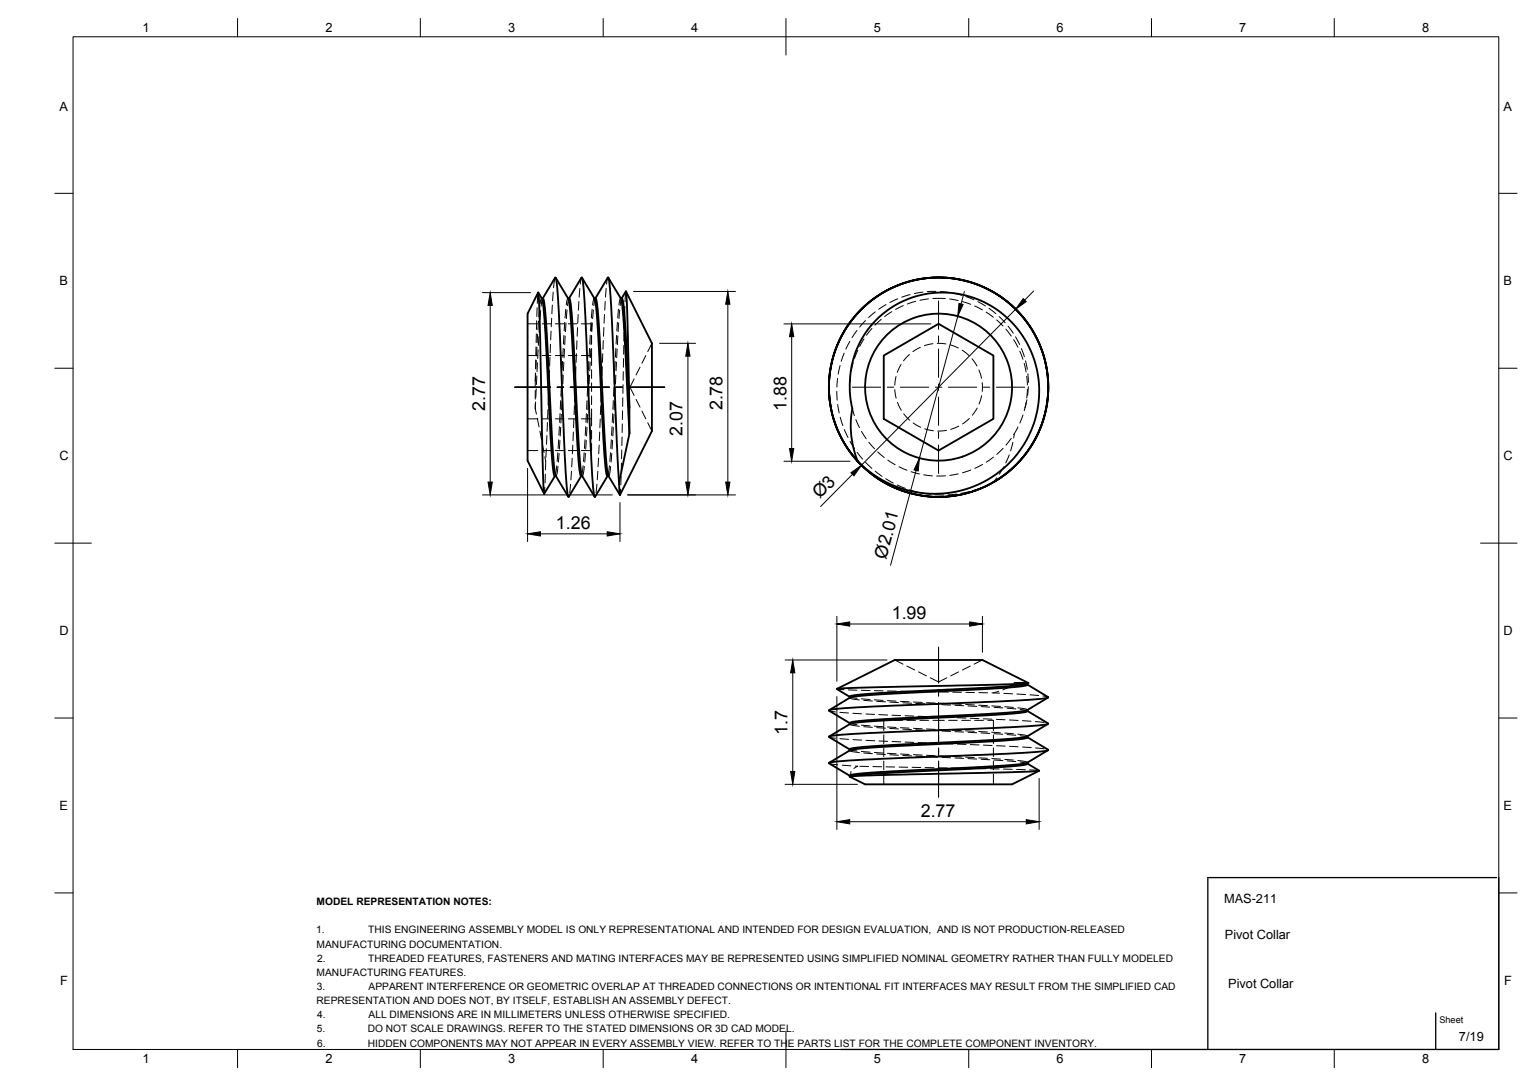
ISO-10303-21;
HEADER;
FILE_DESCRIPTION(
 (''),
 '2;1');
FILE_NAME ( 'Pivot Collar.step', '2026-10-05T20:07:59+06:00', ( '' ), ( '' ), 'STEP AP214', 'Unspecified', '' );
FILE_SCHEMA (('AUTOMOTIVE_DESIGN { 1 0 10303 214 3 1 1 }'));
ENDSEC;
DATA;
#10=MECHANICAL_DESIGN_GEOMETRIC_PRESENTATION_REPRESENTATION('',(#323),#196741);
#313=CONICAL_SURFACE('',#8812,0.119992720241923,1.10714871779409) ;
#314=CONICAL_SURFACE('',#8814,0.239985440483837,1.10714871779409) ;
#315=CONICAL_SURFACE('',#8815,0.199999999999988,1.10714871779409) ;
#323=STYLED_ITEM('',(#196765),#342) ;
#342=MANIFOLD_SOLID_BREP('Pivot Collar',#8719) ;
#369=PLANE('',#8817) ;
#370=PLANE('',#8818) ;
#371=PLANE('',#8819) ;
#372=PLANE('',#8820) ;
#373=PLANE('',#8821) ;
#374=PLANE('',#8822) ;
#375=PLANE('',#8823) ;
#376=PLANE('',#8824) ;
#564=FACE_BOUND('',#1412,.T.) ;
#631=CIRCLE('',#8806,1.21492637222366) ;
#632=CIRCLE('',#8811,1.21492629244945) ;
#633=CIRCLE('',#8813,0.599963601209611) ;
#634=CIRCLE('',#8816,1.00467112588555) ;
#832=B_SPLINE_SURFACE_WITH_KNOTS('',1,3,((#81592,#81593,#81594,#81595,#81596,
#81597,#81598,#81599,#81600,#81601,#81602,#81603,#81604,#81605,#81606,#81607,
#81608,#81609,#81610,#81611,#81612,#81613,#81614,#81615,#81616,#81617,#81618,
#81619,#81620,#81621,#81622,#81623,#81624,#81625,#81626,#81627,#81628,#81629,
#81630,#81631,#81632,#81633,#81634,#81635,#81636,#81637,#81638,#81639,#81640,
#81641,#81642,#81643,#81644,#81645,#81646,#81647,#81648,#81649,#81650,#81651,
#81652,#81653,#81654,#81655,#81656,#81657,#81658,#81659,#81660,#81661,#81662,
#81663,#81664,#81665,#81666,#81667,#81668,#81669,#81670,#81671,#81672,#81673,
#81674,#81675,#81676,#81677,#81678,#81679,#81680,#81681,#81682,#81683,#81684,
#81685,#81686,#81687,#81688,#81689,#81690,#81691,#81692,#81693,#81694,#81695,
#81696,#81697,#81698,#81699,#81700,#81701,#81702,#81703,#81704,#81705,#81706,
#81707,#81708,#81709,#81710,#81711,#81712,#81713,#81714,#81715,#81716,#81717,
#81718,#81719,#81720,#81721,#81722,#81723,#81724,#81725,#81726,#81727,#81728,
#81729,#81730,#81731,#81732,#81733,#81734,#81735,#81736,#81737,#81738,#81739,
#81740,#81741,#81742,#81743,#81744,#81745,#81746,#81747,#81748,#81749,#81750,
#81751,#81752,#81753,#81754,#81755,#81756,#81757,#81758,#81759,#81760,#81761,
#81762,#81763,#81764,#81765,#81766,#81767,#81768,#81769,#81770,#81771,#81772,
#81773,#81774,#81775,#81776,#81777,#81778,#81779,#81780,#81781,#81782,#81783,
#81784,#81785,#81786,#81787,#81788,#81789,#81790,#81791,#81792,#81793,#81794,
#81795,#81796,#81797,#81798,#81799,#81800,#81801,#81802,#81803,#81804,#81805,
#81806,#81807,#81808,#81809,#81810,#81811,#81812,#81813,#81814,#81815,#81816,
#81817,#81818,#81819,#81820,#81821,#81822,#81823,#81824,#81825,#81826,#81827,
#81828,#81829,#81830,#81831,#81832,#81833,#81834,#81835,#81836,#81837,#81838,
#81839,#81840,#81841,#81842,#81843,#81844,#81845,#81846,#81847,#81848,#81849,
#81850,#81851,#81852,#81853,#81854,#81855,#81856,#81857,#81858,#81859,#81860,
#81861,#81862,#81863,#81864,#81865,#81866,#81867,#81868,#81869,#81870,#81871,
#81872,#81873,#81874,#81875,#81876,#81877,#81878,#81879,#81880,#81881,#81882,
#81883,#81884,#81885,#81886,#81887,#81888,#81889,#81890,#81891,#81892,#81893,
#81894,#81895,#81896,#81897,#81898,#81899,#81900,#81901,#81902,#81903,#81904,
#81905,#81906,#81907,#81908,#81909,#81910,#81911,#81912,#81913,#81914,#81915,
#81916,#81917,#81918,#81919,#81920,#81921,#81922,#81923,#81924,#81925,#81926,
#81927,#81928,#81929,#81930,#81931,#81932,#81933,#81934,#81935,#81936,#81937,
#81938,#81939,#81940,#81941,#81942,#81943,#81944,#81945,#81946,#81947,#81948,
#81949,#81950,#81951,#81952,#81953,#81954,#81955,#81956,#81957,#81958,#81959,
#81960,#81961,#81962,#81963,#81964,#81965,#81966,#81967,#81968,#81969,#81970,
#81971,#81972,#81973,#81974,#81975,#81976,#81977,#81978,#81979,#81980,#81981,
#81982,#81983,#81984,#81985,#81986,#81987,#81988,#81989,#81990,#81991,#81992,
#81993,#81994,#81995,#81996,#81997,#81998,#81999,#82000,#82001,#82002,#82003,
#82004,#82005,#82006,#82007,#82008,#82009,#82010,#82011,#82012,#82013,#82014,
#82015,#82016,#82017,#82018,#82019,#82020,#82021,#82022,#82023,#82024,#82025,
#82026,#82027,#82028,#82029,#82030,#82031,#82032,#82033,#82034,#82035,#82036,
#82037,#82038,#82039,#82040,#82041,#82042,#82043,#82044,#82045,#82046,#82047,
#82048,#82049,#82050,#82051,#82052,#82053,#82054,#82055,#82056,#82057,#82058,
#82059,#82060,#82061,#82062,#82063,#82064,#82065,#82066,#82067,#82068,#82069,
#82070,#82071,#82072,#82073,#82074,#82075,#82076,#82077,#82078,#82079,#82080,
#82081,#82082,#82083,#82084,#82085,#82086,#82087,#82088,#82089,#82090,#82091,
#82092,#82093,#82094,#82095,#82096,#82097,#82098,#82099,#82100,#82101,#82102,
#82103,#82104,#82105,#82106,#82107,#82108,#82109,#82110,#82111,#82112,#82113,
#82114,#82115,#82116,#82117,#82118,#82119,#82120,#82121,#82122,#82123,#82124,
#82125,#82126,#82127,#82128,#82129,#82130,#82131,#82132,#82133,#82134,#82135,
#82136,#82137,#82138,#82139,#82140,#82141,#82142,#82143,#82144,#82145,#82146,
#82147,#82148,#82149,#82150,#82151,#82152,#82153,#82154,#82155,#82156,#82157,
#82158,#82159,#82160,#82161,#82162,#82163,#82164,#82165,#82166,#82167,#82168,
#82169,#82170,#82171,#82172,#82173,#82174,#82175,#82176,#82177,#82178,#82179,
#82180,#82181,#82182,#82183,#82184,#82185,#82186,#82187,#82188,#82189,#82190,
#82191,#82192,#82193,#82194,#82195,#82196,#82197,#82198,#82199,#82200,#82201,
#82202,#82203,#82204,#82205,#82206,#82207,#82208,#82209,#82210,#82211,#82212,
#82213,#82214,#82215,#82216,#82217,#82218,#82219,#82220,#82221,#82222,#82223,
#82224,#82225,#82226,#82227,#82228,#82229,#82230,#82231,#82232,#82233,#82234,
#82235,#82236,#82237,#82238,#82239,#82240,#82241,#82242,#82243,#82244,#82245,
#82246,#82247,#82248,#82249,#82250,#82251,#82252,#82253,#82254,#82255,#82256,
#82257,#82258,#82259,#82260,#82261,#82262,#82263,#82264,#82265,#82266,#82267,
#82268,#82269,#82270,#82271,#82272,#82273,#82274,#82275,#82276,#82277,#82278,
#82279,#82280,#82281,#82282,#82283,#82284,#82285,#82286,#82287,#82288,#82289,
#82290,#82291,#82292,#82293,#82294,#82295,#82296,#82297,#82298,#82299,#82300,
#82301,#82302,#82303,#82304,#82305,#82306,#82307,#82308,#82309,#82310,#82311,
#82312,#82313,#82314,#82315,#82316,#82317,#82318,#82319,#82320,#82321,#82322,
#82323,#82324,#82325,#82326,#82327,#82328,#82329,#82330,#82331,#82332,#82333,
#82334,#82335,#82336,#82337,#82338,#82339,#82340,#82341,#82342,#82343,#82344,
#82345,#82346,#82347,#82348,#82349,#82350,#82351,#82352,#82353,#82354,#82355,
#82356,#82357,#82358,#82359,#82360,#82361,#82362,#82363,#82364,#82365,#82366,
#82367,#82368,#82369,#82370,#82371,#82372,#82373,#82374,#82375,#82376,#82377,
#82378,#82379,#82380,#82381,#82382,#82383,#82384,#82385,#82386,#82387,#82388,
#82389,#82390,#82391,#82392,#82393,#82394,#82395,#82396,#82397,#82398,#82399,
#82400,#82401,#82402,#82403,#82404,#82405,#82406,#82407,#82408,#82409,#82410,
#82411,#82412,#82413,#82414,#82415,#82416,#82417,#82418,#82419,#82420,#82421,
#82422,#82423,#82424,#82425,#82426,#82427,#82428,#82429,#82430,#82431,#82432,
#82433,#82434,#82435,#82436,#82437,#82438,#82439,#82440,#82441,#82442,#82443,
#82444,#82445,#82446,#82447,#82448,#82449,#82450,#82451,#82452,#82453,#82454,
#82455,#82456,#82457,#82458,#82459,#82460,#82461,#82462,#82463,#82464,#82465,
#82466,#82467,#82468,#82469,#82470,#82471,#82472,#82473,#82474,#82475,#82476,
#82477,#82478,#82479,#82480,#82481,#82482,#82483,#82484,#82485,#82486,#82487,
#82488,#82489,#82490,#82491,#82492,#82493,#82494,#82495,#82496,#82497,#82498,
#82499,#82500,#82501,#82502,#82503,#82504,#82505,#82506,#82507,#82508,#82509,
#82510,#82511,#82512,#82513,#82514,#82515,#82516,#82517,#82518,#82519,#82520,
#82521,#82522,#82523,#82524,#82525,#82526,#82527,#82528,#82529,#82530,#82531,
#82532,#82533,#82534,#82535,#82536,#82537,#82538,#82539,#82540,#82541,#82542,
#82543,#82544,#82545,#82546,#82547,#82548,#82549,#82550,#82551,#82552,#82553,
#82554,#82555,#82556,#82557,#82558,#82559,#82560,#82561,#82562,#82563,#82564,
#82565,#82566,#82567,#82568,#82569,#82570,#82571,#82572,#82573,#82574,#82575,
#82576,#82577,#82578,#82579,#82580,#82581,#82582,#82583,#82584,#82585,#82586,
#82587,#82588,#82589,#82590,#82591,#82592,#82593,#82594,#82595,#82596,#82597,
#82598,#82599,#82600,#82601,#82602,#82603,#82604,#82605,#82606,#82607,#82608,
#82609,#82610,#82611,#82612,#82613,#82614,#82615,#82616,#82617,#82618,#82619,
#82620,#82621,#82622,#82623,#82624,#82625,#82626,#82627,#82628,#82629,#82630,
#82631,#82632,#82633,#82634,#82635,#82636,#82637,#82638,#82639,#82640,#82641,
#82642,#82643,#82644,#82645,#82646,#82647,#82648,#82649,#82650,#82651,#82652,
#82653,#82654,#82655,#82656,#82657,#82658,#82659,#82660,#82661,#82662,#82663,
#82664,#82665,#82666,#82667,#82668,#82669,#82670,#82671,#82672,#82673,#82674,
#82675,#82676,#82677,#82678,#82679,#82680,#82681,#82682,#82683,#82684,#82685,
#82686,#82687,#82688,#82689,#82690,#82691,#82692,#82693,#82694,#82695,#82696,
#82697,#82698,#82699,#82700,#82701,#82702,#82703,#82704,#82705,#82706,#82707,
#82708,#82709,#82710,#82711,#82712,#82713,#82714,#82715,#82716,#82717,#82718,
#82719,#82720,#82721,#82722,#82723,#82724,#82725,#82726,#82727,#82728,#82729,
#82730,#82731,#82732,#82733,#82734,#82735,#82736,#82737,#82738,#82739,#82740,
#82741,#82742,#82743,#82744,#82745,#82746,#82747,#82748,#82749,#82750,#82751,
#82752,#82753,#82754,#82755,#82756,#82757,#82758,#82759,#82760,#82761,#82762,
#82763,#82764,#82765,#82766,#82767,#82768,#82769,#82770,#82771,#82772,#82773,
#82774,#82775,#82776,#82777,#82778,#82779,#82780,#82781,#82782,#82783,#82784,
#82785,#82786,#82787,#82788,#82789,#82790,#82791,#82792,#82793,#82794,#82795,
#82796,#82797,#82798,#82799,#82800,#82801,#82802,#82803,#82804,#82805,#82806,
#82807,#82808,#82809,#82810,#82811,#82812,#82813,#82814,#82815,#82816,#82817,
#82818,#82819,#82820,#82821,#82822,#82823,#82824,#82825,#82826,#82827,#82828,
#82829,#82830,#82831,#82832,#82833,#82834,#82835,#82836,#82837,#82838,#82839,
#82840,#82841,#82842,#82843,#82844,#82845,#82846,#82847,#82848,#82849,#82850,
#82851,#82852,#82853,#82854,#82855,#82856,#82857,#82858,#82859,#82860,#82861,
#82862,#82863,#82864,#82865,#82866,#82867,#82868,#82869,#82870,#82871,#82872,
#82873,#82874,#82875,#82876,#82877,#82878,#82879,#82880,#82881,#82882,#82883,
#82884,#82885,#82886,#82887,#82888,#82889,#82890,#82891,#82892,#82893,#82894,
#82895,#82896,#82897,#82898,#82899,#82900,#82901,#82902,#82903,#82904,#82905,
#82906,#82907,#82908,#82909,#82910,#82911,#82912,#82913,#82914,#82915,#82916,
#82917,#82918,#82919,#82920,#82921,#82922,#82923,#82924,#82925,#82926,#82927,
#82928,#82929,#82930,#82931,#82932,#82933,#82934,#82935,#82936,#82937,#82938,
#82939,#82940,#82941,#82942,#82943,#82944,#82945,#82946,#82947,#82948,#82949,
#82950,#82951,#82952,#82953,#82954,#82955,#82956,#82957,#82958,#82959,#82960,
#82961,#82962,#82963,#82964,#82965,#82966,#82967,#82968,#82969,#82970,#82971,
#82972,#82973,#82974,#82975,#82976,#82977,#82978,#82979,#82980,#82981,#82982,
#82983,#82984,#82985,#82986,#82987,#82988,#82989,#82990,#82991,#82992,#82993,
#82994,#82995,#82996,#82997,#82998,#82999,#83000,#83001,#83002,#83003,#83004,
#83005,#83006,#83007,#83008,#83009,#83010,#83011,#83012,#83013,#83014,#83015,
#83016,#83017,#83018,#83019,#83020,#83021,#83022,#83023,#83024,#83025,#83026,
#83027,#83028,#83029,#83030,#83031,#83032,#83033,#83034,#83035,#83036,#83037,
#83038,#83039,#83040,#83041,#83042,#83043,#83044,#83045,#83046,#83047,#83048,
#83049,#83050,#83051,#83052,#83053,#83054,#83055,#83056,#83057,#83058,#83059,
#83060,#83061,#83062,#83063,#83064,#83065,#83066,#83067,#83068,#83069,#83070,
#83071,#83072,#83073,#83074,#83075,#83076,#83077,#83078,#83079,#83080,#83081,
#83082,#83083,#83084,#83085,#83086,#83087,#83088,#83089,#83090,#83091,#83092,
#83093,#83094,#83095,#83096,#83097,#83098,#83099,#83100,#83101,#83102,#83103,
#83104,#83105,#83106,#83107,#83108,#83109,#83110,#83111,#83112,#83113,#83114,
#83115,#83116,#83117,#83118,#83119,#83120,#83121,#83122,#83123,#83124,#83125,
#83126,#83127,#83128,#83129,#83130,#83131,#83132,#83133,#83134,#83135,#83136,
#83137,#83138,#83139,#83140,#83141,#83142,#83143,#83144,#83145,#83146,#83147,
#83148,#83149,#83150,#83151,#83152,#83153,#83154,#83155,#83156,#83157,#83158,
#83159,#83160,#83161,#83162,#83163,#83164,#83165,#83166,#83167,#83168,#83169,
#83170,#83171,#83172,#83173,#83174,#83175,#83176,#83177,#83178,#83179,#83180,
#83181,#83182,#83183,#83184,#83185,#83186,#83187,#83188,#83189,#83190,#83191,
#83192,#83193,#83194,#83195,#83196,#83197,#83198,#83199,#83200,#83201,#83202,
#83203,#83204,#83205,#83206,#83207,#83208,#83209,#83210,#83211,#83212,#83213,
#83214,#83215,#83216,#83217,#83218,#83219,#83220,#83221,#83222,#83223,#83224,
#83225,#83226,#83227,#83228,#83229,#83230,#83231,#83232,#83233,#83234,#83235,
#83236,#83237,#83238,#83239,#83240,#83241,#83242,#83243,#83244,#83245,#83246,
#83247,#83248,#83249,#83250,#83251,#83252,#83253,#83254,#83255,#83256,#83257,
#83258,#83259,#83260,#83261,#83262,#83263,#83264,#83265,#83266,#83267,#83268,
#83269,#83270,#83271,#83272,#83273,#83274,#83275,#83276,#83277,#83278,#83279,
#83280,#83281,#83282,#83283,#83284,#83285,#83286,#83287,#83288,#83289,#83290,
#83291,#83292,#83293,#83294,#83295,#83296,#83297,#83298,#83299,#83300,#83301,
#83302,#83303,#83304,#83305,#83306,#83307,#83308,#83309,#83310,#83311,#83312,
#83313,#83314,#83315,#83316,#83317,#83318,#83319,#83320,#83321,#83322,#83323,
#83324,#83325,#83326,#83327,#83328,#83329,#83330,#83331,#83332,#83333,#83334,
#83335,#83336,#83337,#83338,#83339,#83340,#83341,#83342,#83343,#83344,#83345,
#83346,#83347,#83348,#83349,#83350,#83351,#83352,#83353,#83354,#83355,#83356,
#83357,#83358,#83359,#83360,#83361,#83362,#83363,#83364,#83365,#83366,#83367,
#83368,#83369,#83370,#83371,#83372,#83373,#83374,#83375,#83376,#83377,#83378,
#83379,#83380,#83381,#83382,#83383,#83384,#83385,#83386,#83387,#83388,#83389,
#83390,#83391,#83392,#83393,#83394,#83395,#83396,#83397,#83398,#83399,#83400,
#83401,#83402,#83403,#83404,#83405,#83406,#83407,#83408,#83409,#83410,#83411,
#83412,#83413,#83414,#83415,#83416,#83417,#83418,#83419,#83420,#83421,#83422,
#83423,#83424,#83425,#83426,#83427,#83428,#83429,#83430,#83431,#83432,#83433,
#83434,#83435,#83436,#83437,#83438,#83439,#83440,#83441,#83442,#83443,#83444,
#83445,#83446,#83447,#83448,#83449,#83450,#83451,#83452,#83453,#83454,#83455,
#83456,#83457,#83458,#83459,#83460,#83461,#83462,#83463,#83464,#83465,#83466,
#83467,#83468,#83469,#83470,#83471,#83472,#83473,#83474,#83475,#83476,#83477,
#83478,#83479,#83480,#83481,#83482,#83483,#83484,#83485,#83486,#83487,#83488,
#83489,#83490,#83491,#83492,#83493,#83494,#83495,#83496,#83497,#83498,#83499,
#83500,#83501,#83502,#83503,#83504,#83505,#83506,#83507,#83508,#83509,#83510,
#83511,#83512,#83513,#83514,#83515,#83516,#83517,#83518,#83519,#83520,#83521,
#83522,#83523,#83524,#83525,#83526,#83527,#83528,#83529,#83530,#83531,#83532,
#83533,#83534,#83535,#83536,#83537,#83538,#83539,#83540,#83541,#83542,#83543,
#83544,#83545,#83546,#83547,#83548,#83549,#83550,#83551,#83552,#83553,#83554,
#83555,#83556,#83557,#83558,#83559,#83560,#83561,#83562,#83563,#83564,#83565,
#83566,#83567,#83568,#83569,#83570,#83571,#83572,#83573,#83574,#83575,#83576,
#83577,#83578,#83579,#83580,#83581,#83582,#83583,#83584,#83585,#83586,#83587,
#83588,#83589,#83590,#83591,#83592,#83593,#83594,#83595,#83596,#83597,#83598,
#83599,#83600,#83601,#83602,#83603,#83604,#83605,#83606,#83607,#83608,#83609,
#83610,#83611,#83612,#83613,#83614,#83615,#83616,#83617,#83618,#83619,#83620,
#83621,#83622,#83623,#83624,#83625,#83626,#83627,#83628,#83629,#83630,#83631,
#83632,#83633,#83634,#83635,#83636,#83637,#83638,#83639,#83640,#83641,#83642,
#83643,#83644,#83645,#83646,#83647,#83648,#83649,#83650,#83651,#83652,#83653,
#83654,#83655,#83656,#83657,#83658,#83659,#83660,#83661,#83662,#83663,#83664,
#83665,#83666,#83667,#83668,#83669,#83670,#83671,#83672,#83673,#83674,#83675,
#83676,#83677,#83678,#83679,#83680,#83681,#83682,#83683,#83684,#83685,#83686,
#83687,#83688,#83689,#83690,#83691,#83692,#83693,#83694,#83695,#83696,#83697,
#83698,#83699,#83700,#83701,#83702,#83703,#83704,#83705,#83706,#83707,#83708,
#83709,#83710,#83711,#83712,#83713,#83714,#83715,#83716,#83717,#83718,#83719,
#83720,#83721,#83722,#83723,#83724,#83725,#83726,#83727,#83728,#83729,#83730,
#83731,#83732,#83733,#83734,#83735,#83736,#83737,#83738,#83739,#83740,#83741,
#83742,#83743,#83744,#83745,#83746,#83747,#83748,#83749,#83750,#83751,#83752,
#83753,#83754,#83755,#83756,#83757,#83758,#83759,#83760,#83761,#83762,#83763,
#83764,#83765,#83766,#83767,#83768,#83769,#83770,#83771,#83772,#83773,#83774,
#83775,#83776,#83777,#83778,#83779,#83780,#83781,#83782,#83783,#83784,#83785,
#83786,#83787,#83788,#83789,#83790,#83791,#83792,#83793,#83794,#83795,#83796,
#83797,#83798,#83799,#83800,#83801,#83802,#83803,#83804,#83805,#83806,#83807,
#83808,#83809,#83810,#83811,#83812,#83813,#83814,#83815,#83816,#83817,#83818,
#83819,#83820,#83821,#83822,#83823,#83824,#83825,#83826,#83827,#83828,#83829,
#83830,#83831,#83832,#83833,#83834,#83835,#83836,#83837,#83838,#83839,#83840,
#83841,#83842,#83843,#83844,#83845,#83846,#83847,#83848,#83849,#83850,#83851,
#83852,#83853,#83854,#83855,#83856,#83857,#83858,#83859,#83860,#83861,#83862,
#83863,#83864,#83865,#83866,#83867,#83868,#83869,#83870,#83871,#83872,#83873,
#83874,#83875,#83876,#83877,#83878,#83879,#83880,#83881,#83882,#83883,#83884,
#83885,#83886,#83887,#83888,#83889,#83890,#83891,#83892,#83893,#83894,#83895,
#83896,#83897,#83898,#83899,#83900,#83901,#83902,#83903,#83904,#83905,#83906,
#83907,#83908,#83909,#83910,#83911,#83912,#83913,#83914,#83915,#83916,#83917,
#83918,#83919,#83920,#83921,#83922,#83923,#83924,#83925,#83926,#83927,#83928,
#83929,#83930,#83931,#83932,#83933,#83934,#83935,#83936,#83937,#83938,#83939,
#83940,#83941,#83942,#83943,#83944,#83945,#83946,#83947,#83948,#83949,#83950,
#83951,#83952,#83953,#83954,#83955,#83956,#83957,#83958,#83959,#83960,#83961,
#83962,#83963,#83964,#83965,#83966,#83967,#83968,#83969,#83970,#83971,#83972,
#83973,#83974,#83975,#83976,#83977,#83978,#83979,#83980,#83981,#83982,#83983,
#83984,#83985,#83986,#83987,#83988,#83989,#83990,#83991,#83992,#83993,#83994,
#83995,#83996,#83997,#83998,#83999,#84000,#84001,#84002,#84003,#84004,#84005,
#84006,#84007,#84008,#84009,#84010,#84011,#84012,#84013,#84014,#84015,#84016,
#84017,#84018,#84019,#84020,#84021,#84022,#84023,#84024,#84025,#84026,#84027,
#84028,#84029,#84030,#84031,#84032,#84033,#84034,#84035,#84036,#84037,#84038,
#84039,#84040,#84041,#84042,#84043,#84044,#84045,#84046,#84047,#84048,#84049,
#84050,#84051,#84052,#84053,#84054,#84055,#84056,#84057,#84058,#84059,#84060,
#84061,#84062,#84063,#84064,#84065,#84066,#84067,#84068,#84069,#84070,#84071,
#84072,#84073,#84074,#84075,#84076,#84077,#84078,#84079,#84080,#84081,#84082,
#84083,#84084,#84085,#84086,#84087,#84088,#84089,#84090,#84091,#84092,#84093,
#84094,#84095,#84096,#84097,#84098,#84099,#84100,#84101,#84102,#84103,#84104,
#84105,#84106,#84107,#84108,#84109,#84110,#84111,#84112,#84113,#84114,#84115,
#84116,#84117,#84118,#84119,#84120,#84121,#84122,#84123,#84124,#84125,#84126,
#84127,#84128,#84129,#84130,#84131,#84132,#84133,#84134,#84135,#84136,#84137,
#84138,#84139,#84140,#84141,#84142,#84143,#84144,#84145,#84146,#84147,#84148,
#84149,#84150,#84151,#84152,#84153,#84154,#84155,#84156,#84157,#84158,#84159,
#84160,#84161,#84162,#84163,#84164,#84165,#84166,#84167,#84168,#84169,#84170,
#84171,#84172,#84173,#84174,#84175,#84176,#84177,#84178,#84179,#84180,#84181,
#84182,#84183,#84184,#84185,#84186,#84187,#84188,#84189,#84190,#84191,#84192,
#84193,#84194,#84195,#84196,#84197,#84198,#84199,#84200,#84201,#84202,#84203,
#84204,#84205,#84206,#84207,#84208,#84209,#84210,#84211,#84212,#84213,#84214,
#84215,#84216,#84217,#84218,#84219,#84220,#84221,#84222,#84223,#84224,#84225,
#84226,#84227,#84228,#84229,#84230,#84231,#84232,#84233,#84234,#84235,#84236,
#84237,#84238,#84239,#84240,#84241,#84242,#84243,#84244,#84245,#84246,#84247,
#84248,#84249,#84250,#84251,#84252,#84253,#84254,#84255,#84256,#84257,#84258,
#84259,#84260,#84261,#84262,#84263,#84264,#84265,#84266,#84267,#84268,#84269,
#84270,#84271,#84272,#84273,#84274,#84275,#84276,#84277,#84278,#84279,#84280,
#84281,#84282,#84283,#84284,#84285,#84286,#84287,#84288,#84289,#84290,#84291,
#84292,#84293,#84294,#84295,#84296,#84297,#84298,#84299,#84300,#84301,#84302,
#84303,#84304,#84305,#84306,#84307,#84308,#84309,#84310,#84311,#84312,#84313,
#84314,#84315,#84316,#84317,#84318,#84319,#84320,#84321,#84322,#84323,#84324,
#84325,#84326,#84327,#84328,#84329,#84330,#84331,#84332,#84333,#84334,#84335,
#84336,#84337,#84338,#84339,#84340,#84341,#84342,#84343,#84344,#84345,#84346,
#84347,#84348,#84349,#84350,#84351,#84352,#84353,#84354,#84355,#84356,#84357,
#84358,#84359,#84360,#84361,#84362,#84363,#84364,#84365,#84366,#84367,#84368,
#84369,#84370,#84371,#84372,#84373,#84374,#84375,#84376,#84377,#84378,#84379,
#84380,#84381,#84382,#84383,#84384,#84385,#84386,#84387,#84388,#84389,#84390,
#84391,#84392,#84393,#84394,#84395,#84396,#84397,#84398,#84399,#84400,#84401,
#84402,#84403,#84404,#84405,#84406,#84407,#84408,#84409,#84410,#84411,#84412,
#84413,#84414,#84415,#84416,#84417,#84418,#84419,#84420,#84421,#84422,#84423,
#84424,#84425,#84426,#84427,#84428,#84429,#84430,#84431,#84432,#84433,#84434,
#84435,#84436,#84437,#84438,#84439,#84440,#84441,#84442,#84443,#84444,#84445,
#84446,#84447,#84448,#84449,#84450,#84451,#84452,#84453,#84454,#84455,#84456,
#84457,#84458,#84459,#84460,#84461,#84462,#84463,#84464,#84465,#84466,#84467,
#84468,#84469,#84470,#84471,#84472,#84473,#84474,#84475,#84476,#84477,#84478,
#84479,#84480,#84481,#84482,#84483,#84484,#84485,#84486,#84487,#84488,#84489,
#84490,#84491,#84492,#84493,#84494,#84495,#84496,#84497,#84498,#84499,#84500,
#84501,#84502,#84503,#84504,#84505,#84506,#84507,#84508,#84509,#84510,#84511,
#84512,#84513,#84514,#84515,#84516,#84517,#84518,#84519,#84520,#84521,#84522,
#84523,#84524,#84525,#84526,#84527,#84528,#84529,#84530,#84531,#84532,#84533,
#84534,#84535,#84536,#84537,#84538,#84539,#84540,#84541,#84542,#84543,#84544,
#84545,#84546,#84547,#84548,#84549,#84550,#84551,#84552,#84553,#84554,#84555,
#84556,#84557,#84558,#84559,#84560,#84561,#84562,#84563,#84564,#84565,#84566,
#84567,#84568,#84569,#84570,#84571,#84572,#84573,#84574,#84575,#84576,#84577,
#84578,#84579,#84580,#84581,#84582,#84583,#84584,#84585,#84586,#84587,#84588,
#84589,#84590,#84591,#84592,#84593,#84594,#84595,#84596,#84597,#84598,#84599,
#84600,#84601,#84602,#84603,#84604,#84605,#84606,#84607,#84608,#84609,#84610,
#84611,#84612,#84613,#84614,#84615,#84616,#84617,#84618,#84619,#84620,#84621,
#84622,#84623,#84624,#84625,#84626,#84627,#84628,#84629,#84630,#84631,#84632,
#84633,#84634,#84635,#84636,#84637,#84638,#84639,#84640,#84641,#84642,#84643,
#84644,#84645,#84646,#84647,#84648,#84649,#84650,#84651,#84652,#84653,#84654,
#84655,#84656,#84657,#84658,#84659,#84660,#84661,#84662,#84663,#84664,#84665,
#84666,#84667,#84668,#84669,#84670,#84671,#84672,#84673,#84674,#84675,#84676,
#84677,#84678,#84679,#84680,#84681,#84682,#84683,#84684,#84685,#84686,#84687,
#84688,#84689,#84690,#84691,#84692,#84693,#84694,#84695,#84696,#84697,#84698,
#84699,#84700,#84701,#84702,#84703,#84704,#84705,#84706,#84707,#84708,#84709,
#84710,#84711,#84712,#84713,#84714,#84715,#84716,#84717,#84718,#84719,#84720,
#84721,#84722,#84723,#84724,#84725,#84726,#84727,#84728,#84729,#84730,#84731,
#84732,#84733,#84734,#84735,#84736,#84737,#84738,#84739,#84740,#84741,#84742,
#84743,#84744,#84745,#84746,#84747,#84748,#84749,#84750,#84751,#84752,#84753,
#84754,#84755,#84756,#84757,#84758,#84759,#84760,#84761,#84762,#84763,#84764,
#84765,#84766,#84767,#84768,#84769,#84770,#84771,#84772,#84773,#84774,#84775,
#84776,#84777,#84778,#84779,#84780,#84781,#84782,#84783,#84784,#84785,#84786,
#84787,#84788,#84789,#84790,#84791,#84792,#84793,#84794,#84795,#84796,#84797,
#84798,#84799,#84800,#84801,#84802,#84803,#84804,#84805,#84806,#84807,#84808,
#84809,#84810,#84811,#84812,#84813,#84814,#84815,#84816,#84817,#84818,#84819,
#84820,#84821,#84822,#84823,#84824,#84825,#84826,#84827,#84828,#84829,#84830,
#84831,#84832,#84833,#84834,#84835,#84836,#84837,#84838,#84839,#84840,#84841,
#84842,#84843,#84844,#84845,#84846,#84847,#84848,#84849,#84850,#84851,#84852,
#84853,#84854,#84855,#84856,#84857,#84858,#84859,#84860,#84861,#84862,#84863,
#84864,#84865,#84866,#84867,#84868,#84869,#84870,#84871,#84872,#84873,#84874,
#84875,#84876,#84877,#84878,#84879,#84880,#84881,#84882,#84883,#84884,#84885,
#84886,#84887,#84888,#84889,#84890,#84891,#84892,#84893,#84894,#84895,#84896,
#84897,#84898,#84899,#84900,#84901,#84902,#84903,#84904,#84905,#84906,#84907,
#84908,#84909,#84910,#84911,#84912,#84913,#84914,#84915,#84916,#84917,#84918,
#84919,#84920,#84921,#84922,#84923,#84924,#84925,#84926,#84927,#84928,#84929,
#84930,#84931,#84932,#84933,#84934,#84935,#84936,#84937,#84938,#84939,#84940,
#84941,#84942,#84943,#84944,#84945,#84946,#84947,#84948,#84949,#84950,#84951,
#84952,#84953,#84954,#84955,#84956,#84957,#84958,#84959,#84960,#84961,#84962,
#84963,#84964,#84965,#84966,#84967,#84968,#84969,#84970,#84971,#84972,#84973,
#84974,#84975,#84976,#84977,#84978,#84979,#84980,#84981,#84982,#84983,#84984,
#84985,#84986,#84987,#84988,#84989,#84990,#84991,#84992,#84993,#84994,#84995,
#84996,#84997,#84998,#84999,#85000,#85001,#85002,#85003,#85004,#85005,#85006,
#85007,#85008,#85009,#85010,#85011,#85012,#85013,#85014,#85015,#85016,#85017,
#85018,#85019,#85020,#85021,#85022,#85023,#85024,#85025,#85026,#85027,#85028,
#85029,#85030,#85031,#85032,#85033,#85034,#85035,#85036,#85037,#85038,#85039,
#85040,#85041,#85042,#85043,#85044,#85045,#85046,#85047,#85048,#85049,#85050,
#85051,#85052,#85053,#85054,#85055,#85056,#85057,#85058,#85059,#85060,#85061,
#85062,#85063,#85064,#85065,#85066,#85067,#85068,#85069,#85070,#85071,#85072,
#85073,#85074,#85075,#85076),(#85077,#85078,#85079,#85080,#85081,#85082,
#85083,#85084,#85085,#85086,#85087,#85088,#85089,#85090,#85091,#85092,#85093,
#85094,#85095,#85096,#85097,#85098,#85099,#85100,#85101,#85102,#85103,#85104,
#85105,#85106,#85107,#85108,#85109,#85110,#85111,#85112,#85113,#85114,#85115,
#85116,#85117,#85118,#85119,#85120,#85121,#85122,#85123,#85124,#85125,#85126,
#85127,#85128,#85129,#85130,#85131,#85132,#85133,#85134,#85135,#85136,#85137,
#85138,#85139,#85140,#85141,#85142,#85143,#85144,#85145,#85146,#85147,#85148,
#85149,#85150,#85151,#85152,#85153,#85154,#85155,#85156,#85157,#85158,#85159,
#85160,#85161,#85162,#85163,#85164,#85165,#85166,#85167,#85168,#85169,#85170,
#85171,#85172,#85173,#85174,#85175,#85176,#85177,#85178,#85179,#85180,#85181,
#85182,#85183,#85184,#85185,#85186,#85187,#85188,#85189,#85190,#85191,#85192,
#85193,#85194,#85195,#85196,#85197,#85198,#85199,#85200,#85201,#85202,#85203,
#85204,#85205,#85206,#85207,#85208,#85209,#85210,#85211,#85212,#85213,#85214,
#85215,#85216,#85217,#85218,#85219,#85220,#85221,#85222,#85223,#85224,#85225,
#85226,#85227,#85228,#85229,#85230,#85231,#85232,#85233,#85234,#85235,#85236,
#85237,#85238,#85239,#85240,#85241,#85242,#85243,#85244,#85245,#85246,#85247,
#85248,#85249,#85250,#85251,#85252,#85253,#85254,#85255,#85256,#85257,#85258,
#85259,#85260,#85261,#85262,#85263,#85264,#85265,#85266,#85267,#85268,#85269,
#85270,#85271,#85272,#85273,#85274,#85275,#85276,#85277,#85278,#85279,#85280,
#85281,#85282,#85283,#85284,#85285,#85286,#85287,#85288,#85289,#85290,#85291,
#85292,#85293,#85294,#85295,#85296,#85297,#85298,#85299,#85300,#85301,#85302,
#85303,#85304,#85305,#85306,#85307,#85308,#85309,#85310,#85311,#85312,#85313,
#85314,#85315,#85316,#85317,#85318,#85319,#85320,#85321,#85322,#85323,#85324,
#85325,#85326,#85327,#85328,#85329,#85330,#85331,#85332,#85333,#85334,#85335,
#85336,#85337,#85338,#85339,#85340,#85341,#85342,#85343,#85344,#85345,#85346,
#85347,#85348,#85349,#85350,#85351,#85352,#85353,#85354,#85355,#85356,#85357,
#85358,#85359,#85360,#85361,#85362,#85363,#85364,#85365,#85366,#85367,#85368,
#85369,#85370,#85371,#85372,#85373,#85374,#85375,#85376,#85377,#85378,#85379,
#85380,#85381,#85382,#85383,#85384,#85385,#85386,#85387,#85388,#85389,#85390,
#85391,#85392,#85393,#85394,#85395,#85396,#85397,#85398,#85399,#85400,#85401,
#85402,#85403,#85404,#85405,#85406,#85407,#85408,#85409,#85410,#85411,#85412,
#85413,#85414,#85415,#85416,#85417,#85418,#85419,#85420,#85421,#85422,#85423,
#85424,#85425,#85426,#85427,#85428,#85429,#85430,#85431,#85432,#85433,#85434,
#85435,#85436,#85437,#85438,#85439,#85440,#85441,#85442,#85443,#85444,#85445,
#85446,#85447,#85448,#85449,#85450,#85451,#85452,#85453,#85454,#85455,#85456,
#85457,#85458,#85459,#85460,#85461,#85462,#85463,#85464,#85465,#85466,#85467,
#85468,#85469,#85470,#85471,#85472,#85473,#85474,#85475,#85476,#85477,#85478,
#85479,#85480,#85481,#85482,#85483,#85484,#85485,#85486,#85487,#85488,#85489,
#85490,#85491,#85492,#85493,#85494,#85495,#85496,#85497,#85498,#85499,#85500,
#85501,#85502,#85503,#85504,#85505,#85506,#85507,#85508,#85509,#85510,#85511,
#85512,#85513,#85514,#85515,#85516,#85517,#85518,#85519,#85520,#85521,#85522,
#85523,#85524,#85525,#85526,#85527,#85528,#85529,#85530,#85531,#85532,#85533,
#85534,#85535,#85536,#85537,#85538,#85539,#85540,#85541,#85542,#85543,#85544,
#85545,#85546,#85547,#85548,#85549,#85550,#85551,#85552,#85553,#85554,#85555,
#85556,#85557,#85558,#85559,#85560,#85561,#85562,#85563,#85564,#85565,#85566,
#85567,#85568,#85569,#85570,#85571,#85572,#85573,#85574,#85575,#85576,#85577,
#85578,#85579,#85580,#85581,#85582,#85583,#85584,#85585,#85586,#85587,#85588,
#85589,#85590,#85591,#85592,#85593,#85594,#85595,#85596,#85597,#85598,#85599,
#85600,#85601,#85602,#85603,#85604,#85605,#85606,#85607,#85608,#85609,#85610,
#85611,#85612,#85613,#85614,#85615,#85616,#85617,#85618,#85619,#85620,#85621,
#85622,#85623,#85624,#85625,#85626,#85627,#85628,#85629,#85630,#85631,#85632,
#85633,#85634,#85635,#85636,#85637,#85638,#85639,#85640,#85641,#85642,#85643,
#85644,#85645,#85646,#85647,#85648,#85649,#85650,#85651,#85652,#85653,#85654,
#85655,#85656,#85657,#85658,#85659,#85660,#85661,#85662,#85663,#85664,#85665,
#85666,#85667,#85668,#85669,#85670,#85671,#85672,#85673,#85674,#85675,#85676,
#85677,#85678,#85679,#85680,#85681,#85682,#85683,#85684,#85685,#85686,#85687,
#85688,#85689,#85690,#85691,#85692,#85693,#85694,#85695,#85696,#85697,#85698,
#85699,#85700,#85701,#85702,#85703,#85704,#85705,#85706,#85707,#85708,#85709,
#85710,#85711,#85712,#85713,#85714,#85715,#85716,#85717,#85718,#85719,#85720,
#85721,#85722,#85723,#85724,#85725,#85726,#85727,#85728,#85729,#85730,#85731,
#85732,#85733,#85734,#85735,#85736,#85737,#85738,#85739,#85740,#85741,#85742,
#85743,#85744,#85745,#85746,#85747,#85748,#85749,#85750,#85751,#85752,#85753,
#85754,#85755,#85756,#85757,#85758,#85759,#85760,#85761,#85762,#85763,#85764,
#85765,#85766,#85767,#85768,#85769,#85770,#85771,#85772,#85773,#85774,#85775,
#85776,#85777,#85778,#85779,#85780,#85781,#85782,#85783,#85784,#85785,#85786,
#85787,#85788,#85789,#85790,#85791,#85792,#85793,#85794,#85795,#85796,#85797,
#85798,#85799,#85800,#85801,#85802,#85803,#85804,#85805,#85806,#85807,#85808,
#85809,#85810,#85811,#85812,#85813,#85814,#85815,#85816,#85817,#85818,#85819,
#85820,#85821,#85822,#85823,#85824,#85825,#85826,#85827,#85828,#85829,#85830,
#85831,#85832,#85833,#85834,#85835,#85836,#85837,#85838,#85839,#85840,#85841,
#85842,#85843,#85844,#85845,#85846,#85847,#85848,#85849,#85850,#85851,#85852,
#85853,#85854,#85855,#85856,#85857,#85858,#85859,#85860,#85861,#85862,#85863,
#85864,#85865,#85866,#85867,#85868,#85869,#85870,#85871,#85872,#85873,#85874,
#85875,#85876,#85877,#85878,#85879,#85880,#85881,#85882,#85883,#85884,#85885,
#85886,#85887,#85888,#85889,#85890,#85891,#85892,#85893,#85894,#85895,#85896,
#85897,#85898,#85899,#85900,#85901,#85902,#85903,#85904,#85905,#85906,#85907,
#85908,#85909,#85910,#85911,#85912,#85913,#85914,#85915,#85916,#85917,#85918,
#85919,#85920,#85921,#85922,#85923,#85924,#85925,#85926,#85927,#85928,#85929,
#85930,#85931,#85932,#85933,#85934,#85935,#85936,#85937,#85938,#85939,#85940,
#85941,#85942,#85943,#85944,#85945,#85946,#85947,#85948,#85949,#85950,#85951,
#85952,#85953,#85954,#85955,#85956,#85957,#85958,#85959,#85960,#85961,#85962,
#85963,#85964,#85965,#85966,#85967,#85968,#85969,#85970,#85971,#85972,#85973,
#85974,#85975,#85976,#85977,#85978,#85979,#85980,#85981,#85982,#85983,#85984,
#85985,#85986,#85987,#85988,#85989,#85990,#85991,#85992,#85993,#85994,#85995,
#85996,#85997,#85998,#85999,#86000,#86001,#86002,#86003,#86004,#86005,#86006,
#86007,#86008,#86009,#86010,#86011,#86012,#86013,#86014,#86015,#86016,#86017,
#86018,#86019,#86020,#86021,#86022,#86023,#86024,#86025,#86026,#86027,#86028,
#86029,#86030,#86031,#86032,#86033,#86034,#86035,#86036,#86037,#86038,#86039,
#86040,#86041,#86042,#86043,#86044,#86045,#86046,#86047,#86048,#86049,#86050,
#86051,#86052,#86053,#86054,#86055,#86056,#86057,#86058,#86059,#86060,#86061,
#86062,#86063,#86064,#86065,#86066,#86067,#86068,#86069,#86070,#86071,#86072,
#86073,#86074,#86075,#86076,#86077,#86078,#86079,#86080,#86081,#86082,#86083,
#86084,#86085,#86086,#86087,#86088,#86089,#86090,#86091,#86092,#86093,#86094,
#86095,#86096,#86097,#86098,#86099,#86100,#86101,#86102,#86103,#86104,#86105,
#86106,#86107,#86108,#86109,#86110,#86111,#86112,#86113,#86114,#86115,#86116,
#86117,#86118,#86119,#86120,#86121,#86122,#86123,#86124,#86125,#86126,#86127,
#86128,#86129,#86130,#86131,#86132,#86133,#86134,#86135,#86136,#86137,#86138,
#86139,#86140,#86141,#86142,#86143,#86144,#86145,#86146,#86147,#86148,#86149,
#86150,#86151,#86152,#86153,#86154,#86155,#86156,#86157,#86158,#86159,#86160,
#86161,#86162,#86163,#86164,#86165,#86166,#86167,#86168,#86169,#86170,#86171,
#86172,#86173,#86174,#86175,#86176,#86177,#86178,#86179,#86180,#86181,#86182,
#86183,#86184,#86185,#86186,#86187,#86188,#86189,#86190,#86191,#86192,#86193,
#86194,#86195,#86196,#86197,#86198,#86199,#86200,#86201,#86202,#86203,#86204,
#86205,#86206,#86207,#86208,#86209,#86210,#86211,#86212,#86213,#86214,#86215,
#86216,#86217,#86218,#86219,#86220,#86221,#86222,#86223,#86224,#86225,#86226,
#86227,#86228,#86229,#86230,#86231,#86232,#86233,#86234,#86235,#86236,#86237,
#86238,#86239,#86240,#86241,#86242,#86243,#86244,#86245,#86246,#86247,#86248,
#86249,#86250,#86251,#86252,#86253,#86254,#86255,#86256,#86257,#86258,#86259,
#86260,#86261,#86262,#86263,#86264,#86265,#86266,#86267,#86268,#86269,#86270,
#86271,#86272,#86273,#86274,#86275,#86276,#86277,#86278,#86279,#86280,#86281,
#86282,#86283,#86284,#86285,#86286,#86287,#86288,#86289,#86290,#86291,#86292,
#86293,#86294,#86295,#86296,#86297,#86298,#86299,#86300,#86301,#86302,#86303,
#86304,#86305,#86306,#86307,#86308,#86309,#86310,#86311,#86312,#86313,#86314,
#86315,#86316,#86317,#86318,#86319,#86320,#86321,#86322,#86323,#86324,#86325,
#86326,#86327,#86328,#86329,#86330,#86331,#86332,#86333,#86334,#86335,#86336,
#86337,#86338,#86339,#86340,#86341,#86342,#86343,#86344,#86345,#86346,#86347,
#86348,#86349,#86350,#86351,#86352,#86353,#86354,#86355,#86356,#86357,#86358,
#86359,#86360,#86361,#86362,#86363,#86364,#86365,#86366,#86367,#86368,#86369,
#86370,#86371,#86372,#86373,#86374,#86375,#86376,#86377,#86378,#86379,#86380,
#86381,#86382,#86383,#86384,#86385,#86386,#86387,#86388,#86389,#86390,#86391,
#86392,#86393,#86394,#86395,#86396,#86397,#86398,#86399,#86400,#86401,#86402,
#86403,#86404,#86405,#86406,#86407,#86408,#86409,#86410,#86411,#86412,#86413,
#86414,#86415,#86416,#86417,#86418,#86419,#86420,#86421,#86422,#86423,#86424,
#86425,#86426,#86427,#86428,#86429,#86430,#86431,#86432,#86433,#86434,#86435,
#86436,#86437,#86438,#86439,#86440,#86441,#86442,#86443,#86444,#86445,#86446,
#86447,#86448,#86449,#86450,#86451,#86452,#86453,#86454,#86455,#86456,#86457,
#86458,#86459,#86460,#86461,#86462,#86463,#86464,#86465,#86466,#86467,#86468,
#86469,#86470,#86471,#86472,#86473,#86474,#86475,#86476,#86477,#86478,#86479,
#86480,#86481,#86482,#86483,#86484,#86485,#86486,#86487,#86488,#86489,#86490,
#86491,#86492,#86493,#86494,#86495,#86496,#86497,#86498,#86499,#86500,#86501,
#86502,#86503,#86504,#86505,#86506,#86507,#86508,#86509,#86510,#86511,#86512,
#86513,#86514,#86515,#86516,#86517,#86518,#86519,#86520,#86521,#86522,#86523,
#86524,#86525,#86526,#86527,#86528,#86529,#86530,#86531,#86532,#86533,#86534,
#86535,#86536,#86537,#86538,#86539,#86540,#86541,#86542,#86543,#86544,#86545,
#86546,#86547,#86548,#86549,#86550,#86551,#86552,#86553,#86554,#86555,#86556,
#86557,#86558,#86559,#86560,#86561,#86562,#86563,#86564,#86565,#86566,#86567,
#86568,#86569,#86570,#86571,#86572,#86573,#86574,#86575,#86576,#86577,#86578,
#86579,#86580,#86581,#86582,#86583,#86584,#86585,#86586,#86587,#86588,#86589,
#86590,#86591,#86592,#86593,#86594,#86595,#86596,#86597,#86598,#86599,#86600,
#86601,#86602,#86603,#86604,#86605,#86606,#86607,#86608,#86609,#86610,#86611,
#86612,#86613,#86614,#86615,#86616,#86617,#86618,#86619,#86620,#86621,#86622,
#86623,#86624,#86625,#86626,#86627,#86628,#86629,#86630,#86631,#86632,#86633,
#86634,#86635,#86636,#86637,#86638,#86639,#86640,#86641,#86642,#86643,#86644,
#86645,#86646,#86647,#86648,#86649,#86650,#86651,#86652,#86653,#86654,#86655,
#86656,#86657,#86658,#86659,#86660,#86661,#86662,#86663,#86664,#86665,#86666,
#86667,#86668,#86669,#86670,#86671,#86672,#86673,#86674,#86675,#86676,#86677,
#86678,#86679,#86680,#86681,#86682,#86683,#86684,#86685,#86686,#86687,#86688,
#86689,#86690,#86691,#86692,#86693,#86694,#86695,#86696,#86697,#86698,#86699,
#86700,#86701,#86702,#86703,#86704,#86705,#86706,#86707,#86708,#86709,#86710,
#86711,#86712,#86713,#86714,#86715,#86716,#86717,#86718,#86719,#86720,#86721,
#86722,#86723,#86724,#86725,#86726,#86727,#86728,#86729,#86730,#86731,#86732,
#86733,#86734,#86735,#86736,#86737,#86738,#86739,#86740,#86741,#86742,#86743,
#86744,#86745,#86746,#86747,#86748,#86749,#86750,#86751,#86752,#86753,#86754,
#86755,#86756,#86757,#86758,#86759,#86760,#86761,#86762,#86763,#86764,#86765,
#86766,#86767,#86768,#86769,#86770,#86771,#86772,#86773,#86774,#86775,#86776,
#86777,#86778,#86779,#86780,#86781,#86782,#86783,#86784,#86785,#86786,#86787,
#86788,#86789,#86790,#86791,#86792,#86793,#86794,#86795,#86796,#86797,#86798,
#86799,#86800,#86801,#86802,#86803,#86804,#86805,#86806,#86807,#86808,#86809,
#86810,#86811,#86812,#86813,#86814,#86815,#86816,#86817,#86818,#86819,#86820,
#86821,#86822,#86823,#86824,#86825,#86826,#86827,#86828,#86829,#86830,#86831,
#86832,#86833,#86834,#86835,#86836,#86837,#86838,#86839,#86840,#86841,#86842,
#86843,#86844,#86845,#86846,#86847,#86848,#86849,#86850,#86851,#86852,#86853,
#86854,#86855,#86856,#86857,#86858,#86859,#86860,#86861,#86862,#86863,#86864,
#86865,#86866,#86867,#86868,#86869,#86870,#86871,#86872,#86873,#86874,#86875,
#86876,#86877,#86878,#86879,#86880,#86881,#86882,#86883,#86884,#86885,#86886,
#86887,#86888,#86889,#86890,#86891,#86892,#86893,#86894,#86895,#86896,#86897,
#86898,#86899,#86900,#86901,#86902,#86903,#86904,#86905,#86906,#86907,#86908,
#86909,#86910,#86911,#86912,#86913,#86914,#86915,#86916,#86917,#86918,#86919,
#86920,#86921,#86922,#86923,#86924,#86925,#86926,#86927,#86928,#86929,#86930,
#86931,#86932,#86933,#86934,#86935,#86936,#86937,#86938,#86939,#86940,#86941,
#86942,#86943,#86944,#86945,#86946,#86947,#86948,#86949,#86950,#86951,#86952,
#86953,#86954,#86955,#86956,#86957,#86958,#86959,#86960,#86961,#86962,#86963,
#86964,#86965,#86966,#86967,#86968,#86969,#86970,#86971,#86972,#86973,#86974,
#86975,#86976,#86977,#86978,#86979,#86980,#86981,#86982,#86983,#86984,#86985,
#86986,#86987,#86988,#86989,#86990,#86991,#86992,#86993,#86994,#86995,#86996,
#86997,#86998,#86999,#87000,#87001,#87002,#87003,#87004,#87005,#87006,#87007,
#87008,#87009,#87010,#87011,#87012,#87013,#87014,#87015,#87016,#87017,#87018,
#87019,#87020,#87021,#87022,#87023,#87024,#87025,#87026,#87027,#87028,#87029,
#87030,#87031,#87032,#87033,#87034,#87035,#87036,#87037,#87038,#87039,#87040,
#87041,#87042,#87043,#87044,#87045,#87046,#87047,#87048,#87049,#87050,#87051,
#87052,#87053,#87054,#87055,#87056,#87057,#87058,#87059,#87060,#87061,#87062,
#87063,#87064,#87065,#87066,#87067,#87068,#87069,#87070,#87071,#87072,#87073,
#87074,#87075,#87076,#87077,#87078,#87079,#87080,#87081,#87082,#87083,#87084,
#87085,#87086,#87087,#87088,#87089,#87090,#87091,#87092,#87093,#87094,#87095,
#87096,#87097,#87098,#87099,#87100,#87101,#87102,#87103,#87104,#87105,#87106,
#87107,#87108,#87109,#87110,#87111,#87112,#87113,#87114,#87115,#87116,#87117,
#87118,#87119,#87120,#87121,#87122,#87123,#87124,#87125,#87126,#87127,#87128,
#87129,#87130,#87131,#87132,#87133,#87134,#87135,#87136,#87137,#87138,#87139,
#87140,#87141,#87142,#87143,#87144,#87145,#87146,#87147,#87148,#87149,#87150,
#87151,#87152,#87153,#87154,#87155,#87156,#87157,#87158,#87159,#87160,#87161,
#87162,#87163,#87164,#87165,#87166,#87167,#87168,#87169,#87170,#87171,#87172,
#87173,#87174,#87175,#87176,#87177,#87178,#87179,#87180,#87181,#87182,#87183,
#87184,#87185,#87186,#87187,#87188,#87189,#87190,#87191,#87192,#87193,#87194,
#87195,#87196,#87197,#87198,#87199,#87200,#87201,#87202,#87203,#87204,#87205,
#87206,#87207,#87208,#87209,#87210,#87211,#87212,#87213,#87214,#87215,#87216,
#87217,#87218,#87219,#87220,#87221,#87222,#87223,#87224,#87225,#87226,#87227,
#87228,#87229,#87230,#87231,#87232,#87233,#87234,#87235,#87236,#87237,#87238,
#87239,#87240,#87241,#87242,#87243,#87244,#87245,#87246,#87247,#87248,#87249,
#87250,#87251,#87252,#87253,#87254,#87255,#87256,#87257,#87258,#87259,#87260,
#87261,#87262,#87263,#87264,#87265,#87266,#87267,#87268,#87269,#87270,#87271,
#87272,#87273,#87274,#87275,#87276,#87277,#87278,#87279,#87280,#87281,#87282,
#87283,#87284,#87285,#87286,#87287,#87288,#87289,#87290,#87291,#87292,#87293,
#87294,#87295,#87296,#87297,#87298,#87299,#87300,#87301,#87302,#87303,#87304,
#87305,#87306,#87307,#87308,#87309,#87310,#87311,#87312,#87313,#87314,#87315,
#87316,#87317,#87318,#87319,#87320,#87321,#87322,#87323,#87324,#87325,#87326,
#87327,#87328,#87329,#87330,#87331,#87332,#87333,#87334,#87335,#87336,#87337,
#87338,#87339,#87340,#87341,#87342,#87343,#87344,#87345,#87346,#87347,#87348,
#87349,#87350,#87351,#87352,#87353,#87354,#87355,#87356,#87357,#87358,#87359,
#87360,#87361,#87362,#87363,#87364,#87365,#87366,#87367,#87368,#87369,#87370,
#87371,#87372,#87373,#87374,#87375,#87376,#87377,#87378,#87379,#87380,#87381,
#87382,#87383,#87384,#87385,#87386,#87387,#87388,#87389,#87390,#87391,#87392,
#87393,#87394,#87395,#87396,#87397,#87398,#87399,#87400,#87401,#87402,#87403,
#87404,#87405,#87406,#87407,#87408,#87409,#87410,#87411,#87412,#87413,#87414,
#87415,#87416,#87417,#87418,#87419,#87420,#87421,#87422,#87423,#87424,#87425,
#87426,#87427,#87428,#87429,#87430,#87431,#87432,#87433,#87434,#87435,#87436,
#87437,#87438,#87439,#87440,#87441,#87442,#87443,#87444,#87445,#87446,#87447,
#87448,#87449,#87450,#87451,#87452,#87453,#87454,#87455,#87456,#87457,#87458,
#87459,#87460,#87461,#87462,#87463,#87464,#87465,#87466,#87467,#87468,#87469,
#87470,#87471,#87472,#87473,#87474,#87475,#87476,#87477,#87478,#87479,#87480,
#87481,#87482,#87483,#87484,#87485,#87486,#87487,#87488,#87489,#87490,#87491,
#87492,#87493,#87494,#87495,#87496,#87497,#87498,#87499,#87500,#87501,#87502,
#87503,#87504,#87505,#87506,#87507,#87508,#87509,#87510,#87511,#87512,#87513,
#87514,#87515,#87516,#87517,#87518,#87519,#87520,#87521,#87522,#87523,#87524,
#87525,#87526,#87527,#87528,#87529,#87530,#87531,#87532,#87533,#87534,#87535,
#87536,#87537,#87538,#87539,#87540,#87541,#87542,#87543,#87544,#87545,#87546,
#87547,#87548,#87549,#87550,#87551,#87552,#87553,#87554,#87555,#87556,#87557,
#87558,#87559,#87560,#87561,#87562,#87563,#87564,#87565,#87566,#87567,#87568,
#87569,#87570,#87571,#87572,#87573,#87574,#87575,#87576,#87577,#87578,#87579,
#87580,#87581,#87582,#87583,#87584,#87585,#87586,#87587,#87588,#87589,#87590,
#87591,#87592,#87593,#87594,#87595,#87596,#87597,#87598,#87599,#87600,#87601,
#87602,#87603,#87604,#87605,#87606,#87607,#87608,#87609,#87610,#87611,#87612,
#87613,#87614,#87615,#87616,#87617,#87618,#87619,#87620,#87621,#87622,#87623,
#87624,#87625,#87626,#87627,#87628,#87629,#87630,#87631,#87632,#87633,#87634,
#87635,#87636,#87637,#87638,#87639,#87640,#87641,#87642,#87643,#87644,#87645,
#87646,#87647,#87648,#87649,#87650,#87651,#87652,#87653,#87654,#87655,#87656,
#87657,#87658,#87659,#87660,#87661,#87662,#87663,#87664,#87665,#87666,#87667,
#87668,#87669,#87670,#87671,#87672,#87673,#87674,#87675,#87676,#87677,#87678,
#87679,#87680,#87681,#87682,#87683,#87684,#87685,#87686,#87687,#87688,#87689,
#87690,#87691,#87692,#87693,#87694,#87695,#87696,#87697,#87698,#87699,#87700,
#87701,#87702,#87703,#87704,#87705,#87706,#87707,#87708,#87709,#87710,#87711,
#87712,#87713,#87714,#87715,#87716,#87717,#87718,#87719,#87720,#87721,#87722,
#87723,#87724,#87725,#87726,#87727,#87728,#87729,#87730,#87731,#87732,#87733,
#87734,#87735,#87736,#87737,#87738,#87739,#87740,#87741,#87742,#87743,#87744,
#87745,#87746,#87747,#87748,#87749,#87750,#87751,#87752,#87753,#87754,#87755,
#87756,#87757,#87758,#87759,#87760,#87761,#87762,#87763,#87764,#87765,#87766,
#87767,#87768,#87769,#87770,#87771,#87772,#87773,#87774,#87775,#87776,#87777,
#87778,#87779,#87780,#87781,#87782,#87783,#87784,#87785,#87786,#87787,#87788,
#87789,#87790,#87791,#87792,#87793,#87794,#87795,#87796,#87797,#87798,#87799,
#87800,#87801,#87802,#87803,#87804,#87805,#87806,#87807,#87808,#87809,#87810,
#87811,#87812,#87813,#87814,#87815,#87816,#87817,#87818,#87819,#87820,#87821,
#87822,#87823,#87824,#87825,#87826,#87827,#87828,#87829,#87830,#87831,#87832,
#87833,#87834,#87835,#87836,#87837,#87838,#87839,#87840,#87841,#87842,#87843,
#87844,#87845,#87846,#87847,#87848,#87849,#87850,#87851,#87852,#87853,#87854,
#87855,#87856,#87857,#87858,#87859,#87860,#87861,#87862,#87863,#87864,#87865,
#87866,#87867,#87868,#87869,#87870,#87871,#87872,#87873,#87874,#87875,#87876,
#87877,#87878,#87879,#87880,#87881,#87882,#87883,#87884,#87885,#87886,#87887,
#87888,#87889,#87890,#87891,#87892,#87893,#87894,#87895,#87896,#87897,#87898,
#87899,#87900,#87901,#87902,#87903,#87904,#87905,#87906,#87907,#87908,#87909,
#87910,#87911,#87912,#87913,#87914,#87915,#87916,#87917,#87918,#87919,#87920,
#87921,#87922,#87923,#87924,#87925,#87926,#87927,#87928,#87929,#87930,#87931,
#87932,#87933,#87934,#87935,#87936,#87937,#87938,#87939,#87940,#87941,#87942,
#87943,#87944,#87945,#87946,#87947,#87948,#87949,#87950,#87951,#87952,#87953,
#87954,#87955,#87956,#87957,#87958,#87959,#87960,#87961,#87962,#87963,#87964,
#87965,#87966,#87967,#87968,#87969,#87970,#87971,#87972,#87973,#87974,#87975,
#87976,#87977,#87978,#87979,#87980,#87981,#87982,#87983,#87984,#87985,#87986,
#87987,#87988,#87989,#87990,#87991,#87992,#87993,#87994,#87995,#87996,#87997,
#87998,#87999,#88000,#88001,#88002,#88003,#88004,#88005,#88006,#88007,#88008,
#88009,#88010,#88011,#88012,#88013,#88014,#88015,#88016,#88017,#88018,#88019,
#88020,#88021,#88022,#88023,#88024,#88025,#88026,#88027,#88028,#88029,#88030,
#88031,#88032,#88033,#88034,#88035,#88036,#88037,#88038,#88039,#88040,#88041,
#88042,#88043,#88044,#88045,#88046,#88047,#88048,#88049,#88050,#88051,#88052,
#88053,#88054,#88055,#88056,#88057,#88058,#88059,#88060,#88061,#88062,#88063,
#88064,#88065,#88066,#88067,#88068,#88069,#88070,#88071,#88072,#88073,#88074,
#88075,#88076,#88077,#88078,#88079,#88080,#88081,#88082,#88083,#88084,#88085,
#88086,#88087,#88088,#88089,#88090,#88091,#88092,#88093,#88094,#88095,#88096,
#88097,#88098,#88099,#88100,#88101,#88102,#88103,#88104,#88105,#88106,#88107,
#88108,#88109,#88110,#88111,#88112,#88113,#88114,#88115,#88116,#88117,#88118,
#88119,#88120,#88121,#88122,#88123,#88124,#88125,#88126,#88127,#88128,#88129,
#88130,#88131,#88132,#88133,#88134,#88135,#88136,#88137,#88138,#88139,#88140,
#88141,#88142,#88143,#88144,#88145,#88146,#88147,#88148,#88149,#88150,#88151,
#88152,#88153,#88154,#88155,#88156,#88157,#88158,#88159,#88160,#88161,#88162,
#88163,#88164,#88165,#88166,#88167,#88168,#88169,#88170,#88171,#88172,#88173,
#88174,#88175,#88176,#88177,#88178,#88179,#88180,#88181,#88182,#88183,#88184,
#88185,#88186,#88187,#88188,#88189,#88190,#88191,#88192,#88193,#88194,#88195,
#88196,#88197,#88198,#88199,#88200,#88201,#88202,#88203,#88204,#88205,#88206,
#88207,#88208,#88209,#88210,#88211,#88212,#88213,#88214,#88215,#88216,#88217,
#88218,#88219,#88220,#88221,#88222,#88223,#88224,#88225,#88226,#88227,#88228,
#88229,#88230,#88231,#88232,#88233,#88234,#88235,#88236,#88237,#88238,#88239,
#88240,#88241,#88242,#88243,#88244,#88245,#88246,#88247,#88248,#88249,#88250,
#88251,#88252,#88253,#88254,#88255,#88256,#88257,#88258,#88259,#88260,#88261,
#88262,#88263,#88264,#88265,#88266,#88267,#88268,#88269,#88270,#88271,#88272,
#88273,#88274,#88275,#88276,#88277,#88278,#88279,#88280,#88281,#88282,#88283,
#88284,#88285,#88286,#88287,#88288,#88289,#88290,#88291,#88292,#88293,#88294,
#88295,#88296,#88297,#88298,#88299,#88300,#88301,#88302,#88303,#88304,#88305,
#88306,#88307,#88308,#88309,#88310,#88311,#88312,#88313,#88314,#88315,#88316,
#88317,#88318,#88319,#88320,#88321,#88322,#88323,#88324,#88325,#88326,#88327,
#88328,#88329,#88330,#88331,#88332,#88333,#88334,#88335,#88336,#88337,#88338,
#88339,#88340,#88341,#88342,#88343,#88344,#88345,#88346,#88347,#88348,#88349,
#88350,#88351,#88352,#88353,#88354,#88355,#88356,#88357,#88358,#88359,#88360,
#88361,#88362,#88363,#88364,#88365,#88366,#88367,#88368,#88369,#88370,#88371,
#88372,#88373,#88374,#88375,#88376,#88377,#88378,#88379,#88380,#88381,#88382,
#88383,#88384,#88385,#88386,#88387,#88388,#88389,#88390,#88391,#88392,#88393,
#88394,#88395,#88396,#88397,#88398,#88399,#88400,#88401,#88402,#88403,#88404,
#88405,#88406,#88407,#88408,#88409,#88410,#88411,#88412,#88413,#88414,#88415,
#88416,#88417,#88418,#88419,#88420,#88421,#88422,#88423,#88424,#88425,#88426,
#88427,#88428,#88429,#88430,#88431,#88432,#88433,#88434,#88435,#88436,#88437,
#88438,#88439,#88440,#88441,#88442,#88443,#88444,#88445,#88446,#88447,#88448,
#88449,#88450,#88451,#88452,#88453,#88454,#88455,#88456,#88457,#88458,#88459,
#88460,#88461,#88462,#88463,#88464,#88465,#88466,#88467,#88468,#88469,#88470,
#88471,#88472,#88473,#88474,#88475,#88476,#88477,#88478,#88479,#88480,#88481,
#88482,#88483,#88484,#88485,#88486,#88487,#88488,#88489,#88490,#88491,#88492,
#88493,#88494,#88495,#88496,#88497,#88498,#88499,#88500,#88501,#88502,#88503,
#88504,#88505,#88506,#88507,#88508,#88509,#88510,#88511,#88512,#88513,#88514,
#88515,#88516,#88517,#88518,#88519,#88520,#88521,#88522,#88523,#88524,#88525,
#88526,#88527,#88528,#88529,#88530,#88531,#88532,#88533,#88534,#88535,#88536,
#88537,#88538,#88539,#88540,#88541,#88542,#88543,#88544,#88545,#88546,#88547,
#88548,#88549,#88550,#88551,#88552,#88553,#88554,#88555,#88556,#88557,#88558,
#88559,#88560,#88561)),.UNSPECIFIED.,.F.,.F.,.F.,(2,2),(4,1,1,1,1,1,1,1,
1,1,1,1,1,1,1,1,1,1,1,1,1,1,1,1,1,1,1,1,1,1,1,1,1,1,1,1,1,1,1,1,1,1,1,1,
1,1,1,1,1,1,1,1,1,1,1,1,1,1,1,1,1,1,1,1,1,1,1,1,1,1,1,1,1,1,1,1,1,1,1,1,
1,1,1,1,1,1,1,1,1,1,1,1,1,1,1,1,1,1,1,1,1,1,1,1,1,1,1,1,1,1,1,1,1,1,1,1,
1,1,1,1,1,1,1,1,1,1,1,1,1,1,1,1,1,1,1,1,1,1,1,1,1,1,1,1,1,1,1,1,1,1,1,1,
1,1,1,1,1,1,1,1,1,1,1,1,1,1,1,1,1,1,1,1,1,1,1,1,1,1,1,1,1,1,1,1,1,1,1,1,
1,1,1,1,1,1,1,1,1,1,1,1,1,1,1,1,1,1,1,1,1,1,1,1,1,1,1,1,1,1,1,1,1,1,1,1,
1,1,1,1,1,1,1,1,1,1,1,1,1,1,1,1,1,1,1,1,1,1,1,1,1,1,1,1,1,1,1,1,1,1,1,1,
1,1,1,1,1,1,1,1,1,1,1,1,1,1,1,1,1,1,1,1,1,1,1,1,1,1,1,1,1,1,1,1,1,1,1,1,
1,1,1,1,1,1,1,1,1,1,1,1,1,1,1,1,1,1,1,1,1,1,1,1,1,1,1,1,1,1,1,1,1,1,1,1,
1,1,1,1,1,1,1,1,1,1,1,1,1,1,1,1,1,1,1,1,1,1,1,1,1,1,1,1,1,1,1,1,1,1,1,1,
1,1,1,1,1,1,1,1,1,1,1,1,1,1,1,1,1,1,1,1,1,1,1,1,1,1,1,1,1,1,1,1,1,1,1,1,
1,1,1,1,1,1,1,1,1,1,1,1,1,1,1,1,1,1,1,1,1,1,1,1,1,1,1,1,1,1,1,1,1,1,1,1,
1,1,1,1,1,1,1,1,1,1,1,1,1,1,1,1,1,1,1,1,1,1,1,1,1,1,1,1,1,1,1,1,1,1,1,1,
1,1,1,1,1,1,1,1,1,1,1,1,1,1,1,1,1,1,1,1,1,1,1,1,1,1,1,1,1,1,1,1,1,1,1,1,
1,1,1,1,1,1,1,1,1,1,1,1,1,1,1,1,1,1,1,1,1,1,1,1,1,1,1,1,1,1,1,1,1,1,1,1,
1,1,1,1,1,1,1,1,1,1,1,1,1,1,1,1,1,1,1,1,1,1,1,1,1,1,1,1,1,1,1,1,1,1,1,1,
1,1,1,1,1,1,1,1,1,1,1,1,1,1,1,1,1,1,1,1,1,1,1,1,1,1,1,1,1,1,1,1,1,1,1,1,
1,1,1,1,1,1,1,1,1,1,1,1,1,1,1,1,1,1,1,1,1,1,1,1,1,1,1,1,1,1,1,1,1,1,1,1,
1,1,1,1,1,1,1,1,1,1,1,1,1,1,1,1,1,1,1,1,1,1,1,1,1,1,1,1,1,1,1,1,1,1,1,1,
1,1,1,1,1,1,1,1,1,1,1,1,1,1,1,1,1,1,1,1,1,1,1,1,1,1,1,1,1,1,1,1,1,1,1,1,
1,1,1,1,1,1,1,1,1,1,1,1,1,1,1,1,1,1,1,1,1,1,1,1,1,1,1,1,1,1,1,1,1,1,1,1,
1,1,1,1,1,1,1,1,1,1,1,1,1,1,1,1,1,1,1,1,1,1,1,1,1,1,1,1,1,1,1,1,1,1,1,1,
1,1,1,1,1,1,1,1,1,1,1,1,1,1,1,1,1,1,1,1,1,1,1,1,1,1,1,1,1,1,1,1,1,1,1,1,
1,1,1,1,1,1,1,1,1,1,1,1,1,1,1,1,1,1,1,1,1,1,1,1,1,1,1,1,1,1,1,1,1,1,1,1,
1,1,1,1,1,1,1,1,1,1,1,1,1,1,1,1,1,1,1,1,1,1,1,1,1,1,1,1,1,1,1,1,1,1,1,1,
1,1,1,1,1,1,1,1,1,1,1,1,1,1,1,1,1,1,1,1,1,1,1,1,1,1,1,1,1,1,1,1,1,1,1,1,
1,1,1,1,1,1,1,1,1,1,1,1,1,1,1,1,1,1,1,1,1,1,1,1,1,1,1,1,1,1,1,1,1,1,1,1,
1,1,1,1,1,1,1,1,1,1,1,1,1,1,1,1,1,1,1,1,1,1,1,1,1,1,1,1,1,1,1,1,1,1,1,1,
1,1,1,1,1,1,1,1,1,1,1,1,1,1,1,1,1,1,1,1,1,1,1,1,1,1,1,1,1,1,1,1,1,1,1,1,
1,1,1,1,1,1,1,1,1,1,1,1,1,1,1,1,1,1,1,1,1,1,1,1,1,1,1,1,1,1,1,1,1,1,1,1,
1,1,1,1,1,1,1,1,1,1,1,1,1,1,1,1,1,1,1,1,1,1,1,1,1,1,1,1,1,1,1,1,1,1,1,1,
1,1,1,1,1,1,1,1,1,1,1,1,1,1,1,1,1,1,1,1,1,1,1,1,1,1,1,1,1,1,1,1,1,1,1,1,
1,1,1,1,1,1,1,1,1,1,1,1,1,1,1,1,1,1,1,1,1,1,1,1,1,1,1,1,1,1,1,1,1,1,1,1,
1,1,1,1,1,1,1,1,1,1,1,1,1,1,1,1,1,1,1,1,1,1,1,1,1,1,1,1,1,1,1,1,1,1,1,1,
1,1,1,1,1,1,1,1,1,1,1,1,1,1,1,1,1,1,1,1,1,1,1,1,1,1,1,1,1,1,1,1,1,1,1,1,
1,1,1,1,1,1,1,1,1,1,1,1,1,1,1,1,1,1,1,1,1,1,1,1,1,1,1,1,1,1,1,1,1,1,1,1,
1,1,1,1,1,1,1,1,1,1,1,1,1,1,1,1,1,1,1,1,1,1,1,1,1,1,1,1,1,1,1,1,1,1,1,1,
1,1,1,1,1,1,1,1,1,1,1,1,1,1,1,1,1,1,1,1,1,1,1,1,1,1,1,1,1,1,1,1,1,1,1,1,
1,1,1,1,1,1,1,1,1,1,1,1,1,1,1,1,1,1,1,1,1,1,1,1,1,1,1,1,1,1,1,1,1,1,1,1,
1,1,1,1,1,1,1,1,1,1,1,1,1,1,1,1,1,1,1,1,1,1,1,1,1,1,1,1,1,1,1,1,1,1,1,1,
1,1,1,1,1,1,1,1,1,1,1,1,1,1,1,1,1,1,1,1,1,1,1,1,1,1,1,1,1,1,1,1,1,1,1,1,
1,1,1,1,1,1,1,1,1,1,1,1,1,1,1,1,1,1,1,1,1,1,1,1,1,1,1,1,1,1,1,1,1,1,1,1,
1,1,1,1,1,1,1,1,1,1,1,1,1,1,1,1,1,1,1,1,1,1,1,1,1,1,1,1,1,1,1,1,1,1,1,1,
1,1,1,1,1,1,1,1,1,1,1,1,1,1,1,1,1,1,1,1,1,1,1,1,1,1,1,1,1,1,1,1,1,1,1,1,
1,1,1,1,1,1,1,1,1,1,1,1,1,1,1,1,1,1,1,1,1,1,1,1,1,1,1,1,1,1,1,1,1,1,1,1,
1,1,1,1,1,1,1,1,1,1,1,1,1,1,1,1,1,1,1,1,1,1,1,1,1,1,1,1,1,1,1,1,1,1,1,1,
1,1,1,1,1,1,1,1,1,1,1,1,1,1,1,1,1,1,1,1,1,1,1,1,1,1,1,1,1,1,1,1,1,1,1,1,
1,1,1,1,1,1,1,1,1,1,1,1,1,1,1,1,1,1,1,1,1,1,1,1,1,1,1,1,1,1,1,1,1,1,1,1,
1,1,1,1,1,1,1,1,1,1,1,1,1,1,1,1,1,1,1,1,1,1,1,1,1,1,1,1,1,1,1,1,1,1,1,1,
1,1,1,1,1,1,1,1,1,1,1,1,1,1,1,1,1,1,1,1,1,1,1,1,1,1,1,1,1,1,1,1,1,1,1,1,
1,1,1,1,1,1,1,1,1,1,1,1,1,1,1,1,1,1,1,1,1,1,1,1,1,1,1,1,1,1,1,1,1,1,1,1,
1,1,1,1,1,1,1,1,1,1,1,1,1,1,1,1,1,1,1,1,1,1,1,1,1,1,1,1,1,1,1,1,1,1,1,1,
1,1,1,1,1,1,1,1,1,1,1,1,1,1,1,1,1,1,1,1,1,1,1,1,1,1,1,1,1,1,1,1,1,1,1,1,
1,1,1,1,1,1,1,1,1,1,1,1,1,1,1,1,1,1,1,1,1,1,1,1,1,1,1,1,1,1,1,1,1,1,1,1,
1,1,1,1,1,1,1,1,1,1,1,1,1,1,1,1,1,1,1,1,1,1,1,1,1,1,1,1,1,1,1,1,1,1,1,1,
1,1,1,1,1,1,1,1,1,1,1,1,1,1,1,1,1,1,1,1,1,1,1,1,1,1,1,1,1,1,1,1,1,1,1,1,
1,1,1,1,1,1,1,1,1,1,1,1,1,1,1,1,1,1,1,1,1,1,1,1,1,1,1,1,1,1,1,1,1,1,1,1,
1,1,1,1,1,1,1,1,1,1,1,1,1,1,1,1,1,1,1,1,1,1,1,1,1,1,1,1,1,1,1,1,1,1,1,1,
1,1,1,1,1,1,1,1,1,1,1,1,1,1,1,1,1,1,1,1,1,1,1,1,1,1,1,1,1,1,1,1,1,1,1,1,
1,1,1,1,1,1,1,1,1,1,1,1,1,1,1,1,1,1,1,1,1,1,1,1,1,1,1,1,1,1,1,1,1,1,1,1,
1,1,1,1,1,1,1,1,1,1,1,1,1,1,1,1,1,1,1,1,1,1,1,1,1,1,1,1,1,1,1,1,1,1,1,1,
1,1,1,1,1,1,1,1,1,1,1,1,1,1,1,1,1,1,1,1,1,1,1,1,1,1,1,1,1,1,1,1,1,1,1,1,
1,1,1,1,1,1,1,1,1,1,1,1,1,1,1,1,1,1,1,1,1,1,1,1,1,1,1,1,1,1,1,1,1,1,1,1,
1,1,1,1,1,1,1,1,1,1,1,1,1,1,1,1,1,1,1,1,1,1,1,1,1,1,1,1,1,1,1,1,1,1,1,1,
1,1,1,1,1,1,1,1,1,1,1,1,1,1,1,1,1,1,1,1,1,1,1,1,1,1,1,1,1,1,1,1,1,1,1,1,
1,1,1,1,1,1,1,1,1,1,1,1,1,1,1,1,1,1,1,1,1,1,1,1,1,1,1,1,1,1,1,1,1,1,1,1,
1,1,1,1,1,1,1,1,1,1,1,1,1,1,1,1,1,1,1,1,1,1,1,1,1,1,1,1,1,1,1,1,1,1,1,1,
1,1,1,1,1,1,1,1,1,1,1,1,1,1,1,1,1,1,1,1,1,1,1,1,1,1,1,1,1,1,1,1,1,1,1,1,
1,1,1,1,1,1,1,1,1,1,1,1,1,1,1,1,1,1,1,1,1,1,1,1,1,1,1,1,1,1,1,1,1,1,1,1,
1,1,1,1,1,1,1,1,1,1,1,1,1,1,1,1,1,1,1,1,1,1,1,1,1,1,1,1,1,1,1,1,1,1,1,1,
1,1,1,1,1,1,1,1,1,1,1,1,1,1,1,1,1,1,1,1,1,1,1,1,1,1,1,1,1,1,1,1,1,1,1,1,
1,1,1,1,1,1,1,1,1,1,1,1,1,1,1,1,1,1,1,1,1,1,1,1,1,1,1,1,1,1,1,1,1,1,1,1,
1,1,1,1,1,1,1,1,1,1,1,1,1,1,1,1,1,1,1,1,1,1,1,1,1,1,1,1,1,1,1,1,1,1,1,1,
1,1,1,1,1,1,1,1,1,1,1,1,1,1,1,1,1,1,1,1,1,1,1,1,1,1,1,1,1,1,1,1,1,1,1,1,
1,1,1,1,1,1,1,1,1,1,1,1,1,1,1,1,1,1,1,1,1,1,1,1,1,1,1,1,1,1,1,1,1,1,1,1,
1,1,1,1,1,1,1,1,1,1,1,1,1,1,1,1,1,1,1,1,1,1,1,1,1,1,1,1,1,1,1,1,1,1,1,1,
1,1,1,1,1,1,1,1,1,1,1,1,1,1,1,1,1,1,1,1,1,1,1,1,1,1,1,1,1,1,1,1,1,1,1,1,
1,1,1,1,1,1,1,1,1,1,1,1,1,1,1,1,1,1,1,1,1,1,1,1,1,1,1,1,1,1,1,1,1,1,1,1,
1,1,1,1,1,1,1,1,1,1,1,1,1,1,1,1,1,1,1,1,1,1,1,1,1,1,1,1,1,1,1,1,1,1,1,1,
1,1,1,1,1,1,1,1,1,1,1,1,1,1,1,1,1,1,1,1,1,1,1,1,1,1,1,1,1,1,1,1,1,1,1,1,
1,1,1,1,1,1,1,1,1,1,1,1,1,1,1,1,1,1,1,1,1,1,1,1,1,1,1,1,1,1,1,1,1,1,1,1,
1,1,1,1,1,1,1,1,1,1,1,1,1,1,1,1,1,1,1,1,1,1,1,1,1,1,1,1,1,1,1,1,1,1,1,1,
1,1,1,1,1,1,1,1,1,1,1,1,1,1,1,1,1,1,1,1,1,1,1,1,1,1,1,1,1,1,1,1,1,1,1,1,
1,1,1,1,1,1,1,1,1,1,1,1,1,1,1,1,1,1,1,1,1,1,1,1,1,1,1,1,1,1,1,1,1,1,1,1,
1,1,1,1,1,1,1,1,1,1,1,1,1,1,1,1,1,1,1,1,1,1,1,1,1,1,1,1,1,1,1,1,1,1,1,1,
1,1,1,1,1,1,1,1,1,1,1,1,1,1,1,1,1,1,1,1,1,1,1,1,1,1,1,1,1,1,1,1,1,1,1,1,
1,1,1,1,1,1,1,1,1,1,1,1,1,1,1,1,1,1,1,1,1,1,1,1,1,1,1,1,1,1,1,1,1,1,1,1,
1,1,1,1,1,1,1,1,1,1,1,1,1,1,1,1,1,1,1,1,1,1,1,1,1,1,1,1,1,1,1,1,1,1,1,1,
1,1,1,1,1,1,1,1,1,1,1,1,1,1,1,1,1,1,1,1,1,1,1,1,1,1,1,1,1,1,1,1,1,1,1,1,
1,1,1,1,1,1,1,1,1,1,1,1,1,1,1,1,1,1,1,1,1,1,1,1,1,1,1,1,1,1,1,1,1,1,1,1,
1,1,1,1,1,1,1,1,1,1,1,1,1,1,1,1,1,1,1,1,1,1,1,1,1,1,1,1,1,1,1,1,1,1,1,1,
1,1,1,1,1,1,1,1,1,1,1,1,1,1,1,1,1,1,1,1,1,1,1,1,1,1,1,1,1,1,1,1,1,1,1,1,
1,1,1,1,1,1,1,1,1,1,1,1,1,1,1,1,1,1,1,1,1,1,1,1,1,1,1,1,1,1,1,1,1,1,1,1,
1,1,1,1,1,1,1,1,1,1,1,1,1,1,1,1,1,1,1,1,1,1,1,1,1,1,1,1,1,1,1,1,1,1,1,1,
1,1,1,1,1,1,1,1,1,1,1,1,1,1,1,1,1,1,1,1,1,1,1,1,1,1,1,1,1,1,1,1,1,1,1,1,
1,1,1,1,1,1,1,1,1,1,1,1,1,1,1,1,1,1,1,1,1,1,1,1,1,1,1,1,1,1,1,1,1,1,1,1,
1,1,1,1,1,1,1,1,1,1,1,1,1,1,1,1,1,1,4),(-0.58309518948453,0.),(0.,0.869746702321014,
1.7394931589914,2.60923976624962,3.47983908319159,4.35043840179749,5.22018503077054,
6.08993165951504,6.95967828799171,7.82942491616733,8.69917154401062,9.56891817149224,
10.4395174886835,11.3101168056706,12.179863432132,13.049610058144,13.9193566836854,
14.7891033087372,15.6588499332817,16.5285965573034,17.3991958717975,18.2697951860185,
18.7046684974166,19.1395418086746,19.5744151197912,20.0092884307654,20.4441617415962,
20.8790350522825,21.7487816732187,22.1836549834672,22.6185282935685,23.0534016035221,
23.4882749133276,23.9231482229848,24.3588742245859,24.794600226187,25.2294735355468,
26.0992201538203,26.5340934627341,26.9689667714994,27.4038400801166,27.838713388586,
28.2735866969081,28.7084600050832,29.143333313112,29.5782066209952,30.0130799287334,
30.4479532363275,30.8828265437783,31.3185525442794,31.7542785447804,32.1891518519474,
32.6240251589741,33.0588984658616,33.4937717726112,33.928645079224,34.3635183857014,
34.7983916920448,35.2332649982556,35.6681383043353,36.1030116102854,36.5378849161076,
36.9727582218035,37.4076315273749,37.8425048328235,38.2782308323341,38.7139568318446,
39.1488301370532,39.5837034421446,40.0185767471208,40.4534500519838,40.8883233567357,
41.3231966613787,41.7580699659148,42.1929432703463,42.6278165746754,43.0626898789044,
43.4975631830356,43.9324364870714,44.3673097910142,44.8021830948664,45.2379090935952,
45.673635092324,46.1085083960024,46.5433816995978,46.9782550031127,47.4131283065497,
47.8480016099115,48.2828749132006,48.7177482164198,49.1526215195718,49.5874948226593,
50.0223681256851,50.457241428652,50.8921147315628,51.3269880344203,51.7618613372274,
52.197587335454,52.6333133336805,53.0681866363954,53.5030599390685,53.9379332417027,
54.3728065443011,54.8076798468664,55.2425531494018,55.6774264519101,56.1122997543943,
56.5471730568575,56.9820463593026,57.4169196617326,57.8517929641506,58.2866662665595,
58.7215395689624,59.157265567009,59.5929915650557,60.0278648674556,60.4627381698584,
60.8976114722673,61.3324847746853,61.7673580771153,62.2022313795604,62.6371046820236,
63.0719779845079,63.5068512870162,63.9417245895516,64.376597892117,64.8114711947155,
65.2463444973499,65.6812178000231,66.1169437982275,66.5526697964318,66.9875430991915,
67.4224164019987,67.8572897048563,68.2921630077673,68.7270363107343,69.1619096137603,
69.5967829168479,70.0316562200001,70.4665295232194,70.9014028265087,71.3362761298705,
71.7711494333077,72.2060227368227,72.6408960404182,73.0766220391044,73.5123480377905,
73.9472213415547,74.382094645407,74.8169679493499,75.2518412533859,75.6867145575172,
76.1215878617464,76.5564611660756,76.9913344705072,77.4262077750435,77.8610810796866,
78.2959543844386,78.7308276893018,79.1657009942781,79.6005742993696,80.0363002988208,
80.4720262982719,80.9068996035997,81.3417729090484,81.7766462146199,82.211519520316,
82.6463928261383,83.0812661320886,83.5161394381684,83.9510127443794,84.3858860507229,
84.8207593572004,85.2556326638134,85.6905059705631,86.1253792774507,86.5602525844776,
86.995978584908,87.4317045853384,87.8665778926469,88.3014512000977,88.7363245076919,
89.1711978154302,89.6060711233134,90.0409444313423,90.4758177395175,90.9106910478396,
91.345564356309,91.7804376649263,92.2153109736917,92.6501842826055,93.085057591668,
93.5199309008791,93.9556569024059,94.3913829039327,94.8262562134414,95.2611295230986,
95.6960028329042,96.1308761428578,96.5657494529591,97.0006227632077,97.4354960736028,
97.870369384144,98.3052426948304,98.7401160056612,99.1749893166354,99.6098626277522,
100.04473593901,100.915335253024,101.351061255639,101.785934567313,102.220807879124,
102.655681191068,103.090554503145,103.525427815353,104.395174440154,105.264921065453,
105.699794378283,106.134667691232,106.569541004295,107.004414317471,107.8750136343,
108.745612951339,109.615359578629,110.485106206296,111.354852834309,112.224599462639,
113.094346091254,113.964092720119,114.834692038763,115.705291357499,116.575037986826,
117.444784616267,118.314531245777,119.184277875311,120.054024504821,120.923771134261,
121.794370453112,122.66496977189,123.534716400968,124.404463029834,125.274209658448,
126.143956286779,127.013702914792,127.883449542458,128.754048859798,129.624648176939,
130.494394803617,131.364141429857,132.233888055637,133.103634680937,133.973381305737,
134.843127930023,135.71372724472,136.584326559147,137.019199870684,137.454073182083,
137.888946493341,138.323819804458,139.193566426263,140.063313047491,140.498186357887,
140.933059668136,141.367932978237,141.802806288191,142.237679597997,142.673405599673,
143.109131601348,143.544004910857,143.978878220217,144.413751529429,144.848624838491,
145.283498147405,145.718371456171,146.153244764789,146.588118073258,147.022991381581,
147.457864689756,147.892737997785,148.327611305669,148.762484613407,149.197357921002,
149.633083921574,150.068809922147,150.503683229455,150.938556536623,151.37342984365,
151.808303150538,152.243176457288,152.678049763901,153.112923070379,153.547796376722,
153.982669682934,154.417542989014,154.852416294964,155.287289600787,155.722162906483,
156.157036212055,156.592762211626,157.028488211198,157.463361516526,157.898234821735,
158.333108126826,158.767981431803,159.202854736666,159.637728041419,160.072601346062,
160.507474650599,160.94234795503,161.37722125936,161.812094563589,162.246967867721,
162.681841171757,163.1167144757,163.552440474473,163.988166473247,164.423039777011,
164.85791308069,165.292786384286,165.727659687801,166.162532991238,166.597406294601,
167.03227959789,167.46715290111,167.902026204262,168.33689950735,168.771772810376,
169.206646113343,169.641519416254,170.076392719112,170.512118717363,170.947844715614,
171.382718018374,171.817591321089,172.252464623762,172.687337926397,173.122211228996,
173.557084531561,173.991957834097,174.426831136606,174.86170443909,175.296577741554,
175.731451044,176.16632434643,176.601197648848,177.036070951258,177.471796949306,
177.907522947355,178.342396249755,178.777269552155,179.212142854558,179.647016156968,
180.081889459386,180.516762761816,180.951636064262,181.386509366726,181.82138266921,
182.256255971719,182.691129274255,183.12600257682,183.560875879419,183.995749182054,
184.431475180237,184.867201178421,185.302074481136,185.736947783896,186.171821086704,
186.606694389561,187.041567692473,187.47644099544,187.911314298466,188.346187601554,
188.781060904706,189.215934207926,189.650807511215,190.085680814577,190.520554118015,
190.95542742153,191.391153420175,191.82687941882,192.261752722499,192.696626026263,
193.131499330116,193.566372634059,194.001245938095,194.436119242227,194.870992546456,
195.305865850785,195.740739155217,196.175612459754,196.610485764397,197.045359069149,
197.480232374013,197.915105678989,198.350831678382,198.786557677775,199.221430982984,
199.656304288312,200.091177593761,200.526050899333,200.960924205029,201.395797510852,
201.830670816802,202.265544122882,202.700417429093,203.135290735437,203.570164041915,
204.005037348528,204.439910655278,204.874783962166,205.310509962526,205.746235962887,
206.181109270054,206.615982577363,207.050855884814,207.485729192409,207.920602500147,
208.355475808031,208.79034911606,209.225222424235,209.660095732558,210.094969041027,
210.529842349645,210.96471565841,211.399588967324,211.834462276387,212.27018827784,
212.705914279292,213.140787588653,213.575660898161,214.010534207819,214.880280827579,
215.31515413768,215.750027447929,216.184900758324,216.619774068866,217.054647379553,
217.489520690384,218.359267312475,219.22986662628,219.665592628826,220.100465940363,
220.535339252038,220.970212563848,221.83995918787,222.709705812416,223.579452437468,
224.014325750179,224.44919906301,225.318945689022,226.189545005688,227.060144322571,
227.929890949664,228.799637577146,229.66938420499,230.539130833166,231.408877461643,
232.278624090388,233.149223408954,234.019822727623,234.889569356878,235.759315986267,
236.629062615749,237.498809245277,238.368555874806,239.238302504287,240.108901823183,
240.979501142017,241.849247771189,242.718994400167,243.588741028911,244.458487657389,
245.328234285565,246.197980913409,247.068580230891,247.939179548182,248.80892617507,
249.678672801532,250.548419427545,251.418166053087,252.287912678139,253.157659302684,
254.028258617581,254.898857932211,255.333731243885,255.768604555423,256.203477866821,
256.63835117808,257.508097800171,258.377844421689,258.812717732231,259.247591042627,
259.682464352876,260.117337662977,260.552210972931,260.987936974682,261.858536286089,
262.293409595598,262.728282904958,263.16315621417,263.598029523233,264.032902832147,
264.467776140913,264.902649449531,265.337522758001,265.772396066323,266.207269374499,
266.642142682528,267.077015990412,267.511889298151,267.947615298795,268.383341299439,
268.81821460689,269.2530879142,269.687961221367,270.122834528394,270.557707835282,
270.992581142032,271.427454448646,271.862327755124,272.297201061468,272.732074367679,
273.166947673759,273.60182097971,274.036694285533,274.471567591229,274.907293590862,
275.343019590495,275.777892895944,276.212766201272,276.647639506481,277.082512811573,
277.51738611655,277.952259421414,278.387132726166,278.82200603081,279.256879335346,
279.691752639779,280.126625944108,280.561499248338,280.996372552469,281.431245856506,
281.866971855324,282.302697854143,282.737571157996,283.172444461761,283.60731776544,
284.042191069036,284.477064372551,284.911937675989,285.346810979351,285.781684282641,
286.216557585861,286.651430889013,287.086304192101,287.521177495128,287.956050798095,
288.390924101007,288.826650099283,289.262376097559,289.697249400366,290.132122703127,
290.566996005842,291.001869308516,291.43674261115,291.871615913749,292.306489216315,
292.741362518851,293.17623582136,293.611109123845,294.045982426308,294.480855728754,
294.915729031185,295.350602333603,295.786328331655,296.222054329707,296.65692763211,
297.091800934511,297.526674236911,297.961547539314,298.396420841724,298.831294144142,
299.266167446573,299.701040749018,300.135914051482,300.570787353967,301.005660656476,
301.440533959012,301.875407261578,302.310280564177,302.746006562341,303.181732560506,
303.616605863179,304.051479165895,304.486352468655,304.921225771462,305.35609907432,
305.790972377232,306.225845680199,306.660718983226,307.095592286314,307.530465589466,
307.965338892686,308.400212195976,308.835085499338,309.269958802776,309.705684801381,
310.141410799985,310.576284103581,311.01115740726,311.446030711025,311.880904014878,
312.315777318821,312.750650622858,313.185523926989,313.620397231219,314.055270535549,
314.490143839981,314.925017144517,315.359890449161,315.794763753913,316.229637058777,
316.665363058112,317.101089057448,317.53596236254,317.970835667749,318.405708973077,
318.840582278526,319.275455584098,319.710328889795,320.145202195618,320.580075501568,
321.014948807648,321.44982211386,321.884695420204,322.319568726682,322.754442033295,
323.189315340045,323.625041340336,324.060767340628,324.495640647655,324.930513954822,
325.365387262131,325.800260569583,326.235133877177,326.670007184916,327.1048804928,
327.539753800829,327.974627109005,328.409500417327,328.844373725797,329.279247034415,
329.714120343181,330.148993652095,330.584719653474,331.020445654852,331.455318964064,
331.890192273424,332.325065582933,332.759938892591,333.194812202397,333.629685512351,
334.064558822453,334.499432132702,334.934305443098,335.369178753639,335.804052064326,
336.673798686132,337.108671997249,337.544397999725,337.980124002201,338.4149973136,
338.849870625137,339.284743936812,340.154490560568,341.024237184854,341.459110497191,
341.893983809655,342.328857122244,342.763730434955,343.633477060735,344.504076377234,
345.374675693955,346.244422320844,347.114168948136,347.983915575803,348.853662203817,
349.723408832148,350.593155460764,351.463754779246,352.334354097839,353.204100727012,
354.07384735634,354.943593985781,355.813340615292,356.683087244827,357.552833874338,
358.423433193272,359.294032512154,360.163779141409,361.033525770489,361.903272399355,
362.77301902797,363.642765656301,364.512512284316,365.383111601936,366.253710919371,
367.123457546465,367.993204173143,368.862950799383,369.732697425164,370.602444050463,
371.472190675265,372.342789990359,373.21338930519,373.648262617,374.083135928675,
374.952882551611,375.822629173987,376.257502484962,376.692375795793,377.12724910648,
377.562122417021,377.996995727417,378.431869037666,378.866742347767,379.302468349591,
379.738194351416,380.173067661222,380.607940970879,381.042814280388,381.477687589749,
381.91256089896,382.347434208023,382.782307516937,383.217180825703,383.652054134321,
384.086927442791,384.521800751113,384.956674059289,385.391547367318,385.826420675202,
386.262146675918,386.697872676635,387.13274598423,387.567619291681,388.00249259899,
388.437365906157,388.872239213185,389.307112520073,389.741985826823,390.176859133436,
390.611732439914,391.046605746258,391.48147905247,391.91635235855,392.351225664501,
392.786098970323,393.221824970019,393.657550969714,394.092424275286,394.527297580735,
394.962170886063,395.397044191272,395.831917496364,396.266790801341,396.701664106204,
397.136537410957,397.5714107156,398.006284020137,398.441157324569,398.876030628899,
399.310903933128,399.74577723726,400.181503236126,400.617229234991,401.052102538934,
401.486975842787,401.921849146551,402.356722450231,402.791595753827,403.226469057342,
403.66134236078,404.096215664142,404.531088967432,404.965962270651,405.400835573804,
405.835708876892,406.270582179918,406.705455482886,407.141181481189,407.576907479491,
408.01178078235,408.446654085157,408.881527387917,409.316400690633,409.751273993306,
410.186147295941,410.62102059854,411.055893901106,411.490767203642,411.925640506151,
412.360513808636,412.795387111099,413.230260413545,413.665133715976,414.100859714032,
414.536585712088,414.971459014498,415.406332316901,415.841205619301,416.276078921702,
416.710952224105,417.145825526515,417.580698828933,418.015572131364,418.45044543381,
418.885318736273,419.320192038758,419.755065341267,420.189938643803,420.624811946369,
421.060537944515,421.496263942662,421.931137245297,422.36601054797,422.800883850686,
423.235757153446,423.670630456253,424.105503759112,424.540377062023,424.975250364991,
425.410123668017,425.844996971105,426.279870274258,426.714743577477,427.149616880767,
427.584490184129,428.020216182695,428.455942181261,428.890815484776,429.325688788373,
429.760562092052,430.195435395816,430.630308699669,431.065182003612,431.500055307649,
431.93492861178,432.36980191601,432.80467522034,433.239548524772,433.674421829309,
434.109295133952,434.544168438705,434.979894437984,435.415620437262,435.850493742239,
436.285367047331,436.72024035254,437.155113657869,437.589986963318,438.024860268889,
438.459733574586,438.894606880409,439.32948018636,439.76435349244,440.199226798651,
440.634100104995,441.068973411473,441.503846718087,441.939572718309,442.375298718531,
442.810172025419,443.245045332447,443.679918639614,444.114791946923,444.549665254374,
444.984538561969,445.419411869708,445.854285177591,446.289158485621,446.724031793796,
447.158905102119,447.593778410589,448.028651719207,448.463525027973,448.899251029277,
449.334977030581,449.769850339644,450.639596958216,451.074470267725,451.509343577383,
451.944216887189,452.379090197143,452.813963507244,453.248836817493,453.683710127889,
454.118583438431,454.553456749117,454.988330059949,455.423203370923,455.858929373329,
456.294655375734,456.729528686993,457.164401998391,457.599275309929,458.469021933414,
458.90389524536,459.338768557437,459.773641869646,460.208515181983,460.643388494447,
461.078261807036,461.948008432578,462.818607748906,463.689207065461,464.55895369214,
465.428700319234,466.298446946716,467.16819357456,468.037940202737,468.907686831215,
469.778286149605,470.648885468116,471.518632097196,472.388378726451,473.258125355841,
474.127871985322,474.997618614851,475.86736524438,476.737964563343,477.608563882265,
478.478310511593,479.348057140765,480.217803769743,481.087550398488,481.957297026966,
482.827043655142,483.697642972895,484.568242290469,485.43798891776,486.307735544649,
487.177482171112,488.047228797125,488.916975422667,489.78672204772,490.657321363009,
491.09304736596,491.527920678038,492.397667301793,493.267413925005,494.137160547663,
494.57203385878,495.006907169755,495.441780480586,495.876653791273,496.311527101814,
496.74640041221,497.616999724357,498.052725726255,498.487599036209,498.922472346015,
499.357345655673,499.792218965182,500.227092274542,500.661965583754,501.096838892816,
501.531712201731,501.966585510497,502.401458819114,502.836332127584,503.271205435907,
503.706078744082,504.140952052112,504.576678052901,505.01240405369,505.447277361429,
505.882150669023,506.317023976474,506.751897283783,507.186770590951,507.621643897978,
508.056517204866,508.491390511616,508.92626381823,509.361137124708,509.796010431052,
510.230883737263,510.665757043344,511.100630349294,511.536356349053,511.972082348811,
512.406955654506,512.841828960076,513.276702265523,513.711575570849,514.146448876056,
514.581322181146,515.016195486121,515.451068790983,515.885942095733,516.320815400375,
516.75568870491,517.19056200934,517.625435313668,518.060308617896,518.496034616807,
518.931760615718,519.366633919752,519.801507223694,520.236380527545,520.671253831307,
521.106127134985,521.541000438579,521.975873742092,522.410747045528,522.845620348888,
523.280493652176,523.715366955394,524.150240258545,524.585113561631,525.019986864656,
525.455712862985,525.891438861313,526.326312164223,526.761185467079,527.196058769885,
527.630932072643,528.065805375356,528.500678678029,528.935551980661,529.370425283258,
529.805298585822,530.240171888356,530.675045190863,531.109918493346,531.544791795808,
531.979665098252,532.415391096312,532.851117094373,533.285990396789,533.720863699197,
534.155737001598,534.590610303997,535.025483606395,535.460356908796,535.895230211204,
536.330103513621,536.764976816049,537.199850118493,537.634723420955,538.069596723438,
538.504470025945,538.93934332848,539.375069326608,539.810795324736,540.245668627333,
540.680541929966,541.115415232637,541.550288535351,541.985161838109,542.420035140915,
542.854908443771,543.28978174668,543.724655049646,544.15952835267,544.594401655757,
545.029274958907,545.464148262125,545.899021565413,546.334747563939,546.770473562465,
547.205346865901,547.640220169415,548.075093473009,548.509966776686,548.944840080449,
549.3797133843,549.814586688241,550.249459992276,550.684333296405,551.119206600633,
551.554079904961,551.988953209391,552.423826513926,552.858699818567,553.294425817789,
553.73015181701,554.165025121872,554.599898426846,555.034771731937,555.469645037144,
555.90451834247,556.339391647917,556.774264953487,557.209138259182,557.644011565003,
558.078884870951,558.51375817703,558.948631483239,559.383504789581,559.818378096058,
560.254104096209,560.689830096361,561.12470340311,561.559576709996,561.994450017021,
562.429323324187,562.864196631494,563.299069938943,563.733943246536,564.168816554273,
564.603689862154,565.038563170182,565.473436478355,565.908309786676,566.343183095144,
566.77805640376,567.213782404988,567.649508406216,568.084381715128,568.519255024189,
568.954128333399,569.389001642757,569.823874952264,570.258748261921,570.693621571725,
571.128494881677,571.563368191777,572.433114812417,572.867988122957,573.302861433642,
573.737734744471,574.173460746804,574.609186749136,575.044060060251,575.913806682904,
576.783553306113,577.218426617922,577.653299929865,578.08817324194,578.523046554147,
579.392793178944,580.26253980424,581.13313912039,581.568865123709,582.003738436771,
582.87348506323,583.743231690115,584.612978317402,585.482724945065,586.352471573076,
587.222218201403,588.092817519691,588.963416838109,589.833163467083,590.702910096251,
591.572656725575,592.442403355013,593.31214998452,594.181896614051,595.05249593303,
595.92309525198,596.792841881366,597.662588510618,598.532335139693,599.402081768556,
600.271828397167,601.141575025495,602.012174343369,602.882773661074,603.752520288553,
604.622266915642,605.492013542317,606.361760168553,607.23150679433,608.101253419626,
608.971852735101,609.842452050322,610.71219867434,611.581945297822,612.451691920754,
612.886565232011,613.321438543126,613.756311854099,614.191185164928,615.060931786153,
615.931531098516,616.367257100486,616.802130410586,617.237003720538,617.671877030342,
618.106750339998,618.541623649505,618.976496958863,619.411370268073,619.846243577134,
620.281116886046,620.71599019481,621.150863503426,621.585736811894,622.020610120214,
622.455483428388,622.891209429248,623.326935430108,623.761808737989,624.196682045726,
624.631555353319,625.066428660769,625.501301968075,625.936175275241,626.371048582266,
626.805921889153,627.240795195901,627.675668502512,628.110541808988,628.54541511533,
628.98028842154,629.415161727618,629.850887727438,630.286613727259,630.72148703308,
631.156360338774,631.591233644344,632.026106949791,632.460980255118,632.895853560325,
633.330726865415,633.76560017039,634.200473475251,634.635346780002,635.070220084644,
635.505093389179,635.939966693609,636.374839997937,636.810565996897,637.246291995857,
637.681165299986,638.116038604021,638.550911907962,638.985785211813,639.420658515576,
639.855531819253,640.290405122847,640.725278426361,641.160151729796,641.595025033157,
642.029898336444,642.464771639662,642.899644942813,643.334518245899,643.770244244257,
644.205970242616,644.640843545581,645.075716848491,645.510590151347,645.945463454153,
646.380336756911,646.815210059625,647.250083362296,647.684956664929,648.119829967526,
648.55470327009,648.989576572624,649.424449875131,649.859323177614,650.294196480076,
650.729922478144,651.165648476212,651.600521778641,652.035395081057,652.470268383465,
652.905141685866,653.340014988265,653.774888290663,654.209761593065,654.644634895472,
655.079508197889,655.514381500318,655.949254802762,656.384128105224,656.819001407706,
657.253874710213,657.689600708326,658.12532670644,658.560200009004,658.995073311601,
659.429946614234,659.864819916905,660.299693219619,660.734566522377,661.169439825183,
661.604313128039,662.039186430948,662.474059733914,662.908933036938,663.343806340025,
663.778679643175,664.213552946393,664.649278944883,665.085004943373,665.519878246733,
665.954751550169,666.389624853683,666.824498157277,667.259371460954,667.694244764717,
668.129118068568,668.563991372509,668.998864676544,669.433737980674,669.868611284901,
670.303484589229,670.738357893659,671.173231198194,671.608957197361,672.044683196528,
672.479556501278,672.91442980614,673.349303111115,673.784176416205,674.219049721412,
674.653923026738,675.088796332185,675.523669637755,675.95854294345,676.393416249271,
676.82828955522,677.263162861298,677.698036167508,678.13290947385,678.568635473934,
679.004361474018,679.439234780629,679.874108087377,680.308981394264,680.743854701289,
681.178728008455,681.613601315762,682.048474623211,682.483347930804,682.91822123854,
683.353094546422,683.78796785445,684.222841162623,684.657714470944,685.092587779412,
685.528313780566,685.96403978172,686.398913090483,686.833786399396,687.268659708457,
687.703533017666,688.138406327025,688.573279636532,689.008152946187,689.443026255992,
689.877899565944,690.312772876043,690.74764618629,691.182519496684,691.617392807224,
692.052266117909,692.487992120169,692.92371812243,693.358591433403,694.228338055774,
694.663211367171,695.098084678707,695.532957990379,695.967831302188,696.402704614131,
696.837577926207,697.707324550749,698.577071175797,699.011944488507,699.447670491767,
699.883396495028,700.318269807975,701.188016434211,702.057763060886,702.927509687976,
703.797256315454,704.667002943295,705.536749571467,706.407348889651,707.277948207973,
708.147694836835,709.017441465911,709.887188095163,710.756934724548,711.626681354026,
712.496427983551,713.367027302543,714.237626621516,715.107373250954,715.977119880277,
716.846866509446,717.716613138419,718.586359767161,719.456106395635,720.32670571363,
721.197305031464,722.067051659126,722.936798286414,723.806544913299,724.676291539758,
725.546038165767,726.415784791305,727.286384106969,728.156983422381,729.026730046663,
729.896476670415,730.331349982088,730.766223293624,731.201096605021,731.635969916278,
732.505716538366,733.37546315988,733.81033647042,734.246062472462,734.681788474505,
735.116661784752,735.551535094852,735.986408404804,736.421281714608,736.856155024264,
737.291028333771,737.72590164313,738.160774952339,738.5956482614,739.030521570312,
739.465394879076,739.900268187692,740.33514149616,740.77001480448,741.205740805414,
741.641466806347,742.076340114374,742.511213422256,742.946086729993,743.380960037585,
743.815833345035,744.250706652341,744.685579959507,745.120453266533,745.555326573419,
745.990199880167,746.425073186778,746.859946493254,747.294819799596,747.729693105806,
748.165419105691,748.601145105576,749.036018411525,749.470891717346,749.90576502304,
750.34063832861,750.775511634057,751.210384939384,751.645258244591,752.080131549682,
752.515004854656,752.949878159518,753.384751464269,753.81962476891,754.254498073445,
754.689371377875,755.125097376885,755.560823375895,755.995696680123,756.430569984253,
756.865443288287,757.300316592228,757.735189896079,758.170063199842,758.604936503519,
759.039809807113,759.474683110627,759.909556414062,760.344429717423,760.779303020711,
761.214176323929,761.649049627079,762.084775625469,762.520501623858,762.955374926883,
763.390248229848,763.825121532758,764.259994835614,764.694868138419,765.129741441178,
765.564614743891,765.999488046563,766.434361349196,766.869234651793,767.304107954357,
767.738981256891,768.173854559398,768.608727861881,769.044453859958,769.480179858035,
769.915053160479,770.349926462907,770.784799765324,771.219673067731,771.654546370133,
772.089419672531,772.52429297493,772.959166277331,773.394039579739,773.828912882155,
774.263786184584,774.698659487028,775.13353278949,775.568406091973,776.004132090072,
776.439858088172,776.874731390706,777.30960469327,777.744477995867,778.1793512985,
778.614224601171,779.049097903885,779.483971206643,779.918844509449,780.353717812305,
780.788591115215,781.22346441818,781.658337721205,782.093211024291,782.528084327442,
782.963810325897,783.399536324352,783.834409627639,784.269282931,784.704156234435,
785.139029537949,785.573902841543,786.00877614522,786.443649448983,786.878522752834,
787.313396056775,787.74826936081,788.183142664939,788.618015969167,789.052889273495,
789.487762577925,789.923488577038,790.359214576152,790.794087880793,791.228961185544,
791.663834490406,792.098707795381,792.533581100471,792.968454405678,793.403327711004,
793.838201016451,794.273074322021,794.707947627716,795.142820933537,795.577694239486,
796.012567545564,796.447440851774,796.883166851791,797.318892851808,797.753766158284,
798.188639464895,798.623512771643,799.058386078529,799.493259385555,799.92813269272,
800.363006000027,800.797879307477,801.232752615069,801.667625922806,802.102499230688,
802.537372538715,802.972245846889,803.40711915521,803.84284515629,804.27857115737,
804.713444465985,805.148317774749,805.583191083662,806.018064392723,806.452937701933,
806.887811011291,807.322684320798,808.192430940258,808.62730425021,809.06217756031,
809.497050870557,809.931924180951,810.36679749149,810.802523493679,811.238249495867,
811.673122806697,812.542869428785,812.977742740041,813.412616051438,813.847489362974,
814.282362674646,814.717235986455,815.152109298398,816.021855922681,816.891602547478,
817.326475860065,817.762201863265,818.197927866466,818.632801179295,819.502547805304,
820.372294431763,821.242041058648,822.111787685935,822.981534313598,823.851280941609,
824.721880259681,825.5924795779,826.462226206642,827.331972835616,828.201719464785,
829.071466094109,829.941212723546,830.810959353053,831.681558672047,832.552157991036,
833.421904620514,834.2916512499,835.161397879151,836.031144508226,836.900891137089,
837.770637765701,838.641237083811,839.511836401767,840.381583029608,841.251329657086,
842.121076284176,842.990822910851,843.860569537087,844.730316162863,845.600915478712,
846.471514794314,847.341261418855,848.211008042874,848.645881354683,849.080754666356,
849.515627977891,849.950501289288,850.82024791166,851.689994533462,852.124867844147,
852.560593846263,852.996319848379,853.431193158772,853.866066469019,854.300939779119,
855.170686398875,855.605559708531,856.040433018038,856.475306327397,856.910179636606,
857.345052945667,857.77992625458,858.214799563344,858.64967287196,859.084546180427,
859.520272181434,859.95599818244,860.390871490614,860.825744798641,861.260618106523,
861.69549141426,862.130364721852,862.565238029302,863.000111336609,863.434984643774,
863.8698579508,864.304731257686,864.739604564434,865.174477871045,865.609351177521,
866.044224483863,866.479950483814,866.915676483765,867.350549789843,867.785423095792,
868.220296401613,868.655169707307,869.090043012877,869.524916318325,869.959789623651,
870.394662928858,870.829536233948,871.264409538923,871.699282843785,872.134156148535,
872.569029453177,873.003902757712,873.439628756773,873.875354755834,874.310228060162,
874.745101364389,875.179974668519,875.614847972553,876.049721276495,876.484594580346,
876.919467884108,877.354341187786,877.78921449138,878.224087794893,878.658961098329,
879.093834401689,879.528707704977,879.963581008195,880.399307006616,880.835033005038,
881.269906308124,881.704779611148,882.139652914114,882.574526217024,883.00939951988,
883.444272822685,883.879146125444,884.314019428157,884.748892730829,885.183766033462,
885.618639336059,886.053512638623,886.488385941157,886.923259243664,887.358985241751,
887.794711239839,888.2295845423,888.664457844744,889.099331147173,889.534204449589,
889.969077751997,890.403951054398,890.838824356797,891.273697659195,891.708570961597,
892.143444264004,892.578317566421,893.01319086885,893.448064171293,893.882937473755,
894.318663471843,894.75438946993,895.189262772437,895.624136074971,896.059009377535,
896.493882680132,896.928755982765,897.363629285437,897.798502588151,898.233375890909,
898.668249193715,899.103122496571,899.53799579948,899.972869102446,900.40774240547,
900.842615708556,901.278341706978,901.714067705399,902.148941008617,902.583814311905,
903.018687615265,903.453560918701,903.888434222214,904.323307525808,904.758180829485,
905.193054133248,905.627927437099,906.06280074104,906.497674045075,906.932547349205,
907.367420653433,907.80229395776,908.238019956821,908.673745955883,909.108619260417,
909.543492565059,909.978365869809,910.413239174671,910.848112479646,911.282985784736,
911.717859089943,912.152732395269,912.587605700716,913.022479006287,913.457352311981,
913.892225617802,914.327098923751,914.761972229829,915.19769822978,915.633424229731,
916.068297536072,916.503170842548,916.93804414916,917.372917455908,917.807790762794,
918.24266406982,918.677537376985,919.112410684292,919.547283991742,919.982157299334,
920.417030607071,920.851903914953,921.28677722298,921.721650531154,922.15737653216,
922.593102533167,923.027975841635,923.46284915025,923.897722459014,924.332595767926,
924.767469076987,925.202342386197,925.637215695556,926.072089005063,926.506962314719,
926.941835624523,927.376708934475,927.811582244575,928.246455554822,928.681328865215,
929.117054867331,929.987654180132,930.422527490961,930.857400801934,931.292274113049,
931.727147424306,932.162020735703,932.596894047238,933.46664067072,934.336387294739,
934.771260606945,935.20613391928,935.641007231742,936.076733234882,936.94733255073,
937.817079176507,938.686825802743,939.556572429418,940.426319056508,941.296065683986,
942.165812311827,943.036411629783,943.907010947893,944.776757576505,945.646504205367,
946.516250834443,947.385997463694,948.25574409308,949.125490722558,949.996090041546,
950.86668936054,951.736435990048,952.606182619485,953.475929248809,954.345675877978,
955.215422506951,956.085169135693,956.955768453912,957.826367771985,958.696114399995,
959.565861027658,960.435607654946,961.305354281831,962.175100908289,963.044847534298,
963.915446850328,964.786046166116,965.655792790913,966.525539415195,966.960412727138,
967.395286038947,968.265032662155,969.134779284809,969.569652595924,970.004525906897,
970.439399217726,970.875125219914,971.310851222103,971.745724532643,972.615471153283,
973.485217773335,973.920091083139,974.354964392795,974.789837702302,975.22471101166,
975.65958432087,976.094457629931,976.529330938844,976.964204247608,977.399077556223,
977.834803557303,978.270529558383,978.705402866704,979.140276174877,979.575149482905,
980.010022790786,980.444896098523,980.879769406116,981.314642713565,981.749516020872,
982.184389328038,982.619262635063,983.05413594195,983.489009248698,983.923882555309,
984.358755861785,984.794481861802,985.230207861819,985.665081168029,986.099954474107,
986.534827780056,986.969701085877,987.404574391571,987.839447697141,988.274321002589,
988.709194307915,989.144067613122,989.578940918212,990.013814223187,990.448687528048,
990.883560832799,991.31843413744,991.754160136554,992.189886135667,992.624759440097,
993.059632744425,993.494506048653,993.929379352783,994.364252656817,994.799125960758,
995.233999264609,995.668872568372,996.103745872049,996.538619175643,996.973492479157,
997.408365782593,997.843239085953,998.278112389241,998.713838387696,999.149564386151,
999.584437689301,1000.01931099239,1000.45418429541,1000.88905759838,1001.32393090129,
1001.75880420414,1002.19367750695,1002.62855080971,1003.06342411242,1003.49829741509,
1003.93317071773,1004.36804402032,1004.80291732289,1005.23779062542,1005.67351662352,
1006.10924262162,1006.5441159241,1006.97898922656,1007.41386252901,1007.84873583144,
1008.28360913385,1008.71848243626,1009.15335573866,1009.58822904106,1010.02310234346,
1010.45797564586,1010.89284894827,1011.32772225069,1011.76259555311,1012.19746885556,
1012.63319485364,1013.06892085171,1013.5037941542,1013.9386674567,1014.37354075924,
1014.8084140618,1015.2432873644,1015.67816066703,1016.1130339697,1016.54790727242,
1016.98278057517,1017.41765387798,1017.85252718084,1018.28740048375,1018.72227378671,
1019.15714708974,1019.59287308813,1020.02859908651,1020.46347238967,1020.89834569288,
1021.33321899617,1021.76809229953,1022.20296560297,1022.63783890648,1023.07271221007,
1023.50758551375,1023.94245881752,1024.37733212137,1024.81220542531,1025.24707872935,
1025.68195203348,1026.11682533771,1026.55255133672,1026.98827733573,1027.42315064016,
1027.8580239447,1028.29289724934,1028.72777055409,1029.16264385896,1029.59751716393,
1030.03239046902,1030.46726377423,1030.90213707956,1031.33701038501,1031.77188369058,
1032.20675699628,1032.6416303021,1033.07650360805,1033.51222960793,1033.94795560782,
1034.38282891403,1034.81770222038,1035.25257552685,1035.68744883347,1036.12232214022,
1036.5571954471,1036.99206875413,1037.4269420613,1037.86181536861,1038.29668867606,
1038.73156198365,1039.16643529139,1039.60130859927,1040.0361819073,1040.47190790824,
1040.90763390917,1041.34250721749,1041.77738052596,1042.21225383458,1042.64712714334,
1043.08200045226,1043.95174707053,1044.38662037989,1044.8214936894,1045.25636699906,
1045.69124030886,1046.12611361882,1046.56098692892,1046.99586023917,1047.43158624121,
1047.86731224325,1048.3021855538,1048.73705886448,1049.17193217531,1049.60680548629,
1050.0416787974,1050.47655210866,1050.91142542006,1051.78117204327,1052.21604535508,
1052.65091866703,1053.0857919791,1053.52066529131,1053.95553860365,1054.39126460673,
1055.26186392239,1056.13161054793,1057.00135717395,1057.43623048712,1057.87110380041,
1058.7408504273,1059.61059705459,1060.48034368225,1061.35094300009,1062.22154231809,
1063.09128894656,1063.96103557531,1064.83078220429,1065.70052883346,1066.57027546278,
1067.44002209222,1068.3106214112,1069.18122073019,1070.05096735972,1070.9207139892,
1071.79046061859,1072.66020724785,1073.52995387693,1074.39970050579,1075.27029982411,
1076.1408991423,1077.01064577048,1077.88039239832,1078.7501390258,1079.61988565289,
1080.48963227957,1081.35937890581,1082.22997822202,1083.100577538,1083.97032416305,
1084.84007078759,1085.70981741161,1086.5795640351,1087.44931065803,1087.88418396929,
1088.31905728041,1088.75393059138,1089.18965659365,1089.62538259591,1090.06025590659,
1090.93000252753,1091.36487583778,1091.79974914788,1092.23462245783,1092.66949576764,
1093.1043690773,1093.5392423868,1093.97411569616,1094.40898900538,1094.84386231444,
1095.27873562335,1095.71360893212,1096.14933493327,1096.58506093443,1097.0199342429,
1097.45480755122,1097.88968085939,1098.32455416742,1098.75942747531,1099.19430078305,
1099.62917409064,1100.06404739809,1100.4989207054,1100.93379401257,1101.36866731959,
1101.80354062648,1102.23841393323,1102.67328723984,1103.10901323993,1103.54473924001,
1103.97961254636,1104.41448585257,1104.84935915865,1105.2842324646,1105.71910577042,
1106.15397907612,1106.58885238169,1107.02372568714,1107.45859899246,1107.89347229767,
1108.32834560276,1108.76321890774,1109.1980922126,1109.63296551736,1110.06869151652,
1110.50441751569,1110.93929082023,1111.37416412466,1111.80903742899,1112.24391073322,
1112.67878403735,1113.11365734139,1113.54853064533,1113.98340394918,1114.41827725295,
1114.85315055662,1115.28802386022,1115.72289716374,1116.15777046717,1116.59264377053,
1117.02836976903,1117.46409576752,1117.89896907074,1118.33384237389,1118.76871567698,
1119.20358898,1119.63846228297,1120.07333558588,1120.50820888874,1120.94308219154,
1121.3779554943,1121.81282879702,1122.24770209969,1122.68257540233,1123.11744870492,
1123.55232200749,1123.98804800561,1124.42377400372,1124.85864730623,1125.29352060871,
1125.72839391118,1126.16326721362,1126.59814051605,1127.03301381847,1127.46788712088,
1127.90276042328,1128.33763372568,1128.77250702808,1129.20738033048,1129.64225363289,
1130.07712693531,1130.51200023774,1130.94772623581,1131.38345223388,1131.81832553634,
1132.25319883883,1132.68807214134,1133.12294544387,1133.55781874644,1133.99269204904,
1134.42756535167,1134.86243865434,1135.29731195706,1135.73218525982,1136.16705856263,
1136.60193186548,1137.03680516839,1137.47167847136,1137.90740446972,1138.34313046808,
1138.77800377117,1139.21287707432,1139.64775037754,1140.08262368083,1140.51749698419,
1140.95237028763,1141.38724359114,1141.82211689474,1142.25699019842,1142.69186350218,
1143.12673680603,1143.56161010998,1143.99648341401,1144.43135671814,1144.86708271711,
1145.30280871607,1145.7376820204,1146.17255532483,1146.60742862936,1147.04230193401,
1147.47717523876,1147.91204854362,1148.3469218486,1148.78179515369,1149.2166684589,
1149.65154176423,1150.08641506968,1150.52128837525,1150.95616168094,1151.39103498677,
1151.82676098659,1152.26248698641,1152.69736029249,1153.1322335987,1153.56710690504,
1154.00198021152,1154.43685351813,1154.87172682488,1155.30660013177,1155.7414734388,
1156.17634674597,1156.61122005327,1157.04609336073,1157.48096666832,1157.91583997606,
1158.35071328394,1158.7864392848,1159.22216528566,1159.65703859384,1160.09191190216,
1160.52678521063,1160.96165851925,1161.39653182801,1161.83140513693,1162.26627844599,
1162.7011517552,1163.13602506456,1163.57089837407,1164.00577168373,1164.44064499353,
1164.87551830349,1165.74611761556,1166.18184361753,1166.61671692792,1167.05159023846,
1167.48646354915,1167.92133685998,1168.35621017096,1169.22595679333,1170.09570341627,
1170.53057672794,1170.96545003975,1171.4003233517,1171.83519666377,1172.27006997598,
1172.705795979,1173.57639529447,1174.44614191977,1174.8810152326,1175.31588854555,
1176.18563517179,1177.05538179847,1177.92512842556,1178.79487505304,1179.66547437075,
1180.53607368863,1181.40582031696,1182.27556694557,1183.14531357444,1184.01506020352,
1184.88480683277,1185.75455346216,1186.62515278112,1187.4957521001,1188.36549872963,
1189.23524535914,1190.10499198858,1190.97473861791,1191.84448524708,1192.71423187606,
1193.58483119448,1194.45543051277,1195.3251771411,1196.19492376911,1197.06467039678,
1197.93441702407,1198.80416365096,1199.67391027742,1200.5445095938,1201.41510890996,
1202.28485553525,1203.15460216005,1204.02434878434,1204.89409540809,1205.76384203131,
1206.1987153427,1206.63358865396,1207.06846196508,1207.50418796741,1208.37478728058,
1209.2445339018,1209.6794072122,1210.11428052245,1210.54915383255,1210.9840271425,
1211.41890045231,1211.85377376197,1212.28864707147,1212.72352038083,1213.15839369005,
1213.59326699911,1214.02814030802,1214.46386630925,1214.89959231048,1215.3344656191,
1215.76933892757,1216.20421223589,1216.63908554406,1217.07395885209,1217.50883215998,
1217.94370546771,1218.37857877531,1218.81345208276,1219.24832539007,1219.68319869724,
1220.11807200426,1220.55294531115,1220.9878186179,1221.42354461805,1221.85927061821,
1222.29414392468,1222.72901723103,1223.16389053724,1223.59876384332,1224.03363714927,
1224.46851045509,1224.90338376079,1225.33825706636,1225.77313037181,1226.20800367713,
1226.64287698234,1227.07775028743,1227.51262359241,1227.94749689727,1228.3832228965,
1228.81894889572,1229.25382220036,1229.6886955049,1230.12356880933,1230.55844211366,
1230.99331541789,1231.42818872202,1231.86306202606,1232.29793533,1232.73280863385,
1233.16768193762,1233.60255524129,1234.03742854489,1234.4723018484,1234.90717515184,
1235.34290115037,1235.7786271489,1236.21350045219,1236.64837375541,1237.08324705856,
1237.51812036165,1237.95299366467,1238.38786696764,1238.82274027055,1239.25761357341,
1239.69248687621,1240.12736017897,1240.56223348169,1240.99710678436,1241.431980087,
1241.8668533896,1242.30257938773,1242.73830538585,1243.17317868839,1243.6080519909,
1244.04292529338,1244.47779859585,1244.91267189829,1245.34754520072,1245.78241850314,
1246.21729180555,1246.65216510795,1247.08703841035,1247.52191171275,1247.95678501515,
1248.39165831756,1248.82653161998,1249.26225761804,1249.69798361611,1250.13285691855,
1250.56773022101,1251.0026035235,1251.43747682601,1251.87235012854,1252.30722343111,
1252.74209673371,1253.17697003634,1253.61184333901,1254.04671664173,1254.48158994449,
1254.9164632473,1255.35133655015,1255.78620985306,1256.22193585139,1256.65766184973,
1257.09253515275,1257.52740845584,1257.96228175899,1258.39715506221,1258.8320283655,
1259.26690166886,1259.7017749723,1260.13664827581,1260.57152157941,1261.00639488309,
1261.44126818685,1261.8761414907,1262.31101479465,1262.74588809868,1263.1816140976,
1263.61734009651,1264.05221340074,1264.48708670507,1264.9219600095,1265.35683331403,
1265.79170661868,1266.22657992343,1266.66145322829,1267.09632653327,1267.53119983836,
1267.96607314357,1268.4009464489,1268.83581975434,1269.27069305992,1269.70556636561,
1270.14129236537,1270.57701836513,1271.01189167108,1271.44676497716,1271.88163828337,
1272.31651158971,1272.75138489619,1273.1862582028,1273.62113150955,1274.05600481644,
1274.49087812347,1274.92575143063,1275.36062473794,1275.79549804539,1276.23037135299,
1276.66524466073,1277.10097066151,1277.5366966623,1277.97156997033,1278.40644327851,
1278.84131658683,1279.2761898953,1279.71106320392,1280.14593651268,1280.5808098216,
1281.01568313066,1281.45055643987,1281.88542974923,1282.32030305874,1282.75517636839,
1283.1900496782,1283.62492298815,1284.06064899005,1284.49637499195,1284.9312483022,
1285.36612161259,1285.80099492313,1286.23586823382,1286.67074154465,1287.54048816674,
1287.975361478,1288.4102347894,1288.84510810093,1289.27998141261,1289.71485472442,
1290.14972803636,1291.02032735139,1291.89092666668,1292.32579997914,1292.76067329173,
1293.19554660444,1293.63041991727,1294.50016654328,1295.36991316974,1296.23965979663,
1297.10940642392,1297.9800057415,1298.85060505925,1299.72035168742,1300.5900983159,
1301.45984494464,1302.32959157362,1303.19933820279,1304.06908483212,1304.93968415104,
1305.81028347,1306.68003009953,1307.54977672906,1308.41952335854,1309.28926998793,
1310.15901661718,1311.02876324626,1311.89936256477,1312.76996188316,1313.63970851164,
1314.50945513981,1315.37920176765,1316.24894839514,1317.11869502223,1317.98844164891,
1318.85904096546,1319.72964028179,1320.59938690733,1321.46913353238,1322.33888015692,
1323.20862678095,1323.64350009276,1324.07837340443,1324.51324671597,1324.94812002737,
1325.81871934103,1326.68931865441,1327.12419196524,1327.55906527593,1327.99393858647,
1328.42881189686,1328.86368520711,1329.29855851721,1329.73343182716,1330.16830513697,
1330.60317844663,1331.03805175614,1331.4729250655,1331.90779837471,1332.34267168377,
1332.77839768507,1333.21412368638,1333.64899699514,1334.08387030376,1334.51874361223,
1334.95361692055,1335.38849022873,1335.82336353676,1336.25823684464,1336.69311015238,
1337.12798345997,1337.56285676742,1337.99773007473,1338.4326033819,1338.86747668892,
1339.30234999581,1339.73807599603,1340.17380199625,1340.60867530287,1341.04354860934,
1341.47842191569,1341.9132952219,1342.34816852798,1342.78304183393,1343.21791513975,
1343.65278844545,1344.08766175102,1344.52253505647,1344.95740836179,1345.392281667,
1345.82715497209,1346.26202827707,1346.69775427635,1347.13348027563,1347.56835358038,
1348.00322688502,1348.43810018956,1348.87297349399,1349.30784679832,1349.74272010255,
1350.17759340668,1350.61246671072,1351.04734001466,1351.48221331851,1351.91708662228,
1352.35195992595,1352.78683322955,1353.22170653306,1353.65743253163,1354.09315853019,
1354.52803183356,1354.96290513685,1355.39777844007,1355.83265174322,1356.26752504631,
1356.70239834933,1357.1372716523,1357.57214495521,1358.00701825807,1358.44189156087,
1358.87676486363,1359.31163816635,1359.74651146902,1360.18138477166,1360.6171107698,
1361.05283676795,1361.48771007051,1361.92258337305,1362.35745667556,1362.79232997804,
1363.2272032805,1363.66207658295,1364.09694988538,1364.5318231878,1364.96669649021,
1365.40156979261,1365.83644309501,1366.27131639741,1366.70618969981,1367.14106300222,
1367.57678900028,1368.01251499834,1368.44738830077,1368.88226160321,1369.31713490567,
1369.75200820816,1370.18688151067,1370.6217548132,1371.05662811577,1371.49150141837,
1371.926374721,1372.36124802367,1372.79612132639,1373.23099462915,1373.66586793196,
1374.10074123481,1374.53646723311,1374.97219323142,1375.40706653438,1375.84193983741,
1376.2768131405,1376.71168644365,1377.14655974687,1377.58143305016,1378.01630635352,
1378.45117965696,1378.88605296047,1379.32092626407,1379.75579956775,1380.19067287151,
1380.62554617536,1381.06041947931,1381.49614547817,1381.93187147704,1382.36674478117,
1382.8016180854,1383.23649138973,1383.67136469416,1384.10623799869,1384.54111130334,
1384.97598460809,1385.41085791295,1385.84573121793,1386.28060452302,1386.71547782823,
1387.15035113356,1387.585224439,1388.02009774458,1388.45582374427,1388.89154974397,
1389.32642304979,1389.76129635574,1390.19616966182,1390.63104296803,1391.06591627437,
1391.50078958085,1391.93566288746,1392.37053619421,1392.8054095011,1393.24028280813,
1393.6751561153,1394.1100294226,1394.54490273005,1394.97977603765,1395.41550203836,
1395.85122803908,1396.28610134696,1396.72097465499,1397.15584796317,1397.59072127149,
1398.02559457996,1398.46046788858,1398.89534119734,1399.33021450626,1399.76508781532,
1400.19996112453,1400.63483443389,1401.50458105306,1401.93945436286,1402.37518036469,
1402.81090636651,1403.24577967661,1403.68065298686,1404.11552629725,1404.5503996078,
1404.98527291848,1405.85501954029,1406.2898928514,1406.72476616266,1407.15963947406,
1407.5945127856,1408.02938609727,1408.46425940908,1409.33485872391,1410.205458039,
1410.64033135134,1411.07520466381,1411.51007797639,1411.9449512891,1412.81469791488,
1413.68444454112,1414.5541911678,1415.42393779489,1416.29453711233,1417.16513642995,
1418.03488305796,1418.90462968629,1419.77437631491,1420.64412294377,1421.51386957285,
1422.38361620211,1423.25421552099,1424.12481483992,1424.99456146943,1425.86430809896,
1426.73405472847,1427.60380135791,1428.47354798724,1429.34329461641,1430.21389393501,
1431.08449325349,1431.9542398821,1432.82398651043,1433.69373313844,1434.56347976611,
1435.4332263934,1436.30297302029,1437.17357233701,1438.04417165351,1438.91391827929,
1439.78366490459,1440.65341152939,1441.52315815367,1441.95803146562,1442.39290477743,
1442.8277780891,1443.26265140064,1444.13325071451,1445.00385002811,1445.43872333908,
1445.87359664991,1446.3084699606,1446.74334327114,1447.17821658153,1447.61308989178,
1448.48283651184,1448.91770982164,1449.3525831313,1449.78745644081,1450.22232975017,
1450.65720305938,1451.09292906076,1451.52865506214,1451.96352837105,1452.39840167982,
1452.83327498843,1453.2681482969,1453.70302160522,1454.1378949134,1454.57276822143,
1455.00764152931,1455.44251483705,1455.87738814464,1456.31226145209,1456.7471347594,
1457.18200806657,1457.6168813736,1458.05260737389,1458.48833337418,1458.92320668093,
1459.35807998754,1459.79295329402,1460.22782660036,1460.66269990657,1461.09757321265,
1461.5324465186,1461.96731982443,1462.40219313012,1462.83706643569,1463.27193974114,
1463.70681304647,1464.14168635168,1464.57655965677,1465.0122856561,1465.44801165544,
1465.8828849603,1466.31775826505,1466.7526315697,1467.18750487423,1467.62237817866,
1468.05725148299,1468.49212478722,1468.92699809135,1469.36187139539,1469.79674469933,
1470.23161800319,1470.66649130695,1471.10136461063,1471.53623791422,1471.97196391283,
1472.40768991143,1472.84256321487,1473.27743651823,1473.71230982152,1474.14718312474,
1474.58205642789,1475.01692973098,1475.451803034,1475.88667633697,1476.32154963988,
1476.75642294274,1477.19129624555,1477.62616954831,1478.06104285102,1478.4959161537,
1478.93164215186,1479.36736815002,1479.80224145262,1480.23711475519,1480.67198805772,
1481.10686136023,1481.54173466272,1481.97660796518,1482.41148126762,1482.84635457005,
1483.28122787247,1483.71610117488,1484.15097447728,1484.58584777968,1485.02072108208,
1485.45559438449,1485.89132038254,1486.32704638059,1486.76191968301,1487.19679298544,
1487.63166628788,1488.06653959035,1488.50141289283,1488.93628619534,1489.37115949787,
1489.80603280044,1490.24090610304,1490.67577940567,1491.11065270835,1491.54552601106,
1491.98039931382,1492.41527261663,1492.8509986149,1493.28672461318,1493.72159791609,
1494.15647121906,1494.59134452208,1495.02621782517,1495.46109112832,1495.89596443154,
1496.33083773483,1496.76571103819,1497.20058434163,1497.63545764515,1498.07033094874,
1498.50520425242,1498.94007755618,1499.37495086004,1499.81067685885,1500.24640285767,
1500.68127616171,1501.11614946584,1501.55102277007,1501.9858960744,1502.42076937883,
1502.85564268337,1503.29051598801,1503.72538929276,1504.16026259762,1504.5951359026,
1505.03000920769,1505.4648825129,1505.89975581823,1506.33462912368,1506.77035512331,
1507.20608112294,1507.64095442864,1508.07582773446,1508.51070104041,1508.94557434649,
1509.3804476527,1509.81532095904,1510.25019426552,1510.68506757213,1511.11994087888,
1511.55481418577,1511.9896874928,1512.42456079996,1512.85943410727,1513.29430741472,
1513.73003341537,1514.16575941601,1514.60063272375,1515.03550603163,1515.47037933966,
1515.90525264784,1516.34012595616,1516.77499926463,1517.20987257325,1517.64474588201,
1518.07961919093,1518.51449249999,1518.9493658092,1519.38423911856,1519.81911242807,
1520.25398573772,1520.68971173947,1521.12543774122,1521.56031105118,1521.99518436128,
1522.43005767153,1523.29980429246,1523.73467760315,1524.16955091398,1524.60442422495,
1525.03929753607,1525.47417084733,1525.90904415873,1526.77879078194,1527.64939009657,
1528.08511609939,1528.51998941146,1528.95486272367,1529.38973603601,1530.25948266106,
1531.1292292866,1531.99897591261,1532.86872253907,1533.73846916596,1534.60906848325,
1535.47966780073,1536.34941442858,1537.21916105675,1538.08890768523,1538.95865431398,
1539.82840094295,1540.69814757212,1541.56874689096,1542.43934620985,1543.30909283933,
1544.17883946886,1545.04858609839,1545.91833272787,1546.78807935726,1547.65782598651,
1548.52842530518,1549.39902462375,1550.26877125249,1551.13851788097,1552.00826450914,
1552.87801113699,1553.74775776447,1554.61750439156,1555.48810370844,1556.35870302511,
1557.22844965112,1558.09819627666,1558.96794290171,1559.83768952626,1560.27256283834,
1560.70743615028,1561.57718277377,1562.44778208785,1563.31838140165,1563.75325471277,
1564.18812802374,1564.62300133457,1565.05787464526,1565.9276212662,1566.79736788655,
1567.2322411965,1567.66711450631,1568.10198781596,1568.53686112547,1568.97173443483,
1569.40746043628,1569.84318643774,1570.2780597468,1570.71293305571,1571.14780636448,
1571.5826796731,1572.01755298157,1572.45242628989,1572.88729959806,1573.32217290609,
1573.75704621397,1574.19191952171,1574.62679282931,1575.06166613676,1575.49653944407,
1575.93141275123,1576.36713875159,1576.80286475195,1577.23773805884,1577.67261136559,
1578.1074846722,1578.54235797868,1578.97723128502,1579.41210459124,1579.84697789732,
1580.28185120327,1580.71672450909,1581.15159781478,1581.58647112036,1582.0213444258,
1582.45621773113,1582.89109103634,1583.32681703573,1583.76254303513,1584.1974163401,
1584.63228964497,1585.06716294972,1585.50203625436,1585.9369095589,1586.37178286333,
1586.80665616766,1587.24152947189,1587.67640277602,1588.11127608005,1588.546149384,
1588.98102268785,1589.41589599161,1589.85076929529,1590.28649529394,1590.72222129258,
1591.1570945961,1591.59196789953,1592.0268412029,1592.46171450619,1592.8965878094,
1593.33146111256,1593.76633441564,1594.20120771867,1594.63608102164,1595.07095432455,
1595.50582762741,1595.94070093021,1596.37557423297,1596.81044753569,1597.24617353387,
1597.68189953206,1598.11677283469,1598.55164613729,1598.98651943985,1599.42139274239,
1599.8562660449,1600.29113934738,1600.72601264985,1601.16088595229,1601.59575925472,
1602.03063255714,1602.46550585955,1602.90037916195,1603.33525246435,1603.77012576675,
1604.2058517648,1604.64157776285,1605.07645106526,1605.51132436768,1605.94619767011,
1606.38107097255,1606.81594427502,1607.2508175775,1607.68569088001,1608.12056418254,
1608.55543748511,1608.99031078771,1609.42518409034,1609.86005739302,1610.29493069573,
1610.72980399849,1611.16552999674,1611.60125599499,1612.03612929785,1612.47100260076,
1612.90587590373,1613.34074920675,1613.77562250984,1614.21049581299,1614.64536911621,
1615.0802424195,1615.51511572286,1615.9499890263,1616.38486232981,1616.81973563341,
1617.25460893709,1617.68948224085,1618.12520823963,1618.5609342384,1618.99580754234,
1619.43068084638,1619.86555415051,1620.30042745474,1620.73530075907,1621.1701740635,
1621.60504736804,1622.03992067268,1622.47479397743,1622.90966728229,1623.34454058727,
1623.77941389236,1624.21428719757,1624.6491605029,1625.08488650247,1625.52061250204,
1625.95548580761,1626.39035911331,1626.82523241913,1627.26010572508,1627.69497903116,
1628.12985233737,1628.56472564372,1628.99959895019,1629.43447225681,1629.86934556356,
1630.30421887044,1630.73909217747,1631.17396548464,1631.60883879195,1632.04456479252,
1632.48029079309,1632.91516410068,1633.35003740842,1633.78491071631,1634.21978402433,
1634.65465733251,1635.08953064083,1635.5244039493,1635.95927725792,1636.39415056668,
1636.8290238756,1637.26389718466,1637.69877049387,1638.13364380323,1638.56851711274,
1639.00424311442,1639.43996911609,1639.8748424259,1640.30971573585,1640.74458904595,
1641.6143356666,1642.04920897714,1642.48408228782,1642.91895559865,1643.35382890963,
1643.78870222074,1644.223575532,1645.09332215494,1645.52819546661,1645.96392146936,
1646.39964747212,1646.83452078406,1647.26939409614,1647.70426740834,1648.57401403314,
1649.44376065844,1650.31350728422,1650.74838059729,1651.18325391046,1652.05300053714,
1652.92359985428,1653.79419917162,1654.66394579929,1655.5336924273,1656.40343905563,
1657.27318568424,1658.14293231311,1659.01267894219,1659.88327826096,1660.75387757982,
1661.62362420926,1662.49337083877,1663.3631174683,1664.23286409781,1665.10261072725,
1665.97235735658,1666.84295667531,1667.71355599396,1668.58330262282,1669.45304925143,
1670.32279587976,1671.19254250778,1672.06228913544,1672.93203576273,1673.80263507977,
1674.6732343966,1675.54298102284,1676.41272764862,1677.28247427392,1678.15222089872,
1679.021967523,1679.89171414676,1680.76231346105,1681.19803946366,1681.63291277506,
1682.06778608632,1682.50265939743,1682.93753270841,1683.37240601924,1684.24215264047,
1684.67702595086,1685.11189926111,1685.54677257121,1685.98164588116,1686.41651919097,
1686.85139250063,1687.28626581014,1687.72199181166,1688.15771781319,1688.5925911224,
1689.02746443146,1689.46233774038,1689.89721104914,1690.33208435776,1690.76695766623,
1691.20183097455,1691.63670428272,1692.07157759075,1692.50645089864,1692.94132420637,
1693.37619751397,1693.81107082142,1694.24594412873,1694.68167012916,1695.11739612959,
1695.55226943662,1695.9871427435,1696.42201605025,1696.85688935687,1697.29176266334,
1697.72663596969,1698.1615092759,1698.59638258198,1699.03125588793,1699.46612919375,
1699.90100249945,1700.33587580502,1700.77074911047,1701.20562241579,1701.64134841525,
1702.0770744147,1702.51194771979,1702.94682102476,1703.38169432963,1703.81656763438,
1704.25144093902,1704.68631424356,1705.12118754799,1705.55606085232,1705.99093415655,
1706.42580746068,1706.86068076471,1707.29555406866,1707.73042737251,1708.16530067627,
1708.60102667496,1709.03675267365,1709.47162597724,1709.90649928076,1710.34137258419,
1710.77624588756,1711.21111919085,1711.64599249406,1712.08086579722,1712.5157391003,
1712.95061240333,1713.3854857063,1713.82035900921,1714.25523231207,1714.69010561487,
1715.12497891763,1715.56070491584,1715.99643091404,1716.43130421671,1716.86617751935,
1717.30105082195,1717.73592412451,1718.17079742705,1718.60567072956,1719.04054403204,
1719.4754173345,1719.91029063695,1720.34516393938,1720.7800372418,1721.21491054421,
1721.64978384661,1722.08465714901,1722.52038314706,1722.9561091451,1723.39098244751,
1723.82585574992,1724.26072905233,1724.69560235476,1725.13047565721,1725.56534895967,
1726.00022226216,1726.43509556467,1726.8699688672,1727.30484216977,1727.73971547236,
1728.174588775,1728.60946207767,1729.04433538039,1729.48006137861,1729.91578737684,
1730.35066067965,1730.78553398251,1731.22040728542,1731.65528058838,1732.09015389141,
1732.5250271945,1732.95990049765,1733.39477380087,1733.82964710416,1734.26452040752,
1734.69939371096,1735.13426701447,1735.56914031807,1736.00401362175,1736.43973962048,
1736.8754656192,1737.31033892306,1737.745212227,1738.18008553104,1738.61495883517,
1739.0498321394,1739.48470544373,1739.91957874816,1740.35445205269,1740.78932535734,
1741.22419866209,1741.65907196695,1742.09394527193,1742.52881857702,1742.96369188223,
1743.39941788174,1743.83514388125,1744.2700171867,1744.70489049227,1745.13976379797,
1745.57463710379,1746.00951040974,1746.44438371582,1746.87925702203,1747.31413032837,
1747.74900363485,1748.18387694146,1748.61875024821,1749.0536235551,1749.48849686213,
1749.92337016929,1750.3590961698,1750.7948221703,1751.22969547775,1751.66456878534,
1752.09944209308,1752.53431540096,1752.96918870899,1753.40406201717,1753.83893532549,
1754.27380863396,1754.70868194258,1755.14355525134,1755.57842856026,1756.01330186932,
1756.44817517853,1756.88304848789,1757.31877448949,1757.75450049109,1758.18937380075,
1759.05912042051,1759.49399373061,1759.92886704086,1760.36374035125,1760.79861366179,
1761.23348697248,1761.66836028331,1762.10323359429,1762.5381069054,1763.40785352806,
1763.8427268396,1764.27845284228,1764.71417884496,1765.14905215677,1765.58392546872,
1766.0187987808,1766.88854540534,1767.75829203039,1768.1931653431,1768.62803865593,
1769.06291196888,1769.49778528195,1770.36753190841,1771.2381312254,1772.10873054259,
1772.97847717007,1773.84822379791,1774.71797042609,1775.58771705456,1776.45746368331,
1777.32721031228,1778.19780963089,1779.06840894783,1779.93815555508,1780.80790201176,
1781.67764871408),.UNSPECIFIED.) ;
#833=B_SPLINE_SURFACE_WITH_KNOTS('',1,3,((#88677,#88678,#88679,#88680,#88681,
#88682,#88683,#88684,#88685,#88686,#88687,#88688,#88689,#88690,#88691,#88692,
#88693,#88694,#88695,#88696,#88697,#88698,#88699,#88700,#88701,#88702,#88703,
#88704,#88705,#88706,#88707,#88708,#88709,#88710,#88711,#88712,#88713,#88714,
#88715,#88716,#88717,#88718,#88719,#88720,#88721,#88722,#88723,#88724,#88725,
#88726,#88727,#88728,#88729,#88730,#88731,#88732,#88733,#88734,#88735,#88736,
#88737,#88738,#88739,#88740,#88741,#88742,#88743,#88744,#88745,#88746,#88747,
#88748,#88749,#88750,#88751,#88752,#88753,#88754,#88755,#88756,#88757,#88758,
#88759,#88760,#88761,#88762,#88763,#88764,#88765,#88766,#88767,#88768,#88769,
#88770,#88771,#88772,#88773,#88774,#88775,#88776,#88777,#88778,#88779,#88780,
#88781,#88782,#88783,#88784,#88785,#88786,#88787,#88788,#88789,#88790,#88791,
#88792,#88793,#88794,#88795,#88796,#88797,#88798,#88799,#88800,#88801,#88802,
#88803,#88804,#88805,#88806,#88807,#88808,#88809,#88810,#88811,#88812,#88813,
#88814,#88815,#88816,#88817,#88818,#88819,#88820,#88821,#88822,#88823,#88824,
#88825,#88826,#88827,#88828,#88829,#88830,#88831,#88832,#88833,#88834,#88835,
#88836,#88837,#88838,#88839,#88840,#88841,#88842,#88843,#88844,#88845,#88846,
#88847,#88848,#88849,#88850,#88851,#88852,#88853,#88854,#88855,#88856,#88857,
#88858,#88859,#88860,#88861,#88862,#88863,#88864,#88865,#88866,#88867,#88868,
#88869,#88870,#88871,#88872,#88873,#88874,#88875,#88876,#88877,#88878,#88879,
#88880,#88881,#88882,#88883,#88884,#88885,#88886,#88887,#88888,#88889,#88890,
#88891,#88892,#88893,#88894,#88895,#88896,#88897,#88898,#88899,#88900,#88901,
#88902,#88903,#88904,#88905,#88906,#88907,#88908,#88909,#88910,#88911,#88912,
#88913,#88914,#88915,#88916,#88917,#88918,#88919,#88920,#88921,#88922,#88923,
#88924,#88925,#88926,#88927,#88928,#88929,#88930,#88931,#88932,#88933,#88934,
#88935,#88936,#88937,#88938,#88939,#88940,#88941,#88942,#88943,#88944,#88945,
#88946,#88947,#88948,#88949,#88950,#88951,#88952,#88953,#88954,#88955,#88956,
#88957,#88958,#88959,#88960,#88961,#88962,#88963,#88964,#88965,#88966,#88967,
#88968,#88969,#88970,#88971,#88972,#88973,#88974,#88975,#88976,#88977,#88978,
#88979,#88980,#88981,#88982,#88983,#88984,#88985,#88986,#88987,#88988,#88989,
#88990,#88991,#88992,#88993,#88994,#88995,#88996,#88997,#88998,#88999,#89000,
#89001,#89002,#89003,#89004,#89005,#89006,#89007,#89008,#89009,#89010,#89011,
#89012,#89013,#89014,#89015,#89016,#89017,#89018,#89019,#89020,#89021,#89022,
#89023,#89024,#89025,#89026,#89027,#89028,#89029,#89030,#89031,#89032,#89033,
#89034,#89035,#89036,#89037,#89038,#89039,#89040,#89041,#89042,#89043,#89044,
#89045,#89046,#89047,#89048,#89049,#89050,#89051,#89052,#89053,#89054,#89055,
#89056,#89057,#89058,#89059,#89060,#89061,#89062,#89063,#89064,#89065,#89066,
#89067,#89068,#89069,#89070,#89071,#89072,#89073,#89074,#89075,#89076,#89077,
#89078,#89079,#89080,#89081,#89082,#89083,#89084,#89085,#89086,#89087,#89088,
#89089,#89090,#89091,#89092,#89093,#89094,#89095,#89096,#89097,#89098,#89099,
#89100,#89101,#89102,#89103,#89104,#89105,#89106,#89107,#89108,#89109,#89110,
#89111,#89112,#89113,#89114,#89115,#89116,#89117,#89118,#89119,#89120,#89121,
#89122,#89123,#89124,#89125,#89126,#89127,#89128,#89129,#89130,#89131,#89132,
#89133,#89134,#89135,#89136,#89137,#89138,#89139,#89140,#89141,#89142,#89143,
#89144,#89145,#89146,#89147,#89148,#89149,#89150,#89151,#89152,#89153,#89154,
#89155,#89156,#89157,#89158,#89159,#89160,#89161,#89162,#89163,#89164,#89165,
#89166,#89167,#89168,#89169,#89170,#89171,#89172,#89173,#89174,#89175,#89176,
#89177,#89178,#89179,#89180,#89181,#89182,#89183,#89184,#89185,#89186,#89187,
#89188,#89189,#89190,#89191,#89192,#89193,#89194,#89195,#89196,#89197,#89198,
#89199,#89200,#89201,#89202,#89203,#89204,#89205,#89206,#89207,#89208,#89209,
#89210,#89211,#89212,#89213,#89214,#89215,#89216,#89217,#89218,#89219,#89220,
#89221,#89222,#89223,#89224,#89225,#89226,#89227,#89228,#89229,#89230,#89231,
#89232,#89233,#89234,#89235,#89236,#89237,#89238,#89239,#89240,#89241,#89242,
#89243,#89244,#89245,#89246,#89247,#89248,#89249,#89250,#89251,#89252,#89253,
#89254,#89255,#89256,#89257,#89258,#89259,#89260,#89261,#89262,#89263,#89264,
#89265,#89266,#89267,#89268,#89269,#89270,#89271,#89272,#89273,#89274,#89275,
#89276,#89277,#89278,#89279,#89280,#89281,#89282,#89283,#89284,#89285,#89286,
#89287,#89288,#89289,#89290,#89291,#89292,#89293,#89294,#89295,#89296,#89297,
#89298,#89299,#89300,#89301,#89302,#89303,#89304,#89305,#89306,#89307,#89308,
#89309,#89310,#89311,#89312,#89313,#89314,#89315,#89316,#89317,#89318,#89319,
#89320,#89321,#89322,#89323,#89324,#89325,#89326,#89327,#89328,#89329,#89330,
#89331,#89332,#89333,#89334,#89335,#89336,#89337,#89338,#89339,#89340,#89341,
#89342,#89343,#89344,#89345,#89346,#89347,#89348,#89349,#89350,#89351,#89352,
#89353,#89354,#89355,#89356,#89357,#89358,#89359,#89360,#89361,#89362,#89363,
#89364,#89365,#89366,#89367,#89368,#89369,#89370,#89371,#89372,#89373,#89374,
#89375,#89376,#89377,#89378,#89379,#89380,#89381,#89382,#89383,#89384,#89385,
#89386,#89387,#89388,#89389,#89390,#89391,#89392,#89393,#89394,#89395,#89396,
#89397,#89398,#89399,#89400,#89401,#89402,#89403,#89404,#89405,#89406,#89407,
#89408,#89409,#89410,#89411,#89412,#89413,#89414,#89415,#89416,#89417,#89418,
#89419,#89420,#89421,#89422,#89423,#89424,#89425,#89426,#89427,#89428,#89429,
#89430,#89431,#89432,#89433,#89434,#89435,#89436,#89437,#89438,#89439,#89440,
#89441,#89442,#89443,#89444,#89445,#89446,#89447,#89448,#89449,#89450,#89451,
#89452,#89453,#89454,#89455,#89456,#89457,#89458,#89459,#89460,#89461,#89462,
#89463,#89464,#89465,#89466,#89467,#89468,#89469,#89470,#89471,#89472,#89473,
#89474,#89475,#89476,#89477,#89478,#89479,#89480,#89481,#89482,#89483,#89484,
#89485,#89486,#89487,#89488,#89489,#89490,#89491,#89492,#89493,#89494,#89495,
#89496,#89497,#89498,#89499,#89500,#89501,#89502,#89503,#89504,#89505,#89506,
#89507,#89508,#89509,#89510,#89511,#89512,#89513,#89514,#89515,#89516,#89517,
#89518,#89519,#89520,#89521,#89522,#89523,#89524,#89525,#89526,#89527,#89528,
#89529,#89530,#89531,#89532,#89533,#89534,#89535,#89536,#89537,#89538,#89539,
#89540,#89541,#89542,#89543,#89544,#89545,#89546,#89547,#89548,#89549,#89550,
#89551,#89552,#89553,#89554,#89555,#89556,#89557,#89558,#89559,#89560,#89561,
#89562,#89563,#89564,#89565,#89566,#89567,#89568,#89569,#89570,#89571,#89572,
#89573,#89574,#89575,#89576,#89577,#89578,#89579,#89580,#89581,#89582,#89583,
#89584,#89585,#89586,#89587,#89588,#89589,#89590,#89591,#89592,#89593,#89594,
#89595,#89596,#89597,#89598,#89599,#89600,#89601,#89602,#89603,#89604,#89605,
#89606,#89607,#89608,#89609,#89610,#89611,#89612,#89613,#89614,#89615,#89616,
#89617,#89618,#89619,#89620,#89621,#89622,#89623,#89624,#89625,#89626,#89627,
#89628,#89629,#89630,#89631,#89632,#89633,#89634,#89635,#89636,#89637,#89638,
#89639,#89640,#89641,#89642,#89643,#89644,#89645,#89646,#89647,#89648,#89649,
#89650,#89651,#89652,#89653,#89654,#89655,#89656,#89657,#89658,#89659,#89660,
#89661,#89662,#89663,#89664,#89665,#89666,#89667,#89668,#89669,#89670,#89671,
#89672,#89673,#89674,#89675,#89676,#89677,#89678,#89679,#89680,#89681,#89682,
#89683,#89684,#89685,#89686,#89687,#89688,#89689,#89690,#89691,#89692,#89693,
#89694,#89695,#89696,#89697,#89698,#89699,#89700,#89701,#89702,#89703,#89704,
#89705,#89706,#89707,#89708,#89709,#89710,#89711,#89712,#89713,#89714,#89715,
#89716,#89717,#89718,#89719,#89720,#89721,#89722,#89723,#89724,#89725,#89726,
#89727,#89728,#89729,#89730,#89731,#89732,#89733,#89734,#89735,#89736,#89737,
#89738,#89739,#89740,#89741,#89742,#89743,#89744,#89745,#89746,#89747,#89748,
#89749,#89750,#89751,#89752,#89753,#89754,#89755,#89756,#89757,#89758,#89759,
#89760,#89761,#89762,#89763,#89764,#89765,#89766,#89767,#89768,#89769,#89770,
#89771,#89772,#89773,#89774,#89775,#89776,#89777,#89778,#89779,#89780,#89781,
#89782,#89783,#89784,#89785,#89786,#89787,#89788,#89789,#89790,#89791,#89792,
#89793,#89794,#89795,#89796,#89797,#89798,#89799,#89800,#89801,#89802,#89803,
#89804,#89805,#89806,#89807,#89808,#89809,#89810,#89811,#89812,#89813,#89814,
#89815,#89816,#89817,#89818,#89819,#89820,#89821,#89822,#89823,#89824,#89825,
#89826,#89827,#89828,#89829,#89830,#89831,#89832,#89833,#89834,#89835,#89836,
#89837,#89838,#89839,#89840,#89841,#89842,#89843,#89844,#89845,#89846,#89847,
#89848,#89849,#89850,#89851,#89852,#89853,#89854,#89855,#89856,#89857,#89858,
#89859,#89860,#89861,#89862,#89863,#89864,#89865,#89866,#89867,#89868,#89869,
#89870,#89871,#89872,#89873,#89874,#89875,#89876,#89877,#89878,#89879,#89880,
#89881,#89882,#89883,#89884,#89885,#89886,#89887,#89888,#89889,#89890,#89891,
#89892,#89893,#89894,#89895,#89896,#89897,#89898,#89899,#89900,#89901,#89902,
#89903,#89904,#89905,#89906,#89907,#89908,#89909,#89910,#89911,#89912,#89913,
#89914,#89915,#89916,#89917,#89918,#89919,#89920,#89921,#89922,#89923,#89924,
#89925,#89926,#89927,#89928,#89929,#89930,#89931,#89932,#89933,#89934,#89935,
#89936,#89937,#89938,#89939,#89940,#89941,#89942,#89943,#89944,#89945,#89946,
#89947,#89948,#89949,#89950,#89951,#89952,#89953,#89954,#89955,#89956,#89957,
#89958,#89959,#89960,#89961,#89962,#89963,#89964,#89965,#89966,#89967,#89968,
#89969,#89970,#89971,#89972,#89973,#89974,#89975,#89976,#89977,#89978,#89979,
#89980,#89981,#89982,#89983,#89984,#89985,#89986,#89987,#89988,#89989,#89990,
#89991,#89992,#89993,#89994,#89995,#89996,#89997,#89998,#89999,#90000,#90001,
#90002,#90003,#90004,#90005,#90006,#90007,#90008,#90009,#90010,#90011,#90012,
#90013,#90014,#90015,#90016,#90017,#90018,#90019,#90020,#90021,#90022,#90023,
#90024,#90025,#90026,#90027,#90028,#90029,#90030,#90031,#90032,#90033,#90034,
#90035,#90036,#90037,#90038,#90039,#90040,#90041,#90042,#90043,#90044,#90045,
#90046,#90047,#90048,#90049,#90050,#90051,#90052,#90053,#90054,#90055,#90056,
#90057,#90058,#90059,#90060,#90061,#90062,#90063,#90064,#90065,#90066,#90067,
#90068,#90069,#90070,#90071,#90072,#90073,#90074,#90075,#90076,#90077,#90078,
#90079,#90080,#90081,#90082,#90083,#90084,#90085,#90086,#90087,#90088,#90089,
#90090,#90091,#90092,#90093,#90094,#90095,#90096,#90097,#90098,#90099,#90100,
#90101,#90102,#90103,#90104,#90105,#90106,#90107,#90108,#90109,#90110,#90111,
#90112,#90113,#90114,#90115,#90116,#90117,#90118,#90119,#90120,#90121,#90122,
#90123,#90124,#90125,#90126,#90127,#90128,#90129,#90130,#90131,#90132,#90133,
#90134,#90135,#90136,#90137,#90138,#90139,#90140,#90141,#90142,#90143,#90144,
#90145,#90146,#90147,#90148,#90149,#90150,#90151,#90152,#90153,#90154,#90155,
#90156,#90157,#90158,#90159,#90160,#90161,#90162,#90163,#90164,#90165,#90166,
#90167,#90168,#90169,#90170,#90171,#90172,#90173,#90174,#90175,#90176,#90177,
#90178,#90179,#90180,#90181,#90182,#90183,#90184,#90185,#90186,#90187,#90188,
#90189,#90190,#90191,#90192,#90193,#90194,#90195,#90196,#90197,#90198,#90199,
#90200,#90201,#90202,#90203,#90204,#90205,#90206,#90207,#90208,#90209,#90210,
#90211,#90212,#90213,#90214,#90215,#90216,#90217,#90218,#90219,#90220,#90221,
#90222,#90223,#90224,#90225,#90226,#90227,#90228,#90229,#90230,#90231,#90232,
#90233,#90234,#90235,#90236,#90237,#90238,#90239,#90240,#90241,#90242,#90243,
#90244,#90245,#90246,#90247,#90248,#90249,#90250,#90251,#90252,#90253,#90254,
#90255,#90256,#90257,#90258,#90259,#90260,#90261,#90262,#90263,#90264,#90265,
#90266,#90267,#90268,#90269,#90270,#90271,#90272,#90273,#90274,#90275,#90276,
#90277,#90278,#90279,#90280,#90281,#90282,#90283,#90284,#90285,#90286,#90287,
#90288,#90289,#90290,#90291,#90292,#90293,#90294,#90295,#90296,#90297,#90298,
#90299,#90300,#90301,#90302,#90303,#90304,#90305,#90306,#90307,#90308,#90309,
#90310,#90311,#90312,#90313,#90314,#90315,#90316,#90317,#90318,#90319,#90320,
#90321,#90322,#90323,#90324,#90325,#90326,#90327,#90328,#90329,#90330,#90331,
#90332,#90333,#90334,#90335,#90336,#90337,#90338,#90339,#90340,#90341,#90342,
#90343,#90344,#90345,#90346,#90347,#90348,#90349,#90350,#90351,#90352,#90353,
#90354,#90355,#90356,#90357,#90358,#90359,#90360,#90361,#90362,#90363,#90364,
#90365,#90366,#90367,#90368,#90369,#90370,#90371,#90372,#90373,#90374,#90375,
#90376,#90377,#90378,#90379,#90380,#90381,#90382,#90383,#90384,#90385,#90386,
#90387,#90388,#90389,#90390,#90391,#90392,#90393,#90394,#90395,#90396,#90397,
#90398,#90399,#90400,#90401,#90402,#90403,#90404,#90405,#90406,#90407,#90408,
#90409,#90410,#90411,#90412,#90413,#90414,#90415,#90416,#90417,#90418,#90419,
#90420,#90421,#90422,#90423,#90424,#90425,#90426,#90427,#90428,#90429,#90430,
#90431,#90432,#90433,#90434,#90435,#90436,#90437,#90438,#90439,#90440,#90441,
#90442,#90443,#90444,#90445,#90446,#90447,#90448,#90449,#90450,#90451,#90452,
#90453,#90454,#90455,#90456,#90457,#90458,#90459,#90460,#90461,#90462,#90463,
#90464,#90465,#90466,#90467,#90468,#90469,#90470,#90471,#90472,#90473,#90474,
#90475,#90476,#90477,#90478,#90479,#90480,#90481,#90482,#90483,#90484,#90485,
#90486,#90487,#90488,#90489,#90490,#90491,#90492,#90493,#90494,#90495,#90496,
#90497,#90498,#90499,#90500,#90501,#90502,#90503,#90504,#90505,#90506,#90507,
#90508,#90509,#90510,#90511,#90512,#90513,#90514,#90515,#90516,#90517,#90518,
#90519,#90520,#90521,#90522,#90523,#90524,#90525,#90526,#90527,#90528,#90529,
#90530,#90531,#90532,#90533,#90534,#90535,#90536,#90537,#90538,#90539,#90540,
#90541,#90542,#90543,#90544,#90545,#90546,#90547,#90548,#90549,#90550,#90551,
#90552,#90553,#90554,#90555,#90556,#90557,#90558,#90559,#90560,#90561,#90562,
#90563,#90564,#90565,#90566,#90567,#90568,#90569,#90570,#90571,#90572,#90573,
#90574,#90575,#90576,#90577,#90578,#90579,#90580,#90581,#90582,#90583,#90584,
#90585,#90586,#90587,#90588,#90589,#90590,#90591,#90592,#90593,#90594,#90595,
#90596,#90597,#90598,#90599,#90600,#90601,#90602,#90603,#90604,#90605,#90606,
#90607,#90608,#90609,#90610,#90611,#90612,#90613,#90614,#90615,#90616,#90617,
#90618,#90619,#90620,#90621,#90622,#90623,#90624,#90625,#90626,#90627,#90628,
#90629,#90630,#90631,#90632,#90633,#90634,#90635,#90636,#90637,#90638,#90639,
#90640,#90641,#90642,#90643,#90644,#90645,#90646,#90647,#90648,#90649,#90650,
#90651,#90652,#90653,#90654,#90655,#90656,#90657,#90658,#90659,#90660,#90661,
#90662,#90663,#90664,#90665,#90666,#90667,#90668,#90669,#90670,#90671,#90672,
#90673,#90674,#90675,#90676,#90677,#90678,#90679,#90680,#90681,#90682,#90683,
#90684,#90685,#90686,#90687,#90688,#90689,#90690,#90691,#90692,#90693,#90694,
#90695,#90696,#90697,#90698,#90699,#90700,#90701,#90702,#90703,#90704,#90705,
#90706,#90707,#90708,#90709,#90710,#90711,#90712,#90713,#90714,#90715,#90716,
#90717,#90718,#90719,#90720,#90721,#90722,#90723,#90724,#90725,#90726,#90727,
#90728,#90729,#90730,#90731,#90732,#90733,#90734,#90735,#90736,#90737,#90738,
#90739,#90740,#90741,#90742,#90743,#90744,#90745,#90746,#90747,#90748,#90749,
#90750,#90751,#90752,#90753,#90754,#90755,#90756,#90757,#90758,#90759,#90760,
#90761,#90762,#90763,#90764,#90765,#90766,#90767,#90768,#90769,#90770,#90771,
#90772,#90773,#90774,#90775,#90776,#90777,#90778,#90779,#90780,#90781,#90782,
#90783,#90784,#90785,#90786,#90787,#90788,#90789,#90790,#90791,#90792,#90793,
#90794,#90795,#90796,#90797,#90798,#90799,#90800,#90801,#90802,#90803,#90804,
#90805,#90806,#90807,#90808,#90809,#90810,#90811,#90812,#90813,#90814,#90815,
#90816,#90817,#90818,#90819,#90820,#90821,#90822,#90823,#90824,#90825,#90826,
#90827,#90828,#90829,#90830,#90831,#90832,#90833,#90834,#90835,#90836,#90837,
#90838,#90839,#90840,#90841,#90842,#90843,#90844,#90845,#90846,#90847,#90848,
#90849,#90850,#90851,#90852,#90853,#90854,#90855,#90856,#90857,#90858,#90859,
#90860,#90861,#90862,#90863,#90864,#90865,#90866,#90867,#90868,#90869,#90870,
#90871,#90872,#90873,#90874,#90875,#90876,#90877,#90878,#90879,#90880,#90881,
#90882,#90883,#90884,#90885,#90886,#90887,#90888,#90889,#90890,#90891,#90892,
#90893,#90894,#90895,#90896,#90897,#90898,#90899,#90900,#90901,#90902,#90903,
#90904,#90905,#90906,#90907,#90908,#90909,#90910,#90911,#90912,#90913,#90914,
#90915,#90916,#90917,#90918,#90919,#90920,#90921,#90922,#90923,#90924,#90925,
#90926,#90927,#90928,#90929,#90930,#90931,#90932,#90933,#90934,#90935,#90936,
#90937,#90938,#90939,#90940,#90941,#90942,#90943,#90944,#90945,#90946,#90947,
#90948,#90949,#90950,#90951,#90952,#90953,#90954,#90955,#90956,#90957,#90958,
#90959,#90960,#90961,#90962,#90963,#90964,#90965,#90966,#90967,#90968,#90969,
#90970,#90971,#90972,#90973,#90974,#90975,#90976,#90977,#90978,#90979,#90980,
#90981,#90982,#90983,#90984,#90985,#90986,#90987,#90988,#90989,#90990,#90991,
#90992,#90993,#90994,#90995,#90996,#90997,#90998,#90999,#91000,#91001,#91002,
#91003,#91004,#91005,#91006,#91007,#91008,#91009,#91010,#91011,#91012,#91013,
#91014,#91015,#91016,#91017,#91018,#91019,#91020,#91021,#91022,#91023,#91024,
#91025,#91026,#91027,#91028,#91029,#91030,#91031,#91032,#91033,#91034,#91035,
#91036,#91037,#91038,#91039,#91040,#91041,#91042,#91043,#91044,#91045,#91046,
#91047,#91048,#91049,#91050,#91051,#91052,#91053,#91054,#91055,#91056,#91057,
#91058,#91059,#91060,#91061,#91062,#91063,#91064,#91065,#91066,#91067,#91068,
#91069,#91070,#91071,#91072,#91073,#91074,#91075,#91076,#91077,#91078,#91079,
#91080,#91081,#91082,#91083,#91084,#91085,#91086,#91087,#91088,#91089,#91090,
#91091,#91092,#91093,#91094,#91095,#91096,#91097,#91098,#91099,#91100,#91101,
#91102,#91103,#91104,#91105,#91106,#91107,#91108,#91109,#91110,#91111,#91112,
#91113,#91114,#91115,#91116,#91117,#91118,#91119,#91120,#91121,#91122,#91123,
#91124,#91125,#91126,#91127,#91128,#91129,#91130,#91131,#91132,#91133,#91134,
#91135,#91136,#91137,#91138,#91139,#91140,#91141,#91142,#91143,#91144,#91145,
#91146,#91147,#91148,#91149,#91150,#91151,#91152,#91153,#91154,#91155,#91156,
#91157,#91158,#91159,#91160,#91161,#91162,#91163,#91164,#91165,#91166,#91167,
#91168,#91169,#91170,#91171,#91172,#91173,#91174,#91175,#91176,#91177,#91178,
#91179,#91180,#91181,#91182,#91183,#91184,#91185,#91186,#91187,#91188,#91189,
#91190,#91191,#91192,#91193,#91194,#91195,#91196,#91197,#91198,#91199,#91200,
#91201,#91202,#91203,#91204,#91205,#91206,#91207,#91208,#91209,#91210,#91211,
#91212,#91213,#91214,#91215,#91216,#91217,#91218,#91219,#91220,#91221,#91222,
#91223,#91224,#91225,#91226,#91227,#91228,#91229,#91230,#91231,#91232,#91233,
#91234,#91235,#91236,#91237,#91238,#91239,#91240,#91241,#91242,#91243,#91244,
#91245,#91246,#91247,#91248,#91249,#91250,#91251,#91252,#91253,#91254,#91255,
#91256,#91257,#91258,#91259,#91260,#91261,#91262,#91263,#91264,#91265,#91266,
#91267,#91268,#91269,#91270,#91271,#91272,#91273,#91274,#91275,#91276,#91277,
#91278,#91279,#91280,#91281,#91282,#91283,#91284,#91285,#91286,#91287,#91288,
#91289,#91290,#91291,#91292,#91293,#91294,#91295,#91296,#91297,#91298,#91299,
#91300,#91301,#91302,#91303,#91304,#91305,#91306,#91307,#91308,#91309,#91310,
#91311,#91312,#91313,#91314,#91315,#91316,#91317,#91318,#91319,#91320,#91321,
#91322,#91323,#91324,#91325,#91326,#91327,#91328,#91329,#91330,#91331,#91332,
#91333,#91334,#91335,#91336,#91337,#91338,#91339,#91340,#91341,#91342,#91343,
#91344,#91345,#91346,#91347,#91348,#91349,#91350,#91351,#91352,#91353,#91354,
#91355,#91356,#91357,#91358,#91359,#91360,#91361,#91362,#91363,#91364,#91365,
#91366,#91367,#91368,#91369,#91370,#91371,#91372,#91373,#91374,#91375,#91376,
#91377,#91378,#91379,#91380,#91381,#91382,#91383,#91384,#91385,#91386,#91387,
#91388,#91389,#91390,#91391,#91392,#91393,#91394,#91395,#91396,#91397,#91398,
#91399,#91400,#91401,#91402,#91403,#91404,#91405,#91406,#91407,#91408,#91409,
#91410,#91411,#91412,#91413,#91414,#91415,#91416,#91417,#91418,#91419,#91420,
#91421,#91422,#91423,#91424,#91425,#91426,#91427,#91428,#91429,#91430,#91431,
#91432,#91433,#91434,#91435,#91436,#91437,#91438,#91439,#91440,#91441,#91442,
#91443,#91444,#91445,#91446,#91447,#91448,#91449,#91450,#91451,#91452,#91453,
#91454,#91455,#91456,#91457,#91458,#91459,#91460,#91461,#91462,#91463,#91464,
#91465,#91466,#91467,#91468,#91469,#91470,#91471,#91472,#91473,#91474,#91475,
#91476,#91477,#91478,#91479,#91480,#91481,#91482,#91483,#91484,#91485,#91486,
#91487,#91488,#91489,#91490,#91491,#91492,#91493,#91494,#91495,#91496,#91497,
#91498,#91499,#91500,#91501,#91502,#91503,#91504,#91505,#91506,#91507,#91508,
#91509,#91510,#91511,#91512,#91513,#91514,#91515,#91516,#91517,#91518,#91519,
#91520,#91521,#91522,#91523,#91524,#91525,#91526,#91527,#91528,#91529,#91530,
#91531,#91532,#91533,#91534,#91535,#91536,#91537,#91538,#91539,#91540,#91541,
#91542,#91543,#91544,#91545,#91546,#91547,#91548,#91549,#91550,#91551,#91552,
#91553,#91554,#91555,#91556,#91557,#91558,#91559,#91560,#91561,#91562,#91563,
#91564,#91565,#91566,#91567,#91568,#91569,#91570,#91571,#91572,#91573,#91574,
#91575,#91576,#91577,#91578,#91579,#91580,#91581,#91582,#91583,#91584,#91585,
#91586,#91587,#91588,#91589,#91590,#91591,#91592,#91593,#91594,#91595,#91596,
#91597,#91598,#91599,#91600,#91601,#91602,#91603,#91604,#91605,#91606,#91607,
#91608,#91609,#91610,#91611,#91612,#91613,#91614,#91615,#91616,#91617,#91618,
#91619,#91620,#91621,#91622,#91623,#91624,#91625,#91626,#91627,#91628,#91629,
#91630,#91631,#91632,#91633,#91634,#91635,#91636,#91637,#91638,#91639,#91640,
#91641,#91642,#91643,#91644,#91645,#91646,#91647,#91648,#91649,#91650,#91651,
#91652,#91653,#91654,#91655,#91656,#91657,#91658,#91659,#91660,#91661,#91662,
#91663,#91664,#91665,#91666,#91667,#91668,#91669,#91670,#91671,#91672,#91673,
#91674,#91675,#91676,#91677,#91678,#91679,#91680,#91681,#91682,#91683,#91684,
#91685,#91686,#91687,#91688,#91689,#91690,#91691,#91692,#91693,#91694,#91695,
#91696,#91697,#91698,#91699,#91700,#91701,#91702,#91703,#91704,#91705,#91706,
#91707,#91708,#91709,#91710,#91711,#91712,#91713,#91714,#91715,#91716,#91717,
#91718,#91719,#91720,#91721,#91722,#91723,#91724,#91725,#91726,#91727,#91728,
#91729,#91730,#91731,#91732,#91733,#91734,#91735,#91736,#91737,#91738,#91739,
#91740,#91741,#91742,#91743,#91744,#91745,#91746,#91747,#91748,#91749,#91750,
#91751,#91752,#91753,#91754,#91755,#91756,#91757,#91758,#91759,#91760,#91761,
#91762,#91763,#91764,#91765,#91766,#91767,#91768,#91769,#91770,#91771,#91772,
#91773,#91774,#91775,#91776,#91777,#91778,#91779,#91780,#91781,#91782,#91783,
#91784,#91785,#91786,#91787,#91788,#91789,#91790,#91791,#91792,#91793,#91794,
#91795,#91796,#91797,#91798,#91799,#91800,#91801,#91802,#91803,#91804,#91805,
#91806,#91807,#91808,#91809,#91810,#91811,#91812,#91813,#91814,#91815,#91816,
#91817,#91818,#91819,#91820,#91821,#91822,#91823,#91824,#91825,#91826,#91827,
#91828,#91829,#91830,#91831,#91832,#91833,#91834,#91835,#91836,#91837,#91838,
#91839,#91840,#91841,#91842,#91843,#91844,#91845,#91846,#91847,#91848,#91849,
#91850,#91851,#91852,#91853,#91854,#91855,#91856,#91857,#91858,#91859,#91860,
#91861,#91862,#91863,#91864,#91865,#91866,#91867,#91868,#91869,#91870,#91871,
#91872,#91873,#91874,#91875,#91876,#91877,#91878,#91879,#91880,#91881,#91882,
#91883,#91884,#91885,#91886,#91887,#91888,#91889,#91890,#91891,#91892,#91893,
#91894,#91895,#91896,#91897,#91898,#91899,#91900,#91901,#91902,#91903,#91904,
#91905,#91906,#91907,#91908,#91909,#91910,#91911,#91912,#91913,#91914,#91915,
#91916,#91917,#91918,#91919,#91920,#91921,#91922,#91923,#91924,#91925,#91926,
#91927,#91928,#91929,#91930,#91931,#91932,#91933,#91934,#91935,#91936,#91937,
#91938,#91939,#91940,#91941,#91942,#91943,#91944,#91945,#91946,#91947,#91948,
#91949,#91950,#91951,#91952,#91953,#91954,#91955,#91956,#91957,#91958,#91959,
#91960,#91961,#91962,#91963,#91964,#91965,#91966,#91967,#91968,#91969,#91970,
#91971,#91972,#91973,#91974,#91975,#91976,#91977,#91978,#91979,#91980,#91981,
#91982,#91983,#91984,#91985,#91986,#91987,#91988,#91989,#91990,#91991,#91992,
#91993,#91994,#91995,#91996,#91997,#91998,#91999,#92000,#92001,#92002,#92003,
#92004,#92005,#92006,#92007,#92008,#92009,#92010,#92011,#92012,#92013,#92014,
#92015,#92016,#92017,#92018,#92019,#92020,#92021,#92022,#92023,#92024,#92025,
#92026,#92027,#92028,#92029,#92030,#92031,#92032,#92033,#92034,#92035,#92036,
#92037,#92038,#92039,#92040,#92041,#92042,#92043,#92044,#92045,#92046,#92047,
#92048,#92049,#92050,#92051,#92052,#92053,#92054,#92055,#92056,#92057,#92058,
#92059,#92060,#92061,#92062,#92063,#92064,#92065,#92066,#92067,#92068,#92069,
#92070,#92071,#92072,#92073,#92074,#92075,#92076,#92077,#92078,#92079,#92080,
#92081,#92082,#92083,#92084,#92085,#92086,#92087,#92088,#92089,#92090,#92091,
#92092,#92093,#92094,#92095,#92096,#92097,#92098,#92099,#92100,#92101,#92102,
#92103,#92104,#92105,#92106,#92107,#92108,#92109,#92110,#92111,#92112,#92113,
#92114,#92115,#92116,#92117,#92118,#92119,#92120,#92121,#92122,#92123,#92124,
#92125,#92126,#92127,#92128,#92129,#92130,#92131,#92132,#92133,#92134,#92135,
#92136,#92137,#92138,#92139,#92140,#92141,#92142,#92143,#92144,#92145,#92146,
#92147,#92148,#92149,#92150,#92151,#92152,#92153,#92154,#92155,#92156,#92157,
#92158,#92159,#92160,#92161),(#92162,#92163,#92164,#92165,#92166,#92167,
#92168,#92169,#92170,#92171,#92172,#92173,#92174,#92175,#92176,#92177,#92178,
#92179,#92180,#92181,#92182,#92183,#92184,#92185,#92186,#92187,#92188,#92189,
#92190,#92191,#92192,#92193,#92194,#92195,#92196,#92197,#92198,#92199,#92200,
#92201,#92202,#92203,#92204,#92205,#92206,#92207,#92208,#92209,#92210,#92211,
#92212,#92213,#92214,#92215,#92216,#92217,#92218,#92219,#92220,#92221,#92222,
#92223,#92224,#92225,#92226,#92227,#92228,#92229,#92230,#92231,#92232,#92233,
#92234,#92235,#92236,#92237,#92238,#92239,#92240,#92241,#92242,#92243,#92244,
#92245,#92246,#92247,#92248,#92249,#92250,#92251,#92252,#92253,#92254,#92255,
#92256,#92257,#92258,#92259,#92260,#92261,#92262,#92263,#92264,#92265,#92266,
#92267,#92268,#92269,#92270,#92271,#92272,#92273,#92274,#92275,#92276,#92277,
#92278,#92279,#92280,#92281,#92282,#92283,#92284,#92285,#92286,#92287,#92288,
#92289,#92290,#92291,#92292,#92293,#92294,#92295,#92296,#92297,#92298,#92299,
#92300,#92301,#92302,#92303,#92304,#92305,#92306,#92307,#92308,#92309,#92310,
#92311,#92312,#92313,#92314,#92315,#92316,#92317,#92318,#92319,#92320,#92321,
#92322,#92323,#92324,#92325,#92326,#92327,#92328,#92329,#92330,#92331,#92332,
#92333,#92334,#92335,#92336,#92337,#92338,#92339,#92340,#92341,#92342,#92343,
#92344,#92345,#92346,#92347,#92348,#92349,#92350,#92351,#92352,#92353,#92354,
#92355,#92356,#92357,#92358,#92359,#92360,#92361,#92362,#92363,#92364,#92365,
#92366,#92367,#92368,#92369,#92370,#92371,#92372,#92373,#92374,#92375,#92376,
#92377,#92378,#92379,#92380,#92381,#92382,#92383,#92384,#92385,#92386,#92387,
#92388,#92389,#92390,#92391,#92392,#92393,#92394,#92395,#92396,#92397,#92398,
#92399,#92400,#92401,#92402,#92403,#92404,#92405,#92406,#92407,#92408,#92409,
#92410,#92411,#92412,#92413,#92414,#92415,#92416,#92417,#92418,#92419,#92420,
#92421,#92422,#92423,#92424,#92425,#92426,#92427,#92428,#92429,#92430,#92431,
#92432,#92433,#92434,#92435,#92436,#92437,#92438,#92439,#92440,#92441,#92442,
#92443,#92444,#92445,#92446,#92447,#92448,#92449,#92450,#92451,#92452,#92453,
#92454,#92455,#92456,#92457,#92458,#92459,#92460,#92461,#92462,#92463,#92464,
#92465,#92466,#92467,#92468,#92469,#92470,#92471,#92472,#92473,#92474,#92475,
#92476,#92477,#92478,#92479,#92480,#92481,#92482,#92483,#92484,#92485,#92486,
#92487,#92488,#92489,#92490,#92491,#92492,#92493,#92494,#92495,#92496,#92497,
#92498,#92499,#92500,#92501,#92502,#92503,#92504,#92505,#92506,#92507,#92508,
#92509,#92510,#92511,#92512,#92513,#92514,#92515,#92516,#92517,#92518,#92519,
#92520,#92521,#92522,#92523,#92524,#92525,#92526,#92527,#92528,#92529,#92530,
#92531,#92532,#92533,#92534,#92535,#92536,#92537,#92538,#92539,#92540,#92541,
#92542,#92543,#92544,#92545,#92546,#92547,#92548,#92549,#92550,#92551,#92552,
#92553,#92554,#92555,#92556,#92557,#92558,#92559,#92560,#92561,#92562,#92563,
#92564,#92565,#92566,#92567,#92568,#92569,#92570,#92571,#92572,#92573,#92574,
#92575,#92576,#92577,#92578,#92579,#92580,#92581,#92582,#92583,#92584,#92585,
#92586,#92587,#92588,#92589,#92590,#92591,#92592,#92593,#92594,#92595,#92596,
#92597,#92598,#92599,#92600,#92601,#92602,#92603,#92604,#92605,#92606,#92607,
#92608,#92609,#92610,#92611,#92612,#92613,#92614,#92615,#92616,#92617,#92618,
#92619,#92620,#92621,#92622,#92623,#92624,#92625,#92626,#92627,#92628,#92629,
#92630,#92631,#92632,#92633,#92634,#92635,#92636,#92637,#92638,#92639,#92640,
#92641,#92642,#92643,#92644,#92645,#92646,#92647,#92648,#92649,#92650,#92651,
#92652,#92653,#92654,#92655,#92656,#92657,#92658,#92659,#92660,#92661,#92662,
#92663,#92664,#92665,#92666,#92667,#92668,#92669,#92670,#92671,#92672,#92673,
#92674,#92675,#92676,#92677,#92678,#92679,#92680,#92681,#92682,#92683,#92684,
#92685,#92686,#92687,#92688,#92689,#92690,#92691,#92692,#92693,#92694,#92695,
#92696,#92697,#92698,#92699,#92700,#92701,#92702,#92703,#92704,#92705,#92706,
#92707,#92708,#92709,#92710,#92711,#92712,#92713,#92714,#92715,#92716,#92717,
#92718,#92719,#92720,#92721,#92722,#92723,#92724,#92725,#92726,#92727,#92728,
#92729,#92730,#92731,#92732,#92733,#92734,#92735,#92736,#92737,#92738,#92739,
#92740,#92741,#92742,#92743,#92744,#92745,#92746,#92747,#92748,#92749,#92750,
#92751,#92752,#92753,#92754,#92755,#92756,#92757,#92758,#92759,#92760,#92761,
#92762,#92763,#92764,#92765,#92766,#92767,#92768,#92769,#92770,#92771,#92772,
#92773,#92774,#92775,#92776,#92777,#92778,#92779,#92780,#92781,#92782,#92783,
#92784,#92785,#92786,#92787,#92788,#92789,#92790,#92791,#92792,#92793,#92794,
#92795,#92796,#92797,#92798,#92799,#92800,#92801,#92802,#92803,#92804,#92805,
#92806,#92807,#92808,#92809,#92810,#92811,#92812,#92813,#92814,#92815,#92816,
#92817,#92818,#92819,#92820,#92821,#92822,#92823,#92824,#92825,#92826,#92827,
#92828,#92829,#92830,#92831,#92832,#92833,#92834,#92835,#92836,#92837,#92838,
#92839,#92840,#92841,#92842,#92843,#92844,#92845,#92846,#92847,#92848,#92849,
#92850,#92851,#92852,#92853,#92854,#92855,#92856,#92857,#92858,#92859,#92860,
#92861,#92862,#92863,#92864,#92865,#92866,#92867,#92868,#92869,#92870,#92871,
#92872,#92873,#92874,#92875,#92876,#92877,#92878,#92879,#92880,#92881,#92882,
#92883,#92884,#92885,#92886,#92887,#92888,#92889,#92890,#92891,#92892,#92893,
#92894,#92895,#92896,#92897,#92898,#92899,#92900,#92901,#92902,#92903,#92904,
#92905,#92906,#92907,#92908,#92909,#92910,#92911,#92912,#92913,#92914,#92915,
#92916,#92917,#92918,#92919,#92920,#92921,#92922,#92923,#92924,#92925,#92926,
#92927,#92928,#92929,#92930,#92931,#92932,#92933,#92934,#92935,#92936,#92937,
#92938,#92939,#92940,#92941,#92942,#92943,#92944,#92945,#92946,#92947,#92948,
#92949,#92950,#92951,#92952,#92953,#92954,#92955,#92956,#92957,#92958,#92959,
#92960,#92961,#92962,#92963,#92964,#92965,#92966,#92967,#92968,#92969,#92970,
#92971,#92972,#92973,#92974,#92975,#92976,#92977,#92978,#92979,#92980,#92981,
#92982,#92983,#92984,#92985,#92986,#92987,#92988,#92989,#92990,#92991,#92992,
#92993,#92994,#92995,#92996,#92997,#92998,#92999,#93000,#93001,#93002,#93003,
#93004,#93005,#93006,#93007,#93008,#93009,#93010,#93011,#93012,#93013,#93014,
#93015,#93016,#93017,#93018,#93019,#93020,#93021,#93022,#93023,#93024,#93025,
#93026,#93027,#93028,#93029,#93030,#93031,#93032,#93033,#93034,#93035,#93036,
#93037,#93038,#93039,#93040,#93041,#93042,#93043,#93044,#93045,#93046,#93047,
#93048,#93049,#93050,#93051,#93052,#93053,#93054,#93055,#93056,#93057,#93058,
#93059,#93060,#93061,#93062,#93063,#93064,#93065,#93066,#93067,#93068,#93069,
#93070,#93071,#93072,#93073,#93074,#93075,#93076,#93077,#93078,#93079,#93080,
#93081,#93082,#93083,#93084,#93085,#93086,#93087,#93088,#93089,#93090,#93091,
#93092,#93093,#93094,#93095,#93096,#93097,#93098,#93099,#93100,#93101,#93102,
#93103,#93104,#93105,#93106,#93107,#93108,#93109,#93110,#93111,#93112,#93113,
#93114,#93115,#93116,#93117,#93118,#93119,#93120,#93121,#93122,#93123,#93124,
#93125,#93126,#93127,#93128,#93129,#93130,#93131,#93132,#93133,#93134,#93135,
#93136,#93137,#93138,#93139,#93140,#93141,#93142,#93143,#93144,#93145,#93146,
#93147,#93148,#93149,#93150,#93151,#93152,#93153,#93154,#93155,#93156,#93157,
#93158,#93159,#93160,#93161,#93162,#93163,#93164,#93165,#93166,#93167,#93168,
#93169,#93170,#93171,#93172,#93173,#93174,#93175,#93176,#93177,#93178,#93179,
#93180,#93181,#93182,#93183,#93184,#93185,#93186,#93187,#93188,#93189,#93190,
#93191,#93192,#93193,#93194,#93195,#93196,#93197,#93198,#93199,#93200,#93201,
#93202,#93203,#93204,#93205,#93206,#93207,#93208,#93209,#93210,#93211,#93212,
#93213,#93214,#93215,#93216,#93217,#93218,#93219,#93220,#93221,#93222,#93223,
#93224,#93225,#93226,#93227,#93228,#93229,#93230,#93231,#93232,#93233,#93234,
#93235,#93236,#93237,#93238,#93239,#93240,#93241,#93242,#93243,#93244,#93245,
#93246,#93247,#93248,#93249,#93250,#93251,#93252,#93253,#93254,#93255,#93256,
#93257,#93258,#93259,#93260,#93261,#93262,#93263,#93264,#93265,#93266,#93267,
#93268,#93269,#93270,#93271,#93272,#93273,#93274,#93275,#93276,#93277,#93278,
#93279,#93280,#93281,#93282,#93283,#93284,#93285,#93286,#93287,#93288,#93289,
#93290,#93291,#93292,#93293,#93294,#93295,#93296,#93297,#93298,#93299,#93300,
#93301,#93302,#93303,#93304,#93305,#93306,#93307,#93308,#93309,#93310,#93311,
#93312,#93313,#93314,#93315,#93316,#93317,#93318,#93319,#93320,#93321,#93322,
#93323,#93324,#93325,#93326,#93327,#93328,#93329,#93330,#93331,#93332,#93333,
#93334,#93335,#93336,#93337,#93338,#93339,#93340,#93341,#93342,#93343,#93344,
#93345,#93346,#93347,#93348,#93349,#93350,#93351,#93352,#93353,#93354,#93355,
#93356,#93357,#93358,#93359,#93360,#93361,#93362,#93363,#93364,#93365,#93366,
#93367,#93368,#93369,#93370,#93371,#93372,#93373,#93374,#93375,#93376,#93377,
#93378,#93379,#93380,#93381,#93382,#93383,#93384,#93385,#93386,#93387,#93388,
#93389,#93390,#93391,#93392,#93393,#93394,#93395,#93396,#93397,#93398,#93399,
#93400,#93401,#93402,#93403,#93404,#93405,#93406,#93407,#93408,#93409,#93410,
#93411,#93412,#93413,#93414,#93415,#93416,#93417,#93418,#93419,#93420,#93421,
#93422,#93423,#93424,#93425,#93426,#93427,#93428,#93429,#93430,#93431,#93432,
#93433,#93434,#93435,#93436,#93437,#93438,#93439,#93440,#93441,#93442,#93443,
#93444,#93445,#93446,#93447,#93448,#93449,#93450,#93451,#93452,#93453,#93454,
#93455,#93456,#93457,#93458,#93459,#93460,#93461,#93462,#93463,#93464,#93465,
#93466,#93467,#93468,#93469,#93470,#93471,#93472,#93473,#93474,#93475,#93476,
#93477,#93478,#93479,#93480,#93481,#93482,#93483,#93484,#93485,#93486,#93487,
#93488,#93489,#93490,#93491,#93492,#93493,#93494,#93495,#93496,#93497,#93498,
#93499,#93500,#93501,#93502,#93503,#93504,#93505,#93506,#93507,#93508,#93509,
#93510,#93511,#93512,#93513,#93514,#93515,#93516,#93517,#93518,#93519,#93520,
#93521,#93522,#93523,#93524,#93525,#93526,#93527,#93528,#93529,#93530,#93531,
#93532,#93533,#93534,#93535,#93536,#93537,#93538,#93539,#93540,#93541,#93542,
#93543,#93544,#93545,#93546,#93547,#93548,#93549,#93550,#93551,#93552,#93553,
#93554,#93555,#93556,#93557,#93558,#93559,#93560,#93561,#93562,#93563,#93564,
#93565,#93566,#93567,#93568,#93569,#93570,#93571,#93572,#93573,#93574,#93575,
#93576,#93577,#93578,#93579,#93580,#93581,#93582,#93583,#93584,#93585,#93586,
#93587,#93588,#93589,#93590,#93591,#93592,#93593,#93594,#93595,#93596,#93597,
#93598,#93599,#93600,#93601,#93602,#93603,#93604,#93605,#93606,#93607,#93608,
#93609,#93610,#93611,#93612,#93613,#93614,#93615,#93616,#93617,#93618,#93619,
#93620,#93621,#93622,#93623,#93624,#93625,#93626,#93627,#93628,#93629,#93630,
#93631,#93632,#93633,#93634,#93635,#93636,#93637,#93638,#93639,#93640,#93641,
#93642,#93643,#93644,#93645,#93646,#93647,#93648,#93649,#93650,#93651,#93652,
#93653,#93654,#93655,#93656,#93657,#93658,#93659,#93660,#93661,#93662,#93663,
#93664,#93665,#93666,#93667,#93668,#93669,#93670,#93671,#93672,#93673,#93674,
#93675,#93676,#93677,#93678,#93679,#93680,#93681,#93682,#93683,#93684,#93685,
#93686,#93687,#93688,#93689,#93690,#93691,#93692,#93693,#93694,#93695,#93696,
#93697,#93698,#93699,#93700,#93701,#93702,#93703,#93704,#93705,#93706,#93707,
#93708,#93709,#93710,#93711,#93712,#93713,#93714,#93715,#93716,#93717,#93718,
#93719,#93720,#93721,#93722,#93723,#93724,#93725,#93726,#93727,#93728,#93729,
#93730,#93731,#93732,#93733,#93734,#93735,#93736,#93737,#93738,#93739,#93740,
#93741,#93742,#93743,#93744,#93745,#93746,#93747,#93748,#93749,#93750,#93751,
#93752,#93753,#93754,#93755,#93756,#93757,#93758,#93759,#93760,#93761,#93762,
#93763,#93764,#93765,#93766,#93767,#93768,#93769,#93770,#93771,#93772,#93773,
#93774,#93775,#93776,#93777,#93778,#93779,#93780,#93781,#93782,#93783,#93784,
#93785,#93786,#93787,#93788,#93789,#93790,#93791,#93792,#93793,#93794,#93795,
#93796,#93797,#93798,#93799,#93800,#93801,#93802,#93803,#93804,#93805,#93806,
#93807,#93808,#93809,#93810,#93811,#93812,#93813,#93814,#93815,#93816,#93817,
#93818,#93819,#93820,#93821,#93822,#93823,#93824,#93825,#93826,#93827,#93828,
#93829,#93830,#93831,#93832,#93833,#93834,#93835,#93836,#93837,#93838,#93839,
#93840,#93841,#93842,#93843,#93844,#93845,#93846,#93847,#93848,#93849,#93850,
#93851,#93852,#93853,#93854,#93855,#93856,#93857,#93858,#93859,#93860,#93861,
#93862,#93863,#93864,#93865,#93866,#93867,#93868,#93869,#93870,#93871,#93872,
#93873,#93874,#93875,#93876,#93877,#93878,#93879,#93880,#93881,#93882,#93883,
#93884,#93885,#93886,#93887,#93888,#93889,#93890,#93891,#93892,#93893,#93894,
#93895,#93896,#93897,#93898,#93899,#93900,#93901,#93902,#93903,#93904,#93905,
#93906,#93907,#93908,#93909,#93910,#93911,#93912,#93913,#93914,#93915,#93916,
#93917,#93918,#93919,#93920,#93921,#93922,#93923,#93924,#93925,#93926,#93927,
#93928,#93929,#93930,#93931,#93932,#93933,#93934,#93935,#93936,#93937,#93938,
#93939,#93940,#93941,#93942,#93943,#93944,#93945,#93946,#93947,#93948,#93949,
#93950,#93951,#93952,#93953,#93954,#93955,#93956,#93957,#93958,#93959,#93960,
#93961,#93962,#93963,#93964,#93965,#93966,#93967,#93968,#93969,#93970,#93971,
#93972,#93973,#93974,#93975,#93976,#93977,#93978,#93979,#93980,#93981,#93982,
#93983,#93984,#93985,#93986,#93987,#93988,#93989,#93990,#93991,#93992,#93993,
#93994,#93995,#93996,#93997,#93998,#93999,#94000,#94001,#94002,#94003,#94004,
#94005,#94006,#94007,#94008,#94009,#94010,#94011,#94012,#94013,#94014,#94015,
#94016,#94017,#94018,#94019,#94020,#94021,#94022,#94023,#94024,#94025,#94026,
#94027,#94028,#94029,#94030,#94031,#94032,#94033,#94034,#94035,#94036,#94037,
#94038,#94039,#94040,#94041,#94042,#94043,#94044,#94045,#94046,#94047,#94048,
#94049,#94050,#94051,#94052,#94053,#94054,#94055,#94056,#94057,#94058,#94059,
#94060,#94061,#94062,#94063,#94064,#94065,#94066,#94067,#94068,#94069,#94070,
#94071,#94072,#94073,#94074,#94075,#94076,#94077,#94078,#94079,#94080,#94081,
#94082,#94083,#94084,#94085,#94086,#94087,#94088,#94089,#94090,#94091,#94092,
#94093,#94094,#94095,#94096,#94097,#94098,#94099,#94100,#94101,#94102,#94103,
#94104,#94105,#94106,#94107,#94108,#94109,#94110,#94111,#94112,#94113,#94114,
#94115,#94116,#94117,#94118,#94119,#94120,#94121,#94122,#94123,#94124,#94125,
#94126,#94127,#94128,#94129,#94130,#94131,#94132,#94133,#94134,#94135,#94136,
#94137,#94138,#94139,#94140,#94141,#94142,#94143,#94144,#94145,#94146,#94147,
#94148,#94149,#94150,#94151,#94152,#94153,#94154,#94155,#94156,#94157,#94158,
#94159,#94160,#94161,#94162,#94163,#94164,#94165,#94166,#94167,#94168,#94169,
#94170,#94171,#94172,#94173,#94174,#94175,#94176,#94177,#94178,#94179,#94180,
#94181,#94182,#94183,#94184,#94185,#94186,#94187,#94188,#94189,#94190,#94191,
#94192,#94193,#94194,#94195,#94196,#94197,#94198,#94199,#94200,#94201,#94202,
#94203,#94204,#94205,#94206,#94207,#94208,#94209,#94210,#94211,#94212,#94213,
#94214,#94215,#94216,#94217,#94218,#94219,#94220,#94221,#94222,#94223,#94224,
#94225,#94226,#94227,#94228,#94229,#94230,#94231,#94232,#94233,#94234,#94235,
#94236,#94237,#94238,#94239,#94240,#94241,#94242,#94243,#94244,#94245,#94246,
#94247,#94248,#94249,#94250,#94251,#94252,#94253,#94254,#94255,#94256,#94257,
#94258,#94259,#94260,#94261,#94262,#94263,#94264,#94265,#94266,#94267,#94268,
#94269,#94270,#94271,#94272,#94273,#94274,#94275,#94276,#94277,#94278,#94279,
#94280,#94281,#94282,#94283,#94284,#94285,#94286,#94287,#94288,#94289,#94290,
#94291,#94292,#94293,#94294,#94295,#94296,#94297,#94298,#94299,#94300,#94301,
#94302,#94303,#94304,#94305,#94306,#94307,#94308,#94309,#94310,#94311,#94312,
#94313,#94314,#94315,#94316,#94317,#94318,#94319,#94320,#94321,#94322,#94323,
#94324,#94325,#94326,#94327,#94328,#94329,#94330,#94331,#94332,#94333,#94334,
#94335,#94336,#94337,#94338,#94339,#94340,#94341,#94342,#94343,#94344,#94345,
#94346,#94347,#94348,#94349,#94350,#94351,#94352,#94353,#94354,#94355,#94356,
#94357,#94358,#94359,#94360,#94361,#94362,#94363,#94364,#94365,#94366,#94367,
#94368,#94369,#94370,#94371,#94372,#94373,#94374,#94375,#94376,#94377,#94378,
#94379,#94380,#94381,#94382,#94383,#94384,#94385,#94386,#94387,#94388,#94389,
#94390,#94391,#94392,#94393,#94394,#94395,#94396,#94397,#94398,#94399,#94400,
#94401,#94402,#94403,#94404,#94405,#94406,#94407,#94408,#94409,#94410,#94411,
#94412,#94413,#94414,#94415,#94416,#94417,#94418,#94419,#94420,#94421,#94422,
#94423,#94424,#94425,#94426,#94427,#94428,#94429,#94430,#94431,#94432,#94433,
#94434,#94435,#94436,#94437,#94438,#94439,#94440,#94441,#94442,#94443,#94444,
#94445,#94446,#94447,#94448,#94449,#94450,#94451,#94452,#94453,#94454,#94455,
#94456,#94457,#94458,#94459,#94460,#94461,#94462,#94463,#94464,#94465,#94466,
#94467,#94468,#94469,#94470,#94471,#94472,#94473,#94474,#94475,#94476,#94477,
#94478,#94479,#94480,#94481,#94482,#94483,#94484,#94485,#94486,#94487,#94488,
#94489,#94490,#94491,#94492,#94493,#94494,#94495,#94496,#94497,#94498,#94499,
#94500,#94501,#94502,#94503,#94504,#94505,#94506,#94507,#94508,#94509,#94510,
#94511,#94512,#94513,#94514,#94515,#94516,#94517,#94518,#94519,#94520,#94521,
#94522,#94523,#94524,#94525,#94526,#94527,#94528,#94529,#94530,#94531,#94532,
#94533,#94534,#94535,#94536,#94537,#94538,#94539,#94540,#94541,#94542,#94543,
#94544,#94545,#94546,#94547,#94548,#94549,#94550,#94551,#94552,#94553,#94554,
#94555,#94556,#94557,#94558,#94559,#94560,#94561,#94562,#94563,#94564,#94565,
#94566,#94567,#94568,#94569,#94570,#94571,#94572,#94573,#94574,#94575,#94576,
#94577,#94578,#94579,#94580,#94581,#94582,#94583,#94584,#94585,#94586,#94587,
#94588,#94589,#94590,#94591,#94592,#94593,#94594,#94595,#94596,#94597,#94598,
#94599,#94600,#94601,#94602,#94603,#94604,#94605,#94606,#94607,#94608,#94609,
#94610,#94611,#94612,#94613,#94614,#94615,#94616,#94617,#94618,#94619,#94620,
#94621,#94622,#94623,#94624,#94625,#94626,#94627,#94628,#94629,#94630,#94631,
#94632,#94633,#94634,#94635,#94636,#94637,#94638,#94639,#94640,#94641,#94642,
#94643,#94644,#94645,#94646,#94647,#94648,#94649,#94650,#94651,#94652,#94653,
#94654,#94655,#94656,#94657,#94658,#94659,#94660,#94661,#94662,#94663,#94664,
#94665,#94666,#94667,#94668,#94669,#94670,#94671,#94672,#94673,#94674,#94675,
#94676,#94677,#94678,#94679,#94680,#94681,#94682,#94683,#94684,#94685,#94686,
#94687,#94688,#94689,#94690,#94691,#94692,#94693,#94694,#94695,#94696,#94697,
#94698,#94699,#94700,#94701,#94702,#94703,#94704,#94705,#94706,#94707,#94708,
#94709,#94710,#94711,#94712,#94713,#94714,#94715,#94716,#94717,#94718,#94719,
#94720,#94721,#94722,#94723,#94724,#94725,#94726,#94727,#94728,#94729,#94730,
#94731,#94732,#94733,#94734,#94735,#94736,#94737,#94738,#94739,#94740,#94741,
#94742,#94743,#94744,#94745,#94746,#94747,#94748,#94749,#94750,#94751,#94752,
#94753,#94754,#94755,#94756,#94757,#94758,#94759,#94760,#94761,#94762,#94763,
#94764,#94765,#94766,#94767,#94768,#94769,#94770,#94771,#94772,#94773,#94774,
#94775,#94776,#94777,#94778,#94779,#94780,#94781,#94782,#94783,#94784,#94785,
#94786,#94787,#94788,#94789,#94790,#94791,#94792,#94793,#94794,#94795,#94796,
#94797,#94798,#94799,#94800,#94801,#94802,#94803,#94804,#94805,#94806,#94807,
#94808,#94809,#94810,#94811,#94812,#94813,#94814,#94815,#94816,#94817,#94818,
#94819,#94820,#94821,#94822,#94823,#94824,#94825,#94826,#94827,#94828,#94829,
#94830,#94831,#94832,#94833,#94834,#94835,#94836,#94837,#94838,#94839,#94840,
#94841,#94842,#94843,#94844,#94845,#94846,#94847,#94848,#94849,#94850,#94851,
#94852,#94853,#94854,#94855,#94856,#94857,#94858,#94859,#94860,#94861,#94862,
#94863,#94864,#94865,#94866,#94867,#94868,#94869,#94870,#94871,#94872,#94873,
#94874,#94875,#94876,#94877,#94878,#94879,#94880,#94881,#94882,#94883,#94884,
#94885,#94886,#94887,#94888,#94889,#94890,#94891,#94892,#94893,#94894,#94895,
#94896,#94897,#94898,#94899,#94900,#94901,#94902,#94903,#94904,#94905,#94906,
#94907,#94908,#94909,#94910,#94911,#94912,#94913,#94914,#94915,#94916,#94917,
#94918,#94919,#94920,#94921,#94922,#94923,#94924,#94925,#94926,#94927,#94928,
#94929,#94930,#94931,#94932,#94933,#94934,#94935,#94936,#94937,#94938,#94939,
#94940,#94941,#94942,#94943,#94944,#94945,#94946,#94947,#94948,#94949,#94950,
#94951,#94952,#94953,#94954,#94955,#94956,#94957,#94958,#94959,#94960,#94961,
#94962,#94963,#94964,#94965,#94966,#94967,#94968,#94969,#94970,#94971,#94972,
#94973,#94974,#94975,#94976,#94977,#94978,#94979,#94980,#94981,#94982,#94983,
#94984,#94985,#94986,#94987,#94988,#94989,#94990,#94991,#94992,#94993,#94994,
#94995,#94996,#94997,#94998,#94999,#95000,#95001,#95002,#95003,#95004,#95005,
#95006,#95007,#95008,#95009,#95010,#95011,#95012,#95013,#95014,#95015,#95016,
#95017,#95018,#95019,#95020,#95021,#95022,#95023,#95024,#95025,#95026,#95027,
#95028,#95029,#95030,#95031,#95032,#95033,#95034,#95035,#95036,#95037,#95038,
#95039,#95040,#95041,#95042,#95043,#95044,#95045,#95046,#95047,#95048,#95049,
#95050,#95051,#95052,#95053,#95054,#95055,#95056,#95057,#95058,#95059,#95060,
#95061,#95062,#95063,#95064,#95065,#95066,#95067,#95068,#95069,#95070,#95071,
#95072,#95073,#95074,#95075,#95076,#95077,#95078,#95079,#95080,#95081,#95082,
#95083,#95084,#95085,#95086,#95087,#95088,#95089,#95090,#95091,#95092,#95093,
#95094,#95095,#95096,#95097,#95098,#95099,#95100,#95101,#95102,#95103,#95104,
#95105,#95106,#95107,#95108,#95109,#95110,#95111,#95112,#95113,#95114,#95115,
#95116,#95117,#95118,#95119,#95120,#95121,#95122,#95123,#95124,#95125,#95126,
#95127,#95128,#95129,#95130,#95131,#95132,#95133,#95134,#95135,#95136,#95137,
#95138,#95139,#95140,#95141,#95142,#95143,#95144,#95145,#95146,#95147,#95148,
#95149,#95150,#95151,#95152,#95153,#95154,#95155,#95156,#95157,#95158,#95159,
#95160,#95161,#95162,#95163,#95164,#95165,#95166,#95167,#95168,#95169,#95170,
#95171,#95172,#95173,#95174,#95175,#95176,#95177,#95178,#95179,#95180,#95181,
#95182,#95183,#95184,#95185,#95186,#95187,#95188,#95189,#95190,#95191,#95192,
#95193,#95194,#95195,#95196,#95197,#95198,#95199,#95200,#95201,#95202,#95203,
#95204,#95205,#95206,#95207,#95208,#95209,#95210,#95211,#95212,#95213,#95214,
#95215,#95216,#95217,#95218,#95219,#95220,#95221,#95222,#95223,#95224,#95225,
#95226,#95227,#95228,#95229,#95230,#95231,#95232,#95233,#95234,#95235,#95236,
#95237,#95238,#95239,#95240,#95241,#95242,#95243,#95244,#95245,#95246,#95247,
#95248,#95249,#95250,#95251,#95252,#95253,#95254,#95255,#95256,#95257,#95258,
#95259,#95260,#95261,#95262,#95263,#95264,#95265,#95266,#95267,#95268,#95269,
#95270,#95271,#95272,#95273,#95274,#95275,#95276,#95277,#95278,#95279,#95280,
#95281,#95282,#95283,#95284,#95285,#95286,#95287,#95288,#95289,#95290,#95291,
#95292,#95293,#95294,#95295,#95296,#95297,#95298,#95299,#95300,#95301,#95302,
#95303,#95304,#95305,#95306,#95307,#95308,#95309,#95310,#95311,#95312,#95313,
#95314,#95315,#95316,#95317,#95318,#95319,#95320,#95321,#95322,#95323,#95324,
#95325,#95326,#95327,#95328,#95329,#95330,#95331,#95332,#95333,#95334,#95335,
#95336,#95337,#95338,#95339,#95340,#95341,#95342,#95343,#95344,#95345,#95346,
#95347,#95348,#95349,#95350,#95351,#95352,#95353,#95354,#95355,#95356,#95357,
#95358,#95359,#95360,#95361,#95362,#95363,#95364,#95365,#95366,#95367,#95368,
#95369,#95370,#95371,#95372,#95373,#95374,#95375,#95376,#95377,#95378,#95379,
#95380,#95381,#95382,#95383,#95384,#95385,#95386,#95387,#95388,#95389,#95390,
#95391,#95392,#95393,#95394,#95395,#95396,#95397,#95398,#95399,#95400,#95401,
#95402,#95403,#95404,#95405,#95406,#95407,#95408,#95409,#95410,#95411,#95412,
#95413,#95414,#95415,#95416,#95417,#95418,#95419,#95420,#95421,#95422,#95423,
#95424,#95425,#95426,#95427,#95428,#95429,#95430,#95431,#95432,#95433,#95434,
#95435,#95436,#95437,#95438,#95439,#95440,#95441,#95442,#95443,#95444,#95445,
#95446,#95447,#95448,#95449,#95450,#95451,#95452,#95453,#95454,#95455,#95456,
#95457,#95458,#95459,#95460,#95461,#95462,#95463,#95464,#95465,#95466,#95467,
#95468,#95469,#95470,#95471,#95472,#95473,#95474,#95475,#95476,#95477,#95478,
#95479,#95480,#95481,#95482,#95483,#95484,#95485,#95486,#95487,#95488,#95489,
#95490,#95491,#95492,#95493,#95494,#95495,#95496,#95497,#95498,#95499,#95500,
#95501,#95502,#95503,#95504,#95505,#95506,#95507,#95508,#95509,#95510,#95511,
#95512,#95513,#95514,#95515,#95516,#95517,#95518,#95519,#95520,#95521,#95522,
#95523,#95524,#95525,#95526,#95527,#95528,#95529,#95530,#95531,#95532,#95533,
#95534,#95535,#95536,#95537,#95538,#95539,#95540,#95541,#95542,#95543,#95544,
#95545,#95546,#95547,#95548,#95549,#95550,#95551,#95552,#95553,#95554,#95555,
#95556,#95557,#95558,#95559,#95560,#95561,#95562,#95563,#95564,#95565,#95566,
#95567,#95568,#95569,#95570,#95571,#95572,#95573,#95574,#95575,#95576,#95577,
#95578,#95579,#95580,#95581,#95582,#95583,#95584,#95585,#95586,#95587,#95588,
#95589,#95590,#95591,#95592,#95593,#95594,#95595,#95596,#95597,#95598,#95599,
#95600,#95601,#95602,#95603,#95604,#95605,#95606,#95607,#95608,#95609,#95610,
#95611,#95612,#95613,#95614,#95615,#95616,#95617,#95618,#95619,#95620,#95621,
#95622,#95623,#95624,#95625,#95626,#95627,#95628,#95629,#95630,#95631,#95632,
#95633,#95634,#95635,#95636,#95637,#95638,#95639,#95640,#95641,#95642,#95643,
#95644,#95645,#95646)),.UNSPECIFIED.,.F.,.F.,.F.,(2,2),(4,1,1,1,1,1,1,1,
1,1,1,1,1,1,1,1,1,1,1,1,1,1,1,1,1,1,1,1,1,1,1,1,1,1,1,1,1,1,1,1,1,1,1,1,
1,1,1,1,1,1,1,1,1,1,1,1,1,1,1,1,1,1,1,1,1,1,1,1,1,1,1,1,1,1,1,1,1,1,1,1,
1,1,1,1,1,1,1,1,1,1,1,1,1,1,1,1,1,1,1,1,1,1,1,1,1,1,1,1,1,1,1,1,1,1,1,1,
1,1,1,1,1,1,1,1,1,1,1,1,1,1,1,1,1,1,1,1,1,1,1,1,1,1,1,1,1,1,1,1,1,1,1,1,
1,1,1,1,1,1,1,1,1,1,1,1,1,1,1,1,1,1,1,1,1,1,1,1,1,1,1,1,1,1,1,1,1,1,1,1,
1,1,1,1,1,1,1,1,1,1,1,1,1,1,1,1,1,1,1,1,1,1,1,1,1,1,1,1,1,1,1,1,1,1,1,1,
1,1,1,1,1,1,1,1,1,1,1,1,1,1,1,1,1,1,1,1,1,1,1,1,1,1,1,1,1,1,1,1,1,1,1,1,
1,1,1,1,1,1,1,1,1,1,1,1,1,1,1,1,1,1,1,1,1,1,1,1,1,1,1,1,1,1,1,1,1,1,1,1,
1,1,1,1,1,1,1,1,1,1,1,1,1,1,1,1,1,1,1,1,1,1,1,1,1,1,1,1,1,1,1,1,1,1,1,1,
1,1,1,1,1,1,1,1,1,1,1,1,1,1,1,1,1,1,1,1,1,1,1,1,1,1,1,1,1,1,1,1,1,1,1,1,
1,1,1,1,1,1,1,1,1,1,1,1,1,1,1,1,1,1,1,1,1,1,1,1,1,1,1,1,1,1,1,1,1,1,1,1,
1,1,1,1,1,1,1,1,1,1,1,1,1,1,1,1,1,1,1,1,1,1,1,1,1,1,1,1,1,1,1,1,1,1,1,1,
1,1,1,1,1,1,1,1,1,1,1,1,1,1,1,1,1,1,1,1,1,1,1,1,1,1,1,1,1,1,1,1,1,1,1,1,
1,1,1,1,1,1,1,1,1,1,1,1,1,1,1,1,1,1,1,1,1,1,1,1,1,1,1,1,1,1,1,1,1,1,1,1,
1,1,1,1,1,1,1,1,1,1,1,1,1,1,1,1,1,1,1,1,1,1,1,1,1,1,1,1,1,1,1,1,1,1,1,1,
1,1,1,1,1,1,1,1,1,1,1,1,1,1,1,1,1,1,1,1,1,1,1,1,1,1,1,1,1,1,1,1,1,1,1,1,
1,1,1,1,1,1,1,1,1,1,1,1,1,1,1,1,1,1,1,1,1,1,1,1,1,1,1,1,1,1,1,1,1,1,1,1,
1,1,1,1,1,1,1,1,1,1,1,1,1,1,1,1,1,1,1,1,1,1,1,1,1,1,1,1,1,1,1,1,1,1,1,1,
1,1,1,1,1,1,1,1,1,1,1,1,1,1,1,1,1,1,1,1,1,1,1,1,1,1,1,1,1,1,1,1,1,1,1,1,
1,1,1,1,1,1,1,1,1,1,1,1,1,1,1,1,1,1,1,1,1,1,1,1,1,1,1,1,1,1,1,1,1,1,1,1,
1,1,1,1,1,1,1,1,1,1,1,1,1,1,1,1,1,1,1,1,1,1,1,1,1,1,1,1,1,1,1,1,1,1,1,1,
1,1,1,1,1,1,1,1,1,1,1,1,1,1,1,1,1,1,1,1,1,1,1,1,1,1,1,1,1,1,1,1,1,1,1,1,
1,1,1,1,1,1,1,1,1,1,1,1,1,1,1,1,1,1,1,1,1,1,1,1,1,1,1,1,1,1,1,1,1,1,1,1,
1,1,1,1,1,1,1,1,1,1,1,1,1,1,1,1,1,1,1,1,1,1,1,1,1,1,1,1,1,1,1,1,1,1,1,1,
1,1,1,1,1,1,1,1,1,1,1,1,1,1,1,1,1,1,1,1,1,1,1,1,1,1,1,1,1,1,1,1,1,1,1,1,
1,1,1,1,1,1,1,1,1,1,1,1,1,1,1,1,1,1,1,1,1,1,1,1,1,1,1,1,1,1,1,1,1,1,1,1,
1,1,1,1,1,1,1,1,1,1,1,1,1,1,1,1,1,1,1,1,1,1,1,1,1,1,1,1,1,1,1,1,1,1,1,1,
1,1,1,1,1,1,1,1,1,1,1,1,1,1,1,1,1,1,1,1,1,1,1,1,1,1,1,1,1,1,1,1,1,1,1,1,
1,1,1,1,1,1,1,1,1,1,1,1,1,1,1,1,1,1,1,1,1,1,1,1,1,1,1,1,1,1,1,1,1,1,1,1,
1,1,1,1,1,1,1,1,1,1,1,1,1,1,1,1,1,1,1,1,1,1,1,1,1,1,1,1,1,1,1,1,1,1,1,1,
1,1,1,1,1,1,1,1,1,1,1,1,1,1,1,1,1,1,1,1,1,1,1,1,1,1,1,1,1,1,1,1,1,1,1,1,
1,1,1,1,1,1,1,1,1,1,1,1,1,1,1,1,1,1,1,1,1,1,1,1,1,1,1,1,1,1,1,1,1,1,1,1,
1,1,1,1,1,1,1,1,1,1,1,1,1,1,1,1,1,1,1,1,1,1,1,1,1,1,1,1,1,1,1,1,1,1,1,1,
1,1,1,1,1,1,1,1,1,1,1,1,1,1,1,1,1,1,1,1,1,1,1,1,1,1,1,1,1,1,1,1,1,1,1,1,
1,1,1,1,1,1,1,1,1,1,1,1,1,1,1,1,1,1,1,1,1,1,1,1,1,1,1,1,1,1,1,1,1,1,1,1,
1,1,1,1,1,1,1,1,1,1,1,1,1,1,1,1,1,1,1,1,1,1,1,1,1,1,1,1,1,1,1,1,1,1,1,1,
1,1,1,1,1,1,1,1,1,1,1,1,1,1,1,1,1,1,1,1,1,1,1,1,1,1,1,1,1,1,1,1,1,1,1,1,
1,1,1,1,1,1,1,1,1,1,1,1,1,1,1,1,1,1,1,1,1,1,1,1,1,1,1,1,1,1,1,1,1,1,1,1,
1,1,1,1,1,1,1,1,1,1,1,1,1,1,1,1,1,1,1,1,1,1,1,1,1,1,1,1,1,1,1,1,1,1,1,1,
1,1,1,1,1,1,1,1,1,1,1,1,1,1,1,1,1,1,1,1,1,1,1,1,1,1,1,1,1,1,1,1,1,1,1,1,
1,1,1,1,1,1,1,1,1,1,1,1,1,1,1,1,1,1,1,1,1,1,1,1,1,1,1,1,1,1,1,1,1,1,1,1,
1,1,1,1,1,1,1,1,1,1,1,1,1,1,1,1,1,1,1,1,1,1,1,1,1,1,1,1,1,1,1,1,1,1,1,1,
1,1,1,1,1,1,1,1,1,1,1,1,1,1,1,1,1,1,1,1,1,1,1,1,1,1,1,1,1,1,1,1,1,1,1,1,
1,1,1,1,1,1,1,1,1,1,1,1,1,1,1,1,1,1,1,1,1,1,1,1,1,1,1,1,1,1,1,1,1,1,1,1,
1,1,1,1,1,1,1,1,1,1,1,1,1,1,1,1,1,1,1,1,1,1,1,1,1,1,1,1,1,1,1,1,1,1,1,1,
1,1,1,1,1,1,1,1,1,1,1,1,1,1,1,1,1,1,1,1,1,1,1,1,1,1,1,1,1,1,1,1,1,1,1,1,
1,1,1,1,1,1,1,1,1,1,1,1,1,1,1,1,1,1,1,1,1,1,1,1,1,1,1,1,1,1,1,1,1,1,1,1,
1,1,1,1,1,1,1,1,1,1,1,1,1,1,1,1,1,1,1,1,1,1,1,1,1,1,1,1,1,1,1,1,1,1,1,1,
1,1,1,1,1,1,1,1,1,1,1,1,1,1,1,1,1,1,1,1,1,1,1,1,1,1,1,1,1,1,1,1,1,1,1,1,
1,1,1,1,1,1,1,1,1,1,1,1,1,1,1,1,1,1,1,1,1,1,1,1,1,1,1,1,1,1,1,1,1,1,1,1,
1,1,1,1,1,1,1,1,1,1,1,1,1,1,1,1,1,1,1,1,1,1,1,1,1,1,1,1,1,1,1,1,1,1,1,1,
1,1,1,1,1,1,1,1,1,1,1,1,1,1,1,1,1,1,1,1,1,1,1,1,1,1,1,1,1,1,1,1,1,1,1,1,
1,1,1,1,1,1,1,1,1,1,1,1,1,1,1,1,1,1,1,1,1,1,1,1,1,1,1,1,1,1,1,1,1,1,1,1,
1,1,1,1,1,1,1,1,1,1,1,1,1,1,1,1,1,1,1,1,1,1,1,1,1,1,1,1,1,1,1,1,1,1,1,1,
1,1,1,1,1,1,1,1,1,1,1,1,1,1,1,1,1,1,1,1,1,1,1,1,1,1,1,1,1,1,1,1,1,1,1,1,
1,1,1,1,1,1,1,1,1,1,1,1,1,1,1,1,1,1,1,1,1,1,1,1,1,1,1,1,1,1,1,1,1,1,1,1,
1,1,1,1,1,1,1,1,1,1,1,1,1,1,1,1,1,1,1,1,1,1,1,1,1,1,1,1,1,1,1,1,1,1,1,1,
1,1,1,1,1,1,1,1,1,1,1,1,1,1,1,1,1,1,1,1,1,1,1,1,1,1,1,1,1,1,1,1,1,1,1,1,
1,1,1,1,1,1,1,1,1,1,1,1,1,1,1,1,1,1,1,1,1,1,1,1,1,1,1,1,1,1,1,1,1,1,1,1,
1,1,1,1,1,1,1,1,1,1,1,1,1,1,1,1,1,1,1,1,1,1,1,1,1,1,1,1,1,1,1,1,1,1,1,1,
1,1,1,1,1,1,1,1,1,1,1,1,1,1,1,1,1,1,1,1,1,1,1,1,1,1,1,1,1,1,1,1,1,1,1,1,
1,1,1,1,1,1,1,1,1,1,1,1,1,1,1,1,1,1,1,1,1,1,1,1,1,1,1,1,1,1,1,1,1,1,1,1,
1,1,1,1,1,1,1,1,1,1,1,1,1,1,1,1,1,1,1,1,1,1,1,1,1,1,1,1,1,1,1,1,1,1,1,1,
1,1,1,1,1,1,1,1,1,1,1,1,1,1,1,1,1,1,1,1,1,1,1,1,1,1,1,1,1,1,1,1,1,1,1,1,
1,1,1,1,1,1,1,1,1,1,1,1,1,1,1,1,1,1,1,1,1,1,1,1,1,1,1,1,1,1,1,1,1,1,1,1,
1,1,1,1,1,1,1,1,1,1,1,1,1,1,1,1,1,1,1,1,1,1,1,1,1,1,1,1,1,1,1,1,1,1,1,1,
1,1,1,1,1,1,1,1,1,1,1,1,1,1,1,1,1,1,1,1,1,1,1,1,1,1,1,1,1,1,1,1,1,1,1,1,
1,1,1,1,1,1,1,1,1,1,1,1,1,1,1,1,1,1,1,1,1,1,1,1,1,1,1,1,1,1,1,1,1,1,1,1,
1,1,1,1,1,1,1,1,1,1,1,1,1,1,1,1,1,1,1,1,1,1,1,1,1,1,1,1,1,1,1,1,1,1,1,1,
1,1,1,1,1,1,1,1,1,1,1,1,1,1,1,1,1,1,1,1,1,1,1,1,1,1,1,1,1,1,1,1,1,1,1,1,
1,1,1,1,1,1,1,1,1,1,1,1,1,1,1,1,1,1,1,1,1,1,1,1,1,1,1,1,1,1,1,1,1,1,1,1,
1,1,1,1,1,1,1,1,1,1,1,1,1,1,1,1,1,1,1,1,1,1,1,1,1,1,1,1,1,1,1,1,1,1,1,1,
1,1,1,1,1,1,1,1,1,1,1,1,1,1,1,1,1,1,1,1,1,1,1,1,1,1,1,1,1,1,1,1,1,1,1,1,
1,1,1,1,1,1,1,1,1,1,1,1,1,1,1,1,1,1,1,1,1,1,1,1,1,1,1,1,1,1,1,1,1,1,1,1,
1,1,1,1,1,1,1,1,1,1,1,1,1,1,1,1,1,1,1,1,1,1,1,1,1,1,1,1,1,1,1,1,1,1,1,1,
1,1,1,1,1,1,1,1,1,1,1,1,1,1,1,1,1,1,1,1,1,1,1,1,1,1,1,1,1,1,1,1,1,1,1,1,
1,1,1,1,1,1,1,1,1,1,1,1,1,1,1,1,1,1,1,1,1,1,1,1,1,1,1,1,1,1,1,1,1,1,1,1,
1,1,1,1,1,1,1,1,1,1,1,1,1,1,1,1,1,1,1,1,1,1,1,1,1,1,1,1,1,1,1,1,1,1,1,1,
1,1,1,1,1,1,1,1,1,1,1,1,1,1,1,1,1,1,1,1,1,1,1,1,1,1,1,1,1,1,1,1,1,1,1,1,
1,1,1,1,1,1,1,1,1,1,1,1,1,1,1,1,1,1,1,1,1,1,1,1,1,1,1,1,1,1,1,1,1,1,1,1,
1,1,1,1,1,1,1,1,1,1,1,1,1,1,1,1,1,1,1,1,1,1,1,1,1,1,1,1,1,1,1,1,1,1,1,1,
1,1,1,1,1,1,1,1,1,1,1,1,1,1,1,1,1,1,1,1,1,1,1,1,1,1,1,1,1,1,1,1,1,1,1,1,
1,1,1,1,1,1,1,1,1,1,1,1,1,1,1,1,1,1,1,1,1,1,1,1,1,1,1,1,1,1,1,1,1,1,1,1,
1,1,1,1,1,1,1,1,1,1,1,1,1,1,1,1,1,1,1,1,1,1,1,1,1,1,1,1,1,1,1,1,1,1,1,1,
1,1,1,1,1,1,1,1,1,1,1,1,1,1,1,1,1,1,1,1,1,1,1,1,1,1,1,1,1,1,1,1,1,1,1,1,
1,1,1,1,1,1,1,1,1,1,1,1,1,1,1,1,1,1,1,1,1,1,1,1,1,1,1,1,1,1,1,1,1,1,1,1,
1,1,1,1,1,1,1,1,1,1,1,1,1,1,1,1,1,1,1,1,1,1,1,1,1,1,1,1,1,1,1,1,1,1,1,1,
1,1,1,1,1,1,1,1,1,1,1,1,1,1,1,1,1,1,1,1,1,1,1,1,1,1,1,1,1,1,1,1,1,1,1,1,
1,1,1,1,1,1,1,1,1,1,1,1,1,1,1,1,1,1,1,1,1,1,1,1,1,1,1,1,1,1,1,1,1,1,1,1,
1,1,1,1,1,1,1,1,1,1,1,1,1,1,1,1,1,1,1,1,1,1,1,1,1,1,1,1,1,1,1,1,1,1,1,1,
1,1,1,1,1,1,1,1,1,1,1,1,1,1,1,1,1,1,1,1,1,1,1,1,1,1,1,1,1,1,1,1,1,1,1,1,
1,1,1,1,1,1,1,1,1,1,1,1,1,1,1,1,1,1,1,1,1,1,1,1,1,1,1,1,1,1,1,1,1,1,1,1,
1,1,1,1,1,1,1,1,1,1,1,1,1,1,1,1,1,1,1,1,1,1,1,1,1,1,1,1,1,1,1,1,1,1,1,1,
1,1,1,1,1,1,1,1,1,1,1,1,1,1,1,1,1,1,1,1,1,1,1,1,1,1,1,1,1,1,1,1,1,1,1,1,
1,1,1,1,1,1,1,1,1,1,1,1,1,1,1,1,1,1,1,1,1,1,1,1,1,1,1,1,1,1,1,1,1,1,1,1,
1,1,1,1,1,1,1,1,1,1,1,1,1,1,1,1,1,1,1,1,1,1,1,1,1,1,1,1,1,1,1,1,1,1,1,1,
1,1,1,1,1,1,1,1,1,1,1,1,1,1,1,1,1,1,4),(-1.76619037896906,-1.18309518948453),
(0.,0.869746702321014,1.7394931589914,2.60923976624962,3.47983908319159,
4.35043840179749,5.22018503077054,6.08993165951504,6.95967828799171,7.82942491616733,
8.69917154401062,9.56891817149224,10.4395174886835,11.3101168056706,12.179863432132,
13.049610058144,13.9193566836854,14.7891033087372,15.6588499332817,16.5285965573034,
17.3991958717975,18.2697951860185,18.7046684974166,19.1395418086746,19.5744151197912,
20.0092884307654,20.4441617415962,20.8790350522825,21.7487816732187,22.1836549834672,
22.6185282935685,23.0534016035221,23.4882749133276,23.9231482229848,24.3588742245859,
24.794600226187,25.2294735355468,26.0992201538203,26.5340934627341,26.9689667714994,
27.4038400801166,27.838713388586,28.2735866969081,28.7084600050832,29.143333313112,
29.5782066209952,30.0130799287334,30.4479532363275,30.8828265437783,31.3185525442794,
31.7542785447804,32.1891518519474,32.6240251589741,33.0588984658616,33.4937717726112,
33.928645079224,34.3635183857014,34.7983916920448,35.2332649982556,35.6681383043353,
36.1030116102854,36.5378849161076,36.9727582218035,37.4076315273749,37.8425048328235,
38.2782308323341,38.7139568318446,39.1488301370532,39.5837034421446,40.0185767471208,
40.4534500519838,40.8883233567357,41.3231966613787,41.7580699659148,42.1929432703463,
42.6278165746754,43.0626898789044,43.4975631830356,43.9324364870714,44.3673097910142,
44.8021830948664,45.2379090935952,45.673635092324,46.1085083960024,46.5433816995978,
46.9782550031127,47.4131283065497,47.8480016099115,48.2828749132006,48.7177482164198,
49.1526215195718,49.5874948226593,50.0223681256851,50.457241428652,50.8921147315628,
51.3269880344203,51.7618613372274,52.197587335454,52.6333133336805,53.0681866363954,
53.5030599390685,53.9379332417027,54.3728065443011,54.8076798468664,55.2425531494018,
55.6774264519101,56.1122997543943,56.5471730568575,56.9820463593026,57.4169196617326,
57.8517929641506,58.2866662665595,58.7215395689624,59.157265567009,59.5929915650557,
60.0278648674556,60.4627381698584,60.8976114722673,61.3324847746853,61.7673580771153,
62.2022313795604,62.6371046820236,63.0719779845079,63.5068512870162,63.9417245895516,
64.376597892117,64.8114711947155,65.2463444973499,65.6812178000231,66.1169437982275,
66.5526697964318,66.9875430991915,67.4224164019987,67.8572897048563,68.2921630077673,
68.7270363107343,69.1619096137603,69.5967829168479,70.0316562200001,70.4665295232194,
70.9014028265087,71.3362761298705,71.7711494333077,72.2060227368227,72.6408960404182,
73.0766220391044,73.5123480377905,73.9472213415547,74.382094645407,74.8169679493499,
75.2518412533859,75.6867145575172,76.1215878617464,76.5564611660756,76.9913344705072,
77.4262077750435,77.8610810796866,78.2959543844386,78.7308276893018,79.1657009942781,
79.6005742993696,80.0363002988208,80.4720262982719,80.9068996035997,81.3417729090484,
81.7766462146199,82.211519520316,82.6463928261383,83.0812661320886,83.5161394381684,
83.9510127443794,84.3858860507229,84.8207593572004,85.2556326638134,85.6905059705631,
86.1253792774507,86.5602525844776,86.995978584908,87.4317045853384,87.8665778926469,
88.3014512000977,88.7363245076919,89.1711978154302,89.6060711233134,90.0409444313423,
90.4758177395175,90.9106910478396,91.345564356309,91.7804376649263,92.2153109736917,
92.6501842826055,93.085057591668,93.5199309008791,93.9556569024059,94.3913829039327,
94.8262562134414,95.2611295230986,95.6960028329042,96.1308761428578,96.5657494529591,
97.0006227632077,97.4354960736028,97.870369384144,98.3052426948304,98.7401160056612,
99.1749893166354,99.6098626277522,100.04473593901,100.915335253024,101.351061255639,
101.785934567313,102.220807879124,102.655681191068,103.090554503145,103.525427815353,
104.395174440154,105.264921065453,105.699794378283,106.134667691232,106.569541004295,
107.004414317471,107.8750136343,108.745612951339,109.615359578629,110.485106206296,
111.354852834309,112.224599462639,113.094346091254,113.964092720119,114.834692038763,
115.705291357499,116.575037986826,117.444784616267,118.314531245777,119.184277875311,
120.054024504821,120.923771134261,121.794370453112,122.66496977189,123.534716400968,
124.404463029834,125.274209658448,126.143956286779,127.013702914792,127.883449542458,
128.754048859798,129.624648176939,130.494394803617,131.364141429857,132.233888055637,
133.103634680937,133.973381305737,134.843127930023,135.71372724472,136.584326559147,
137.019199870684,137.454073182083,137.888946493341,138.323819804458,139.193566426263,
140.063313047491,140.498186357887,140.933059668136,141.367932978237,141.802806288191,
142.237679597997,142.673405599673,143.109131601348,143.544004910857,143.978878220217,
144.413751529429,144.848624838491,145.283498147405,145.718371456171,146.153244764789,
146.588118073258,147.022991381581,147.457864689756,147.892737997785,148.327611305669,
148.762484613407,149.197357921002,149.633083921574,150.068809922147,150.503683229455,
150.938556536623,151.37342984365,151.808303150538,152.243176457288,152.678049763901,
153.112923070379,153.547796376722,153.982669682934,154.417542989014,154.852416294964,
155.287289600787,155.722162906483,156.157036212055,156.592762211626,157.028488211198,
157.463361516526,157.898234821735,158.333108126826,158.767981431803,159.202854736666,
159.637728041419,160.072601346062,160.507474650599,160.94234795503,161.37722125936,
161.812094563589,162.246967867721,162.681841171757,163.1167144757,163.552440474473,
163.988166473247,164.423039777011,164.85791308069,165.292786384286,165.727659687801,
166.162532991238,166.597406294601,167.03227959789,167.46715290111,167.902026204262,
168.33689950735,168.771772810376,169.206646113343,169.641519416254,170.076392719112,
170.512118717363,170.947844715614,171.382718018374,171.817591321089,172.252464623762,
172.687337926397,173.122211228996,173.557084531561,173.991957834097,174.426831136606,
174.86170443909,175.296577741554,175.731451044,176.16632434643,176.601197648848,
177.036070951258,177.471796949306,177.907522947355,178.342396249755,178.777269552155,
179.212142854558,179.647016156968,180.081889459386,180.516762761816,180.951636064262,
181.386509366726,181.82138266921,182.256255971719,182.691129274255,183.12600257682,
183.560875879419,183.995749182054,184.431475180237,184.867201178421,185.302074481136,
185.736947783896,186.171821086704,186.606694389561,187.041567692473,187.47644099544,
187.911314298466,188.346187601554,188.781060904706,189.215934207926,189.650807511215,
190.085680814577,190.520554118015,190.95542742153,191.391153420175,191.82687941882,
192.261752722499,192.696626026263,193.131499330116,193.566372634059,194.001245938095,
194.436119242227,194.870992546456,195.305865850785,195.740739155217,196.175612459754,
196.610485764397,197.045359069149,197.480232374013,197.915105678989,198.350831678382,
198.786557677775,199.221430982984,199.656304288312,200.091177593761,200.526050899333,
200.960924205029,201.395797510852,201.830670816802,202.265544122882,202.700417429093,
203.135290735437,203.570164041915,204.005037348528,204.439910655278,204.874783962166,
205.310509962526,205.746235962887,206.181109270054,206.615982577363,207.050855884814,
207.485729192409,207.920602500147,208.355475808031,208.79034911606,209.225222424235,
209.660095732558,210.094969041027,210.529842349645,210.96471565841,211.399588967324,
211.834462276387,212.27018827784,212.705914279292,213.140787588653,213.575660898161,
214.010534207819,214.880280827579,215.31515413768,215.750027447929,216.184900758324,
216.619774068866,217.054647379553,217.489520690384,218.359267312475,219.22986662628,
219.665592628826,220.100465940363,220.535339252038,220.970212563848,221.83995918787,
222.709705812416,223.579452437468,224.014325750179,224.44919906301,225.318945689022,
226.189545005688,227.060144322571,227.929890949664,228.799637577146,229.66938420499,
230.539130833166,231.408877461643,232.278624090388,233.149223408954,234.019822727623,
234.889569356878,235.759315986267,236.629062615749,237.498809245277,238.368555874806,
239.238302504287,240.108901823183,240.979501142017,241.849247771189,242.718994400167,
243.588741028911,244.458487657389,245.328234285565,246.197980913409,247.068580230891,
247.939179548182,248.80892617507,249.678672801532,250.548419427545,251.418166053087,
252.287912678139,253.157659302684,254.028258617581,254.898857932211,255.333731243885,
255.768604555423,256.203477866821,256.63835117808,257.508097800171,258.377844421689,
258.812717732231,259.247591042627,259.682464352876,260.117337662977,260.552210972931,
260.987936974682,261.858536286089,262.293409595598,262.728282904958,263.16315621417,
263.598029523233,264.032902832147,264.467776140913,264.902649449531,265.337522758001,
265.772396066323,266.207269374499,266.642142682528,267.077015990412,267.511889298151,
267.947615298795,268.383341299439,268.81821460689,269.2530879142,269.687961221367,
270.122834528394,270.557707835282,270.992581142032,271.427454448646,271.862327755124,
272.297201061468,272.732074367679,273.166947673759,273.60182097971,274.036694285533,
274.471567591229,274.907293590862,275.343019590495,275.777892895944,276.212766201272,
276.647639506481,277.082512811573,277.51738611655,277.952259421414,278.387132726166,
278.82200603081,279.256879335346,279.691752639779,280.126625944108,280.561499248338,
280.996372552469,281.431245856506,281.866971855324,282.302697854143,282.737571157996,
283.172444461761,283.60731776544,284.042191069036,284.477064372551,284.911937675989,
285.346810979351,285.781684282641,286.216557585861,286.651430889013,287.086304192101,
287.521177495128,287.956050798095,288.390924101007,288.826650099283,289.262376097559,
289.697249400366,290.132122703127,290.566996005842,291.001869308516,291.43674261115,
291.871615913749,292.306489216315,292.741362518851,293.17623582136,293.611109123845,
294.045982426308,294.480855728754,294.915729031185,295.350602333603,295.786328331655,
296.222054329707,296.65692763211,297.091800934511,297.526674236911,297.961547539314,
298.396420841724,298.831294144142,299.266167446573,299.701040749018,300.135914051482,
300.570787353967,301.005660656476,301.440533959012,301.875407261578,302.310280564177,
302.746006562341,303.181732560506,303.616605863179,304.051479165895,304.486352468655,
304.921225771462,305.35609907432,305.790972377232,306.225845680199,306.660718983226,
307.095592286314,307.530465589466,307.965338892686,308.400212195976,308.835085499338,
309.269958802776,309.705684801381,310.141410799985,310.576284103581,311.01115740726,
311.446030711025,311.880904014878,312.315777318821,312.750650622858,313.185523926989,
313.620397231219,314.055270535549,314.490143839981,314.925017144517,315.359890449161,
315.794763753913,316.229637058777,316.665363058112,317.101089057448,317.53596236254,
317.970835667749,318.405708973077,318.840582278526,319.275455584098,319.710328889795,
320.145202195618,320.580075501568,321.014948807648,321.44982211386,321.884695420204,
322.319568726682,322.754442033295,323.189315340045,323.625041340336,324.060767340628,
324.495640647655,324.930513954822,325.365387262131,325.800260569583,326.235133877177,
326.670007184916,327.1048804928,327.539753800829,327.974627109005,328.409500417327,
328.844373725797,329.279247034415,329.714120343181,330.148993652095,330.584719653474,
331.020445654852,331.455318964064,331.890192273424,332.325065582933,332.759938892591,
333.194812202397,333.629685512351,334.064558822453,334.499432132702,334.934305443098,
335.369178753639,335.804052064326,336.673798686132,337.108671997249,337.544397999725,
337.980124002201,338.4149973136,338.849870625137,339.284743936812,340.154490560568,
341.024237184854,341.459110497191,341.893983809655,342.328857122244,342.763730434955,
343.633477060735,344.504076377234,345.374675693955,346.244422320844,347.114168948136,
347.983915575803,348.853662203817,349.723408832148,350.593155460764,351.463754779246,
352.334354097839,353.204100727012,354.07384735634,354.943593985781,355.813340615292,
356.683087244827,357.552833874338,358.423433193272,359.294032512154,360.163779141409,
361.033525770489,361.903272399355,362.77301902797,363.642765656301,364.512512284316,
365.383111601936,366.253710919371,367.123457546465,367.993204173143,368.862950799383,
369.732697425164,370.602444050463,371.472190675265,372.342789990359,373.21338930519,
373.648262617,374.083135928675,374.952882551611,375.822629173987,376.257502484962,
376.692375795793,377.12724910648,377.562122417021,377.996995727417,378.431869037666,
378.866742347767,379.302468349591,379.738194351416,380.173067661222,380.607940970879,
381.042814280388,381.477687589749,381.91256089896,382.347434208023,382.782307516937,
383.217180825703,383.652054134321,384.086927442791,384.521800751113,384.956674059289,
385.391547367318,385.826420675202,386.262146675918,386.697872676635,387.13274598423,
387.567619291681,388.00249259899,388.437365906157,388.872239213185,389.307112520073,
389.741985826823,390.176859133436,390.611732439914,391.046605746258,391.48147905247,
391.91635235855,392.351225664501,392.786098970323,393.221824970019,393.657550969714,
394.092424275286,394.527297580735,394.962170886063,395.397044191272,395.831917496364,
396.266790801341,396.701664106204,397.136537410957,397.5714107156,398.006284020137,
398.441157324569,398.876030628899,399.310903933128,399.74577723726,400.181503236126,
400.617229234991,401.052102538934,401.486975842787,401.921849146551,402.356722450231,
402.791595753827,403.226469057342,403.66134236078,404.096215664142,404.531088967432,
404.965962270651,405.400835573804,405.835708876892,406.270582179918,406.705455482886,
407.141181481189,407.576907479491,408.01178078235,408.446654085157,408.881527387917,
409.316400690633,409.751273993306,410.186147295941,410.62102059854,411.055893901106,
411.490767203642,411.925640506151,412.360513808636,412.795387111099,413.230260413545,
413.665133715976,414.100859714032,414.536585712088,414.971459014498,415.406332316901,
415.841205619301,416.276078921702,416.710952224105,417.145825526515,417.580698828933,
418.015572131364,418.45044543381,418.885318736273,419.320192038758,419.755065341267,
420.189938643803,420.624811946369,421.060537944515,421.496263942662,421.931137245297,
422.36601054797,422.800883850686,423.235757153446,423.670630456253,424.105503759112,
424.540377062023,424.975250364991,425.410123668017,425.844996971105,426.279870274258,
426.714743577477,427.149616880767,427.584490184129,428.020216182695,428.455942181261,
428.890815484776,429.325688788373,429.760562092052,430.195435395816,430.630308699669,
431.065182003612,431.500055307649,431.93492861178,432.36980191601,432.80467522034,
433.239548524772,433.674421829309,434.109295133952,434.544168438705,434.979894437984,
435.415620437262,435.850493742239,436.285367047331,436.72024035254,437.155113657869,
437.589986963318,438.024860268889,438.459733574586,438.894606880409,439.32948018636,
439.76435349244,440.199226798651,440.634100104995,441.068973411473,441.503846718087,
441.939572718309,442.375298718531,442.810172025419,443.245045332447,443.679918639614,
444.114791946923,444.549665254374,444.984538561969,445.419411869708,445.854285177591,
446.289158485621,446.724031793796,447.158905102119,447.593778410589,448.028651719207,
448.463525027973,448.899251029277,449.334977030581,449.769850339644,450.639596958216,
451.074470267725,451.509343577383,451.944216887189,452.379090197143,452.813963507244,
453.248836817493,453.683710127889,454.118583438431,454.553456749117,454.988330059949,
455.423203370923,455.858929373329,456.294655375734,456.729528686993,457.164401998391,
457.599275309929,458.469021933414,458.90389524536,459.338768557437,459.773641869646,
460.208515181983,460.643388494447,461.078261807036,461.948008432578,462.818607748906,
463.689207065461,464.55895369214,465.428700319234,466.298446946716,467.16819357456,
468.037940202737,468.907686831215,469.778286149605,470.648885468116,471.518632097196,
472.388378726451,473.258125355841,474.127871985322,474.997618614851,475.86736524438,
476.737964563343,477.608563882265,478.478310511593,479.348057140765,480.217803769743,
481.087550398488,481.957297026966,482.827043655142,483.697642972895,484.568242290469,
485.43798891776,486.307735544649,487.177482171112,488.047228797125,488.916975422667,
489.78672204772,490.657321363009,491.09304736596,491.527920678038,492.397667301793,
493.267413925005,494.137160547663,494.57203385878,495.006907169755,495.441780480586,
495.876653791273,496.311527101814,496.74640041221,497.616999724357,498.052725726255,
498.487599036209,498.922472346015,499.357345655673,499.792218965182,500.227092274542,
500.661965583754,501.096838892816,501.531712201731,501.966585510497,502.401458819114,
502.836332127584,503.271205435907,503.706078744082,504.140952052112,504.576678052901,
505.01240405369,505.447277361429,505.882150669023,506.317023976474,506.751897283783,
507.186770590951,507.621643897978,508.056517204866,508.491390511616,508.92626381823,
509.361137124708,509.796010431052,510.230883737263,510.665757043344,511.100630349294,
511.536356349053,511.972082348811,512.406955654506,512.841828960076,513.276702265523,
513.711575570849,514.146448876056,514.581322181146,515.016195486121,515.451068790983,
515.885942095733,516.320815400375,516.75568870491,517.19056200934,517.625435313668,
518.060308617896,518.496034616807,518.931760615718,519.366633919752,519.801507223694,
520.236380527545,520.671253831307,521.106127134985,521.541000438579,521.975873742092,
522.410747045528,522.845620348888,523.280493652176,523.715366955394,524.150240258545,
524.585113561631,525.019986864656,525.455712862985,525.891438861313,526.326312164223,
526.761185467079,527.196058769885,527.630932072643,528.065805375356,528.500678678029,
528.935551980661,529.370425283258,529.805298585822,530.240171888356,530.675045190863,
531.109918493346,531.544791795808,531.979665098252,532.415391096312,532.851117094373,
533.285990396789,533.720863699197,534.155737001598,534.590610303997,535.025483606395,
535.460356908796,535.895230211204,536.330103513621,536.764976816049,537.199850118493,
537.634723420955,538.069596723438,538.504470025945,538.93934332848,539.375069326608,
539.810795324736,540.245668627333,540.680541929966,541.115415232637,541.550288535351,
541.985161838109,542.420035140915,542.854908443771,543.28978174668,543.724655049646,
544.15952835267,544.594401655757,545.029274958907,545.464148262125,545.899021565413,
546.334747563939,546.770473562465,547.205346865901,547.640220169415,548.075093473009,
548.509966776686,548.944840080449,549.3797133843,549.814586688241,550.249459992276,
550.684333296405,551.119206600633,551.554079904961,551.988953209391,552.423826513926,
552.858699818567,553.294425817789,553.73015181701,554.165025121872,554.599898426846,
555.034771731937,555.469645037144,555.90451834247,556.339391647917,556.774264953487,
557.209138259182,557.644011565003,558.078884870951,558.51375817703,558.948631483239,
559.383504789581,559.818378096058,560.254104096209,560.689830096361,561.12470340311,
561.559576709996,561.994450017021,562.429323324187,562.864196631494,563.299069938943,
563.733943246536,564.168816554273,564.603689862154,565.038563170182,565.473436478355,
565.908309786676,566.343183095144,566.77805640376,567.213782404988,567.649508406216,
568.084381715128,568.519255024189,568.954128333399,569.389001642757,569.823874952264,
570.258748261921,570.693621571725,571.128494881677,571.563368191777,572.433114812417,
572.867988122957,573.302861433642,573.737734744471,574.173460746804,574.609186749136,
575.044060060251,575.913806682904,576.783553306113,577.218426617922,577.653299929865,
578.08817324194,578.523046554147,579.392793178944,580.26253980424,581.13313912039,
581.568865123709,582.003738436771,582.87348506323,583.743231690115,584.612978317402,
585.482724945065,586.352471573076,587.222218201403,588.092817519691,588.963416838109,
589.833163467083,590.702910096251,591.572656725575,592.442403355013,593.31214998452,
594.181896614051,595.05249593303,595.92309525198,596.792841881366,597.662588510618,
598.532335139693,599.402081768556,600.271828397167,601.141575025495,602.012174343369,
602.882773661074,603.752520288553,604.622266915642,605.492013542317,606.361760168553,
607.23150679433,608.101253419626,608.971852735101,609.842452050322,610.71219867434,
611.581945297822,612.451691920754,612.886565232011,613.321438543126,613.756311854099,
614.191185164928,615.060931786153,615.931531098516,616.367257100486,616.802130410586,
617.237003720538,617.671877030342,618.106750339998,618.541623649505,618.976496958863,
619.411370268073,619.846243577134,620.281116886046,620.71599019481,621.150863503426,
621.585736811894,622.020610120214,622.455483428388,622.891209429248,623.326935430108,
623.761808737989,624.196682045726,624.631555353319,625.066428660769,625.501301968075,
625.936175275241,626.371048582266,626.805921889153,627.240795195901,627.675668502512,
628.110541808988,628.54541511533,628.98028842154,629.415161727618,629.850887727438,
630.286613727259,630.72148703308,631.156360338774,631.591233644344,632.026106949791,
632.460980255118,632.895853560325,633.330726865415,633.76560017039,634.200473475251,
634.635346780002,635.070220084644,635.505093389179,635.939966693609,636.374839997937,
636.810565996897,637.246291995857,637.681165299986,638.116038604021,638.550911907962,
638.985785211813,639.420658515576,639.855531819253,640.290405122847,640.725278426361,
641.160151729796,641.595025033157,642.029898336444,642.464771639662,642.899644942813,
643.334518245899,643.770244244257,644.205970242616,644.640843545581,645.075716848491,
645.510590151347,645.945463454153,646.380336756911,646.815210059625,647.250083362296,
647.684956664929,648.119829967526,648.55470327009,648.989576572624,649.424449875131,
649.859323177614,650.294196480076,650.729922478144,651.165648476212,651.600521778641,
652.035395081057,652.470268383465,652.905141685866,653.340014988265,653.774888290663,
654.209761593065,654.644634895472,655.079508197889,655.514381500318,655.949254802762,
656.384128105224,656.819001407706,657.253874710213,657.689600708326,658.12532670644,
658.560200009004,658.995073311601,659.429946614234,659.864819916905,660.299693219619,
660.734566522377,661.169439825183,661.604313128039,662.039186430948,662.474059733914,
662.908933036938,663.343806340025,663.778679643175,664.213552946393,664.649278944883,
665.085004943373,665.519878246733,665.954751550169,666.389624853683,666.824498157277,
667.259371460954,667.694244764717,668.129118068568,668.563991372509,668.998864676544,
669.433737980674,669.868611284901,670.303484589229,670.738357893659,671.173231198194,
671.608957197361,672.044683196528,672.479556501278,672.91442980614,673.349303111115,
673.784176416205,674.219049721412,674.653923026738,675.088796332185,675.523669637755,
675.95854294345,676.393416249271,676.82828955522,677.263162861298,677.698036167508,
678.13290947385,678.568635473934,679.004361474018,679.439234780629,679.874108087377,
680.308981394264,680.743854701289,681.178728008455,681.613601315762,682.048474623211,
682.483347930804,682.91822123854,683.353094546422,683.78796785445,684.222841162623,
684.657714470944,685.092587779412,685.528313780566,685.96403978172,686.398913090483,
686.833786399396,687.268659708457,687.703533017666,688.138406327025,688.573279636532,
689.008152946187,689.443026255992,689.877899565944,690.312772876043,690.74764618629,
691.182519496684,691.617392807224,692.052266117909,692.487992120169,692.92371812243,
693.358591433403,694.228338055774,694.663211367171,695.098084678707,695.532957990379,
695.967831302188,696.402704614131,696.837577926207,697.707324550749,698.577071175797,
699.011944488507,699.447670491767,699.883396495028,700.318269807975,701.188016434211,
702.057763060886,702.927509687976,703.797256315454,704.667002943295,705.536749571467,
706.407348889651,707.277948207973,708.147694836835,709.017441465911,709.887188095163,
710.756934724548,711.626681354026,712.496427983551,713.367027302543,714.237626621516,
715.107373250954,715.977119880277,716.846866509446,717.716613138419,718.586359767161,
719.456106395635,720.32670571363,721.197305031464,722.067051659126,722.936798286414,
723.806544913299,724.676291539758,725.546038165767,726.415784791305,727.286384106969,
728.156983422381,729.026730046663,729.896476670415,730.331349982088,730.766223293624,
731.201096605021,731.635969916278,732.505716538366,733.37546315988,733.81033647042,
734.246062472462,734.681788474505,735.116661784752,735.551535094852,735.986408404804,
736.421281714608,736.856155024264,737.291028333771,737.72590164313,738.160774952339,
738.5956482614,739.030521570312,739.465394879076,739.900268187692,740.33514149616,
740.77001480448,741.205740805414,741.641466806347,742.076340114374,742.511213422256,
742.946086729993,743.380960037585,743.815833345035,744.250706652341,744.685579959507,
745.120453266533,745.555326573419,745.990199880167,746.425073186778,746.859946493254,
747.294819799596,747.729693105806,748.165419105691,748.601145105576,749.036018411525,
749.470891717346,749.90576502304,750.34063832861,750.775511634057,751.210384939384,
751.645258244591,752.080131549682,752.515004854656,752.949878159518,753.384751464269,
753.81962476891,754.254498073445,754.689371377875,755.125097376885,755.560823375895,
755.995696680123,756.430569984253,756.865443288287,757.300316592228,757.735189896079,
758.170063199842,758.604936503519,759.039809807113,759.474683110627,759.909556414062,
760.344429717423,760.779303020711,761.214176323929,761.649049627079,762.084775625469,
762.520501623858,762.955374926883,763.390248229848,763.825121532758,764.259994835614,
764.694868138419,765.129741441178,765.564614743891,765.999488046563,766.434361349196,
766.869234651793,767.304107954357,767.738981256891,768.173854559398,768.608727861881,
769.044453859958,769.480179858035,769.915053160479,770.349926462907,770.784799765324,
771.219673067731,771.654546370133,772.089419672531,772.52429297493,772.959166277331,
773.394039579739,773.828912882155,774.263786184584,774.698659487028,775.13353278949,
775.568406091973,776.004132090072,776.439858088172,776.874731390706,777.30960469327,
777.744477995867,778.1793512985,778.614224601171,779.049097903885,779.483971206643,
779.918844509449,780.353717812305,780.788591115215,781.22346441818,781.658337721205,
782.093211024291,782.528084327442,782.963810325897,783.399536324352,783.834409627639,
784.269282931,784.704156234435,785.139029537949,785.573902841543,786.00877614522,
786.443649448983,786.878522752834,787.313396056775,787.74826936081,788.183142664939,
788.618015969167,789.052889273495,789.487762577925,789.923488577038,790.359214576152,
790.794087880793,791.228961185544,791.663834490406,792.098707795381,792.533581100471,
792.968454405678,793.403327711004,793.838201016451,794.273074322021,794.707947627716,
795.142820933537,795.577694239486,796.012567545564,796.447440851774,796.883166851791,
797.318892851808,797.753766158284,798.188639464895,798.623512771643,799.058386078529,
799.493259385555,799.92813269272,800.363006000027,800.797879307477,801.232752615069,
801.667625922806,802.102499230688,802.537372538715,802.972245846889,803.40711915521,
803.84284515629,804.27857115737,804.713444465985,805.148317774749,805.583191083662,
806.018064392723,806.452937701933,806.887811011291,807.322684320798,808.192430940258,
808.62730425021,809.06217756031,809.497050870557,809.931924180951,810.36679749149,
810.802523493679,811.238249495867,811.673122806697,812.542869428785,812.977742740041,
813.412616051438,813.847489362974,814.282362674646,814.717235986455,815.152109298398,
816.021855922681,816.891602547478,817.326475860065,817.762201863265,818.197927866466,
818.632801179295,819.502547805304,820.372294431763,821.242041058648,822.111787685935,
822.981534313598,823.851280941609,824.721880259681,825.5924795779,826.462226206642,
827.331972835616,828.201719464785,829.071466094109,829.941212723546,830.810959353053,
831.681558672047,832.552157991036,833.421904620514,834.2916512499,835.161397879151,
836.031144508226,836.900891137089,837.770637765701,838.641237083811,839.511836401767,
840.381583029608,841.251329657086,842.121076284176,842.990822910851,843.860569537087,
844.730316162863,845.600915478712,846.471514794314,847.341261418855,848.211008042874,
848.645881354683,849.080754666356,849.515627977891,849.950501289288,850.82024791166,
851.689994533462,852.124867844147,852.560593846263,852.996319848379,853.431193158772,
853.866066469019,854.300939779119,855.170686398875,855.605559708531,856.040433018038,
856.475306327397,856.910179636606,857.345052945667,857.77992625458,858.214799563344,
858.64967287196,859.084546180427,859.520272181434,859.95599818244,860.390871490614,
860.825744798641,861.260618106523,861.69549141426,862.130364721852,862.565238029302,
863.000111336609,863.434984643774,863.8698579508,864.304731257686,864.739604564434,
865.174477871045,865.609351177521,866.044224483863,866.479950483814,866.915676483765,
867.350549789843,867.785423095792,868.220296401613,868.655169707307,869.090043012877,
869.524916318325,869.959789623651,870.394662928858,870.829536233948,871.264409538923,
871.699282843785,872.134156148535,872.569029453177,873.003902757712,873.439628756773,
873.875354755834,874.310228060162,874.745101364389,875.179974668519,875.614847972553,
876.049721276495,876.484594580346,876.919467884108,877.354341187786,877.78921449138,
878.224087794893,878.658961098329,879.093834401689,879.528707704977,879.963581008195,
880.399307006616,880.835033005038,881.269906308124,881.704779611148,882.139652914114,
882.574526217024,883.00939951988,883.444272822685,883.879146125444,884.314019428157,
884.748892730829,885.183766033462,885.618639336059,886.053512638623,886.488385941157,
886.923259243664,887.358985241751,887.794711239839,888.2295845423,888.664457844744,
889.099331147173,889.534204449589,889.969077751997,890.403951054398,890.838824356797,
891.273697659195,891.708570961597,892.143444264004,892.578317566421,893.01319086885,
893.448064171293,893.882937473755,894.318663471843,894.75438946993,895.189262772437,
895.624136074971,896.059009377535,896.493882680132,896.928755982765,897.363629285437,
897.798502588151,898.233375890909,898.668249193715,899.103122496571,899.53799579948,
899.972869102446,900.40774240547,900.842615708556,901.278341706978,901.714067705399,
902.148941008617,902.583814311905,903.018687615265,903.453560918701,903.888434222214,
904.323307525808,904.758180829485,905.193054133248,905.627927437099,906.06280074104,
906.497674045075,906.932547349205,907.367420653433,907.80229395776,908.238019956821,
908.673745955883,909.108619260417,909.543492565059,909.978365869809,910.413239174671,
910.848112479646,911.282985784736,911.717859089943,912.152732395269,912.587605700716,
913.022479006287,913.457352311981,913.892225617802,914.327098923751,914.761972229829,
915.19769822978,915.633424229731,916.068297536072,916.503170842548,916.93804414916,
917.372917455908,917.807790762794,918.24266406982,918.677537376985,919.112410684292,
919.547283991742,919.982157299334,920.417030607071,920.851903914953,921.28677722298,
921.721650531154,922.15737653216,922.593102533167,923.027975841635,923.46284915025,
923.897722459014,924.332595767926,924.767469076987,925.202342386197,925.637215695556,
926.072089005063,926.506962314719,926.941835624523,927.376708934475,927.811582244575,
928.246455554822,928.681328865215,929.117054867331,929.987654180132,930.422527490961,
930.857400801934,931.292274113049,931.727147424306,932.162020735703,932.596894047238,
933.46664067072,934.336387294739,934.771260606945,935.20613391928,935.641007231742,
936.076733234882,936.94733255073,937.817079176507,938.686825802743,939.556572429418,
940.426319056508,941.296065683986,942.165812311827,943.036411629783,943.907010947893,
944.776757576505,945.646504205367,946.516250834443,947.385997463694,948.25574409308,
949.125490722558,949.996090041546,950.86668936054,951.736435990048,952.606182619485,
953.475929248809,954.345675877978,955.215422506951,956.085169135693,956.955768453912,
957.826367771985,958.696114399995,959.565861027658,960.435607654946,961.305354281831,
962.175100908289,963.044847534298,963.915446850328,964.786046166116,965.655792790913,
966.525539415195,966.960412727138,967.395286038947,968.265032662155,969.134779284809,
969.569652595924,970.004525906897,970.439399217726,970.875125219914,971.310851222103,
971.745724532643,972.615471153283,973.485217773335,973.920091083139,974.354964392795,
974.789837702302,975.22471101166,975.65958432087,976.094457629931,976.529330938844,
976.964204247608,977.399077556223,977.834803557303,978.270529558383,978.705402866704,
979.140276174877,979.575149482905,980.010022790786,980.444896098523,980.879769406116,
981.314642713565,981.749516020872,982.184389328038,982.619262635063,983.05413594195,
983.489009248698,983.923882555309,984.358755861785,984.794481861802,985.230207861819,
985.665081168029,986.099954474107,986.534827780056,986.969701085877,987.404574391571,
987.839447697141,988.274321002589,988.709194307915,989.144067613122,989.578940918212,
990.013814223187,990.448687528048,990.883560832799,991.31843413744,991.754160136554,
992.189886135667,992.624759440097,993.059632744425,993.494506048653,993.929379352783,
994.364252656817,994.799125960758,995.233999264609,995.668872568372,996.103745872049,
996.538619175643,996.973492479157,997.408365782593,997.843239085953,998.278112389241,
998.713838387696,999.149564386151,999.584437689301,1000.01931099239,1000.45418429541,
1000.88905759838,1001.32393090129,1001.75880420414,1002.19367750695,1002.62855080971,
1003.06342411242,1003.49829741509,1003.93317071773,1004.36804402032,1004.80291732289,
1005.23779062542,1005.67351662352,1006.10924262162,1006.5441159241,1006.97898922656,
1007.41386252901,1007.84873583144,1008.28360913385,1008.71848243626,1009.15335573866,
1009.58822904106,1010.02310234346,1010.45797564586,1010.89284894827,1011.32772225069,
1011.76259555311,1012.19746885556,1012.63319485364,1013.06892085171,1013.5037941542,
1013.9386674567,1014.37354075924,1014.8084140618,1015.2432873644,1015.67816066703,
1016.1130339697,1016.54790727242,1016.98278057517,1017.41765387798,1017.85252718084,
1018.28740048375,1018.72227378671,1019.15714708974,1019.59287308813,1020.02859908651,
1020.46347238967,1020.89834569288,1021.33321899617,1021.76809229953,1022.20296560297,
1022.63783890648,1023.07271221007,1023.50758551375,1023.94245881752,1024.37733212137,
1024.81220542531,1025.24707872935,1025.68195203348,1026.11682533771,1026.55255133672,
1026.98827733573,1027.42315064016,1027.8580239447,1028.29289724934,1028.72777055409,
1029.16264385896,1029.59751716393,1030.03239046902,1030.46726377423,1030.90213707956,
1031.33701038501,1031.77188369058,1032.20675699628,1032.6416303021,1033.07650360805,
1033.51222960793,1033.94795560782,1034.38282891403,1034.81770222038,1035.25257552685,
1035.68744883347,1036.12232214022,1036.5571954471,1036.99206875413,1037.4269420613,
1037.86181536861,1038.29668867606,1038.73156198365,1039.16643529139,1039.60130859927,
1040.0361819073,1040.47190790824,1040.90763390917,1041.34250721749,1041.77738052596,
1042.21225383458,1042.64712714334,1043.08200045226,1043.95174707053,1044.38662037989,
1044.8214936894,1045.25636699906,1045.69124030886,1046.12611361882,1046.56098692892,
1046.99586023917,1047.43158624121,1047.86731224325,1048.3021855538,1048.73705886448,
1049.17193217531,1049.60680548629,1050.0416787974,1050.47655210866,1050.91142542006,
1051.78117204327,1052.21604535508,1052.65091866703,1053.0857919791,1053.52066529131,
1053.95553860365,1054.39126460673,1055.26186392239,1056.13161054793,1057.00135717395,
1057.43623048712,1057.87110380041,1058.7408504273,1059.61059705459,1060.48034368225,
1061.35094300009,1062.22154231809,1063.09128894656,1063.96103557531,1064.83078220429,
1065.70052883346,1066.57027546278,1067.44002209222,1068.3106214112,1069.18122073019,
1070.05096735972,1070.9207139892,1071.79046061859,1072.66020724785,1073.52995387693,
1074.39970050579,1075.27029982411,1076.1408991423,1077.01064577048,1077.88039239832,
1078.7501390258,1079.61988565289,1080.48963227957,1081.35937890581,1082.22997822202,
1083.100577538,1083.97032416305,1084.84007078759,1085.70981741161,1086.5795640351,
1087.44931065803,1087.88418396929,1088.31905728041,1088.75393059138,1089.18965659365,
1089.62538259591,1090.06025590659,1090.93000252753,1091.36487583778,1091.79974914788,
1092.23462245783,1092.66949576764,1093.1043690773,1093.5392423868,1093.97411569616,
1094.40898900538,1094.84386231444,1095.27873562335,1095.71360893212,1096.14933493327,
1096.58506093443,1097.0199342429,1097.45480755122,1097.88968085939,1098.32455416742,
1098.75942747531,1099.19430078305,1099.62917409064,1100.06404739809,1100.4989207054,
1100.93379401257,1101.36866731959,1101.80354062648,1102.23841393323,1102.67328723984,
1103.10901323993,1103.54473924001,1103.97961254636,1104.41448585257,1104.84935915865,
1105.2842324646,1105.71910577042,1106.15397907612,1106.58885238169,1107.02372568714,
1107.45859899246,1107.89347229767,1108.32834560276,1108.76321890774,1109.1980922126,
1109.63296551736,1110.06869151652,1110.50441751569,1110.93929082023,1111.37416412466,
1111.80903742899,1112.24391073322,1112.67878403735,1113.11365734139,1113.54853064533,
1113.98340394918,1114.41827725295,1114.85315055662,1115.28802386022,1115.72289716374,
1116.15777046717,1116.59264377053,1117.02836976903,1117.46409576752,1117.89896907074,
1118.33384237389,1118.76871567698,1119.20358898,1119.63846228297,1120.07333558588,
1120.50820888874,1120.94308219154,1121.3779554943,1121.81282879702,1122.24770209969,
1122.68257540233,1123.11744870492,1123.55232200749,1123.98804800561,1124.42377400372,
1124.85864730623,1125.29352060871,1125.72839391118,1126.16326721362,1126.59814051605,
1127.03301381847,1127.46788712088,1127.90276042328,1128.33763372568,1128.77250702808,
1129.20738033048,1129.64225363289,1130.07712693531,1130.51200023774,1130.94772623581,
1131.38345223388,1131.81832553634,1132.25319883883,1132.68807214134,1133.12294544387,
1133.55781874644,1133.99269204904,1134.42756535167,1134.86243865434,1135.29731195706,
1135.73218525982,1136.16705856263,1136.60193186548,1137.03680516839,1137.47167847136,
1137.90740446972,1138.34313046808,1138.77800377117,1139.21287707432,1139.64775037754,
1140.08262368083,1140.51749698419,1140.95237028763,1141.38724359114,1141.82211689474,
1142.25699019842,1142.69186350218,1143.12673680603,1143.56161010998,1143.99648341401,
1144.43135671814,1144.86708271711,1145.30280871607,1145.7376820204,1146.17255532483,
1146.60742862936,1147.04230193401,1147.47717523876,1147.91204854362,1148.3469218486,
1148.78179515369,1149.2166684589,1149.65154176423,1150.08641506968,1150.52128837525,
1150.95616168094,1151.39103498677,1151.82676098659,1152.26248698641,1152.69736029249,
1153.1322335987,1153.56710690504,1154.00198021152,1154.43685351813,1154.87172682488,
1155.30660013177,1155.7414734388,1156.17634674597,1156.61122005327,1157.04609336073,
1157.48096666832,1157.91583997606,1158.35071328394,1158.7864392848,1159.22216528566,
1159.65703859384,1160.09191190216,1160.52678521063,1160.96165851925,1161.39653182801,
1161.83140513693,1162.26627844599,1162.7011517552,1163.13602506456,1163.57089837407,
1164.00577168373,1164.44064499353,1164.87551830349,1165.74611761556,1166.18184361753,
1166.61671692792,1167.05159023846,1167.48646354915,1167.92133685998,1168.35621017096,
1169.22595679333,1170.09570341627,1170.53057672794,1170.96545003975,1171.4003233517,
1171.83519666377,1172.27006997598,1172.705795979,1173.57639529447,1174.44614191977,
1174.8810152326,1175.31588854555,1176.18563517179,1177.05538179847,1177.92512842556,
1178.79487505304,1179.66547437075,1180.53607368863,1181.40582031696,1182.27556694557,
1183.14531357444,1184.01506020352,1184.88480683277,1185.75455346216,1186.62515278112,
1187.4957521001,1188.36549872963,1189.23524535914,1190.10499198858,1190.97473861791,
1191.84448524708,1192.71423187606,1193.58483119448,1194.45543051277,1195.3251771411,
1196.19492376911,1197.06467039678,1197.93441702407,1198.80416365096,1199.67391027742,
1200.5445095938,1201.41510890996,1202.28485553525,1203.15460216005,1204.02434878434,
1204.89409540809,1205.76384203131,1206.1987153427,1206.63358865396,1207.06846196508,
1207.50418796741,1208.37478728058,1209.2445339018,1209.6794072122,1210.11428052245,
1210.54915383255,1210.9840271425,1211.41890045231,1211.85377376197,1212.28864707147,
1212.72352038083,1213.15839369005,1213.59326699911,1214.02814030802,1214.46386630925,
1214.89959231048,1215.3344656191,1215.76933892757,1216.20421223589,1216.63908554406,
1217.07395885209,1217.50883215998,1217.94370546771,1218.37857877531,1218.81345208276,
1219.24832539007,1219.68319869724,1220.11807200426,1220.55294531115,1220.9878186179,
1221.42354461805,1221.85927061821,1222.29414392468,1222.72901723103,1223.16389053724,
1223.59876384332,1224.03363714927,1224.46851045509,1224.90338376079,1225.33825706636,
1225.77313037181,1226.20800367713,1226.64287698234,1227.07775028743,1227.51262359241,
1227.94749689727,1228.3832228965,1228.81894889572,1229.25382220036,1229.6886955049,
1230.12356880933,1230.55844211366,1230.99331541789,1231.42818872202,1231.86306202606,
1232.29793533,1232.73280863385,1233.16768193762,1233.60255524129,1234.03742854489,
1234.4723018484,1234.90717515184,1235.34290115037,1235.7786271489,1236.21350045219,
1236.64837375541,1237.08324705856,1237.51812036165,1237.95299366467,1238.38786696764,
1238.82274027055,1239.25761357341,1239.69248687621,1240.12736017897,1240.56223348169,
1240.99710678436,1241.431980087,1241.8668533896,1242.30257938773,1242.73830538585,
1243.17317868839,1243.6080519909,1244.04292529338,1244.47779859585,1244.91267189829,
1245.34754520072,1245.78241850314,1246.21729180555,1246.65216510795,1247.08703841035,
1247.52191171275,1247.95678501515,1248.39165831756,1248.82653161998,1249.26225761804,
1249.69798361611,1250.13285691855,1250.56773022101,1251.0026035235,1251.43747682601,
1251.87235012854,1252.30722343111,1252.74209673371,1253.17697003634,1253.61184333901,
1254.04671664173,1254.48158994449,1254.9164632473,1255.35133655015,1255.78620985306,
1256.22193585139,1256.65766184973,1257.09253515275,1257.52740845584,1257.96228175899,
1258.39715506221,1258.8320283655,1259.26690166886,1259.7017749723,1260.13664827581,
1260.57152157941,1261.00639488309,1261.44126818685,1261.8761414907,1262.31101479465,
1262.74588809868,1263.1816140976,1263.61734009651,1264.05221340074,1264.48708670507,
1264.9219600095,1265.35683331403,1265.79170661868,1266.22657992343,1266.66145322829,
1267.09632653327,1267.53119983836,1267.96607314357,1268.4009464489,1268.83581975434,
1269.27069305992,1269.70556636561,1270.14129236537,1270.57701836513,1271.01189167108,
1271.44676497716,1271.88163828337,1272.31651158971,1272.75138489619,1273.1862582028,
1273.62113150955,1274.05600481644,1274.49087812347,1274.92575143063,1275.36062473794,
1275.79549804539,1276.23037135299,1276.66524466073,1277.10097066151,1277.5366966623,
1277.97156997033,1278.40644327851,1278.84131658683,1279.2761898953,1279.71106320392,
1280.14593651268,1280.5808098216,1281.01568313066,1281.45055643987,1281.88542974923,
1282.32030305874,1282.75517636839,1283.1900496782,1283.62492298815,1284.06064899005,
1284.49637499195,1284.9312483022,1285.36612161259,1285.80099492313,1286.23586823382,
1286.67074154465,1287.54048816674,1287.975361478,1288.4102347894,1288.84510810093,
1289.27998141261,1289.71485472442,1290.14972803636,1291.02032735139,1291.89092666668,
1292.32579997914,1292.76067329173,1293.19554660444,1293.63041991727,1294.50016654328,
1295.36991316974,1296.23965979663,1297.10940642392,1297.9800057415,1298.85060505925,
1299.72035168742,1300.5900983159,1301.45984494464,1302.32959157362,1303.19933820279,
1304.06908483212,1304.93968415104,1305.81028347,1306.68003009953,1307.54977672906,
1308.41952335854,1309.28926998793,1310.15901661718,1311.02876324626,1311.89936256477,
1312.76996188316,1313.63970851164,1314.50945513981,1315.37920176765,1316.24894839514,
1317.11869502223,1317.98844164891,1318.85904096546,1319.72964028179,1320.59938690733,
1321.46913353238,1322.33888015692,1323.20862678095,1323.64350009276,1324.07837340443,
1324.51324671597,1324.94812002737,1325.81871934103,1326.68931865441,1327.12419196524,
1327.55906527593,1327.99393858647,1328.42881189686,1328.86368520711,1329.29855851721,
1329.73343182716,1330.16830513697,1330.60317844663,1331.03805175614,1331.4729250655,
1331.90779837471,1332.34267168377,1332.77839768507,1333.21412368638,1333.64899699514,
1334.08387030376,1334.51874361223,1334.95361692055,1335.38849022873,1335.82336353676,
1336.25823684464,1336.69311015238,1337.12798345997,1337.56285676742,1337.99773007473,
1338.4326033819,1338.86747668892,1339.30234999581,1339.73807599603,1340.17380199625,
1340.60867530287,1341.04354860934,1341.47842191569,1341.9132952219,1342.34816852798,
1342.78304183393,1343.21791513975,1343.65278844545,1344.08766175102,1344.52253505647,
1344.95740836179,1345.392281667,1345.82715497209,1346.26202827707,1346.69775427635,
1347.13348027563,1347.56835358038,1348.00322688502,1348.43810018956,1348.87297349399,
1349.30784679832,1349.74272010255,1350.17759340668,1350.61246671072,1351.04734001466,
1351.48221331851,1351.91708662228,1352.35195992595,1352.78683322955,1353.22170653306,
1353.65743253163,1354.09315853019,1354.52803183356,1354.96290513685,1355.39777844007,
1355.83265174322,1356.26752504631,1356.70239834933,1357.1372716523,1357.57214495521,
1358.00701825807,1358.44189156087,1358.87676486363,1359.31163816635,1359.74651146902,
1360.18138477166,1360.6171107698,1361.05283676795,1361.48771007051,1361.92258337305,
1362.35745667556,1362.79232997804,1363.2272032805,1363.66207658295,1364.09694988538,
1364.5318231878,1364.96669649021,1365.40156979261,1365.83644309501,1366.27131639741,
1366.70618969981,1367.14106300222,1367.57678900028,1368.01251499834,1368.44738830077,
1368.88226160321,1369.31713490567,1369.75200820816,1370.18688151067,1370.6217548132,
1371.05662811577,1371.49150141837,1371.926374721,1372.36124802367,1372.79612132639,
1373.23099462915,1373.66586793196,1374.10074123481,1374.53646723311,1374.97219323142,
1375.40706653438,1375.84193983741,1376.2768131405,1376.71168644365,1377.14655974687,
1377.58143305016,1378.01630635352,1378.45117965696,1378.88605296047,1379.32092626407,
1379.75579956775,1380.19067287151,1380.62554617536,1381.06041947931,1381.49614547817,
1381.93187147704,1382.36674478117,1382.8016180854,1383.23649138973,1383.67136469416,
1384.10623799869,1384.54111130334,1384.97598460809,1385.41085791295,1385.84573121793,
1386.28060452302,1386.71547782823,1387.15035113356,1387.585224439,1388.02009774458,
1388.45582374427,1388.89154974397,1389.32642304979,1389.76129635574,1390.19616966182,
1390.63104296803,1391.06591627437,1391.50078958085,1391.93566288746,1392.37053619421,
1392.8054095011,1393.24028280813,1393.6751561153,1394.1100294226,1394.54490273005,
1394.97977603765,1395.41550203836,1395.85122803908,1396.28610134696,1396.72097465499,
1397.15584796317,1397.59072127149,1398.02559457996,1398.46046788858,1398.89534119734,
1399.33021450626,1399.76508781532,1400.19996112453,1400.63483443389,1401.50458105306,
1401.93945436286,1402.37518036469,1402.81090636651,1403.24577967661,1403.68065298686,
1404.11552629725,1404.5503996078,1404.98527291848,1405.85501954029,1406.2898928514,
1406.72476616266,1407.15963947406,1407.5945127856,1408.02938609727,1408.46425940908,
1409.33485872391,1410.205458039,1410.64033135134,1411.07520466381,1411.51007797639,
1411.9449512891,1412.81469791488,1413.68444454112,1414.5541911678,1415.42393779489,
1416.29453711233,1417.16513642995,1418.03488305796,1418.90462968629,1419.77437631491,
1420.64412294377,1421.51386957285,1422.38361620211,1423.25421552099,1424.12481483992,
1424.99456146943,1425.86430809896,1426.73405472847,1427.60380135791,1428.47354798724,
1429.34329461641,1430.21389393501,1431.08449325349,1431.9542398821,1432.82398651043,
1433.69373313844,1434.56347976611,1435.4332263934,1436.30297302029,1437.17357233701,
1438.04417165351,1438.91391827929,1439.78366490459,1440.65341152939,1441.52315815367,
1441.95803146562,1442.39290477743,1442.8277780891,1443.26265140064,1444.13325071451,
1445.00385002811,1445.43872333908,1445.87359664991,1446.3084699606,1446.74334327114,
1447.17821658153,1447.61308989178,1448.48283651184,1448.91770982164,1449.3525831313,
1449.78745644081,1450.22232975017,1450.65720305938,1451.09292906076,1451.52865506214,
1451.96352837105,1452.39840167982,1452.83327498843,1453.2681482969,1453.70302160522,
1454.1378949134,1454.57276822143,1455.00764152931,1455.44251483705,1455.87738814464,
1456.31226145209,1456.7471347594,1457.18200806657,1457.6168813736,1458.05260737389,
1458.48833337418,1458.92320668093,1459.35807998754,1459.79295329402,1460.22782660036,
1460.66269990657,1461.09757321265,1461.5324465186,1461.96731982443,1462.40219313012,
1462.83706643569,1463.27193974114,1463.70681304647,1464.14168635168,1464.57655965677,
1465.0122856561,1465.44801165544,1465.8828849603,1466.31775826505,1466.7526315697,
1467.18750487423,1467.62237817866,1468.05725148299,1468.49212478722,1468.92699809135,
1469.36187139539,1469.79674469933,1470.23161800319,1470.66649130695,1471.10136461063,
1471.53623791422,1471.97196391283,1472.40768991143,1472.84256321487,1473.27743651823,
1473.71230982152,1474.14718312474,1474.58205642789,1475.01692973098,1475.451803034,
1475.88667633697,1476.32154963988,1476.75642294274,1477.19129624555,1477.62616954831,
1478.06104285102,1478.4959161537,1478.93164215186,1479.36736815002,1479.80224145262,
1480.23711475519,1480.67198805772,1481.10686136023,1481.54173466272,1481.97660796518,
1482.41148126762,1482.84635457005,1483.28122787247,1483.71610117488,1484.15097447728,
1484.58584777968,1485.02072108208,1485.45559438449,1485.89132038254,1486.32704638059,
1486.76191968301,1487.19679298544,1487.63166628788,1488.06653959035,1488.50141289283,
1488.93628619534,1489.37115949787,1489.80603280044,1490.24090610304,1490.67577940567,
1491.11065270835,1491.54552601106,1491.98039931382,1492.41527261663,1492.8509986149,
1493.28672461318,1493.72159791609,1494.15647121906,1494.59134452208,1495.02621782517,
1495.46109112832,1495.89596443154,1496.33083773483,1496.76571103819,1497.20058434163,
1497.63545764515,1498.07033094874,1498.50520425242,1498.94007755618,1499.37495086004,
1499.81067685885,1500.24640285767,1500.68127616171,1501.11614946584,1501.55102277007,
1501.9858960744,1502.42076937883,1502.85564268337,1503.29051598801,1503.72538929276,
1504.16026259762,1504.5951359026,1505.03000920769,1505.4648825129,1505.89975581823,
1506.33462912368,1506.77035512331,1507.20608112294,1507.64095442864,1508.07582773446,
1508.51070104041,1508.94557434649,1509.3804476527,1509.81532095904,1510.25019426552,
1510.68506757213,1511.11994087888,1511.55481418577,1511.9896874928,1512.42456079996,
1512.85943410727,1513.29430741472,1513.73003341537,1514.16575941601,1514.60063272375,
1515.03550603163,1515.47037933966,1515.90525264784,1516.34012595616,1516.77499926463,
1517.20987257325,1517.64474588201,1518.07961919093,1518.51449249999,1518.9493658092,
1519.38423911856,1519.81911242807,1520.25398573772,1520.68971173947,1521.12543774122,
1521.56031105118,1521.99518436128,1522.43005767153,1523.29980429246,1523.73467760315,
1524.16955091398,1524.60442422495,1525.03929753607,1525.47417084733,1525.90904415873,
1526.77879078194,1527.64939009657,1528.08511609939,1528.51998941146,1528.95486272367,
1529.38973603601,1530.25948266106,1531.1292292866,1531.99897591261,1532.86872253907,
1533.73846916596,1534.60906848325,1535.47966780073,1536.34941442858,1537.21916105675,
1538.08890768523,1538.95865431398,1539.82840094295,1540.69814757212,1541.56874689096,
1542.43934620985,1543.30909283933,1544.17883946886,1545.04858609839,1545.91833272787,
1546.78807935726,1547.65782598651,1548.52842530518,1549.39902462375,1550.26877125249,
1551.13851788097,1552.00826450914,1552.87801113699,1553.74775776447,1554.61750439156,
1555.48810370844,1556.35870302511,1557.22844965112,1558.09819627666,1558.96794290171,
1559.83768952626,1560.27256283834,1560.70743615028,1561.57718277377,1562.44778208785,
1563.31838140165,1563.75325471277,1564.18812802374,1564.62300133457,1565.05787464526,
1565.9276212662,1566.79736788655,1567.2322411965,1567.66711450631,1568.10198781596,
1568.53686112547,1568.97173443483,1569.40746043628,1569.84318643774,1570.2780597468,
1570.71293305571,1571.14780636448,1571.5826796731,1572.01755298157,1572.45242628989,
1572.88729959806,1573.32217290609,1573.75704621397,1574.19191952171,1574.62679282931,
1575.06166613676,1575.49653944407,1575.93141275123,1576.36713875159,1576.80286475195,
1577.23773805884,1577.67261136559,1578.1074846722,1578.54235797868,1578.97723128502,
1579.41210459124,1579.84697789732,1580.28185120327,1580.71672450909,1581.15159781478,
1581.58647112036,1582.0213444258,1582.45621773113,1582.89109103634,1583.32681703573,
1583.76254303513,1584.1974163401,1584.63228964497,1585.06716294972,1585.50203625436,
1585.9369095589,1586.37178286333,1586.80665616766,1587.24152947189,1587.67640277602,
1588.11127608005,1588.546149384,1588.98102268785,1589.41589599161,1589.85076929529,
1590.28649529394,1590.72222129258,1591.1570945961,1591.59196789953,1592.0268412029,
1592.46171450619,1592.8965878094,1593.33146111256,1593.76633441564,1594.20120771867,
1594.63608102164,1595.07095432455,1595.50582762741,1595.94070093021,1596.37557423297,
1596.81044753569,1597.24617353387,1597.68189953206,1598.11677283469,1598.55164613729,
1598.98651943985,1599.42139274239,1599.8562660449,1600.29113934738,1600.72601264985,
1601.16088595229,1601.59575925472,1602.03063255714,1602.46550585955,1602.90037916195,
1603.33525246435,1603.77012576675,1604.2058517648,1604.64157776285,1605.07645106526,
1605.51132436768,1605.94619767011,1606.38107097255,1606.81594427502,1607.2508175775,
1607.68569088001,1608.12056418254,1608.55543748511,1608.99031078771,1609.42518409034,
1609.86005739302,1610.29493069573,1610.72980399849,1611.16552999674,1611.60125599499,
1612.03612929785,1612.47100260076,1612.90587590373,1613.34074920675,1613.77562250984,
1614.21049581299,1614.64536911621,1615.0802424195,1615.51511572286,1615.9499890263,
1616.38486232981,1616.81973563341,1617.25460893709,1617.68948224085,1618.12520823963,
1618.5609342384,1618.99580754234,1619.43068084638,1619.86555415051,1620.30042745474,
1620.73530075907,1621.1701740635,1621.60504736804,1622.03992067268,1622.47479397743,
1622.90966728229,1623.34454058727,1623.77941389236,1624.21428719757,1624.6491605029,
1625.08488650247,1625.52061250204,1625.95548580761,1626.39035911331,1626.82523241913,
1627.26010572508,1627.69497903116,1628.12985233737,1628.56472564372,1628.99959895019,
1629.43447225681,1629.86934556356,1630.30421887044,1630.73909217747,1631.17396548464,
1631.60883879195,1632.04456479252,1632.48029079309,1632.91516410068,1633.35003740842,
1633.78491071631,1634.21978402433,1634.65465733251,1635.08953064083,1635.5244039493,
1635.95927725792,1636.39415056668,1636.8290238756,1637.26389718466,1637.69877049387,
1638.13364380323,1638.56851711274,1639.00424311442,1639.43996911609,1639.8748424259,
1640.30971573585,1640.74458904595,1641.6143356666,1642.04920897714,1642.48408228782,
1642.91895559865,1643.35382890963,1643.78870222074,1644.223575532,1645.09332215494,
1645.52819546661,1645.96392146936,1646.39964747212,1646.83452078406,1647.26939409614,
1647.70426740834,1648.57401403314,1649.44376065844,1650.31350728422,1650.74838059729,
1651.18325391046,1652.05300053714,1652.92359985428,1653.79419917162,1654.66394579929,
1655.5336924273,1656.40343905563,1657.27318568424,1658.14293231311,1659.01267894219,
1659.88327826096,1660.75387757982,1661.62362420926,1662.49337083877,1663.3631174683,
1664.23286409781,1665.10261072725,1665.97235735658,1666.84295667531,1667.71355599396,
1668.58330262282,1669.45304925143,1670.32279587976,1671.19254250778,1672.06228913544,
1672.93203576273,1673.80263507977,1674.6732343966,1675.54298102284,1676.41272764862,
1677.28247427392,1678.15222089872,1679.021967523,1679.89171414676,1680.76231346105,
1681.19803946366,1681.63291277506,1682.06778608632,1682.50265939743,1682.93753270841,
1683.37240601924,1684.24215264047,1684.67702595086,1685.11189926111,1685.54677257121,
1685.98164588116,1686.41651919097,1686.85139250063,1687.28626581014,1687.72199181166,
1688.15771781319,1688.5925911224,1689.02746443146,1689.46233774038,1689.89721104914,
1690.33208435776,1690.76695766623,1691.20183097455,1691.63670428272,1692.07157759075,
1692.50645089864,1692.94132420637,1693.37619751397,1693.81107082142,1694.24594412873,
1694.68167012916,1695.11739612959,1695.55226943662,1695.9871427435,1696.42201605025,
1696.85688935687,1697.29176266334,1697.72663596969,1698.1615092759,1698.59638258198,
1699.03125588793,1699.46612919375,1699.90100249945,1700.33587580502,1700.77074911047,
1701.20562241579,1701.64134841525,1702.0770744147,1702.51194771979,1702.94682102476,
1703.38169432963,1703.81656763438,1704.25144093902,1704.68631424356,1705.12118754799,
1705.55606085232,1705.99093415655,1706.42580746068,1706.86068076471,1707.29555406866,
1707.73042737251,1708.16530067627,1708.60102667496,1709.03675267365,1709.47162597724,
1709.90649928076,1710.34137258419,1710.77624588756,1711.21111919085,1711.64599249406,
1712.08086579722,1712.5157391003,1712.95061240333,1713.3854857063,1713.82035900921,
1714.25523231207,1714.69010561487,1715.12497891763,1715.56070491584,1715.99643091404,
1716.43130421671,1716.86617751935,1717.30105082195,1717.73592412451,1718.17079742705,
1718.60567072956,1719.04054403204,1719.4754173345,1719.91029063695,1720.34516393938,
1720.7800372418,1721.21491054421,1721.64978384661,1722.08465714901,1722.52038314706,
1722.9561091451,1723.39098244751,1723.82585574992,1724.26072905233,1724.69560235476,
1725.13047565721,1725.56534895967,1726.00022226216,1726.43509556467,1726.8699688672,
1727.30484216977,1727.73971547236,1728.174588775,1728.60946207767,1729.04433538039,
1729.48006137861,1729.91578737684,1730.35066067965,1730.78553398251,1731.22040728542,
1731.65528058838,1732.09015389141,1732.5250271945,1732.95990049765,1733.39477380087,
1733.82964710416,1734.26452040752,1734.69939371096,1735.13426701447,1735.56914031807,
1736.00401362175,1736.43973962048,1736.8754656192,1737.31033892306,1737.745212227,
1738.18008553104,1738.61495883517,1739.0498321394,1739.48470544373,1739.91957874816,
1740.35445205269,1740.78932535734,1741.22419866209,1741.65907196695,1742.09394527193,
1742.52881857702,1742.96369188223,1743.39941788174,1743.83514388125,1744.2700171867,
1744.70489049227,1745.13976379797,1745.57463710379,1746.00951040974,1746.44438371582,
1746.87925702203,1747.31413032837,1747.74900363485,1748.18387694146,1748.61875024821,
1749.0536235551,1749.48849686213,1749.92337016929,1750.3590961698,1750.7948221703,
1751.22969547775,1751.66456878534,1752.09944209308,1752.53431540096,1752.96918870899,
1753.40406201717,1753.83893532549,1754.27380863396,1754.70868194258,1755.14355525134,
1755.57842856026,1756.01330186932,1756.44817517853,1756.88304848789,1757.31877448949,
1757.75450049109,1758.18937380075,1759.05912042051,1759.49399373061,1759.92886704086,
1760.36374035125,1760.79861366179,1761.23348697248,1761.66836028331,1762.10323359429,
1762.5381069054,1763.40785352806,1763.8427268396,1764.27845284228,1764.71417884496,
1765.14905215677,1765.58392546872,1766.0187987808,1766.88854540534,1767.75829203039,
1768.1931653431,1768.62803865593,1769.06291196888,1769.49778528195,1770.36753190841,
1771.2381312254,1772.10873054259,1772.97847717007,1773.84822379791,1774.71797042609,
1775.58771705456,1776.45746368331,1777.32721031228,1778.19780963089,1779.06840894783,
1779.93815555508,1780.80790201176,1781.67764871408),.UNSPECIFIED.) ;
#918=FACE_OUTER_BOUND('',#1401,.T.) ;
#919=FACE_OUTER_BOUND('',#1402,.T.) ;
#920=FACE_OUTER_BOUND('',#1403,.T.) ;
#921=FACE_OUTER_BOUND('',#1404,.T.) ;
#922=FACE_OUTER_BOUND('',#1405,.T.) ;
#923=FACE_OUTER_BOUND('',#1406,.T.) ;
#924=FACE_OUTER_BOUND('',#1407,.T.) ;
#925=FACE_OUTER_BOUND('',#1408,.T.) ;
#926=FACE_OUTER_BOUND('',#1409,.T.) ;
#927=FACE_OUTER_BOUND('',#1410,.T.) ;
#928=FACE_OUTER_BOUND('',#1411,.T.) ;
#929=FACE_OUTER_BOUND('',#1413,.T.) ;
#930=FACE_OUTER_BOUND('',#1414,.T.) ;
#931=FACE_OUTER_BOUND('',#1415,.T.) ;
#932=FACE_OUTER_BOUND('',#1416,.T.) ;
#933=FACE_OUTER_BOUND('',#1417,.T.) ;
#934=FACE_OUTER_BOUND('',#1418,.T.) ;
#935=FACE_OUTER_BOUND('',#1419,.T.) ;
#1401=EDGE_LOOP('',(#5902,#5903,#5904,#5905)) ;
#1402=EDGE_LOOP('',(#5906,#5907,#5908,#5909)) ;
#1403=EDGE_LOOP('',(#5910,#5911,#5912,#5913)) ;
#1404=EDGE_LOOP('',(#5914,#5915,#5916,#5917)) ;
#1405=EDGE_LOOP('',(#5918,#5919,#5920,#5921)) ;
#1406=EDGE_LOOP('',(#5922,#5923,#5924)) ;
#1407=EDGE_LOOP('',(#5925,#5926,#5927,#5928,#5929,#5930,#5931)) ;
#1408=EDGE_LOOP('',(#5932,#5933,#5934,#5935,#5936,#5937,#5938,#5939,#5940)) ;
#1409=EDGE_LOOP('',(#5941,#5942,#5943,#5944,#5945,#5946,#5947,#5948,#5949)) ;
#1410=EDGE_LOOP('',(#5950,#5951,#5952,#5953,#5954,#5955,#5956)) ;
#1411=EDGE_LOOP('',(#5957)) ;
#1412=EDGE_LOOP('',(#5958,#5959,#5960,#5961,#5962,#5963)) ;
#1413=EDGE_LOOP('',(#5964,#5965,#5966,#5967)) ;
#1414=EDGE_LOOP('',(#5968,#5969,#5970,#5971)) ;
#1415=EDGE_LOOP('',(#5972,#5973,#5974,#5975)) ;
#1416=EDGE_LOOP('',(#5976,#5977,#5978,#5979)) ;
#1417=EDGE_LOOP('',(#5980,#5981,#5982,#5983)) ;
#1418=EDGE_LOOP('',(#5984,#5985,#5986,#5987)) ;
#1419=EDGE_LOOP('',(#5988,#5989,#5990,#5991,#5992,#5993)) ;
#1906=LINE('',#79316,#2609) ;
#1907=LINE('',#79633,#2610) ;
#1908=LINE('',#80089,#2611) ;
#1909=LINE('',#80536,#2612) ;
#1910=LINE('',#81518,#2613) ;
#1911=LINE('',#81591,#2614) ;
#1912=LINE('',#95701,#2615) ;
#1913=LINE('',#95705,#2616) ;
#1914=LINE('',#95707,#2617) ;
#1915=LINE('',#95709,#2618) ;
#1916=LINE('',#95711,#2619) ;
#1917=LINE('',#95713,#2620) ;
#1918=LINE('',#95714,#2621) ;
#1919=LINE('',#95717,#2622) ;
#1920=LINE('',#95719,#2623) ;
#1921=LINE('',#95720,#2624) ;
#1922=LINE('',#95723,#2625) ;
#1923=LINE('',#95724,#2626) ;
#1924=LINE('',#95727,#2627) ;
#1925=LINE('',#95728,#2628) ;
#1926=LINE('',#95731,#2629) ;
#1927=LINE('',#95732,#2630) ;
#1928=LINE('',#95735,#2631) ;
#1929=LINE('',#95736,#2632) ;
#1930=LINE('',#95738,#2633) ;
#2609=VECTOR('',#9618,1.21492629244945) ;
#2610=VECTOR('',#9623,1.21492629244945) ;
#2611=VECTOR('',#9626,1.21492629244945) ;
#2612=VECTOR('',#9629,1.21492629244945) ;
#2613=VECTOR('',#9636,0.119992720241923) ;
#2614=VECTOR('',#9641,0.239985440483837) ;
#2615=VECTOR('',#9646,0.199999999999989) ;
#2616=VECTOR('',#9649,10.) ;
#2617=VECTOR('',#9650,10.) ;
#2618=VECTOR('',#9651,10.) ;
#2619=VECTOR('',#9652,10.) ;
#2620=VECTOR('',#9653,10.) ;
#2621=VECTOR('',#9654,10.) ;
#2622=VECTOR('',#9657,10.) ;
#2623=VECTOR('',#9658,10.) ;
#2624=VECTOR('',#9659,10.) ;
#2625=VECTOR('',#9662,10.) ;
#2626=VECTOR('',#9663,10.) ;
#2627=VECTOR('',#9666,10.) ;
#2628=VECTOR('',#9667,10.) ;
#2629=VECTOR('',#9670,10.) ;
#2630=VECTOR('',#9671,10.) ;
#2631=VECTOR('',#9674,10.) ;
#2632=VECTOR('',#9675,10.) ;
#2633=VECTOR('',#9678,10.) ;
#3374=B_SPLINE_CURVE_WITH_KNOTS('',3,(#79318,#79319,#79320,#79321,#79322,
#79323,#79324,#79325,#79326,#79327,#79328,#79329,#79330,#79331,#79332,#79333,
#79334,#79335,#79336,#79337,#79338,#79339,#79340,#79341,#79342,#79343,#79344,
#79345,#79346,#79347,#79348,#79349,#79350,#79351,#79352,#79353,#79354,#79355,
#79356,#79357,#79358,#79359,#79360,#79361,#79362,#79363,#79364,#79365,#79366,
#79367,#79368,#79369,#79370,#79371,#79372,#79373,#79374,#79375,#79376,#79377,
#79378,#79379,#79380,#79381,#79382,#79383,#79384,#79385,#79386,#79387,#79388,
#79389,#79390,#79391,#79392,#79393,#79394,#79395,#79396,#79397,#79398,#79399,
#79400,#79401,#79402,#79403,#79404,#79405,#79406,#79407,#79408,#79409,#79410,
#79411,#79412,#79413,#79414,#79415,#79416,#79417,#79418,#79419,#79420,#79421,
#79422,#79423,#79424,#79425,#79426,#79427,#79428,#79429,#79430,#79431,#79432,
#79433,#79434,#79435,#79436,#79437,#79438,#79439,#79440,#79441,#79442,#79443,
#79444,#79445,#79446,#79447,#79448,#79449,#79450,#79451,#79452,#79453,#79454,
#79455,#79456,#79457,#79458,#79459,#79460,#79461,#79462,#79463,#79464,#79465,
#79466,#79467,#79468,#79469,#79470,#79471,#79472,#79473,#79474,#79475,#79476,
#79477,#79478,#79479,#79480,#79481,#79482,#79483,#79484,#79485),
 .UNSPECIFIED.,.F.,.F.,(4,2,2,2,2,2,2,2,2,2,2,2,2,2,2,2,2,2,2,2,2,2,2,2,
2,2,2,2,2,2,2,2,2,2,2,2,2,2,2,2,2,2,2,2,2,2,2,2,2,2,2,2,2,2,2,2,2,2,2,2,
2,2,2,2,2,2,2,2,2,2,2,2,2,2,2,2,2,2,2,2,2,2,2,4),(-0.220763983380471,-0.212810338743189,
-0.210826302908365,-0.209271007576308,-0.207760980376256,-0.205729488094328,
-0.198550181809563,-0.194693795352243,-0.191844661325702,-0.190288509145287,
-0.188362306697201,-0.184999537283139,-0.180416472909434,-0.177999557055194,
-0.176979917204659,-0.17545943341679,-0.169329841502711,-0.167326009010082,
-0.165010107168382,-0.163313661316864,-0.161023174884449,-0.15372738344787,
-0.149942801988463,-0.147940388957888,-0.146174507780922,-0.14492471603392,
-0.143254578734082,-0.139977364430561,-0.132761299778805,-0.129907182850962,
-0.12772776186146,-0.12769522261391,-0.127662280121649,-0.127628703111083,
-0.127594235626406,-0.127558587343492,-0.127521421133998,-0.127482336198394,
-0.125819004945782,-0.123790181619449,-0.118018980404149,-0.115257240279385,
-0.113532448213236,-0.112659152515239,-0.111622338612391,-0.110439445580995,
-0.105393490852793,-0.101142710955009,-0.0984836507689282,-0.0959423330614772,
-0.0924670231571394,-0.0856704509335571,-0.0830826422246745,-0.0810670415820549,
-0.0801905444928017,-0.0800237634118451,-0.0798508645920698,-0.0797151871859187,
-0.0796106920962894,-0.0765192041817014,-0.0724898724816029,-0.0649233609992019,
-0.0628333596238857,-0.0625221421103429,-0.0613894549744398,-0.0592211973507973,
-0.0578457591077455,-0.0536661847240215,-0.0503751810208162,-0.0488118397384947,
-0.0471863838408071,-0.0401191690844113,-0.036693088908186,-0.0347854974643231,
-0.0327365419518084,-0.0288818466209434,-0.0233041197359696,-0.0196358343583312,
-0.0180950601031717,-0.016951466256656,-0.0158400932091164,-0.0145364062440794,
-0.0126256867425368,-1.00000005442968E-6),.UNSPECIFIED.) ;
#3375=B_SPLINE_CURVE_WITH_KNOTS('',3,(#79488,#79489,#79490,#79491,#79492,
#79493,#79494,#79495,#79496,#79497,#79498,#79499,#79500,#79501,#79502,#79503,
#79504,#79505,#79506,#79507,#79508,#79509,#79510,#79511,#79512,#79513,#79514,
#79515,#79516,#79517,#79518,#79519,#79520,#79521,#79522,#79523,#79524,#79525,
#79526,#79527,#79528,#79529,#79530,#79531,#79532,#79533,#79534,#79535,#79536,
#79537,#79538,#79539,#79540,#79541,#79542,#79543,#79544,#79545,#79546,#79547,
#79548,#79549,#79550,#79551,#79552,#79553,#79554,#79555,#79556,#79557,#79558,
#79559,#79560,#79561,#79562,#79563,#79564,#79565,#79566,#79567,#79568,#79569,
#79570,#79571,#79572,#79573,#79574,#79575,#79576,#79577,#79578,#79579,#79580,
#79581,#79582,#79583,#79584,#79585,#79586,#79587,#79588,#79589,#79590,#79591,
#79592,#79593,#79594,#79595,#79596,#79597,#79598,#79599,#79600,#79601,#79602,
#79603,#79604,#79605,#79606,#79607,#79608,#79609,#79610,#79611,#79612,#79613,
#79614,#79615,#79616,#79617,#79618,#79619,#79620,#79621,#79622,#79623,#79624,
#79625,#79626,#79627,#79628,#79629),.UNSPECIFIED.,.F.,.F.,(4,2,2,2,2,2,
2,2,2,2,2,2,2,2,2,2,2,2,2,2,2,2,2,2,2,2,2,2,2,2,2,2,2,2,2,2,2,2,2,2,2,2,
2,2,2,2,2,2,2,2,2,2,2,2,2,2,2,2,2,2,2,2,2,2,2,2,2,2,2,2,4),(-0.18252474525029,
-0.179400066977439,-0.175252692305652,-0.169924729691008,-0.168066528920694,
-0.166743109385763,-0.165501096667492,-0.164280350194813,-0.162567505415626,
-0.153584789316722,-0.149881802737214,-0.148075117524774,-0.147659331879399,
-0.147475574264912,-0.147253803230242,-0.147096076826089,-0.146984500314822,
-0.146905539465106,-0.146333073448781,-0.145369009076629,-0.144414998280596,
-0.142823355979458,-0.1369286174308,-0.132413903090164,-0.129285936821479,
-0.127635850380881,-0.12651547712041,-0.125561653504244,-0.124579822074233,
-0.123247741481105,-0.120332181776785,-0.114069642881635,-0.11110441261796,
-0.108953824687521,-0.106802809676022,-0.104459564364395,-0.0976458556504293,
-0.0940738777335949,-0.0913404381349576,-0.0885028731082607,-0.0798366421232186,
-0.0769226509456521,-0.074379646873931,-0.0720421619700198,-0.0689755666210176,
-0.0630996412878632,-0.0613131008382774,-0.0599974512973652,-0.0595480234483862,
-0.0594019673736506,-0.0592683762327051,-0.0591333251245316,-0.0589867853784717,
-0.0588186846865954,-0.0586168250482456,-0.0583652072776119,-0.0566822399161281,
-0.0538546350878509,-0.0440464063710776,-0.04191636283755,-0.0403248468776896,
-0.0387643875176817,-0.0368436467110806,-0.0336193237703689,-0.025875309571662,
-0.0229828527660033,-0.0202624149178314,-0.0102148474703489,-0.00824309809122128,
-0.00659087878765106,-6.19471680093315E-6),.UNSPECIFIED.) ;
#3376=B_SPLINE_CURVE_WITH_KNOTS('',3,(#79634,#79635,#79636,#79637,#79638,
#79639,#79640,#79641,#79642,#79643,#79644,#79645,#79646,#79647,#79648,#79649,
#79650,#79651,#79652,#79653,#79654,#79655,#79656,#79657,#79658,#79659,#79660,
#79661,#79662,#79663,#79664,#79665,#79666,#79667,#79668,#79669,#79670,#79671,
#79672,#79673,#79674,#79675,#79676,#79677,#79678,#79679,#79680,#79681,#79682,
#79683,#79684,#79685,#79686,#79687,#79688,#79689,#79690,#79691,#79692,#79693,
#79694,#79695,#79696,#79697,#79698,#79699,#79700,#79701,#79702,#79703,#79704,
#79705,#79706,#79707,#79708,#79709,#79710,#79711,#79712,#79713,#79714,#79715,
#79716,#79717,#79718,#79719,#79720,#79721,#79722,#79723,#79724,#79725,#79726,
#79727,#79728,#79729,#79730,#79731,#79732,#79733,#79734,#79735,#79736,#79737,
#79738,#79739,#79740,#79741,#79742,#79743,#79744,#79745,#79746,#79747,#79748,
#79749,#79750,#79751,#79752,#79753,#79754,#79755,#79756,#79757,#79758,#79759,
#79760,#79761,#79762,#79763,#79764,#79765,#79766,#79767,#79768,#79769,#79770,
#79771,#79772,#79773,#79774,#79775,#79776,#79777,#79778,#79779,#79780,#79781,
#79782,#79783,#79784,#79785,#79786,#79787,#79788,#79789,#79790,#79791,#79792,
#79793,#79794,#79795,#79796,#79797,#79798,#79799,#79800,#79801,#79802,#79803,
#79804,#79805,#79806,#79807,#79808,#79809,#79810,#79811,#79812,#79813,#79814,
#79815,#79816,#79817,#79818,#79819,#79820,#79821,#79822,#79823,#79824,#79825,
#79826,#79827,#79828,#79829,#79830,#79831,#79832,#79833,#79834,#79835,#79836,
#79837,#79838,#79839,#79840,#79841,#79842,#79843,#79844,#79845,#79846,#79847,
#79848,#79849,#79850,#79851,#79852,#79853),.UNSPECIFIED.,.F.,.F.,(4,3,3,
3,3,3,3,3,3,3,3,3,3,3,3,3,3,3,3,3,3,3,3,3,3,3,3,3,3,3,3,3,3,3,3,3,3,3,3,
3,3,3,3,3,3,3,3,3,3,3,3,3,3,3,3,3,3,3,3,3,3,3,3,3,3,3,3,3,3,3,3,3,3,4),
(0.,0.114554107952554,0.219999579637262,0.40798083050021,0.571675274172504,
0.925887608273928,1.24364764883742,1.27682344199313,1.56513289539867,1.63103573085445,
1.92276380563121,1.98481039669498,2.30553261810542,2.33719940646081,2.68985168871465,
2.85597213219828,3.02278753371246,3.04298755913573,3.13367446983352,3.18807481875432,
3.3009537204216,3.39425414698803,3.57785099270887,3.7486975888156,4.10139086880436,
4.41302871221882,4.45537183311384,4.74928777620892,4.80732327925073,5.09839243438881,
5.16153555014084,5.47412129432304,5.51418781350788,5.86492791526386,6.04203405015412,
6.21914018504438,6.31436263900441,6.37615253991527,6.48557261069783,6.57181603734208,
6.75160383616011,6.92446829765038,7.27760414977274,7.59380314034735,7.6294205837199,
7.91857835915048,7.98363285125545,8.27582882629675,8.33593536794668,8.66001538388278,
8.6877517844213,9.04173195324679,9.21866661258249,9.39560127191819,9.49526269149975,
9.56422015730585,9.66918811922697,9.74731942042791,9.92430999212726,10.1013005638266,
10.4534629350241,10.7676564343516,10.8062607636447,11.0976054309995,11.1594970582837,
11.454185960616,11.5115370732495,11.8216297039995,11.8657493811883,12.2168162078705,
12.3939223660536,12.5710285242368,12.6749025971548,12.7522862024853),
 .UNSPECIFIED.) ;
#3377=B_SPLINE_CURVE_WITH_KNOTS('',3,(#79854,#79855,#79856,#79857,#79858,
#79859,#79860,#79861,#79862,#79863,#79864,#79865,#79866,#79867,#79868,#79869,
#79870,#79871,#79872,#79873,#79874,#79875,#79876,#79877,#79878,#79879,#79880,
#79881,#79882,#79883,#79884,#79885,#79886,#79887,#79888,#79889,#79890,#79891,
#79892,#79893,#79894,#79895,#79896,#79897,#79898,#79899,#79900,#79901,#79902,
#79903,#79904,#79905,#79906,#79907,#79908,#79909,#79910,#79911,#79912,#79913,
#79914,#79915,#79916,#79917,#79918,#79919,#79920,#79921,#79922,#79923,#79924,
#79925,#79926,#79927,#79928,#79929,#79930,#79931,#79932,#79933,#79934,#79935,
#79936,#79937,#79938,#79939,#79940,#79941,#79942,#79943,#79944,#79945,#79946,
#79947,#79948,#79949,#79950,#79951,#79952,#79953,#79954,#79955,#79956,#79957,
#79958,#79959,#79960,#79961,#79962,#79963,#79964,#79965,#79966,#79967,#79968,
#79969,#79970,#79971,#79972,#79973,#79974,#79975,#79976,#79977,#79978,#79979,
#79980,#79981,#79982,#79983,#79984,#79985,#79986,#79987,#79988,#79989,#79990,
#79991,#79992,#79993,#79994,#79995,#79996,#79997,#79998,#79999,#80000,#80001,
#80002,#80003,#80004,#80005,#80006,#80007,#80008,#80009,#80010,#80011,#80012,
#80013,#80014,#80015,#80016,#80017,#80018,#80019,#80020,#80021,#80022,#80023,
#80024,#80025,#80026,#80027,#80028,#80029,#80030,#80031,#80032,#80033,#80034,
#80035,#80036,#80037,#80038,#80039,#80040,#80041,#80042,#80043,#80044,#80045,
#80046,#80047,#80048,#80049,#80050,#80051,#80052,#80053,#80054,#80055,#80056,
#80057,#80058,#80059,#80060,#80061,#80062,#80063,#80064,#80065,#80066,#80067,
#80068,#80069,#80070,#80071,#80072,#80073,#80074,#80075,#80076,#80077,#80078,
#80079,#80080,#80081,#80082,#80083,#80084,#80085),.UNSPECIFIED.,.F.,.F.,
(4,3,3,3,3,3,3,3,3,3,3,3,3,3,3,3,3,3,3,3,3,3,3,3,3,3,3,3,3,3,3,3,3,3,3,
3,3,3,3,3,3,3,3,3,3,3,3,3,3,3,3,3,3,3,3,3,3,3,3,3,3,3,3,3,3,3,3,3,3,3,3,
3,3,3,3,3,3,4),(0.,0.0894148861877891,0.133889678145916,0.297921036677569,
0.461212171674198,0.484629898594515,0.837282234412057,1.15861202910842,
1.19149448755028,1.48838290165772,1.54321518660845,1.8334631648485,1.89765827078402,
2.20002485219279,2.25210099027431,2.60280642166565,2.79655675959504,2.95701869061026,
3.07760215573877,3.18808892718112,3.26981110624916,3.31092626983993,3.47259185576712,
3.633470010557,3.6613092422968,4.01460245905827,4.34133219129516,4.36881472280183,
4.66775371996431,4.71935092585698,5.00902512576176,5.07356320109738,5.375729168866,
5.42777545310502,5.77865470103715,5.97878115250132,6.13136950553454,6.25595693487507,
6.37618626099941,6.4513335487717,6.483550843245,6.64287768424873,6.80133273686597,
6.83734305486834,7.19132473436349,7.52405859388823,7.5426224094343,7.8336538016193,
7.89706722798282,8.18493486313129,8.25104693288396,8.56343455351041,8.6015832902021,
8.95491331887032,9.16001611295106,9.30912556946611,9.4367215799293,9.56431759039249,
9.63444066958202,9.65993050174436,9.81702320746632,9.97319560073537,10.012728542287,
10.3669408040578,10.7013854790574,10.719103527886,11.0117551593669,11.0733158373996,
11.3671781532315,11.4245578244276,11.7283639906824,11.7787701291327,12.1305869844538,
12.3455036127973,12.4828898638758,12.6089564690771,12.7358311186926,12.7524660495637),
 .UNSPECIFIED.) ;
#3378=B_SPLINE_CURVE_WITH_KNOTS('',3,(#80090,#80091,#80092,#80093,#80094,
#80095,#80096,#80097,#80098,#80099,#80100,#80101,#80102,#80103,#80104,#80105,
#80106,#80107,#80108,#80109,#80110,#80111,#80112,#80113,#80114,#80115,#80116,
#80117,#80118,#80119,#80120,#80121,#80122,#80123,#80124,#80125,#80126,#80127,
#80128,#80129,#80130,#80131,#80132,#80133,#80134,#80135,#80136,#80137,#80138,
#80139,#80140,#80141,#80142,#80143,#80144,#80145,#80146,#80147,#80148,#80149,
#80150,#80151,#80152,#80153,#80154,#80155,#80156,#80157,#80158,#80159,#80160,
#80161,#80162,#80163,#80164,#80165,#80166,#80167,#80168,#80169,#80170,#80171,
#80172,#80173,#80174,#80175,#80176,#80177,#80178,#80179,#80180,#80181,#80182,
#80183,#80184,#80185,#80186,#80187,#80188,#80189,#80190,#80191,#80192,#80193,
#80194,#80195,#80196,#80197,#80198,#80199,#80200,#80201,#80202,#80203,#80204,
#80205,#80206,#80207,#80208,#80209,#80210,#80211,#80212,#80213,#80214,#80215,
#80216,#80217,#80218,#80219,#80220,#80221,#80222,#80223,#80224,#80225,#80226,
#80227,#80228,#80229,#80230,#80231,#80232,#80233,#80234,#80235,#80236,#80237,
#80238,#80239,#80240,#80241,#80242,#80243,#80244,#80245,#80246,#80247,#80248,
#80249,#80250,#80251,#80252,#80253,#80254,#80255,#80256,#80257,#80258,#80259,
#80260,#80261,#80262,#80263,#80264,#80265,#80266,#80267,#80268,#80269,#80270,
#80271,#80272,#80273,#80274,#80275,#80276,#80277,#80278,#80279,#80280,#80281,
#80282,#80283,#80284,#80285,#80286,#80287,#80288,#80289,#80290,#80291,#80292,
#80293,#80294,#80295,#80296,#80297,#80298,#80299,#80300,#80301,#80302,#80303,
#80304,#80305,#80306,#80307,#80308,#80309,#80310,#80311,#80312),
 .UNSPECIFIED.,.F.,.F.,(4,3,3,3,3,3,3,3,3,3,3,3,3,3,3,3,3,3,3,3,3,3,3,3,
3,3,3,3,3,3,3,3,3,3,3,3,3,3,3,3,3,3,3,3,3,3,3,3,3,3,3,3,3,3,3,3,3,3,3,3,
3,3,3,3,3,3,3,3,3,3,3,3,3,3,4),(0.,0.100762857825756,0.17045455738185,0.347415762439074,
0.524376967496299,0.877381484509634,1.19821800653056,1.22826049812016,1.51697376328285,
1.58247279915011,1.87779658023047,1.93391776317192,2.25164505566527,2.28836068050304,
2.64280331320604,2.82167316119906,2.99350875161294,3.10266796924014,3.18807250430072,
3.28423663368526,3.34738831255791,3.5233640520366,3.69933979151529,4.05355206803615,
4.37985223749883,4.40620435589301,4.70171242540885,4.75694454204997,5.04601965453119,
5.11115683439866,5.42764767481781,5.46361882765795,5.81783110946781,6.00081498008659,
6.16978259404898,6.2828607180743,6.37613838180102,6.46714712814609,6.52211297837991,
6.68925611334493,6.85570174442494,6.87524886950579,7.22706540888955,7.5427802441183,
7.58104611352649,7.87520812138854,7.93428224769233,8.2234903967075,8.28872622840582,
8.59531361187601,8.64114684774855,8.99188712842038,9.18026879928742,9.34609939086034,
9.46276931651261,9.56422046408461,9.65091384739663,9.69916314071276,9.86319775131977,
10.0264998248966,10.0499034623499,10.4041157271119,10.7307046869009,10.7583279856935,
11.0558356759019,11.1095696963186,11.3979727180052,11.4637819917093,11.7745585768663,
11.8159445691956,12.1687425517332,12.3621786336217,12.5198069536285,12.6375810196589,
12.7523053453689),.UNSPECIFIED.) ;
#3379=B_SPLINE_CURVE_WITH_KNOTS('',3,(#80313,#80314,#80315,#80316,#80317,
#80318,#80319,#80320,#80321,#80322,#80323,#80324,#80325,#80326,#80327,#80328,
#80329,#80330,#80331,#80332,#80333,#80334,#80335,#80336,#80337,#80338,#80339,
#80340,#80341,#80342,#80343,#80344,#80345,#80346,#80347,#80348,#80349,#80350,
#80351,#80352,#80353,#80354,#80355,#80356,#80357,#80358,#80359,#80360,#80361,
#80362,#80363,#80364,#80365,#80366,#80367,#80368,#80369,#80370,#80371,#80372,
#80373,#80374,#80375,#80376,#80377,#80378,#80379,#80380,#80381,#80382,#80383,
#80384,#80385,#80386,#80387,#80388,#80389,#80390,#80391,#80392,#80393,#80394,
#80395,#80396,#80397,#80398,#80399,#80400,#80401,#80402,#80403,#80404,#80405,
#80406,#80407,#80408,#80409,#80410,#80411,#80412,#80413,#80414,#80415,#80416,
#80417,#80418,#80419,#80420,#80421,#80422,#80423,#80424,#80425,#80426,#80427,
#80428,#80429,#80430,#80431,#80432,#80433,#80434,#80435,#80436,#80437,#80438,
#80439,#80440,#80441,#80442,#80443,#80444,#80445,#80446,#80447,#80448,#80449,
#80450,#80451,#80452,#80453,#80454,#80455,#80456,#80457,#80458,#80459,#80460,
#80461,#80462,#80463,#80464,#80465,#80466,#80467,#80468,#80469,#80470,#80471,
#80472,#80473,#80474,#80475,#80476,#80477,#80478,#80479,#80480,#80481,#80482,
#80483,#80484,#80485,#80486,#80487,#80488,#80489,#80490,#80491,#80492,#80493,
#80494,#80495,#80496,#80497,#80498,#80499,#80500,#80501,#80502,#80503,#80504,
#80505,#80506,#80507,#80508,#80509,#80510,#80511,#80512,#80513,#80514,#80515,
#80516,#80517,#80518,#80519,#80520,#80521,#80522,#80523,#80524,#80525,#80526,
#80527,#80528,#80529,#80530,#80531,#80532),.UNSPECIFIED.,.F.,.F.,(4,3,3,
3,3,3,3,3,3,3,3,3,3,3,3,3,3,3,3,3,3,3,3,3,3,3,3,3,3,3,3,3,3,3,3,3,3,3,3,
3,3,3,3,3,3,3,3,3,3,3,3,3,3,3,3,3,3,3,3,3,3,3,3,3,3,3,3,3,3,3,3,3,3,4),
(0.,0.103893003810878,0.181262498396716,0.358368655155245,0.535474811913774,
0.886541640300103,1.19673532348644,1.24075395493171,1.53528792411396,1.59279396171985,
1.88431414393547,1.94603026773208,2.25997509560389,2.29882808755841,2.65099046906085,
2.82798104483141,3.00497162060198,3.10991086391462,3.18806738078836,3.28775562074012,
3.35668976127941,3.5336244263954,3.71055909151139,4.06453925695613,4.38847961223419,
4.41635566929646,4.70870697419377,4.76865819735123,5.05774592416977,5.12287046168214,
5.43899161304988,5.47468689392592,5.82782275374672,6.00761036936649,6.18047500641398,
6.28988375072362,6.37613695915723,6.4713735827455,6.53315086103547,6.71025699441627,
6.88736312779706,7.23810322232236,7.55101366328478,7.59075550121641,7.88163753031553,
7.94496776270377,8.23896747477361,8.29691921461726,8.60855780948375,8.65090019138673,
9.00359345967117,9.18722179851666,9.35803689449882,9.47088359281189,9.56421233698863,
9.65492998924632,9.70930349363768,9.87612791713462,10.0422522333714,10.0624393716107,
10.4150916485022,10.7357912645928,10.7674806581858,11.0593569652461,11.1212553350823,
11.409386398908,11.4754676140256,11.7933709583769,11.826403454723,12.180615789613,
12.3685389651704,12.5322914820512,12.6468674178292,12.7522978599647),
 .UNSPECIFIED.) ;
#3380=B_SPLINE_CURVE_WITH_KNOTS('',3,(#80537,#80538,#80539,#80540,#80541,
#80542,#80543,#80544,#80545,#80546,#80547,#80548,#80549,#80550,#80551,#80552,
#80553,#80554,#80555,#80556,#80557,#80558,#80559,#80560,#80561,#80562,#80563,
#80564,#80565,#80566,#80567,#80568,#80569,#80570,#80571,#80572,#80573,#80574,
#80575,#80576,#80577,#80578,#80579,#80580,#80581,#80582,#80583,#80584,#80585,
#80586,#80587,#80588,#80589,#80590,#80591,#80592,#80593,#80594,#80595,#80596,
#80597,#80598,#80599,#80600,#80601,#80602,#80603,#80604,#80605,#80606,#80607,
#80608,#80609,#80610,#80611,#80612,#80613,#80614,#80615,#80616,#80617,#80618,
#80619,#80620,#80621,#80622,#80623,#80624,#80625,#80626,#80627,#80628,#80629,
#80630,#80631,#80632,#80633,#80634,#80635,#80636,#80637,#80638,#80639,#80640,
#80641,#80642,#80643,#80644,#80645,#80646,#80647,#80648,#80649,#80650,#80651,
#80652,#80653,#80654,#80655,#80656,#80657,#80658,#80659,#80660,#80661,#80662,
#80663,#80664,#80665,#80666,#80667,#80668,#80669,#80670,#80671,#80672,#80673,
#80674,#80675,#80676,#80677,#80678,#80679,#80680,#80681,#80682,#80683,#80684,
#80685,#80686,#80687,#80688,#80689,#80690,#80691,#80692,#80693,#80694,#80695,
#80696,#80697,#80698,#80699,#80700,#80701,#80702,#80703,#80704,#80705,#80706,
#80707,#80708,#80709,#80710,#80711,#80712,#80713,#80714,#80715,#80716,#80717,
#80718,#80719,#80720,#80721,#80722,#80723,#80724,#80725,#80726,#80727,#80728,
#80729,#80730,#80731,#80732,#80733,#80734,#80735,#80736,#80737,#80738,#80739,
#80740,#80741,#80742,#80743,#80744,#80745,#80746,#80747,#80748,#80749,#80750,
#80751,#80752,#80753,#80754,#80755,#80756,#80757,#80758,#80759,#80760,#80761,
#80762,#80763,#80764,#80765),.UNSPECIFIED.,.F.,.F.,(4,3,3,3,3,3,3,3,3,3,
3,3,3,3,3,3,3,3,3,3,3,3,3,3,3,3,3,3,3,3,3,3,3,3,3,3,3,3,3,3,3,3,3,3,3,3,
3,3,3,3,3,3,3,3,3,3,3,3,3,3,3,3,3,3,3,3,3,3,3,3,3,3,3,3,3,3,4),(0.,0.0849567058115355,
0.121410866737072,0.283571067642219,0.444919421038145,0.475392252089173,
0.827665187221835,1.14808607613794,1.18210927518942,1.47839116596738,1.53459228457289,
1.82885507160418,1.88547168452342,2.19314502783543,2.23968397375804,2.59214615040927,
2.79038879486852,2.94635842870424,3.06998802803527,3.18810817019483,3.26440590431521,
3.29802675005529,3.45757822076252,3.61627514247094,3.65067925900212,4.00489154138233,
4.35563223002435,4.64617975589709,4.70984452935805,5.00046832574839,5.06284926268752,
5.36685554190499,5.41550181494416,5.76624256865231,5.97273593786443,6.1202225757179,
6.24822644256217,6.37623030940644,6.44733815583808,6.47439716292745,6.63221404230345,
6.78911562829056,6.82800759658552,7.18091231497168,7.51065136477143,7.53272928162441,
7.82487629705489,7.88694158774125,8.18083977413766,8.23818376656191,8.54281082978249,
8.59239607694621,8.94455897340147,9.1575282370111,9.2973571803608,9.4308647738549,
9.564372367349,9.62916114633184,9.64818402988998,9.80361159264067,9.95805838375808,
10.002396297147,10.3566085447957,10.5648455268548,10.7090424934517,10.9238830828392,
11.1385418510569,11.3532131814733,11.4174022576871,11.6640729394278,11.7698515234467,
12.1227348772726,12.3436966068405,12.4771776993501,12.6049451701728,12.7335676446473,
12.7552103037919),.UNSPECIFIED.) ;
#3381=B_SPLINE_CURVE_WITH_KNOTS('',3,(#80766,#80767,#80768,#80769,#80770,
#80771,#80772,#80773,#80774,#80775,#80776,#80777,#80778,#80779,#80780,#80781,
#80782,#80783,#80784,#80785,#80786,#80787,#80788,#80789,#80790,#80791,#80792,
#80793,#80794,#80795,#80796,#80797,#80798,#80799,#80800,#80801,#80802,#80803,
#80804,#80805,#80806,#80807,#80808,#80809,#80810,#80811,#80812,#80813,#80814,
#80815,#80816,#80817,#80818,#80819,#80820,#80821,#80822,#80823,#80824,#80825,
#80826,#80827,#80828,#80829,#80830,#80831,#80832,#80833,#80834,#80835,#80836,
#80837,#80838,#80839,#80840,#80841,#80842,#80843,#80844,#80845,#80846,#80847,
#80848,#80849,#80850,#80851,#80852,#80853,#80854,#80855,#80856,#80857,#80858,
#80859,#80860,#80861,#80862,#80863,#80864,#80865,#80866,#80867,#80868,#80869,
#80870,#80871,#80872,#80873,#80874,#80875,#80876,#80877,#80878,#80879,#80880,
#80881,#80882,#80883,#80884,#80885,#80886,#80887,#80888,#80889,#80890,#80891,
#80892,#80893,#80894,#80895,#80896,#80897,#80898,#80899,#80900,#80901,#80902,
#80903,#80904,#80905,#80906,#80907,#80908,#80909,#80910,#80911,#80912,#80913,
#80914,#80915,#80916,#80917,#80918,#80919,#80920,#80921,#80922,#80923,#80924,
#80925,#80926,#80927,#80928,#80929,#80930,#80931,#80932,#80933,#80934,#80935,
#80936,#80937,#80938,#80939,#80940,#80941,#80942,#80943,#80944,#80945,#80946,
#80947,#80948,#80949,#80950,#80951,#80952,#80953,#80954,#80955,#80956,#80957,
#80958,#80959,#80960,#80961,#80962,#80963,#80964,#80965,#80966,#80967,#80968,
#80969,#80970,#80971,#80972,#80973,#80974,#80975,#80976,#80977,#80978,#80979,
#80980,#80981,#80982,#80983,#80984,#80985,#80986,#80987,#80988),
 .UNSPECIFIED.,.F.,.F.,(4,3,3,3,3,3,3,3,3,3,3,3,3,3,3,3,3,3,3,3,3,3,3,3,
3,3,3,3,3,3,3,3,3,3,3,3,3,3,3,3,3,3,3,3,3,3,3,3,3,3,3,3,3,3,3,3,3,3,3,3,
3,3,3,3,3,3,3,3,3,3,3,3,3,3,4),(0.,0.117766852480119,0.232496353538427,
0.425959269805488,0.58356076372737,0.936358747455187,1.24721516299566,1.28852133052573,
1.57691037403893,1.64273362456121,1.94009683856486,1.99397533075514,2.32101174159844,
2.34818760451099,2.70239985630971,2.86567318626521,3.02967152715542,3.05314018006163,
3.13984623840259,3.18808443459044,3.30474613545493,3.40620393305099,3.59458496913141,
3.76041618591283,4.11115646630507,4.4179620031712,4.46357709690046,4.75264568629906,
4.81802107035101,5.11225950860045,5.17125721849527,5.48698227134708,5.525237914481,
5.87705445117265,6.04348549182013,6.21060943622194,6.23019035170545,6.32120249042149,
6.37616561501542,6.4892370938465,6.58252073706138,6.76552124705007,6.93447223265948,
7.2886845102342,7.60525585812541,7.64114650722471,7.93025277521774,7.99535880099052,
8.29066722847324,8.34609897805127,8.67287428691527,8.69875128326739,9.05296354724675,
9.22893929137685,9.40491503550695,9.50113431130131,9.56423800268766,9.67334187672587,
9.75879459828048,9.93770082835329,10.109500019499,10.4639426784075,10.7812408318919,
10.8183855714955,11.1138898609533,11.1698305545815,11.4585507849351,11.5240428555817,
11.8445810390484,11.8749218597236,12.2279263926025,12.4048875910266,12.5818487894507,
12.6825950545204,12.7522985291244),.UNSPECIFIED.) ;
#3382=B_SPLINE_CURVE_WITH_KNOTS('',3,(#80991,#80992,#80993,#80994,#80995,
#80996,#80997,#80998,#80999,#81000,#81001,#81002,#81003,#81004,#81005,#81006,
#81007,#81008,#81009,#81010,#81011,#81012,#81013,#81014,#81015,#81016,#81017,
#81018,#81019,#81020,#81021,#81022,#81023,#81024,#81025,#81026,#81027,#81028,
#81029,#81030,#81031,#81032,#81033,#81034,#81035,#81036,#81037,#81038,#81039,
#81040,#81041,#81042,#81043,#81044,#81045,#81046,#81047,#81048,#81049,#81050,
#81051,#81052,#81053,#81054,#81055,#81056,#81057,#81058,#81059,#81060,#81061,
#81062,#81063,#81064,#81065,#81066,#81067,#81068,#81069,#81070,#81071,#81072,
#81073,#81074,#81075,#81076,#81077,#81078,#81079,#81080,#81081,#81082,#81083,
#81084,#81085,#81086,#81087,#81088,#81089,#81090,#81091,#81092,#81093,#81094,
#81095,#81096,#81097,#81098,#81099,#81100,#81101,#81102,#81103,#81104,#81105,
#81106,#81107,#81108,#81109,#81110,#81111,#81112,#81113,#81114,#81115,#81116,
#81117,#81118,#81119,#81120,#81121,#81122,#81123,#81124,#81125,#81126,#81127,
#81128,#81129,#81130,#81131,#81132,#81133,#81134,#81135,#81136,#81137,#81138,
#81139,#81140,#81141,#81142,#81143,#81144,#81145,#81146,#81147,#81148,#81149,
#81150,#81151,#81152,#81153,#81154,#81155,#81156,#81157,#81158,#81159,#81160,
#81161,#81162,#81163,#81164,#81165,#81166,#81167,#81168,#81169,#81170,#81171,
#81172,#81173,#81174,#81175,#81176,#81177,#81178,#81179,#81180,#81181,#81182,
#81183,#81184,#81185,#81186,#81187,#81188,#81189,#81190,#81191,#81192,#81193,
#81194,#81195,#81196,#81197,#81198,#81199,#81200,#81201,#81202,#81203,#81204,
#81205,#81206,#81207,#81208,#81209,#81210,#81211,#81212,#81213,#81214,#81215,
#81216,#81217,#81218,#81219,#81220,#81221,#81222,#81223,#81224,#81225,#81226,
#81227,#81228,#81229,#81230,#81231,#81232,#81233,#81234,#81235,#81236,#81237,
#81238,#81239,#81240,#81241,#81242,#81243,#81244,#81245,#81246,#81247,#81248,
#81249,#81250,#81251,#81252,#81253,#81254,#81255,#81256,#81257,#81258,#81259,
#81260,#81261,#81262,#81263,#81264,#81265,#81266,#81267,#81268,#81269,#81270,
#81271,#81272,#81273,#81274,#81275,#81276,#81277,#81278,#81279,#81280,#81281,
#81282,#81283,#81284,#81285,#81286,#81287,#81288,#81289,#81290),
 .UNSPECIFIED.,.F.,.F.,(4,2,2,2,2,2,2,2,2,2,2,2,2,2,2,2,2,2,2,2,2,2,2,2,
2,2,2,2,2,2,2,2,2,2,2,2,2,2,2,2,2,2,2,2,2,2,2,2,2,2,2,2,2,2,2,2,2,2,2,2,
2,2,2,2,2,2,2,2,2,2,2,2,2,2,2,2,2,2,2,2,2,2,2,2,2,2,2,2,2,2,2,2,2,2,2,2,
2,2,2,2,2,2,2,2,2,2,2,2,2,2,2,2,2,2,2,2,2,2,2,2,2,2,2,2,2,2,2,2,2,2,2,2,
2,2,2,2,2,2,2,2,2,2,2,2,2,2,2,2,2,4),(-0.257894959744042,-0.253220611148935,
-0.252082519774515,-0.251189207858128,-0.2502706763012,-0.249204820691145,
-0.24734086125322,-0.238825211955683,-0.234956710782849,-0.232265582687393,
-0.232163656503359,-0.232079890411829,-0.232009429589355,-0.23194885477312,
-0.23189570103474,-0.231848145732546,-0.231804802747511,-0.231764583881055,
-0.231726602097676,-0.231690100812442,-0.231654398403906,-0.23161884023568,
-0.230646507521808,-0.229652146135218,-0.2283254697423,-0.225431560706624,
-0.219432808035315,-0.215918365425081,-0.213951525208257,-0.211667593912582,
-0.211297017030229,-0.210798316724895,-0.210069641212601,-0.209184079408535,
-0.20233480803109,-0.199071711636883,-0.196674826367858,-0.192673413721236,
-0.188338844281775,-0.185309143004634,-0.183063435515454,-0.180463010870351,
-0.172247574976944,-0.169227557805637,-0.166969106489589,-0.165718950597125,
-0.164550297675546,-0.162998755449737,-0.159450634129076,-0.151301404921013,
-0.148434861925196,-0.146764543296957,-0.145289493301241,-0.144420952767203,
-0.143261735333598,-0.141671941428281,-0.136953553242676,-0.134633536768281,
-0.129065614489829,-0.12586894668411,-0.124659009655095,-0.123667875186939,
-0.122712953941796,-0.122706902779335,-0.122700817345473,-0.122694696393175,
-0.122688538768037,-0.122682343223882,-0.122676108667069,-0.122669833751837,
-0.122663517479823,-0.122657158550683,-0.122650755298769,-0.122644306826007,
-0.122637811485778,-0.12263126801403,-0.122624675086352,-0.122618031304535,
-0.122611335124305,-0.122604585099646,-0.122597779832967,-0.122590917682396,
-0.122583997138402,-0.122577016970953,-0.122569975346635,-0.122562870404742,
-0.122555700497586,-0.122548464327288,-0.12254116008541,-0.122533785780757,
-0.122526339564397,-0.12251881963144,-0.122511223909231,-0.122503550667778,
-0.122495797889482,-0.122487963729255,-0.122480045927489,-0.122472042536743,
-0.122463951294876,-0.122455769992845,-0.122447496191321,-0.122439127884568,
-0.122430662619054,-0.1224220978723,-0.122413431228693,-0.121283105168391,
-0.119557604757718,-0.116062880165473,-0.107074205096058,-0.105202142314451,
-0.103854487638451,-0.102970526354438,-0.102907177308501,-0.102857423197713,
-0.101281612623738,-0.0993316703532008,-0.0956795824111655,-0.0888309643124724,
-0.0861370748464511,-0.0859955520258133,-0.0832106391533367,-0.0773048156889599,
-0.0731571830179152,-0.0730096294887505,-0.0728620764216494,-0.0727002874126334,
-0.0725018367868773,-0.0721447246476089,-0.0707043294314262,-0.0691077557991271,
-0.0654637854118928,-0.0610601613559754,-0.0589585948592443,-0.0572180043633603,
-0.0567189271384514,-0.0545935015097311,-0.0477781729190308,-0.0424783830991959,
-0.0401182720840394,-0.0381028158238574,-0.0355564513823461,-0.032173028311343,
-0.0238920353908075,-0.0211071460799632,-0.0181412510164185,-0.0145766045458494,
-0.00910418362044593,-0.00751977868442608,-0.00619932980695214,-1.00000002645206E-6),
 .UNSPECIFIED.) ;
#3383=B_SPLINE_CURVE_WITH_KNOTS('',3,(#81293,#81294,#81295,#81296,#81297,
#81298,#81299,#81300,#81301,#81302,#81303,#81304,#81305,#81306,#81307,#81308,
#81309,#81310,#81311,#81312,#81313,#81314,#81315,#81316,#81317,#81318,#81319,
#81320,#81321,#81322,#81323,#81324,#81325,#81326,#81327,#81328,#81329,#81330,
#81331,#81332,#81333,#81334,#81335,#81336,#81337,#81338,#81339,#81340,#81341,
#81342,#81343,#81344,#81345,#81346,#81347,#81348,#81349,#81350,#81351,#81352,
#81353,#81354,#81355,#81356,#81357,#81358,#81359,#81360,#81361,#81362,#81363,
#81364,#81365,#81366,#81367,#81368,#81369,#81370,#81371,#81372,#81373,#81374,
#81375,#81376,#81377,#81378,#81379,#81380,#81381,#81382,#81383,#81384,#81385,
#81386,#81387,#81388,#81389,#81390,#81391,#81392,#81393,#81394,#81395,#81396,
#81397,#81398,#81399,#81400,#81401,#81402,#81403,#81404,#81405,#81406,#81407,
#81408,#81409,#81410,#81411,#81412,#81413,#81414,#81415,#81416,#81417,#81418,
#81419,#81420,#81421,#81422,#81423,#81424,#81425,#81426,#81427,#81428,#81429,
#81430,#81431,#81432,#81433,#81434,#81435,#81436,#81437,#81438,#81439,#81440,
#81441,#81442,#81443,#81444,#81445,#81446,#81447,#81448,#81449,#81450,#81451,
#81452,#81453,#81454,#81455,#81456,#81457,#81458,#81459,#81460,#81461,#81462,
#81463,#81464,#81465,#81466,#81467,#81468,#81469,#81470,#81471,#81472,#81473,
#81474,#81475,#81476,#81477,#81478,#81479,#81480,#81481,#81482,#81483,#81484,
#81485,#81486,#81487,#81488,#81489,#81490,#81491,#81492,#81493,#81494,#81495,
#81496,#81497,#81498,#81499,#81500,#81501,#81502,#81503,#81504,#81505,#81506,
#81507,#81508,#81509,#81510,#81511,#81512,#81513,#81514),.UNSPECIFIED.,
 .F.,.F.,(4,2,2,2,2,2,2,2,2,2,2,2,2,2,2,2,2,2,2,2,2,2,2,2,2,2,2,2,2,2,2,
2,2,2,2,2,2,2,2,2,2,2,2,2,2,2,2,2,2,2,2,2,2,2,2,2,2,2,2,2,2,2,2,2,2,2,2,
2,2,2,2,2,2,2,2,2,2,2,2,2,2,2,2,2,2,2,2,2,2,2,2,2,2,2,2,2,2,2,2,2,2,2,2,
2,2,2,2,2,2,2,4),(-0.21974730496944,-0.209497995751659,-0.207816227696814,
-0.206696348350822,-0.205767284698091,-0.20485397757947,-0.203644123970965,
-0.201163237535781,-0.199234334828623,-0.198913491876631,-0.192586005200389,
-0.188020363992073,-0.186092144364173,-0.185276519404618,-0.18332163303194,
-0.180721422658237,-0.173766453776646,-0.167938864952367,-0.166365261811103,
-0.163770327311883,-0.162358826389358,-0.160690850220444,-0.158448304110901,
-0.15228425029622,-0.144121818826867,-0.140893235816109,-0.138947282236318,
-0.138865006212637,-0.138785648892571,-0.138708812553493,-0.13863412632672,
-0.138561240968116,-0.138489823995273,-0.138419554947308,-0.138350120526013,
-0.138281209859491,-0.138212509414666,-0.138143697486611,-0.138074437950374,
-0.138004373215554,-0.137933115704807,-0.137860237518485,-0.137835732211627,
-0.136432771655794,-0.135030470253392,-0.133174489972427,-0.127354264807073,
-0.118311869408989,-0.114833620138255,-0.112062908143053,-0.111005128554945,
-0.110976089279789,-0.110945776024287,-0.110914132197716,-0.110881098781024,
-0.110846614335611,-0.110827740276134,-0.110804551101557,-0.110776089351518,
-0.11074120029057,-0.110698498801103,-0.110646335319223,-0.110582763233192,
-0.110521525369985,-0.110345951017164,-0.109869688106184,-0.108311784083106,
-0.10827868299426,-0.10824520687847,-0.10821132013487,-0.108176986417272,
-0.108142168373755,-0.108106827535724,-0.108070924329374,-0.108034417795035,
-0.10799726554041,-0.107959423681245,-0.107920846522564,-0.107881486501138,
-0.107841294113589,-0.10780021763837,-0.107758203039857,-0.107715193781533,
-0.104792570233929,-0.100834668518422,-0.0917717565902828,-0.0882811157453522,
-0.0867437366547149,-0.0853447743443662,-0.0838272385342882,-0.0790014398889958,
-0.0692014603300877,-0.0663858360611473,-0.0620178835475202,-0.0533675339317639,
-0.0502666772550644,-0.0473136918819925,-0.0441141213159802,-0.0372988874541403,
-0.0353544452877392,-0.0341090803360572,-0.0338991174967524,-0.032528273487166,
-0.030619718825037,-0.0274728686588918,-0.0176254071723615,-0.0155915957491533,
-0.0140813196430058,-0.0126105676500786,-0.0108387771806254,-5.22571535866158E-5),
 .UNSPECIFIED.) ;
#3384=B_SPLINE_CURVE_WITH_KNOTS('',3,(#81522,#81523,#81524,#81525,#81526,
#81527,#81528,#81529,#81530,#81531,#81532,#81533,#81534,#81535,#81536,#81537,
#81538,#81539,#81540,#81541,#81542,#81543,#81544,#81545,#81546,#81547),
 .UNSPECIFIED.,.F.,.F.,(4,2,2,2,2,2,2,2,2,2,2,2,4),(9.99999996900801E-7,
0.0217536568115777,0.0435354891955391,0.0879397153262638,0.112564023697292,
0.137318935333563,0.162458662654742,0.187567234819558,0.213124132495112,
0.238695964082357,0.264191632957232,0.29041955787013,0.311836241868587),
 .UNSPECIFIED.) ;
#3385=B_SPLINE_CURVE_WITH_KNOTS('',3,(#81549,#81550,#81551,#81552,#81553,
#81554,#81555,#81556),.UNSPECIFIED.,.F.,.F.,(4,2,2,4),(0.,0.0328258807040897,
0.0479820964185046,0.0625119124690952),.UNSPECIFIED.) ;
#3386=B_SPLINE_CURVE_WITH_KNOTS('',3,(#81557,#81558,#81559,#81560,#81561,
#81562,#81563,#81564,#81565,#81566,#81567,#81568,#81569,#81570,#81571,#81572,
#81573,#81574,#81575,#81576,#81577,#81578,#81579,#81580,#81581,#81582,#81583,
#81584,#81585,#81586,#81587,#81588,#81589,#81590),.UNSPECIFIED.,.F.,.F.,
(4,2,2,2,2,2,2,2,2,2,2,2,2,2,2,2,4),(0.311836241868587,0.316507424623957,
0.342892888009964,0.369492419893424,0.396264677446643,0.409779859619715,
0.436779117207306,0.464022317104011,0.491926865768048,0.519205487048488,
0.547669956804294,0.575175692029193,0.603824409330207,0.632256986799627,
0.689732978983562,0.718666448865442,0.747725957477036),.UNSPECIFIED.) ;
#3387=B_SPLINE_CURVE_WITH_KNOTS('',3,(#88563,#88564,#88565,#88566,#88567,
#88568,#88569,#88570,#88571,#88572,#88573,#88574,#88575,#88576,#88577,#88578,
#88579,#88580,#88581,#88582,#88583,#88584,#88585,#88586,#88587,#88588,#88589,
#88590,#88591,#88592,#88593,#88594,#88595,#88596,#88597,#88598,#88599,#88600,
#88601,#88602,#88603,#88604,#88605,#88606,#88607,#88608,#88609,#88610,#88611,
#88612,#88613,#88614,#88615,#88616,#88617,#88618,#88619,#88620,#88621,#88622,
#88623,#88624,#88625,#88626,#88627,#88628,#88629,#88630,#88631,#88632,#88633,
#88634,#88635,#88636,#88637,#88638,#88639,#88640,#88641,#88642,#88643,#88644,
#88645,#88646,#88647,#88648,#88649,#88650,#88651,#88652,#88653,#88654,#88655,
#88656,#88657,#88658,#88659,#88660,#88661,#88662,#88663,#88664,#88665,#88666),
 .UNSPECIFIED.,.F.,.F.,(4,1,1,1,1,1,1,1,1,1,1,1,1,1,1,1,1,1,1,1,1,1,1,1,
1,1,1,1,1,1,1,1,1,1,1,1,1,1,1,1,1,1,1,1,1,1,1,1,1,1,1,1,1,1,1,1,1,1,1,1,
1,1,1,1,1,1,1,1,1,1,1,1,1,1,1,1,1,1,1,1,1,1,1,1,1,1,1,1,1,1,1,1,1,1,1,1,
1,1,1,1,1,4),(32.7489697872148,33.0588984658616,33.4937717726112,33.928645079224,
34.3635183857014,34.7983916920448,35.2332649982556,35.6681383043353,36.1030116102854,
36.5378849161076,36.9727582218035,37.4076315273749,37.8425048328235,38.2782308323341,
38.7139568318446,39.1488301370532,39.5837034421446,40.0185767471208,40.4534500519838,
40.8883233567357,41.3231966613787,41.7580699659148,42.1929432703463,42.6278165746754,
43.0626898789044,43.4975631830356,43.9324364870714,44.3673097910142,44.8021830948664,
45.2379090935952,45.673635092324,46.1085083960024,46.5433816995978,46.9782550031127,
47.4131283065497,47.8480016099115,48.2828749132006,48.7177482164198,49.1526215195718,
49.5874948226593,50.0223681256851,50.457241428652,50.8921147315628,51.3269880344203,
51.7618613372274,52.197587335454,52.6333133336805,53.0681866363954,53.5030599390685,
53.9379332417027,54.3728065443011,54.8076798468664,55.2425531494018,55.6774264519101,
56.1122997543943,56.5471730568575,56.9820463593026,57.4169196617326,57.8517929641506,
58.2866662665595,58.7215395689624,59.157265567009,59.5929915650557,60.0278648674556,
60.4627381698584,60.8976114722673,61.3324847746853,61.7673580771153,62.2022313795604,
62.6371046820236,63.0719779845079,63.5068512870162,63.9417245895516,64.376597892117,
64.8114711947155,65.2463444973499,65.6812178000231,66.1169437982275,66.5526697964318,
66.9875430991915,67.4224164019987,67.8572897048563,68.2921630077673,68.7270363107343,
69.1619096137603,69.5967829168479,70.0316562200001,70.4665295232194,70.9014028265087,
71.3362761298705,71.7711494333077,72.2060227368227,72.6408960404182,73.0766220391044,
73.5123480377905,73.9472213415547,74.382094645407,74.8169679493499,75.2518412533859,
75.6867145575172,76.1215878617464,76.5237606401499),.UNSPECIFIED.) ;
#3388=B_SPLINE_CURVE_WITH_KNOTS('',3,(#88667,#88668,#88669,#88670,#88671,
#88672,#88673,#88674,#88675,#88676),.UNSPECIFIED.,.F.,.F.,(4,2,2,2,4),(-0.0826694635875258,
-0.0593216231105862,-0.0376236853894878,-0.0193344026424728,0.),
 .UNSPECIFIED.) ;
#3389=B_SPLINE_CURVE_WITH_KNOTS('',3,(#95648,#95649,#95650,#95651,#95652,
#95653,#95654,#95655,#95656,#95657),.UNSPECIFIED.,.F.,.F.,(4,2,2,2,4),(1.00000014359794E-6,
0.0360372518640473,0.0809925104139904,0.121401369748062,0.142937500220573),
 .UNSPECIFIED.) ;
#3390=B_SPLINE_CURVE_WITH_KNOTS('',3,(#95658,#95659,#95660,#95661,#95662,
#95663,#95664,#95665,#95666,#95667,#95668,#95669,#95670,#95671,#95672,#95673,
#95674,#95675,#95676,#95677,#95678,#95679,#95680,#95681,#95682,#95683,#95684,
#95685,#95686,#95687,#95688,#95689,#95690,#95691,#95692,#95693,#95694,#95695,
#95696,#95697),.UNSPECIFIED.,.F.,.F.,(4,2,2,2,2,2,2,2,2,2,2,2,2,2,2,2,2,
2,2,4),(0.142937500220573,0.212621082019458,0.320815840090966,0.375504796790274,
0.430559656121251,0.485436696366515,0.542481778298955,0.598023802517587,
0.655309402277618,0.713243686022327,0.770798519845424,0.886328666912018,
0.944969358407582,1.06329674263614,1.1820699816098,1.24254840068009,1.30316653563122,
1.40054089198694,1.44934143852683,1.49830020415347),.UNSPECIFIED.) ;
#3561=VERTEX_POINT('',#79314) ;
#3562=VERTEX_POINT('',#79315) ;
#3563=VERTEX_POINT('',#79317) ;
#3564=VERTEX_POINT('',#79486) ;
#3565=VERTEX_POINT('',#79631) ;
#3566=VERTEX_POINT('',#79632) ;
#3567=VERTEX_POINT('',#80087) ;
#3568=VERTEX_POINT('',#80088) ;
#3569=VERTEX_POINT('',#80534) ;
#3570=VERTEX_POINT('',#80535) ;
#3571=VERTEX_POINT('',#80990) ;
#3572=VERTEX_POINT('',#81291) ;
#3573=VERTEX_POINT('',#81516) ;
#3574=VERTEX_POINT('',#81517) ;
#3575=VERTEX_POINT('',#81521) ;
#3576=VERTEX_POINT('',#81548) ;
#3577=VERTEX_POINT('',#88562) ;
#3578=VERTEX_POINT('',#95647) ;
#3579=VERTEX_POINT('',#95699) ;
#3580=VERTEX_POINT('',#95703) ;
#3581=VERTEX_POINT('',#95704) ;
#3582=VERTEX_POINT('',#95706) ;
#3583=VERTEX_POINT('',#95708) ;
#3584=VERTEX_POINT('',#95710) ;
#3585=VERTEX_POINT('',#95712) ;
#3586=VERTEX_POINT('',#95716) ;
#3587=VERTEX_POINT('',#95718) ;
#3588=VERTEX_POINT('',#95722) ;
#3589=VERTEX_POINT('',#95726) ;
#3590=VERTEX_POINT('',#95730) ;
#3591=VERTEX_POINT('',#95734) ;
#4459=EDGE_CURVE('',#3561,#3562,#1906,.T.) ;
#4460=EDGE_CURVE('',#3563,#3561,#3374,.T.) ;
#4461=EDGE_CURVE('',#3563,#3564,#631,.T.) ;
#4462=EDGE_CURVE('',#3562,#3564,#3375,.T.) ;
#4463=EDGE_CURVE('',#3565,#3566,#1907,.T.) ;
#4464=EDGE_CURVE('',#3561,#3565,#3376,.T.) ;
#4465=EDGE_CURVE('',#3566,#3562,#3377,.T.) ;
#4466=EDGE_CURVE('',#3567,#3568,#1908,.T.) ;
#4467=EDGE_CURVE('',#3565,#3567,#3378,.T.) ;
#4468=EDGE_CURVE('',#3568,#3566,#3379,.T.) ;
#4469=EDGE_CURVE('',#3569,#3570,#1909,.T.) ;
#4470=EDGE_CURVE('',#3567,#3569,#3380,.T.) ;
#4471=EDGE_CURVE('',#3570,#3568,#3381,.T.) ;
#4472=EDGE_CURVE('',#3571,#3570,#3382,.T.) ;
#4473=EDGE_CURVE('',#3572,#3571,#632,.T.) ;
#4474=EDGE_CURVE('',#3569,#3572,#3383,.T.) ;
#4475=EDGE_CURVE('',#3573,#3574,#1910,.T.) ;
#4476=EDGE_CURVE('',#3574,#3574,#633,.T.) ;
#4477=EDGE_CURVE('',#3572,#3575,#3384,.T.) ;
#4478=EDGE_CURVE('',#3576,#3571,#3385,.T.) ;
#4479=EDGE_CURVE('',#3575,#3576,#3386,.T.) ;
#4480=EDGE_CURVE('',#3575,#3574,#1911,.T.) ;
#4481=EDGE_CURVE('',#3576,#3577,#3387,.T.) ;
#4482=EDGE_CURVE('',#3563,#3577,#3388,.T.) ;
#4483=EDGE_CURVE('',#3578,#3564,#3389,.F.) ;
#4484=EDGE_CURVE('',#3577,#3578,#3390,.F.) ;
#4485=EDGE_CURVE('',#3579,#3579,#634,.T.) ;
#4486=EDGE_CURVE('',#3579,#3578,#1912,.T.) ;
#4487=EDGE_CURVE('',#3580,#3581,#1913,.T.) ;
#4488=EDGE_CURVE('',#3581,#3582,#1914,.T.) ;
#4489=EDGE_CURVE('',#3582,#3583,#1915,.T.) ;
#4490=EDGE_CURVE('',#3583,#3584,#1916,.T.) ;
#4491=EDGE_CURVE('',#3584,#3585,#1917,.T.) ;
#4492=EDGE_CURVE('',#3585,#3580,#1918,.T.) ;
#4493=EDGE_CURVE('',#3580,#3586,#1919,.T.) ;
#4494=EDGE_CURVE('',#3586,#3587,#1920,.T.) ;
#4495=EDGE_CURVE('',#3581,#3587,#1921,.T.) ;
#4496=EDGE_CURVE('',#3587,#3588,#1922,.T.) ;
#4497=EDGE_CURVE('',#3582,#3588,#1923,.T.) ;
#4498=EDGE_CURVE('',#3588,#3589,#1924,.T.) ;
#4499=EDGE_CURVE('',#3583,#3589,#1925,.T.) ;
#4500=EDGE_CURVE('',#3589,#3590,#1926,.T.) ;
#4501=EDGE_CURVE('',#3584,#3590,#1927,.T.) ;
#4502=EDGE_CURVE('',#3590,#3591,#1928,.T.) ;
#4503=EDGE_CURVE('',#3585,#3591,#1929,.T.) ;
#4504=EDGE_CURVE('',#3591,#3586,#1930,.T.) ;
#5902=ORIENTED_EDGE('',*,*,#4459,.F.) ;
#5903=ORIENTED_EDGE('',*,*,#4460,.F.) ;
#5904=ORIENTED_EDGE('',*,*,#4461,.T.) ;
#5905=ORIENTED_EDGE('',*,*,#4462,.F.) ;
#5906=ORIENTED_EDGE('',*,*,#4463,.F.) ;
#5907=ORIENTED_EDGE('',*,*,#4464,.F.) ;
#5908=ORIENTED_EDGE('',*,*,#4459,.T.) ;
#5909=ORIENTED_EDGE('',*,*,#4465,.F.) ;
#5910=ORIENTED_EDGE('',*,*,#4466,.F.) ;
#5911=ORIENTED_EDGE('',*,*,#4467,.F.) ;
#5912=ORIENTED_EDGE('',*,*,#4463,.T.) ;
#5913=ORIENTED_EDGE('',*,*,#4468,.F.) ;
#5914=ORIENTED_EDGE('',*,*,#4469,.F.) ;
#5915=ORIENTED_EDGE('',*,*,#4470,.F.) ;
#5916=ORIENTED_EDGE('',*,*,#4466,.T.) ;
#5917=ORIENTED_EDGE('',*,*,#4471,.F.) ;
#5918=ORIENTED_EDGE('',*,*,#4469,.T.) ;
#5919=ORIENTED_EDGE('',*,*,#4472,.F.) ;
#5920=ORIENTED_EDGE('',*,*,#4473,.F.) ;
#5921=ORIENTED_EDGE('',*,*,#4474,.F.) ;
#5922=ORIENTED_EDGE('',*,*,#4475,.T.) ;
#5923=ORIENTED_EDGE('',*,*,#4476,.T.) ;
#5924=ORIENTED_EDGE('',*,*,#4475,.F.) ;
#5925=ORIENTED_EDGE('',*,*,#4477,.F.) ;
#5926=ORIENTED_EDGE('',*,*,#4473,.T.) ;
#5927=ORIENTED_EDGE('',*,*,#4478,.F.) ;
#5928=ORIENTED_EDGE('',*,*,#4479,.F.) ;
#5929=ORIENTED_EDGE('',*,*,#4480,.T.) ;
#5930=ORIENTED_EDGE('',*,*,#4476,.F.) ;
#5931=ORIENTED_EDGE('',*,*,#4480,.F.) ;
#5932=ORIENTED_EDGE('',*,*,#4460,.T.) ;
#5933=ORIENTED_EDGE('',*,*,#4464,.T.) ;
#5934=ORIENTED_EDGE('',*,*,#4467,.T.) ;
#5935=ORIENTED_EDGE('',*,*,#4470,.T.) ;
#5936=ORIENTED_EDGE('',*,*,#4474,.T.) ;
#5937=ORIENTED_EDGE('',*,*,#4477,.T.) ;
#5938=ORIENTED_EDGE('',*,*,#4479,.T.) ;
#5939=ORIENTED_EDGE('',*,*,#4481,.T.) ;
#5940=ORIENTED_EDGE('',*,*,#4482,.F.) ;
#5941=ORIENTED_EDGE('',*,*,#4481,.F.) ;
#5942=ORIENTED_EDGE('',*,*,#4478,.T.) ;
#5943=ORIENTED_EDGE('',*,*,#4472,.T.) ;
#5944=ORIENTED_EDGE('',*,*,#4471,.T.) ;
#5945=ORIENTED_EDGE('',*,*,#4468,.T.) ;
#5946=ORIENTED_EDGE('',*,*,#4465,.T.) ;
#5947=ORIENTED_EDGE('',*,*,#4462,.T.) ;
#5948=ORIENTED_EDGE('',*,*,#4483,.F.) ;
#5949=ORIENTED_EDGE('',*,*,#4484,.F.) ;
#5950=ORIENTED_EDGE('',*,*,#4485,.F.) ;
#5951=ORIENTED_EDGE('',*,*,#4486,.T.) ;
#5952=ORIENTED_EDGE('',*,*,#4483,.T.) ;
#5953=ORIENTED_EDGE('',*,*,#4461,.F.) ;
#5954=ORIENTED_EDGE('',*,*,#4482,.T.) ;
#5955=ORIENTED_EDGE('',*,*,#4484,.T.) ;
#5956=ORIENTED_EDGE('',*,*,#4486,.F.) ;
#5957=ORIENTED_EDGE('',*,*,#4485,.T.) ;
#5958=ORIENTED_EDGE('',*,*,#4487,.T.) ;
#5959=ORIENTED_EDGE('',*,*,#4488,.T.) ;
#5960=ORIENTED_EDGE('',*,*,#4489,.T.) ;
#5961=ORIENTED_EDGE('',*,*,#4490,.T.) ;
#5962=ORIENTED_EDGE('',*,*,#4491,.T.) ;
#5963=ORIENTED_EDGE('',*,*,#4492,.T.) ;
#5964=ORIENTED_EDGE('',*,*,#4493,.T.) ;
#5965=ORIENTED_EDGE('',*,*,#4494,.T.) ;
#5966=ORIENTED_EDGE('',*,*,#4495,.F.) ;
#5967=ORIENTED_EDGE('',*,*,#4487,.F.) ;
#5968=ORIENTED_EDGE('',*,*,#4495,.T.) ;
#5969=ORIENTED_EDGE('',*,*,#4496,.T.) ;
#5970=ORIENTED_EDGE('',*,*,#4497,.F.) ;
#5971=ORIENTED_EDGE('',*,*,#4488,.F.) ;
#5972=ORIENTED_EDGE('',*,*,#4497,.T.) ;
#5973=ORIENTED_EDGE('',*,*,#4498,.T.) ;
#5974=ORIENTED_EDGE('',*,*,#4499,.F.) ;
#5975=ORIENTED_EDGE('',*,*,#4489,.F.) ;
#5976=ORIENTED_EDGE('',*,*,#4499,.T.) ;
#5977=ORIENTED_EDGE('',*,*,#4500,.T.) ;
#5978=ORIENTED_EDGE('',*,*,#4501,.F.) ;
#5979=ORIENTED_EDGE('',*,*,#4490,.F.) ;
#5980=ORIENTED_EDGE('',*,*,#4501,.T.) ;
#5981=ORIENTED_EDGE('',*,*,#4502,.T.) ;
#5982=ORIENTED_EDGE('',*,*,#4503,.F.) ;
#5983=ORIENTED_EDGE('',*,*,#4491,.F.) ;
#5984=ORIENTED_EDGE('',*,*,#4503,.T.) ;
#5985=ORIENTED_EDGE('',*,*,#4504,.T.) ;
#5986=ORIENTED_EDGE('',*,*,#4493,.F.) ;
#5987=ORIENTED_EDGE('',*,*,#4492,.F.) ;
#5988=ORIENTED_EDGE('',*,*,#4504,.F.) ;
#5989=ORIENTED_EDGE('',*,*,#4502,.F.) ;
#5990=ORIENTED_EDGE('',*,*,#4500,.F.) ;
#5991=ORIENTED_EDGE('',*,*,#4498,.F.) ;
#5992=ORIENTED_EDGE('',*,*,#4496,.F.) ;
#5993=ORIENTED_EDGE('',*,*,#4494,.F.) ;
#8144=CYLINDRICAL_SURFACE('',#8805,1.21492629244945) ;
#8145=CYLINDRICAL_SURFACE('',#8807,1.21492629244945) ;
#8146=CYLINDRICAL_SURFACE('',#8808,1.21492629244945) ;
#8147=CYLINDRICAL_SURFACE('',#8809,1.21492629244945) ;
#8148=CYLINDRICAL_SURFACE('',#8810,1.21492629244945) ;
#8301=ADVANCED_FACE('',(#918),#8144,.T.) ;
#8302=ADVANCED_FACE('',(#919),#8145,.T.) ;
#8303=ADVANCED_FACE('',(#920),#8146,.T.) ;
#8304=ADVANCED_FACE('',(#921),#8147,.T.) ;
#8305=ADVANCED_FACE('',(#922),#8148,.T.) ;
#8306=ADVANCED_FACE('',(#923),#313,.F.) ;
#8307=ADVANCED_FACE('',(#924),#314,.T.) ;
#8308=ADVANCED_FACE('',(#925),#832,.T.) ;
#8309=ADVANCED_FACE('',(#926),#833,.T.) ;
#8310=ADVANCED_FACE('',(#927),#315,.T.) ;
#8311=ADVANCED_FACE('',(#928,#564),#369,.T.) ;
#8312=ADVANCED_FACE('',(#929),#370,.T.) ;
#8313=ADVANCED_FACE('',(#930),#371,.T.) ;
#8314=ADVANCED_FACE('',(#931),#372,.T.) ;
#8315=ADVANCED_FACE('',(#932),#373,.T.) ;
#8316=ADVANCED_FACE('',(#933),#374,.T.) ;
#8317=ADVANCED_FACE('',(#934),#375,.T.) ;
#8318=ADVANCED_FACE('',(#935),#376,.T.) ;
#8719=CLOSED_SHELL('',(#8301,#8302,#8303,#8304,#8305,#8306,#8307,#8308,
#8309,#8310,#8311,#8312,#8313,#8314,#8315,#8316,#8317,#8318)) ;
#8805=AXIS2_PLACEMENT_3D('',#79313,#9616,#9617) ;
#8806=AXIS2_PLACEMENT_3D('',#79487,#9619,#9620) ;
#8807=AXIS2_PLACEMENT_3D('',#79630,#9621,#9622) ;
#8808=AXIS2_PLACEMENT_3D('',#80086,#9624,#9625) ;
#8809=AXIS2_PLACEMENT_3D('',#80533,#9627,#9628) ;
#8810=AXIS2_PLACEMENT_3D('',#80989,#9630,#9631) ;
#8811=AXIS2_PLACEMENT_3D('',#81292,#9632,#9633) ;
#8812=AXIS2_PLACEMENT_3D('',#81515,#9634,#9635) ;
#8813=AXIS2_PLACEMENT_3D('',#81519,#9637,#9638) ;
#8814=AXIS2_PLACEMENT_3D('',#81520,#9639,#9640) ;
#8815=AXIS2_PLACEMENT_3D('',#95698,#9642,#9643) ;
#8816=AXIS2_PLACEMENT_3D('',#95700,#9644,#9645) ;
#8817=AXIS2_PLACEMENT_3D('',#95702,#9647,#9648) ;
#8818=AXIS2_PLACEMENT_3D('',#95715,#9655,#9656) ;
#8819=AXIS2_PLACEMENT_3D('',#95721,#9660,#9661) ;
#8820=AXIS2_PLACEMENT_3D('',#95725,#9664,#9665) ;
#8821=AXIS2_PLACEMENT_3D('',#95729,#9668,#9669) ;
#8822=AXIS2_PLACEMENT_3D('',#95733,#9672,#9673) ;
#8823=AXIS2_PLACEMENT_3D('',#95737,#9676,#9677) ;
#8824=AXIS2_PLACEMENT_3D('',#95739,#9679,#9680) ;
#9616=DIRECTION('center_axis',(0.,-1.,0.)) ;
#9617=DIRECTION('ref_axis',(-0.946101641249535,0.,-0.323869857234253)) ;
#9618=DIRECTION('',(0.,1.,0.)) ;
#9619=DIRECTION('center_axis',(3.75494695140922E-9,-1.,-3.24758869446514E-8)) ;
#9620=DIRECTION('ref_axis',(0.389434122263594,3.1374361622722E-8,-0.921054322185605)) ;
#9621=DIRECTION('center_axis',(0.,-1.,0.)) ;
#9622=DIRECTION('ref_axis',(-0.946101641249535,0.,-0.323869857234253)) ;
#9623=DIRECTION('',(0.,1.,0.)) ;
#9624=DIRECTION('center_axis',(0.,-1.,0.)) ;
#9625=DIRECTION('ref_axis',(-0.946101641249535,0.,-0.323869857234253)) ;
#9626=DIRECTION('',(0.,1.,0.)) ;
#9627=DIRECTION('center_axis',(0.,-1.,0.)) ;
#9628=DIRECTION('ref_axis',(-0.946101641249535,0.,-0.323869857234253)) ;
#9629=DIRECTION('',(0.,1.,0.)) ;
#9630=DIRECTION('center_axis',(0.,-1.,0.)) ;
#9631=DIRECTION('ref_axis',(-0.946101641249535,0.,-0.323869857234253)) ;
#9632=DIRECTION('center_axis',(0.,-1.,0.)) ;
#9633=DIRECTION('ref_axis',(-0.946101641249535,0.,-0.323869857234253)) ;
#9634=DIRECTION('center_axis',(-2.38472166595684E-16,-1.,-1.12237188351893E-14)) ;
#9635=DIRECTION('ref_axis',(-0.958165701602871,-2.98389028785182E-15,0.286214060227441)) ;
#9636=DIRECTION('',(0.85700945699712,-0.447213595499954,-0.255997637913916)) ;
#9637=DIRECTION('center_axis',(-1.89537453127107E-15,-1.,-3.74799467464299E-17)) ;
#9638=DIRECTION('ref_axis',(-0.95816570160281,0.,0.286214060227646)) ;
#9639=DIRECTION('center_axis',(-1.05069562641528E-15,1.,-5.42645984197838E-15)) ;
#9640=DIRECTION('ref_axis',(-0.958165701602825,5.46388591979422E-16,0.286214060227598)) ;
#9641=DIRECTION('',(-0.857009456997078,-0.447213595499957,0.255997637914053)) ;
#9642=DIRECTION('center_axis',(-1.00269417211326E-16,-1.,-1.95454945674237E-15)) ;
#9643=DIRECTION('ref_axis',(-0.95816570160282,-4.63344819438314E-16,0.286214060227614)) ;
#9644=DIRECTION('center_axis',(1.81627551085956E-15,1.,1.3519073427862E-15)) ;
#9645=DIRECTION('ref_axis',(-0.58175859519622,2.21012228981213E-15,-0.813361504446406)) ;
#9646=DIRECTION('',(0.857009456997073,-0.447213595499959,-0.255997637914066)) ;
#9647=DIRECTION('center_axis',(0.,1.,0.)) ;
#9648=DIRECTION('ref_axis',(0.,0.,1.)) ;
#9649=DIRECTION('',(0.946101641249534,0.,0.323869857234258)) ;
#9650=DIRECTION('',(0.192571296739865,0.,0.981282984501376)) ;
#9651=DIRECTION('',(-0.753530344509659,0.,0.657413127267136)) ;
#9652=DIRECTION('',(-0.946101641249533,0.,-0.323869857234258)) ;
#9653=DIRECTION('',(-0.192571296739865,0.,-0.981282984501376)) ;
#9654=DIRECTION('',(0.753530344509681,0.,-0.65741312726711)) ;
#9655=DIRECTION('center_axis',(-0.323869857234258,0.,0.946101641249534)) ;
#9656=DIRECTION('ref_axis',(0.946101641249534,0.,0.323869857234258)) ;
#9657=DIRECTION('',(0.,-1.,0.)) ;
#9658=DIRECTION('',(0.946101641249534,0.,0.323869857234258)) ;
#9659=DIRECTION('',(0.,-1.,0.)) ;
#9660=DIRECTION('center_axis',(-0.981282984501376,0.,0.192571296739865)) ;
#9661=DIRECTION('ref_axis',(0.192571296739865,0.,0.981282984501376)) ;
#9662=DIRECTION('',(0.192571296739865,0.,0.981282984501376)) ;
#9663=DIRECTION('',(0.,-1.,0.)) ;
#9664=DIRECTION('center_axis',(-0.657413127267136,0.,-0.753530344509659)) ;
#9665=DIRECTION('ref_axis',(-0.753530344509659,0.,0.657413127267136)) ;
#9666=DIRECTION('',(-0.753530344509659,0.,0.657413127267136)) ;
#9667=DIRECTION('',(0.,-1.,0.)) ;
#9668=DIRECTION('center_axis',(0.323869857234259,0.,-0.946101641249534)) ;
#9669=DIRECTION('ref_axis',(-0.946101641249533,0.,-0.323869857234259)) ;
#9670=DIRECTION('',(-0.946101641249533,0.,-0.323869857234258)) ;
#9671=DIRECTION('',(0.,-1.,0.)) ;
#9672=DIRECTION('center_axis',(0.981282984501376,0.,-0.192571296739865)) ;
#9673=DIRECTION('ref_axis',(-0.192571296739865,0.,-0.981282984501376)) ;
#9674=DIRECTION('',(-0.192571296739865,0.,-0.981282984501376)) ;
#9675=DIRECTION('',(0.,-1.,0.)) ;
#9676=DIRECTION('center_axis',(0.65741312726711,0.,0.753530344509681)) ;
#9677=DIRECTION('ref_axis',(0.753530344509681,0.,-0.65741312726711)) ;
#9678=DIRECTION('',(0.753530344509681,0.,-0.65741312726711)) ;
#9679=DIRECTION('center_axis',(0.,1.,0.)) ;
#9680=DIRECTION('ref_axis',(0.,0.,1.)) ;
#79313=CARTESIAN_POINT('Origin',(-19.4092696390626,-30.19753203383,123.411833654984)) ;
#79314=CARTESIAN_POINT('',(-18.259825879779,13.5907660201144,123.80531165987)) ;
#79315=CARTESIAN_POINT('',(-18.259825879779,13.6088050314641,123.80531165987)) ;
#79316=CARTESIAN_POINT('',(-18.259825879779,-30.19753203383,123.80531165987)) ;
#79317=CARTESIAN_POINT('',(-19.3053878987246,13.6947924674767,122.201356690909)) ;
#79318=CARTESIAN_POINT('Ctrl Pts',(-19.3053878987355,13.694792467579,122.201356691093)) ;
#79319=CARTESIAN_POINT('Ctrl Pts',(-19.2790015565985,13.6935493748007,122.203621136616)) ;
#79320=CARTESIAN_POINT('Ctrl Pts',(-19.2527011620726,13.6923108864917,122.206747112924)) ;
#79321=CARTESIAN_POINT('Ctrl Pts',(-19.2199880841637,13.6907569978569,122.211724480067)) ;
#79322=CARTESIAN_POINT('Ctrl Pts',(-19.2134652193957,13.6904465142337,122.212771451581)) ;
#79323=CARTESIAN_POINT('Ctrl Pts',(-19.2018448836823,13.6898920627905,122.214733957618)) ;
#79324=CARTESIAN_POINT('Ctrl Pts',(-19.1967441127338,13.6896482264073,122.215628983934)) ;
#79325=CARTESIAN_POINT('Ctrl Pts',(-19.1867026363573,13.6891672331473,122.217457204583)) ;
#79326=CARTESIAN_POINT('Ctrl Pts',(-19.1817616917867,13.6889300932055,122.218388511836)) ;
#79327=CARTESIAN_POINT('Ctrl Pts',(-19.170187435375,13.6883734502378,122.220644606035)) ;
#79328=CARTESIAN_POINT('Ctrl Pts',(-19.1635591325312,13.6880537931767,122.221994171274)) ;
#79329=CARTESIAN_POINT('Ctrl Pts',(-19.1335591030364,13.6866029476454,122.228363745616)) ;
#79330=CARTESIAN_POINT('Ctrl Pts',(-19.110327483493,13.6854677830628,122.234017497673)) ;
#79331=CARTESIAN_POINT('Ctrl Pts',(-19.0748968568967,13.6837233529636,122.243755912942)) ;
#79332=CARTESIAN_POINT('Ctrl Pts',(-19.0625704385601,13.6831141537349,122.247355044169)) ;
#79333=CARTESIAN_POINT('Ctrl Pts',(-19.0412403253723,13.6820565260515,122.253951832279)) ;
#79334=CARTESIAN_POINT('Ctrl Pts',(-19.0322104100108,13.6816076912566,122.2568608285)) ;
#79335=CARTESIAN_POINT('Ctrl Pts',(-19.0183025659665,13.6809146446045,122.261521744582)) ;
#79336=CARTESIAN_POINT('Ctrl Pts',(-19.0134002434702,13.6806700133047,122.263199611754)) ;
#79337=CARTESIAN_POINT('Ctrl Pts',(-19.0024541715424,13.680122974838,122.2670244107)) ;
#79338=CARTESIAN_POINT('Ctrl Pts',(-18.9964163838097,13.6798206715914,122.269187944209)) ;
#79339=CARTESIAN_POINT('Ctrl Pts',(-18.9798855947754,13.6789912693134,122.275259587945)) ;
#79340=CARTESIAN_POINT('Ctrl Pts',(-18.9694290404278,13.6784647192872,122.279265106809)) ;
#79341=CARTESIAN_POINT('Ctrl Pts',(-18.9448557167229,13.6772214310784,122.28906988723)) ;
#79342=CARTESIAN_POINT('Ctrl Pts',(-18.930789934561,13.676505161048,122.294991705033)) ;
#79343=CARTESIAN_POINT('Ctrl Pts',(-18.9094825532098,13.6754097066074,122.304438726192)) ;
#79344=CARTESIAN_POINT('Ctrl Pts',(-18.9021582627929,13.6750312228838,122.307773552056)) ;
#79345=CARTESIAN_POINT('Ctrl Pts',(-18.8917919371076,13.6744922007744,122.312618366463)) ;
#79346=CARTESIAN_POINT('Ctrl Pts',(-18.8887222491793,13.6743321618287,122.314068726864)) ;
#79347=CARTESIAN_POINT('Ctrl Pts',(-18.8810902940327,13.673933144125,122.317713868788)) ;
#79348=CARTESIAN_POINT('Ctrl Pts',(-18.8765356006337,13.6736940262475,122.319924331301)) ;
#79349=CARTESIAN_POINT('Ctrl Pts',(-18.8536896123915,13.6724900149245,122.331188813133)) ;
#79350=CARTESIAN_POINT('Ctrl Pts',(-18.8356147093884,13.6715227048952,122.340674254182)) ;
#79351=CARTESIAN_POINT('Ctrl Pts',(-18.811959369325,13.6702410508436,122.353858771432)) ;
#79352=CARTESIAN_POINT('Ctrl Pts',(-18.8061582505,13.6699254410493,122.357154999757)) ;
#79353=CARTESIAN_POINT('Ctrl Pts',(-18.7937117196621,13.6692455629943,122.364363461565)) ;
#79354=CARTESIAN_POINT('Ctrl Pts',(-18.7870757996362,13.6688813880778,122.368291521219)) ;
#79355=CARTESIAN_POINT('Ctrl Pts',(-18.7756444743745,13.6682511221836,122.37520597176)) ;
#79356=CARTESIAN_POINT('Ctrl Pts',(-18.7708316770778,13.6679848572748,122.378163121457)) ;
#79357=CARTESIAN_POINT('Ctrl Pts',(-18.7595696537421,13.6673596131151,122.385191560434)) ;
#79358=CARTESIAN_POINT('Ctrl Pts',(-18.7531377884541,13.6670008331259,122.38929022978)) ;
#79359=CARTESIAN_POINT('Ctrl Pts',(-18.7263820034781,13.6655008841968,122.406696592065)) ;
#79360=CARTESIAN_POINT('Ctrl Pts',(-18.7064210224811,13.6643642512426,122.420551724848)) ;
#79361=CARTESIAN_POINT('Ctrl Pts',(-18.6767567000718,13.6626373161165,122.442488778044)) ;
#79362=CARTESIAN_POINT('Ctrl Pts',(-18.6667418496699,13.6620472269139,122.45013870501)) ;
#79363=CARTESIAN_POINT('Ctrl Pts',(-18.6516129483,13.6611432125891,122.462072269252)) ;
#79364=CARTESIAN_POINT('Ctrl Pts',(-18.6464121468389,13.6608301163655,122.466244528018)) ;
#79365=CARTESIAN_POINT('Ctrl Pts',(-18.6366900289319,13.6602402178117,122.47417635375)) ;
#79366=CARTESIAN_POINT('Ctrl Pts',(-18.6321611485509,13.659963505509,122.477926345771)) ;
#79367=CARTESIAN_POINT('Ctrl Pts',(-18.6244737906184,13.6594904298314,122.484386249689)) ;
#79368=CARTESIAN_POINT('Ctrl Pts',(-18.621301684346,13.6592942226465,122.487079787436)) ;
#79369=CARTESIAN_POINT('Ctrl Pts',(-18.6139230797762,13.658835460276,122.493410728789)) ;
#79370=CARTESIAN_POINT('Ctrl Pts',(-18.6097275973186,13.6585727898024,122.497060817645)) ;
#79371=CARTESIAN_POINT('Ctrl Pts',(-18.5973742601353,13.6577939240769,122.507958187457)) ;
#79372=CARTESIAN_POINT('Ctrl Pts',(-18.5892888471,13.6572770052471,122.515286686829)) ;
#79373=CARTESIAN_POINT('Ctrl Pts',(-18.5637199521017,13.6556195581763,122.539097206545)) ;
#79374=CARTESIAN_POINT('Ctrl Pts',(-18.5466262454901,13.654476487476,122.555989302032)) ;
#79375=CARTESIAN_POINT('Ctrl Pts',(-18.523486285956,13.6528853022747,122.580254400298)) ;
#79376=CARTESIAN_POINT('Ctrl Pts',(-18.5170087993465,13.652434788866,122.587208406547)) ;
#79377=CARTESIAN_POINT('Ctrl Pts',(-18.505730095759,13.6516413298043,122.599605331651)) ;
#79378=CARTESIAN_POINT('Ctrl Pts',(-18.5008948212632,13.6512981445459,122.605016608537)) ;
#79379=CARTESIAN_POINT('Ctrl Pts',(-18.4960368415869,13.6509502176703,122.61055232771)) ;
#79380=CARTESIAN_POINT('Ctrl Pts',(-18.4959653887577,13.6509450995473,122.610633770936)) ;
#79381=CARTESIAN_POINT('Ctrl Pts',(-18.4958216195361,13.650934800045,122.610797685917)) ;
#79382=CARTESIAN_POINT('Ctrl Pts',(-18.4957493034679,13.6509296186715,122.61088015785)) ;
#79383=CARTESIAN_POINT('Ctrl Pts',(-18.4956033009723,13.6509191562993,122.61104671002)) ;
#79384=CARTESIAN_POINT('Ctrl Pts',(-18.4955296150436,13.6509138753085,122.611130790565)) ;
#79385=CARTESIAN_POINT('Ctrl Pts',(-18.4953803125252,13.6509031734559,122.611301202115)) ;
#79386=CARTESIAN_POINT('Ctrl Pts',(-18.4953046965139,13.6508977525956,122.61138753372)) ;
#79387=CARTESIAN_POINT('Ctrl Pts',(-18.495150898894,13.6508867253586,122.611563176305)) ;
#79388=CARTESIAN_POINT('Ctrl Pts',(-18.4950727181454,13.650881118989,122.611652488023)) ;
#79389=CARTESIAN_POINT('Ctrl Pts',(-18.4949130543925,13.6508696677346,122.611834937817)) ;
#79390=CARTESIAN_POINT('Ctrl Pts',(-18.4948315724147,13.6508638228506,122.611928077016)) ;
#79391=CARTESIAN_POINT('Ctrl Pts',(-18.4946644310987,13.6508518315636,122.612119189324)) ;
#79392=CARTESIAN_POINT('Ctrl Pts',(-18.4945787733826,13.6508456851806,122.612217163619)) ;
#79393=CARTESIAN_POINT('Ctrl Pts',(-18.4908484797438,13.6505779734918,122.616485213669)) ;
#79394=CARTESIAN_POINT('Ctrl Pts',(-18.4872323786622,13.6503166335513,122.620680155562)) ;
#79395=CARTESIAN_POINT('Ctrl Pts',(-18.4792695286078,13.6497369943918,122.630046391917)) ;
#79396=CARTESIAN_POINT('Ctrl Pts',(-18.4749369697328,13.6494188087734,122.635229512879)) ;
#79397=CARTESIAN_POINT('Ctrl Pts',(-18.4584470181595,13.6481965312508,122.655294493191)) ;
#79398=CARTESIAN_POINT('Ctrl Pts',(-18.4466001150082,13.647294652107,122.670427861931)) ;
#79399=CARTESIAN_POINT('Ctrl Pts',(-18.4296220647914,13.6459607527988,122.693209213516)) ;
#79400=CARTESIAN_POINT('Ctrl Pts',(-18.4242109104843,13.6455289737106,122.700644679848)) ;
#79401=CARTESIAN_POINT('Ctrl Pts',(-18.4155583177141,13.6448266814834,122.712822433335)) ;
#79402=CARTESIAN_POINT('Ctrl Pts',(-18.4122651750663,13.6445564929113,122.717527543225)) ;
#79403=CARTESIAN_POINT('Ctrl Pts',(-18.4073550932428,13.6441490076542,122.724649841005)) ;
#79404=CARTESIAN_POINT('Ctrl Pts',(-18.4057132684771,13.644011961902,122.727049774961)) ;
#79405=CARTESIAN_POINT('Ctrl Pts',(-18.4021410832575,13.6437120665719,122.732311848014)) ;
#79406=CARTESIAN_POINT('Ctrl Pts',(-18.4002142742678,13.6435491915603,122.735176367436)) ;
#79407=CARTESIAN_POINT('Ctrl Pts',(-18.396115383237,13.6432003403124,122.741326486652)) ;
#79408=CARTESIAN_POINT('Ctrl Pts',(-18.3939470158841,13.6430143445044,122.744614515806)) ;
#79409=CARTESIAN_POINT('Ctrl Pts',(-18.3826132896108,13.6420345896768,122.761983734693)) ;
#79410=CARTESIAN_POINT('Ctrl Pts',(-18.3737247711066,13.6412398806722,122.77624337438)) ;
#79411=CARTESIAN_POINT('Ctrl Pts',(-18.3578985921804,13.6397765946518,122.802846674507)) ;
#79412=CARTESIAN_POINT('Ctrl Pts',(-18.350875427845,13.6391079725304,122.815136146935)) ;
#79413=CARTESIAN_POINT('Ctrl Pts',(-18.3398105772798,13.6380224992468,122.835308199664)) ;
#79414=CARTESIAN_POINT('Ctrl Pts',(-18.3356375516177,13.6376051463502,122.843117181785)) ;
#79415=CARTESIAN_POINT('Ctrl Pts',(-18.327643930231,13.6367896562752,122.858477238561)) ;
#79416=CARTESIAN_POINT('Ctrl Pts',(-18.3238161303173,13.6363915084997,122.866024000894)) ;
#79417=CARTESIAN_POINT('Ctrl Pts',(-18.3149411037336,13.6354496403047,122.88398437991)) ;
#79418=CARTESIAN_POINT('Ctrl Pts',(-18.3099632008601,13.6349062543894,122.894431339147)) ;
#79419=CARTESIAN_POINT('Ctrl Pts',(-18.2956934700033,13.633301241689,122.925514670719)) ;
#79420=CARTESIAN_POINT('Ctrl Pts',(-18.2868281617792,13.6322406103379,122.946341262557)) ;
#79421=CARTESIAN_POINT('Ctrl Pts',(-18.2753976843105,13.6307720674936,122.975422687535)) ;
#79422=CARTESIAN_POINT('Ctrl Pts',(-18.2723310610967,13.6303667541518,122.98347538022)) ;
#79423=CARTESIAN_POINT('Ctrl Pts',(-18.267028754269,13.6296449177385,122.997856966129)) ;
#79424=CARTESIAN_POINT('Ctrl Pts',(-18.2647593636358,13.6293285924177,123.004173052405)) ;
#79425=CARTESIAN_POINT('Ctrl Pts',(-18.2615783781736,13.6288742876962,123.013262227138)) ;
#79426=CARTESIAN_POINT('Ctrl Pts',(-18.2606242585385,13.6287365493174,123.016020311112)) ;
#79427=CARTESIAN_POINT('Ctrl Pts',(-18.2595004286607,13.6285725369429,123.019307264429)) ;
#79428=CARTESIAN_POINT('Ctrl Pts',(-18.2593211307022,13.6285463155574,123.01983284811)) ;
#79429=CARTESIAN_POINT('Ctrl Pts',(-18.2589566920424,13.6284929069755,123.020903544316)) ;
#79430=CARTESIAN_POINT('Ctrl Pts',(-18.2587715783088,13.6284657196391,123.021448665889)) ;
#79431=CARTESIAN_POINT('Ctrl Pts',(-18.2584418935593,13.6284171940844,123.022421790307)) ;
#79432=CARTESIAN_POINT('Ctrl Pts',(-18.2582971736603,13.6283958566734,123.022849742647)) ;
#79433=CARTESIAN_POINT('Ctrl Pts',(-18.2580414169979,13.628358083488,123.023607435025)) ;
#79434=CARTESIAN_POINT('Ctrl Pts',(-18.2579302831241,13.6283416482388,123.023937142227)) ;
#79435=CARTESIAN_POINT('Ctrl Pts',(-18.2545355857349,13.6278389528537,123.034022696292)) ;
#79436=CARTESIAN_POINT('Ctrl Pts',(-18.2513760090569,13.6273520380258,123.043819803597)) ;
#79437=CARTESIAN_POINT('Ctrl Pts',(-18.2443860235532,13.6262291937492,123.066475791756)) ;
#79438=CARTESIAN_POINT('Ctrl Pts',(-18.2406433585346,13.6255929325413,123.079360338553)) ;
#79439=CARTESIAN_POINT('Ctrl Pts',(-18.2304888521251,13.6237608650259,123.116610903915)) ;
#79440=CARTESIAN_POINT('Ctrl Pts',(-18.2246204691796,13.6225650397346,123.141117983595)) ;
#79441=CARTESIAN_POINT('Ctrl Pts',(-18.2181089382832,13.6210446163846,123.172604666996)) ;
#79442=CARTESIAN_POINT('Ctrl Pts',(-18.2167581942384,13.6207158728074,123.17943146443)) ;
#79443=CARTESIAN_POINT('Ctrl Pts',(-18.2152737832695,13.6203385587359,123.18728774374)) ;
#79444=CARTESIAN_POINT('Ctrl Pts',(-18.2150826942761,13.620289663212,123.188306227561)) ;
#79445=CARTESIAN_POINT('Ctrl Pts',(-18.2142021764829,13.6200628449607,123.193032649327)) ;
#79446=CARTESIAN_POINT('Ctrl Pts',(-18.2135287120729,13.6198850141926,123.196743544139)) ;
#79447=CARTESIAN_POINT('Ctrl Pts',(-18.2116164479277,13.6193670423708,123.207567033146)) ;
#79448=CARTESIAN_POINT('Ctrl Pts',(-18.2104237530695,13.6190271646022,123.214687614956)) ;
#79449=CARTESIAN_POINT('Ctrl Pts',(-18.2085783113974,13.6184721435695,123.226341859156)) ;
#79450=CARTESIAN_POINT('Ctrl Pts',(-18.2078876103002,13.6182568361054,123.230869316774)) ;
#79451=CARTESIAN_POINT('Ctrl Pts',(-18.2052015149846,13.617387620246,123.249169814321)) ;
#79452=CARTESIAN_POINT('Ctrl Pts',(-18.2034172405489,13.6167345433705,123.262972760568)) ;
#79453=CARTESIAN_POINT('Ctrl Pts',(-18.2006525764722,13.6155665999296,123.287693524581)) ;
#79454=CARTESIAN_POINT('Ctrl Pts',(-18.1995820592074,13.6150519101811,123.298599677515)) ;
#79455=CARTESIAN_POINT('Ctrl Pts',(-18.1982208540007,13.6142911221513,123.314705734439)) ;
#79456=CARTESIAN_POINT('Ctrl Pts',(-18.1978158199284,13.6140458528795,123.319895433881)) ;
#79457=CARTESIAN_POINT('Ctrl Pts',(-18.1970577169954,13.6135451521361,123.330485979255)) ;
#79458=CARTESIAN_POINT('Ctrl Pts',(-18.1967073600709,13.6132897117557,123.335886912264)) ;
#79459=CARTESIAN_POINT('Ctrl Pts',(-18.1950267723857,13.6119228512249,123.364781718951)) ;
#79460=CARTESIAN_POINT('Ctrl Pts',(-18.1943432320815,13.61080917445,123.388308161591)) ;
#79461=CARTESIAN_POINT('Ctrl Pts',(-18.1943434021578,13.609157782117,123.423247243905)) ;
#79462=CARTESIAN_POINT('Ctrl Pts',(-18.194504127961,13.6086189937792,123.434654376293)) ;
#79463=CARTESIAN_POINT('Ctrl Pts',(-18.1950044016075,13.6077812304192,123.452406709026)) ;
#79464=CARTESIAN_POINT('Ctrl Pts',(-18.1952331124391,13.607481816352,123.458754352997)) ;
#79465=CARTESIAN_POINT('Ctrl Pts',(-18.1958107050816,13.6068612975726,123.471915735628)) ;
#79466=CARTESIAN_POINT('Ctrl Pts',(-18.1961672260551,13.606540240931,123.478728922459)) ;
#79467=CARTESIAN_POINT('Ctrl Pts',(-18.1973597663866,13.605616062619,123.498350087162)) ;
#79468=CARTESIAN_POINT('Ctrl Pts',(-18.1983413870918,13.6050137915715,123.511148327642)) ;
#79469=CARTESIAN_POINT('Ctrl Pts',(-18.2012391874975,13.6035427352008,123.542421767675)) ;
#79470=CARTESIAN_POINT('Ctrl Pts',(-18.2033765847497,13.6026750236002,123.56087314896)) ;
#79471=CARTESIAN_POINT('Ctrl Pts',(-18.2076194582323,13.6012333141427,123.591366190679)) ;
#79472=CARTESIAN_POINT('Ctrl Pts',(-18.209485124377,13.600660581677,123.60343794615)) ;
#79473=CARTESIAN_POINT('Ctrl Pts',(-18.2123924361722,13.5998452096326,123.620537218982)) ;
#79474=CARTESIAN_POINT('Ctrl Pts',(-18.2132844079912,13.5996037878829,123.625589457785)) ;
#79475=CARTESIAN_POINT('Ctrl Pts',(-18.2148941212654,13.5991826940958,123.634381443263)) ;
#79476=CARTESIAN_POINT('Ctrl Pts',(-18.2155974947312,13.5990031494525,123.638123750475)) ;
#79477=CARTESIAN_POINT('Ctrl Pts',(-18.2170190896535,13.5986488044543,123.645496269393)) ;
#79478=CARTESIAN_POINT('Ctrl Pts',(-18.2177363267868,13.5984740148728,123.649126629111)) ;
#79479=CARTESIAN_POINT('Ctrl Pts',(-18.2193309282037,13.5980938559592,123.657008293661)) ;
#79480=CARTESIAN_POINT('Ctrl Pts',(-18.2202145129041,13.5978884315067,123.661258284551)) ;
#79481=CARTESIAN_POINT('Ctrl Pts',(-18.2224492113203,13.5973814111263,123.671725255282)) ;
#79482=CARTESIAN_POINT('Ctrl Pts',(-18.2238264152357,13.5970795796651,123.677936518863)) ;
#79483=CARTESIAN_POINT('Ctrl Pts',(-18.234673827614,13.5947801931096,123.725102814226)) ;
#79484=CARTESIAN_POINT('Ctrl Pts',(-18.2462119199981,13.5927605622578,123.765542013498)) ;
#79485=CARTESIAN_POINT('Ctrl Pts',(-18.259825879779,13.5907660201144,123.80531165987)) ;
#79486=CARTESIAN_POINT('',(-18.9360879630843,13.6947924664109,122.292840804082)) ;
#79487=CARTESIAN_POINT('Origin',(-19.4092696481994,13.6947924276734,123.411833733891)) ;
#79488=CARTESIAN_POINT('Ctrl Pts',(-18.259825879779,13.6088050314641,123.80531165987)) ;
#79489=CARTESIAN_POINT('Ctrl Pts',(-18.2564562893653,13.6092962280985,123.795468276951)) ;
#79490=CARTESIAN_POINT('Ctrl Pts',(-18.2532163611542,13.6097873550664,123.785591544476)) ;
#79491=CARTESIAN_POINT('Ctrl Pts',(-18.2459652224294,13.6109330714525,123.762489366047)) ;
#79492=CARTESIAN_POINT('Ctrl Pts',(-18.2420547455701,13.6115880006948,123.749244356245)) ;
#79493=CARTESIAN_POINT('Ctrl Pts',(-18.2336384625199,13.613086132159,123.718838447372)) ;
#79494=CARTESIAN_POINT('Ctrl Pts',(-18.2292810266786,13.613929052619,123.701639598016)) ;
#79495=CARTESIAN_POINT('Ctrl Pts',(-18.2239139371324,13.6150630225712,123.67832199731)) ;
#79496=CARTESIAN_POINT('Ctrl Pts',(-18.2225721890224,13.6153559808195,123.672281997486)) ;
#79497=CARTESIAN_POINT('Ctrl Pts',(-18.2203539340453,13.615857027945,123.661923158797)) ;
#79498=CARTESIAN_POINT('Ctrl Pts',(-18.2194546811356,13.6160652740971,123.65760932423)) ;
#79499=CARTESIAN_POINT('Ctrl Pts',(-18.2177570205037,13.6164686039618,123.649237694831)) ;
#79500=CARTESIAN_POINT('Ctrl Pts',(-18.2169558232867,13.6166637067782,123.64518052803)) ;
#79501=CARTESIAN_POINT('Ctrl Pts',(-18.2154082507614,13.617050237762,123.637127692457)) ;
#79502=CARTESIAN_POINT('Ctrl Pts',(-18.2146611815556,13.6172416691909,123.633132211637)) ;
#79503=CARTESIAN_POINT('Ctrl Pts',(-18.2129141051487,13.6177013032481,123.623521773489)) ;
#79504=CARTESIAN_POINT('Ctrl Pts',(-18.2119335561518,13.6179693390961,123.617903371218)) ;
#79505=CARTESIAN_POINT('Ctrl Pts',(-18.2060579317768,13.6196410747871,123.582778325726)) ;
#79506=CARTESIAN_POINT('Ctrl Pts',(-18.202214341137,13.6210342463854,123.553106455399)) ;
#79507=CARTESIAN_POINT('Ctrl Pts',(-18.1983381607293,13.623004567995,123.511044929049)) ;
#79508=CARTESIAN_POINT('Ctrl Pts',(-18.1973936704148,13.6235802564231,123.49875060712)) ;
#79509=CARTESIAN_POINT('Ctrl Pts',(-18.1962670461933,13.6244391662219,123.48043973661)) ;
#79510=CARTESIAN_POINT('Ctrl Pts',(-18.1959422151088,13.6247211671628,123.474432749139)) ;
#79511=CARTESIAN_POINT('Ctrl Pts',(-18.1955975267177,13.6250685924995,123.467040687546)) ;
#79512=CARTESIAN_POINT('Ctrl Pts',(-18.1955354054134,13.6251336119667,123.465657653257)) ;
#79513=CARTESIAN_POINT('Ctrl Pts',(-18.1954492384305,13.6252273999616,123.463663235883)) ;
#79514=CARTESIAN_POINT('Ctrl Pts',(-18.1954232903798,13.6252561500617,123.463051935274)) ;
#79515=CARTESIAN_POINT('Ctrl Pts',(-18.1953670456238,13.6253196076563,123.461702833796)) ;
#79516=CARTESIAN_POINT('Ctrl Pts',(-18.1953369597583,13.625354317194,123.460965024485)) ;
#79517=CARTESIAN_POINT('Ctrl Pts',(-18.1952866275414,13.6254137239474,123.459702430108)) ;
#79518=CARTESIAN_POINT('Ctrl Pts',(-18.195266048772,13.6254384178796,123.459177658353)) ;
#79519=CARTESIAN_POINT('Ctrl Pts',(-18.1952314934586,13.6254805861963,123.458281637977)) ;
#79520=CARTESIAN_POINT('Ctrl Pts',(-18.1952173469225,13.6254980588921,123.457910395917)) ;
#79521=CARTESIAN_POINT('Ctrl Pts',(-18.1951934799149,13.6255278996214,123.457276421153)) ;
#79522=CARTESIAN_POINT('Ctrl Pts',(-18.195183674439,13.6255402668077,123.457013691635)) ;
#79523=CARTESIAN_POINT('Ctrl Pts',(-18.1951034828839,13.6256423030949,123.454846147898)) ;
#79524=CARTESIAN_POINT('Ctrl Pts',(-18.1950374944242,13.6257320159899,123.452941175793)) ;
#79525=CARTESIAN_POINT('Ctrl Pts',(-18.1948724114947,13.6259729329115,123.447827735397)) ;
#79526=CARTESIAN_POINT('Ctrl Pts',(-18.1947815494378,13.6261242199306,123.444619021083)) ;
#79527=CARTESIAN_POINT('Ctrl Pts',(-18.1946260758413,13.6264254778985,123.438234424099)) ;
#79528=CARTESIAN_POINT('Ctrl Pts',(-18.1945612010521,13.6265754449172,123.435058573375)) ;
#79529=CARTESIAN_POINT('Ctrl Pts',(-18.1944213280746,13.6269759534525,123.426583664769)) ;
#79530=CARTESIAN_POINT('Ctrl Pts',(-18.1943685459481,13.6272267195798,123.421284321665)) ;
#79531=CARTESIAN_POINT('Ctrl Pts',(-18.1942833764605,13.6284078058714,123.396357802433)) ;
#79532=CARTESIAN_POINT('Ctrl Pts',(-18.1946919357149,13.6293425243796,123.376732255174)) ;
#79533=CARTESIAN_POINT('Ctrl Pts',(-18.1962526191702,13.6309963678789,123.342108738325)) ;
#79534=CARTESIAN_POINT('Ctrl Pts',(-18.1972081455711,13.6317144393419,123.32710590241)) ;
#79535=CARTESIAN_POINT('Ctrl Pts',(-18.1992965550747,13.6329274508423,123.301745061226)) ;
#79536=CARTESIAN_POINT('Ctrl Pts',(-18.2002847244539,13.633423138966,123.291376854638)) ;
#79537=CARTESIAN_POINT('Ctrl Pts',(-18.2019976366522,13.6341784956299,123.275560424387)) ;
#79538=CARTESIAN_POINT('Ctrl Pts',(-18.2026262317556,13.6344390207153,123.27010232765)) ;
#79539=CARTESIAN_POINT('Ctrl Pts',(-18.2037437577747,13.6348758282347,123.260945744652)) ;
#79540=CARTESIAN_POINT('Ctrl Pts',(-18.204212738107,13.6350523041372,123.257244918266)) ;
#79541=CARTESIAN_POINT('Ctrl Pts',(-18.2051125264461,13.6353787046762,123.250397505548)) ;
#79542=CARTESIAN_POINT('Ctrl Pts',(-18.2055386416694,13.6355286752487,123.247250338092)) ;
#79543=CARTESIAN_POINT('Ctrl Pts',(-18.2064284190062,13.6358327684773,123.240867042304)) ;
#79544=CARTESIAN_POINT('Ctrl Pts',(-18.2068928124685,13.6359868824479,123.237631042295)) ;
#79545=CARTESIAN_POINT('Ctrl Pts',(-18.2080180331836,13.6363497851968,123.230009157782)) ;
#79546=CARTESIAN_POINT('Ctrl Pts',(-18.2086898284105,13.6365584629146,123.225624936459)) ;
#79547=CARTESIAN_POINT('Ctrl Pts',(-18.2109085125464,13.6372231778854,123.211656862707)) ;
#79548=CARTESIAN_POINT('Ctrl Pts',(-18.2125462712004,13.6376783420359,123.202087808503)) ;
#79549=CARTESIAN_POINT('Ctrl Pts',(-18.2180623851035,13.6391088997323,123.172029585398)) ;
#79550=CARTESIAN_POINT('Ctrl Pts',(-18.2223536006575,13.6400811046775,123.151620229648)) ;
#79551=CARTESIAN_POINT('Ctrl Pts',(-18.2294474806769,13.6415183580902,123.121724966207)) ;
#79552=CARTESIAN_POINT('Ctrl Pts',(-18.2318440194524,13.6419809828871,123.112146675963)) ;
#79553=CARTESIAN_POINT('Ctrl Pts',(-18.2361796364587,13.6427804358337,123.095673857986)) ;
#79554=CARTESIAN_POINT('Ctrl Pts',(-18.238063424983,13.6431168898146,123.088765279786)) ;
#79555=CARTESIAN_POINT('Ctrl Pts',(-18.2419533084532,13.6437905745017,123.074980904348)) ;
#79556=CARTESIAN_POINT('Ctrl Pts',(-18.243959351904,13.6441277922126,123.068105382182)) ;
#79557=CARTESIAN_POINT('Ctrl Pts',(-18.2482774810884,13.6448330024152,123.053777824394)) ;
#79558=CARTESIAN_POINT('Ctrl Pts',(-18.2506007962213,13.6452010358916,123.046329508825)) ;
#79559=CARTESIAN_POINT('Ctrl Pts',(-18.2599595808061,13.6466403538199,123.017312449718)) ;
#79560=CARTESIAN_POINT('Ctrl Pts',(-18.2675268759253,13.6477135559427,122.995920143408)) ;
#79561=CARTESIAN_POINT('Ctrl Pts',(-18.279967349156,13.6493493626998,122.963655473976)) ;
#79562=CARTESIAN_POINT('Ctrl Pts',(-18.284408754828,13.649911866091,122.952622009087)) ;
#79563=CARTESIAN_POINT('Ctrl Pts',(-18.2925336316627,13.6509038972777,122.933263473938)) ;
#79564=CARTESIAN_POINT('Ctrl Pts',(-18.2961500094947,13.6513335568294,122.924911259401)) ;
#79565=CARTESIAN_POINT('Ctrl Pts',(-18.3037111180125,13.6522084660053,122.907973042786)) ;
#79566=CARTESIAN_POINT('Ctrl Pts',(-18.3076628452589,13.6526536996475,122.899390846101)) ;
#79567=CARTESIAN_POINT('Ctrl Pts',(-18.3240877969109,13.6544578782878,122.864788056701)) ;
#79568=CARTESIAN_POINT('Ctrl Pts',(-18.3373860627355,13.6558145092602,122.839169604252)) ;
#79569=CARTESIAN_POINT('Ctrl Pts',(-18.3563577046227,13.6576311507509,122.805602270166)) ;
#79570=CARTESIAN_POINT('Ctrl Pts',(-18.3612326411174,13.6580885406466,122.797213053388)) ;
#79571=CARTESIAN_POINT('Ctrl Pts',(-18.3705490569635,13.6589459487467,122.781613739776)) ;
#79572=CARTESIAN_POINT('Ctrl Pts',(-18.3749664481735,13.659345833808,122.77438993363)) ;
#79573=CARTESIAN_POINT('Ctrl Pts',(-18.383588437236,13.6601141598129,122.760615917939)) ;
#79574=CARTESIAN_POINT('Ctrl Pts',(-18.387781179161,13.6604825122246,122.754058773662)) ;
#79575=CARTESIAN_POINT('Ctrl Pts',(-18.3976194324177,13.6613351856627,122.73899340026)) ;
#79576=CARTESIAN_POINT('Ctrl Pts',(-18.4033097695088,13.6618198828758,122.730515162381)) ;
#79577=CARTESIAN_POINT('Ctrl Pts',(-18.4202130063289,13.6632335594721,122.706003909944)) ;
#79578=CARTESIAN_POINT('Ctrl Pts',(-18.4317072109679,13.6641623326182,122.690168663861)) ;
#79579=CARTESIAN_POINT('Ctrl Pts',(-18.4471883399265,13.6653693068245,122.669889685581)) ;
#79580=CARTESIAN_POINT('Ctrl Pts',(-18.4508325225009,13.6656504282505,122.665188107336)) ;
#79581=CARTESIAN_POINT('Ctrl Pts',(-18.4572200824706,13.6661380218222,122.657070958923)) ;
#79582=CARTESIAN_POINT('Ctrl Pts',(-18.4599476723875,13.6663446364539,122.653643118703)) ;
#79583=CARTESIAN_POINT('Ctrl Pts',(-18.4636318105319,13.6666215935145,122.649064205802)) ;
#79584=CARTESIAN_POINT('Ctrl Pts',(-18.464572027648,13.666692092101,122.647900046385)) ;
#79585=CARTESIAN_POINT('Ctrl Pts',(-18.4658206461076,13.6667854740941,122.646359860348)) ;
#79586=CARTESIAN_POINT('Ctrl Pts',(-18.4661271252323,13.6668083759759,122.645982278287)) ;
#79587=CARTESIAN_POINT('Ctrl Pts',(-18.4667143615206,13.6668522210344,122.645259690702)) ;
#79588=CARTESIAN_POINT('Ctrl Pts',(-18.4669950815863,13.6668731645636,122.644914655173)) ;
#79589=CARTESIAN_POINT('Ctrl Pts',(-18.4675599706263,13.6669152768415,122.64422112339)) ;
#79590=CARTESIAN_POINT('Ctrl Pts',(-18.4678441437124,13.6669364455462,122.643872630588)) ;
#79591=CARTESIAN_POINT('Ctrl Pts',(-18.4684370675434,13.666980579879,122.643146328095)) ;
#79592=CARTESIAN_POINT('Ctrl Pts',(-18.468745852542,13.667003545173,122.642768546466)) ;
#79593=CARTESIAN_POINT('Ctrl Pts',(-18.4694093438442,13.6670528500513,122.641957798217)) ;
#79594=CARTESIAN_POINT('Ctrl Pts',(-18.4697641219677,13.6670791889417,122.641524890455)) ;
#79595=CARTESIAN_POINT('Ctrl Pts',(-18.4705455851007,13.6671371499667,122.640572675589)) ;
#79596=CARTESIAN_POINT('Ctrl Pts',(-18.470972402171,13.6671687708286,122.640053477041)) ;
#79597=CARTESIAN_POINT('Ctrl Pts',(-18.4719322138242,13.6672397978661,122.638887894127)) ;
#79598=CARTESIAN_POINT('Ctrl Pts',(-18.4724654466735,13.6672792017572,122.638241706278)) ;
#79599=CARTESIAN_POINT('Ctrl Pts',(-18.4765703910961,13.667582113637,122.633277677682)) ;
#79600=CARTESIAN_POINT('Ctrl Pts',(-18.4801712756447,13.6678453409675,122.628984034479)) ;
#79601=CARTESIAN_POINT('Ctrl Pts',(-18.4899014074659,13.668550155612,122.617543663116)) ;
#79602=CARTESIAN_POINT('Ctrl Pts',(-18.4960842433719,13.6689912538493,122.610443007093)) ;
#79603=CARTESIAN_POINT('Ctrl Pts',(-18.5240798442053,13.6709605208992,122.579036278452)) ;
#79604=CARTESIAN_POINT('Ctrl Pts',(-18.5467846894472,13.6724847048018,122.555543893391)) ;
#79605=CARTESIAN_POINT('Ctrl Pts',(-18.5755388343141,13.6743523945134,122.528097754247)) ;
#79606=CARTESIAN_POINT('Ctrl Pts',(-18.5807119573899,13.6746859996298,122.523245806392)) ;
#79607=CARTESIAN_POINT('Ctrl Pts',(-18.589823996568,13.6752695688853,122.514848250222)) ;
#79608=CARTESIAN_POINT('Ctrl Pts',(-18.5937441841526,13.6755193482774,122.511282596168)) ;
#79609=CARTESIAN_POINT('Ctrl Pts',(-18.6015539987737,13.67601446339,122.504271901532)) ;
#79610=CARTESIAN_POINT('Ctrl Pts',(-18.6054426484631,13.6762597855394,122.500825937737)) ;
#79611=CARTESIAN_POINT('Ctrl Pts',(-18.6141667967013,13.676807500341,122.493194298984)) ;
#79612=CARTESIAN_POINT('Ctrl Pts',(-18.6190134795332,13.6771099844421,122.489021649032)) ;
#79613=CARTESIAN_POINT('Ctrl Pts',(-18.6320838473187,13.6779208912446,122.477947475206)) ;
#79614=CARTESIAN_POINT('Ctrl Pts',(-18.640366430774,13.6784297276285,122.471116371774)) ;
#79615=CARTESIAN_POINT('Ctrl Pts',(-18.6688459104096,13.6801616749723,122.448255203425)) ;
#79616=CARTESIAN_POINT('Ctrl Pts',(-18.6894622650883,13.6813849840397,122.4327585348)) ;
#79617=CARTESIAN_POINT('Ctrl Pts',(-18.7184348985361,13.6830594541009,122.412390805274)) ;
#79618=CARTESIAN_POINT('Ctrl Pts',(-18.7263792448967,13.6835143183134,122.406945920495)) ;
#79619=CARTESIAN_POINT('Ctrl Pts',(-18.7419195041533,13.684396193969,122.396564359429)) ;
#79620=CARTESIAN_POINT('Ctrl Pts',(-18.7495075505735,13.6848232259129,122.391617044542)) ;
#79621=CARTESIAN_POINT('Ctrl Pts',(-18.7853774019248,13.6868261288562,122.36879789083)) ;
#79622=CARTESIAN_POINT('Ctrl Pts',(-18.8143341811245,13.6883969627492,122.352014367238)) ;
#79623=CARTESIAN_POINT('Ctrl Pts',(-18.8497577460213,13.6902829323459,122.333392446661)) ;
#79624=CARTESIAN_POINT('Ctrl Pts',(-18.855593582267,13.6905925376429,122.330384709293)) ;
#79625=CARTESIAN_POINT('Ctrl Pts',(-18.8663637957803,13.6911621852468,122.3249438696)) ;
#79626=CARTESIAN_POINT('Ctrl Pts',(-18.8712908755244,13.6914221133452,122.322496696073)) ;
#79627=CARTESIAN_POINT('Ctrl Pts',(-18.8959361022421,13.6927185803656,122.31046393456)) ;
#79628=CARTESIAN_POINT('Ctrl Pts',(-18.9158945839319,13.6937564904598,122.30137985629)) ;
#79629=CARTESIAN_POINT('Ctrl Pts',(-18.9360879635506,13.6947924657244,122.292840805121)) ;
#79630=CARTESIAN_POINT('Origin',(-19.4092696390626,-30.19753203383,123.411833654984)) ;
#79631=CARTESIAN_POINT('',(-18.259825879779,13.2308616644972,123.80531165987)) ;
#79632=CARTESIAN_POINT('',(-18.259825879779,13.2488777185652,123.80531165987)) ;
#79633=CARTESIAN_POINT('',(-18.259825879779,-30.19753203383,123.80531165987)) ;
#79634=CARTESIAN_POINT('Ctrl Pts',(-18.259825879779,13.5907660201144,123.80531165987)) ;
#79635=CARTESIAN_POINT('Ctrl Pts',(-18.2670498048973,13.5897076635949,123.82641448021)) ;
#79636=CARTESIAN_POINT('Ctrl Pts',(-18.2749563117422,13.5886447944099,123.847601447194)) ;
#79637=CARTESIAN_POINT('Ctrl Pts',(-18.2834835869921,13.5875842682099,123.868617697009)) ;
#79638=CARTESIAN_POINT('Ctrl Pts',(-18.2913328258975,13.5866080685136,123.887962864235)) ;
#79639=CARTESIAN_POINT('Ctrl Pts',(-18.2997074255637,13.5856338540164,123.907163230561)) ;
#79640=CARTESIAN_POINT('Ctrl Pts',(-18.3085224981892,13.5846669715988,123.926033643261)) ;
#79641=CARTESIAN_POINT('Ctrl Pts',(-18.3242374298226,13.582943277225,123.959674573753)) ;
#79642=CARTESIAN_POINT('Ctrl Pts',(-18.3415966595897,13.5811956620891,123.992803532846)) ;
#79643=CARTESIAN_POINT('Ctrl Pts',(-18.3605241308919,13.5794267489625,124.02516778511)) ;
#79644=CARTESIAN_POINT('Ctrl Pts',(-18.3770062101987,13.5778863759261,124.053350639755)) ;
#79645=CARTESIAN_POINT('Ctrl Pts',(-18.3946766021965,13.5763298527071,124.080953537037)) ;
#79646=CARTESIAN_POINT('Ctrl Pts',(-18.4134553013666,13.5747589111888,124.10782194578)) ;
#79647=CARTESIAN_POINT('Ctrl Pts',(-18.4540898318688,13.5713596091144,124.165961498721)) ;
#79648=CARTESIAN_POINT('Ctrl Pts',(-18.4997513226257,13.568019599761,124.220445584582)) ;
#79649=CARTESIAN_POINT('Ctrl Pts',(-18.5498882588795,13.5647273358169,124.270617410932)) ;
#79650=CARTESIAN_POINT('Ctrl Pts',(-18.5948655602435,13.5617738815645,124.315626011823)) ;
#79651=CARTESIAN_POINT('Ctrl Pts',(-18.6433284015354,13.5587726665132,124.357044740922)) ;
#79652=CARTESIAN_POINT('Ctrl Pts',(-18.6947613526575,13.5557426318646,124.394444363629)) ;
#79653=CARTESIAN_POINT('Ctrl Pts',(-18.7001312190031,13.555426280562,124.398349077843)) ;
#79654=CARTESIAN_POINT('Ctrl Pts',(-18.705533431782,13.5551096151131,124.40221001865)) ;
#79655=CARTESIAN_POINT('Ctrl Pts',(-18.7109673834869,13.5547926570741,124.406026722725)) ;
#79656=CARTESIAN_POINT('Ctrl Pts',(-18.7581903583382,13.5520381788752,124.439195239911)) ;
#79657=CARTESIAN_POINT('Ctrl Pts',(-18.8077515425201,13.5493260681322,124.468976363899)) ;
#79658=CARTESIAN_POINT('Ctrl Pts',(-18.8591950807205,13.5466198502772,124.495099031681)) ;
#79659=CARTESIAN_POINT('Ctrl Pts',(-18.8709542339264,13.5460012530446,124.501070247179)) ;
#79660=CARTESIAN_POINT('Ctrl Pts',(-18.8828116330102,13.5453829637183,124.50685049238)) ;
#79661=CARTESIAN_POINT('Ctrl Pts',(-18.8947616420897,13.5447645466604,124.51243686102)) ;
#79662=CARTESIAN_POINT('Ctrl Pts',(-18.9476600207136,13.5420270374701,124.537165699424)) ;
#79663=CARTESIAN_POINT('Ctrl Pts',(-19.0023100478866,13.5392673299222,124.55806150127)) ;
#79664=CARTESIAN_POINT('Ctrl Pts',(-19.0582017493017,13.5365087036994,124.574931773315)) ;
#79665=CARTESIAN_POINT('Ctrl Pts',(-19.0700891535024,13.5359219814469,124.578519850573)) ;
#79666=CARTESIAN_POINT('Ctrl Pts',(-19.0820326607393,13.5353353081087,124.581926006936)) ;
#79667=CARTESIAN_POINT('Ctrl Pts',(-19.0940272594464,13.534748907658,124.585148675846)) ;
#79668=CARTESIAN_POINT('Ctrl Pts',(-19.1560279959301,13.5317177716688,124.601806827629)) ;
#79669=CARTESIAN_POINT('Ctrl Pts',(-19.2192945917692,13.5286932114462,124.613531456762)) ;
#79670=CARTESIAN_POINT('Ctrl Pts',(-19.2831523162566,13.5256682002,124.620196314525)) ;
#79671=CARTESIAN_POINT('Ctrl Pts',(-19.2894573643986,13.5253695230754,124.620854375072)) ;
#79672=CARTESIAN_POINT('Ctrl Pts',(-19.2957681666485,13.5250708415538,124.621463150064)) ;
#79673=CARTESIAN_POINT('Ctrl Pts',(-19.30208406715,13.5247721488717,124.622022544893)) ;
#79674=CARTESIAN_POINT('Ctrl Pts',(-19.3724201145366,13.5214458040943,124.628252158739)) ;
#79675=CARTESIAN_POINT('Ctrl Pts',(-19.4431858765432,13.5181307274801,124.628339299033)) ;
#79676=CARTESIAN_POINT('Ctrl Pts',(-19.5135678275382,13.5147860917316,124.622274807608)) ;
#79677=CARTESIAN_POINT('Ctrl Pts',(-19.5467219612299,13.5132105670525,124.619418067256)) ;
#79678=CARTESIAN_POINT('Ctrl Pts',(-19.5797175096476,13.5116375405296,124.615198391511)) ;
#79679=CARTESIAN_POINT('Ctrl Pts',(-19.6123170938337,13.5100766230102,124.609672386699)) ;
#79680=CARTESIAN_POINT('Ctrl Pts',(-19.645053057037,13.5085091754567,124.604123264074)) ;
#79681=CARTESIAN_POINT('Ctrl Pts',(-19.6773891298795,13.5069539384338,124.597257065943)) ;
#79682=CARTESIAN_POINT('Ctrl Pts',(-19.7091004801917,13.5054206439141,124.589181251403)) ;
#79683=CARTESIAN_POINT('Ctrl Pts',(-19.7129404738416,13.5052349740778,124.588203334151)) ;
#79684=CARTESIAN_POINT('Ctrl Pts',(-19.7167713319802,13.505049625991,124.587207737506)) ;
#79685=CARTESIAN_POINT('Ctrl Pts',(-19.7205926771953,13.5048646169337,124.586194699133)) ;
#79686=CARTESIAN_POINT('Ctrl Pts',(-19.7377483977952,13.5040340288771,124.581646718692)) ;
#79687=CARTESIAN_POINT('Ctrl Pts',(-19.755025123028,13.5031929130004,124.576659824249)) ;
#79688=CARTESIAN_POINT('Ctrl Pts',(-19.7721228851667,13.5023530749188,124.571309147557)) ;
#79689=CARTESIAN_POINT('Ctrl Pts',(-19.7823793181949,13.5018492813248,124.568099437614)) ;
#79690=CARTESIAN_POINT('Ctrl Pts',(-19.7925715867773,13.5013459475377,124.564759803787)) ;
#79691=CARTESIAN_POINT('Ctrl Pts',(-19.802637638995,13.500845621912,124.561315065323)) ;
#79692=CARTESIAN_POINT('Ctrl Pts',(-19.8235243601466,13.499807462999,124.554167348404)) ;
#79693=CARTESIAN_POINT('Ctrl Pts',(-19.8444590456297,13.4987524949004,124.546362707362)) ;
#79694=CARTESIAN_POINT('Ctrl Pts',(-19.8651875154715,13.4976925462973,124.537970763003)) ;
#79695=CARTESIAN_POINT('Ctrl Pts',(-19.8823207002362,13.4968164423014,124.531034373856)) ;
#79696=CARTESIAN_POINT('Ctrl Pts',(-19.89931310562,13.495936935673,124.523697697217)) ;
#79697=CARTESIAN_POINT('Ctrl Pts',(-19.9160308813858,13.4950607059879,124.516025186995)) ;
#79698=CARTESIAN_POINT('Ctrl Pts',(-19.9489281682582,13.4933364587125,124.50092719948)) ;
#79699=CARTESIAN_POINT('Ctrl Pts',(-19.9813803950063,13.4916076553557,124.484248940504)) ;
#79700=CARTESIAN_POINT('Ctrl Pts',(-20.0131369162587,13.489881514982,124.466058587158)) ;
#79701=CARTESIAN_POINT('Ctrl Pts',(-20.0426880424715,13.4882752498737,124.449131499229)) ;
#79702=CARTESIAN_POINT('Ctrl Pts',(-20.0716364343538,13.4866712907194,124.430895680783)) ;
#79703=CARTESIAN_POINT('Ctrl Pts',(-20.0997951305476,13.4850754545887,124.411443799838)) ;
#79704=CARTESIAN_POINT('Ctrl Pts',(-20.1579255419641,13.4817810332065,124.371287613829)) ;
#79705=CARTESIAN_POINT('Ctrl Pts',(-20.2124359544786,13.4784584750556,124.326139804631)) ;
#79706=CARTESIAN_POINT('Ctrl Pts',(-20.2626925415402,13.475090394799,124.276538949065)) ;
#79707=CARTESIAN_POINT('Ctrl Pts',(-20.3070989856034,13.4721143775988,124.232711905747)) ;
#79708=CARTESIAN_POINT('Ctrl Pts',(-20.3480830615047,13.4691715788273,124.185503789056)) ;
#79709=CARTESIAN_POINT('Ctrl Pts',(-20.385229376745,13.4662550237275,124.135400159535)) ;
#79710=CARTESIAN_POINT('Ctrl Pts',(-20.3902765523376,13.4658587430838,124.128592436767)) ;
#79711=CARTESIAN_POINT('Ctrl Pts',(-20.3952529375974,13.4654629469358,124.121731309245)) ;
#79712=CARTESIAN_POINT('Ctrl Pts',(-20.4001575465819,13.465067617788,124.114818043728)) ;
#79713=CARTESIAN_POINT('Ctrl Pts',(-20.4342018669983,13.462323522954,124.066831052892)) ;
#79714=CARTESIAN_POINT('Ctrl Pts',(-20.4647325078032,13.459550472373,124.016402693801)) ;
#79715=CARTESIAN_POINT('Ctrl Pts',(-20.4914654231896,13.4567592247756,123.96400951547)) ;
#79716=CARTESIAN_POINT('Ctrl Pts',(-20.4967440010575,13.4562080758426,123.953664161528)) ;
#79717=CARTESIAN_POINT('Ctrl Pts',(-20.501874650527,13.4556562174276,123.943242282805)) ;
#79718=CARTESIAN_POINT('Ctrl Pts',(-20.5068553925641,13.4551037323577,123.932747668806)) ;
#79719=CARTESIAN_POINT('Ctrl Pts',(-20.5318356253654,13.4523328187946,123.880113362731)) ;
#79720=CARTESIAN_POINT('Ctrl Pts',(-20.5530104114493,13.4495960832782,123.8257128765)) ;
#79721=CARTESIAN_POINT('Ctrl Pts',(-20.5701853289561,13.446858214099,123.77005238292)) ;
#79722=CARTESIAN_POINT('Ctrl Pts',(-20.5739111713719,13.4462642741797,123.75797766828)) ;
#79723=CARTESIAN_POINT('Ctrl Pts',(-20.5774489589816,13.4456702809093,123.745843724806)) ;
#79724=CARTESIAN_POINT('Ctrl Pts',(-20.5807970102927,13.4450758737854,123.733655833437)) ;
#79725=CARTESIAN_POINT('Ctrl Pts',(-20.5973713129412,13.4421333013296,123.673320497615)) ;
#79726=CARTESIAN_POINT('Ctrl Pts',(-20.6092661588775,13.4391667165855,123.611755506316)) ;
#79727=CARTESIAN_POINT('Ctrl Pts',(-20.6163604562517,13.4362229685556,123.549593065344)) ;
#79728=CARTESIAN_POINT('Ctrl Pts',(-20.6172697869142,13.4358456457278,123.541625227143)) ;
#79729=CARTESIAN_POINT('Ctrl Pts',(-20.6181003156493,13.4354686980963,123.533647586815)) ;
#79730=CARTESIAN_POINT('Ctrl Pts',(-20.6188518480512,13.4350922243203,123.525661488941)) ;
#79731=CARTESIAN_POINT('Ctrl Pts',(-20.6254307212966,13.4317965936244,123.455751628091)) ;
#79732=CARTESIAN_POINT('Ctrl Pts',(-20.6259390008459,13.4285013031375,123.385373714551)) ;
#79733=CARTESIAN_POINT('Ctrl Pts',(-20.6203564137095,13.4251593702564,123.315320856039)) ;
#79734=CARTESIAN_POINT('Ctrl Pts',(-20.6175374876002,13.4234718620055,123.279947681009)) ;
#79735=CARTESIAN_POINT('Ctrl Pts',(-20.613167621542,13.4217961608826,123.24474822006)) ;
#79736=CARTESIAN_POINT('Ctrl Pts',(-20.607312809919,13.4201356010657,123.209995955708)) ;
#79737=CARTESIAN_POINT('Ctrl Pts',(-20.601457998296,13.4184750412487,123.175243691355)) ;
#79738=CARTESIAN_POINT('Ctrl Pts',(-20.594118544722,13.4168296227376,123.140939361691)) ;
#79739=CARTESIAN_POINT('Ctrl Pts',(-20.5854193236931,13.4152026797105,123.107337652665)) ;
#79740=CARTESIAN_POINT('Ctrl Pts',(-20.5807421216615,13.4143279414774,123.089271439471)) ;
#79741=CARTESIAN_POINT('Ctrl Pts',(-20.5755898553748,13.4134404278288,123.071103158856)) ;
#79742=CARTESIAN_POINT('Ctrl Pts',(-20.5700329379717,13.4125540267447,123.053121430505)) ;
#79743=CARTESIAN_POINT('Ctrl Pts',(-20.5664270513197,13.4119788406107,123.041453077436)) ;
#79744=CARTESIAN_POINT('Ctrl Pts',(-20.5626518230741,13.4114041229464,123.029863049017)) ;
#79745=CARTESIAN_POINT('Ctrl Pts',(-20.558737719952,13.4108336684169,123.018426706518)) ;
#79746=CARTESIAN_POINT('Ctrl Pts',(-20.5518064668773,13.4098234843242,122.998174765872)) ;
#79747=CARTESIAN_POINT('Ctrl Pts',(-20.5442541788444,13.4087998151319,122.977868574445)) ;
#79748=CARTESIAN_POINT('Ctrl Pts',(-20.5361542599015,13.4077755235017,122.957766537256)) ;
#79749=CARTESIAN_POINT('Ctrl Pts',(-20.5297700128418,13.406968190629,122.941922382182)) ;
#79750=CARTESIAN_POINT('Ctrl Pts',(-20.5230465750099,13.4061604710741,122.926204877764)) ;
#79751=CARTESIAN_POINT('Ctrl Pts',(-20.5160412115277,13.4053586630578,122.910732285531)) ;
#79752=CARTESIAN_POINT('Ctrl Pts',(-20.5014374448478,13.4036871698909,122.87847726729)) ;
#79753=CARTESIAN_POINT('Ctrl Pts',(-20.4853106051582,13.4020080189064,122.846621324877)) ;
#79754=CARTESIAN_POINT('Ctrl Pts',(-20.4677249928207,13.400320627094,122.815412528442)) ;
#79755=CARTESIAN_POINT('Ctrl Pts',(-20.4508165739698,13.3986982140109,122.785405532278)) ;
#79756=CARTESIAN_POINT('Ctrl Pts',(-20.4325600323781,13.3970681825614,122.755997236008)) ;
#79757=CARTESIAN_POINT('Ctrl Pts',(-20.4130548688169,13.3954300145273,122.727391467059)) ;
#79758=CARTESIAN_POINT('Ctrl Pts',(-20.373208780757,13.3920834859253,122.668954223763)) ;
#79759=CARTESIAN_POINT('Ctrl Pts',(-20.3283321095217,13.388742198361,122.614105775861)) ;
#79760=CARTESIAN_POINT('Ctrl Pts',(-20.2789586274543,13.3854302875451,122.563489998466)) ;
#79761=CARTESIAN_POINT('Ctrl Pts',(-20.2347494510225,13.3824647918284,122.518168466757)) ;
#79762=CARTESIAN_POINT('Ctrl Pts',(-20.1870441586748,13.3794885282217,122.47635664903)) ;
#79763=CARTESIAN_POINT('Ctrl Pts',(-20.1363457553147,13.3764859557234,122.438485712437)) ;
#79764=CARTESIAN_POINT('Ctrl Pts',(-20.1306349606425,13.3761477384643,122.434219835632)) ;
#79765=CARTESIAN_POINT('Ctrl Pts',(-20.1248862229821,13.3758091873893,122.430003920129)) ;
#79766=CARTESIAN_POINT('Ctrl Pts',(-20.1191002882995,13.3754702802864,122.425838550793)) ;
#79767=CARTESIAN_POINT('Ctrl Pts',(-20.0721275737193,13.3727188861751,122.392022285028)) ;
#79768=CARTESIAN_POINT('Ctrl Pts',(-20.0227645008983,13.3699925972803,122.361586840403)) ;
#79769=CARTESIAN_POINT('Ctrl Pts',(-19.9714671039411,13.3672751518641,122.334810021739)) ;
#79770=CARTESIAN_POINT('Ctrl Pts',(-19.9599262553494,13.3666637831014,122.328785793838)) ;
#79771=CARTESIAN_POINT('Ctrl Pts',(-19.9482876062243,13.3660528619572,122.322946570311)) ;
#79772=CARTESIAN_POINT('Ctrl Pts',(-19.9365565347091,13.3654422032513,122.317295201679)) ;
#79773=CARTESIAN_POINT('Ctrl Pts',(-19.8838657555059,13.3626993947195,122.29191175598)) ;
#79774=CARTESIAN_POINT('Ctrl Pts',(-19.8293730012894,13.3599341452415,122.270352805618)) ;
#79775=CARTESIAN_POINT('Ctrl Pts',(-19.7735878256428,13.3571721468246,122.252817626186)) ;
#79776=CARTESIAN_POINT('Ctrl Pts',(-19.7621124657137,13.356603986456,122.24921052998)) ;
#79777=CARTESIAN_POINT('Ctrl Pts',(-19.7505824797019,13.3560359636562,122.245773535587)) ;
#79778=CARTESIAN_POINT('Ctrl Pts',(-19.7390024009182,13.3554683020607,122.242508122105)) ;
#79779=CARTESIAN_POINT('Ctrl Pts',(-19.6765654013214,13.3524076072702,122.224901797997)) ;
#79780=CARTESIAN_POINT('Ctrl Pts',(-19.6127730746103,13.349358790227,122.212316229204)) ;
#79781=CARTESIAN_POINT('Ctrl Pts',(-19.5483163855901,13.3462943624021,122.204890450701)) ;
#79782=CARTESIAN_POINT('Ctrl Pts',(-19.5427998573992,13.3460320932297,122.204254915165)) ;
#79783=CARTESIAN_POINT('Ctrl Pts',(-19.5372784701475,13.3457697097115,122.203657143319)) ;
#79784=CARTESIAN_POINT('Ctrl Pts',(-19.5317526615641,13.345507194615,122.203097205098)) ;
#79785=CARTESIAN_POINT('Ctrl Pts',(-19.4612306537588,13.3421568991061,122.195951107477)) ;
#79786=CARTESIAN_POINT('Ctrl Pts',(-19.390200308206,13.338828645327,122.194989532534)) ;
#79787=CARTESIAN_POINT('Ctrl Pts',(-19.3194902776855,13.3354839544011,122.200229114569)) ;
#79788=CARTESIAN_POINT('Ctrl Pts',(-19.2841463339745,13.333812132639,122.202848085189)) ;
#79789=CARTESIAN_POINT('Ctrl Pts',(-19.248961668752,13.3321383322381,122.207015164986)) ;
#79790=CARTESIAN_POINT('Ctrl Pts',(-19.2142000902938,13.3304754178574,122.212669876667)) ;
#79791=CARTESIAN_POINT('Ctrl Pts',(-19.1794385118355,13.3288125034767,122.218324588348)) ;
#79792=CARTESIAN_POINT('Ctrl Pts',(-19.1451007148001,13.3271604751162,122.225466660224)) ;
#79793=CARTESIAN_POINT('Ctrl Pts',(-19.111433296722,13.3255321974351,122.233979924988)) ;
#79794=CARTESIAN_POINT('Ctrl Pts',(-19.0924695578372,13.3246150426742,122.238775164399)) ;
#79795=CARTESIAN_POINT('Ctrl Pts',(-19.073423771037,13.3236891386708,122.244082894318)) ;
#79796=CARTESIAN_POINT('Ctrl Pts',(-19.0545747338385,13.3227643623052,122.249836486187)) ;
#79797=CARTESIAN_POINT('Ctrl Pts',(-19.0415327578809,13.3221244934886,122.253817496253)) ;
#79798=CARTESIAN_POINT('Ctrl Pts',(-19.028584767259,13.3214851645282,122.258010882909)) ;
#79799=CARTESIAN_POINT('Ctrl Pts',(-19.0158187797981,13.3208496471916,122.26238060356)) ;
#79800=CARTESIAN_POINT('Ctrl Pts',(-18.9963862256864,13.3198822543386,122.269032249839)) ;
#79801=CARTESIAN_POINT('Ctrl Pts',(-18.9768916946246,13.3188995497272,122.276260202074)) ;
#79802=CARTESIAN_POINT('Ctrl Pts',(-18.9575999785989,13.3179143486395,122.28398596407)) ;
#79803=CARTESIAN_POINT('Ctrl Pts',(-18.9432404840646,13.3171810292388,122.289736517157)) ;
#79804=CARTESIAN_POINT('Ctrl Pts',(-18.9289931167333,13.3164463267048,122.29576181833)) ;
#79805=CARTESIAN_POINT('Ctrl Pts',(-18.9149602389802,13.3157155258924,122.302011996755)) ;
#79806=CARTESIAN_POINT('Ctrl Pts',(-18.8831716085858,13.3140600452897,122.316170504749)) ;
#79807=CARTESIAN_POINT('Ctrl Pts',(-18.8517338620342,13.3123990969106,122.331814182501)) ;
#79808=CARTESIAN_POINT('Ctrl Pts',(-18.820896479701,13.3107371594226,122.348883552003)) ;
#79809=CARTESIAN_POINT('Ctrl Pts',(-18.7900590973678,13.3090752219345,122.365952921505)) ;
#79810=CARTESIAN_POINT('Ctrl Pts',(-18.7598227168092,13.3074122953375,122.384447785143)) ;
#79811=CARTESIAN_POINT('Ctrl Pts',(-18.7304179291922,13.3057528582991,122.404259215009)) ;
#79812=CARTESIAN_POINT('Ctrl Pts',(-18.6719105203943,13.3024510367574,122.443678490575)) ;
#79813=CARTESIAN_POINT('Ctrl Pts',(-18.6169579423831,13.2991176447074,122.488113239888)) ;
#79814=CARTESIAN_POINT('Ctrl Pts',(-18.5661897539316,13.2957819799608,122.537040991908)) ;
#79815=CARTESIAN_POINT('Ctrl Pts',(-18.5208952077543,13.2928059545105,122.580693530847)) ;
#79816=CARTESIAN_POINT('Ctrl Pts',(-18.4790410742417,13.2898555176067,122.627821648461)) ;
#79817=CARTESIAN_POINT('Ctrl Pts',(-18.4410561529531,13.2868881760101,122.677934110496)) ;
#79818=CARTESIAN_POINT('Ctrl Pts',(-18.4363890213519,13.28652358466,122.684091328867)) ;
#79819=CARTESIAN_POINT('Ctrl Pts',(-18.4317802523929,13.2861587381074,122.690293558696)) ;
#79820=CARTESIAN_POINT('Ctrl Pts',(-18.4272306008306,13.2857935575323,122.696539852779)) ;
#79821=CARTESIAN_POINT('Ctrl Pts',(-18.3928946404529,13.2830375605983,122.743680277318)) ;
#79822=CARTESIAN_POINT('Ctrl Pts',(-18.3619793344174,13.2802762462414,122.793264184408)) ;
#79823=CARTESIAN_POINT('Ctrl Pts',(-18.3347692281603,13.2775362339647,122.844828572947)) ;
#79824=CARTESIAN_POINT('Ctrl Pts',(-18.3289888657802,13.2769541611226,122.855782622478)) ;
#79825=CARTESIAN_POINT('Ctrl Pts',(-18.3233755523965,13.2763730496085,122.866825952029)) ;
#79826=CARTESIAN_POINT('Ctrl Pts',(-18.3179317557798,13.275793154619,122.877953967605)) ;
#79827=CARTESIAN_POINT('Ctrl Pts',(-18.2920118289675,13.2730320603415,122.930938560821)) ;
#79828=CARTESIAN_POINT('Ctrl Pts',(-18.2699705362575,13.2702660520453,122.985779701527)) ;
#79829=CARTESIAN_POINT('Ctrl Pts',(-18.2520148528673,13.2674654035193,123.041959006065)) ;
#79830=CARTESIAN_POINT('Ctrl Pts',(-18.2485203934141,13.2669203531024,123.052892385628)) ;
#79831=CARTESIAN_POINT('Ctrl Pts',(-18.2451805305577,13.2663739906762,123.063876390402)) ;
#79832=CARTESIAN_POINT('Ctrl Pts',(-18.2419965766553,13.265826097125,123.074907114232)) ;
#79833=CARTESIAN_POINT('Ctrl Pts',(-18.2247812063434,13.2628636828863,123.134549307986)) ;
#79834=CARTESIAN_POINT('Ctrl Pts',(-18.212156748074,13.259927864432,123.195458074127)) ;
#79835=CARTESIAN_POINT('Ctrl Pts',(-18.2042480633993,13.257032547975,123.257014734077)) ;
#79836=CARTESIAN_POINT('Ctrl Pts',(-18.2031228234541,13.2566206051722,123.265772955642)) ;
#79837=CARTESIAN_POINT('Ctrl Pts',(-18.2020929619901,13.2562094822643,123.274544276068)) ;
#79838=CARTESIAN_POINT('Ctrl Pts',(-18.2011587547338,13.255799219304,123.28332689543)) ;
#79839=CARTESIAN_POINT('Ctrl Pts',(-18.193725128791,13.2525346959724,123.35321150261)) ;
#79840=CARTESIAN_POINT('Ctrl Pts',(-18.1923663812627,13.2492233617159,123.423646288282)) ;
#79841=CARTESIAN_POINT('Ctrl Pts',(-18.197112972822,13.2458562753417,123.493822145477)) ;
#79842=CARTESIAN_POINT('Ctrl Pts',(-18.1995075328647,13.244157647939,123.52922445501)) ;
#79843=CARTESIAN_POINT('Ctrl Pts',(-18.2034542366403,13.24247686509,123.564473609004)) ;
#79844=CARTESIAN_POINT('Ctrl Pts',(-18.2088967701383,13.240815458859,123.59931931213)) ;
#79845=CARTESIAN_POINT('Ctrl Pts',(-18.2143393036362,13.239154052628,123.634165015255)) ;
#79846=CARTESIAN_POINT('Ctrl Pts',(-18.2212774273562,13.237512023015,123.668606637015)) ;
#79847=CARTESIAN_POINT('Ctrl Pts',(-18.2296037713618,13.235890902084,123.702409525742)) ;
#79848=CARTESIAN_POINT('Ctrl Pts',(-18.2344872337623,13.2349401026566,123.722235170229)) ;
#79849=CARTESIAN_POINT('Ctrl Pts',(-18.2399200625566,13.2339772581505,123.742120798444)) ;
#79850=CARTESIAN_POINT('Ctrl Pts',(-18.2458383478562,13.2330133138735,123.761795833979)) ;
#79851=CARTESIAN_POINT('Ctrl Pts',(-18.2502473234648,13.2322951993201,123.77645324696)) ;
#79852=CARTESIAN_POINT('Ctrl Pts',(-18.2549246370229,13.2315764744071,123.790993952581)) ;
#79853=CARTESIAN_POINT('Ctrl Pts',(-18.259825879779,13.2308616644972,123.80531165987)) ;
#79854=CARTESIAN_POINT('Ctrl Pts',(-18.259825879779,13.2488777185653,123.80531165987)) ;
#79855=CARTESIAN_POINT('Ctrl Pts',(-18.2541317465942,13.2497016709429,123.788677729199)) ;
#79856=CARTESIAN_POINT('Ctrl Pts',(-18.2487422399998,13.250529359594,123.771741871465)) ;
#79857=CARTESIAN_POINT('Ctrl Pts',(-18.2437569527338,13.2513511967269,123.754800233664)) ;
#79858=CARTESIAN_POINT('Ctrl Pts',(-18.2412772804615,13.251759976932,123.746373495694)) ;
#79859=CARTESIAN_POINT('Ctrl Pts',(-18.2388968414335,13.2521673094432,123.737945589492)) ;
#79860=CARTESIAN_POINT('Ctrl Pts',(-18.2366232729461,13.2525720143994,123.729554280879)) ;
#79861=CARTESIAN_POINT('Ctrl Pts',(-18.2282379267472,13.2540646420395,123.698605563838)) ;
#79862=CARTESIAN_POINT('Ctrl Pts',(-18.2209951205408,13.255586209498,123.667003461305)) ;
#79863=CARTESIAN_POINT('Ctrl Pts',(-18.215009722541,13.2571241718318,123.634968474936)) ;
#79864=CARTESIAN_POINT('Ctrl Pts',(-18.2090513348184,13.2586551938101,123.603078052698)) ;
#79865=CARTESIAN_POINT('Ctrl Pts',(-18.2043392572502,13.2602024630274,123.570759231022)) ;
#79866=CARTESIAN_POINT('Ctrl Pts',(-18.2009378272616,13.2617536036098,123.538246188677)) ;
#79867=CARTESIAN_POINT('Ctrl Pts',(-18.2004500251613,13.2619760540604,123.533583464354)) ;
#79868=CARTESIAN_POINT('Ctrl Pts',(-18.1999890932779,13.2621985841322,123.528916764725)) ;
#79869=CARTESIAN_POINT('Ctrl Pts',(-18.1995551349332,13.2624211573227,123.524246797382)) ;
#79870=CARTESIAN_POINT('Ctrl Pts',(-18.1930200675268,13.2657729324878,123.453920804724)) ;
#79871=CARTESIAN_POINT('Ctrl Pts',(-18.1926313247632,13.2690704371052,123.383157341937)) ;
#79872=CARTESIAN_POINT('Ctrl Pts',(-18.1983875184517,13.2724062706453,123.312786261935)) ;
#79873=CARTESIAN_POINT('Ctrl Pts',(-18.2036324476591,13.2754458158226,123.248665533407)) ;
#79874=CARTESIAN_POINT('Ctrl Pts',(-18.213969116443,13.2784896509119,123.185031555617)) ;
#79875=CARTESIAN_POINT('Ctrl Pts',(-18.2292826636117,13.2815090524663,123.122564517586)) ;
#79876=CARTESIAN_POINT('Ctrl Pts',(-18.230849736092,13.2818180351619,123.116172113844)) ;
#79877=CARTESIAN_POINT('Ctrl Pts',(-18.232468881758,13.2821267619913,123.109791922641)) ;
#79878=CARTESIAN_POINT('Ctrl Pts',(-18.2341399470166,13.282435202174,123.10342466848)) ;
#79879=CARTESIAN_POINT('Ctrl Pts',(-18.2492276240946,13.2852200400791,123.045936144818)) ;
#79880=CARTESIAN_POINT('Ctrl Pts',(-18.268526186191,13.2880215829812,122.98960118557)) ;
#79881=CARTESIAN_POINT('Ctrl Pts',(-18.2918470092261,13.2908335603714,122.93495572258)) ;
#79882=CARTESIAN_POINT('Ctrl Pts',(-18.296154129185,13.2913529041323,122.924863258693)) ;
#79883=CARTESIAN_POINT('Ctrl Pts',(-18.3005983157538,13.2918726038172,122.914828374478)) ;
#79884=CARTESIAN_POINT('Ctrl Pts',(-18.3051781978976,13.292392619923,122.904854379638)) ;
#79885=CARTESIAN_POINT('Ctrl Pts',(-18.3294212425568,13.2951452614277,122.852058260708)) ;
#79886=CARTESIAN_POINT('Ctrl Pts',(-18.3574408850354,13.2978714559953,122.801033976254)) ;
#79887=CARTESIAN_POINT('Ctrl Pts',(-18.3889760997798,13.3006089004558,122.75225273517)) ;
#79888=CARTESIAN_POINT('Ctrl Pts',(-18.395950847592,13.3012143501068,122.741463626636)) ;
#79889=CARTESIAN_POINT('Ctrl Pts',(-18.403097392957,13.301820350076,122.730784143262)) ;
#79890=CARTESIAN_POINT('Ctrl Pts',(-18.4104126119089,13.3024273082157,122.720219213702)) ;
#79891=CARTESIAN_POINT('Ctrl Pts',(-18.4448681629127,13.3052861532175,122.670457139358)) ;
#79892=CARTESIAN_POINT('Ctrl Pts',(-18.4830184064348,13.3081529411829,122.623312068044)) ;
#79893=CARTESIAN_POINT('Ctrl Pts',(-18.5244875760069,13.3109950558311,122.579243361395)) ;
#79894=CARTESIAN_POINT('Ctrl Pts',(-18.5316297482361,13.3114845489298,122.571653474834)) ;
#79895=CARTESIAN_POINT('Ctrl Pts',(-18.5388702725273,13.3119733101524,122.564154761581)) ;
#79896=CARTESIAN_POINT('Ctrl Pts',(-18.5462071080853,13.3124611728706,122.556749469826)) ;
#79897=CARTESIAN_POINT('Ctrl Pts',(-18.5956168411068,13.315746671975,122.506878720283)) ;
#79898=CARTESIAN_POINT('Ctrl Pts',(-18.649288677809,13.3190556659508,122.461354165491)) ;
#79899=CARTESIAN_POINT('Ctrl Pts',(-18.7066052679516,13.3223924544114,122.420718788959)) ;
#79900=CARTESIAN_POINT('Ctrl Pts',(-18.7382703284698,13.3242358929042,122.398269413415)) ;
#79901=CARTESIAN_POINT('Ctrl Pts',(-18.7709693636302,13.3260622110372,122.377372531742)) ;
#79902=CARTESIAN_POINT('Ctrl Pts',(-18.8044599660106,13.3278792028658,122.35814909333)) ;
#79903=CARTESIAN_POINT('Ctrl Pts',(-18.8321965201051,13.3293840158152,122.342228449882)) ;
#79904=CARTESIAN_POINT('Ctrl Pts',(-18.8604753323463,13.3308824318777,122.327454862663)) ;
#79905=CARTESIAN_POINT('Ctrl Pts',(-18.889148703445,13.3323788784877,122.313871857645)) ;
#79906=CARTESIAN_POINT('Ctrl Pts',(-18.9106960849462,13.3335034238329,122.303664540547)) ;
#79907=CARTESIAN_POINT('Ctrl Pts',(-18.9326603708187,13.334638759352,122.294041202817)) ;
#79908=CARTESIAN_POINT('Ctrl Pts',(-18.9548108444622,13.3357694147718,122.285106935635)) ;
#79909=CARTESIAN_POINT('Ctrl Pts',(-18.9751066148332,13.3368053981615,122.276920752438)) ;
#79910=CARTESIAN_POINT('Ctrl Pts',(-18.9955581376258,13.3378374523875,122.269312619075)) ;
#79911=CARTESIAN_POINT('Ctrl Pts',(-19.0159746201976,13.3388536769403,122.262327272131)) ;
#79912=CARTESIAN_POINT('Ctrl Pts',(-19.0310757895312,13.3396053333041,122.257160519891)) ;
#79913=CARTESIAN_POINT('Ctrl Pts',(-19.0465094020696,13.340366364494,122.252217020429)) ;
#79914=CARTESIAN_POINT('Ctrl Pts',(-19.0619560302779,13.3411223178931,122.247608954491)) ;
#79915=CARTESIAN_POINT('Ctrl Pts',(-19.0697273679117,13.34150264485,122.245290595057)) ;
#79916=CARTESIAN_POINT('Ctrl Pts',(-19.0775017289523,13.3418816865233,122.243056359391)) ;
#79917=CARTESIAN_POINT('Ctrl Pts',(-19.0852370091252,13.342257602426,122.24091574547)) ;
#79918=CARTESIAN_POINT('Ctrl Pts',(-19.1156522742549,13.3437357107289,122.232498811823)) ;
#79919=CARTESIAN_POINT('Ctrl Pts',(-19.1467267842854,13.34523529048,122.225179703659)) ;
#79920=CARTESIAN_POINT('Ctrl Pts',(-19.1782417556261,13.3467486313542,122.219075501309)) ;
#79921=CARTESIAN_POINT('Ctrl Pts',(-19.2096032257156,13.3482546011375,122.213001030944)) ;
#79922=CARTESIAN_POINT('Ctrl Pts',(-19.2414002980428,13.3497741983166,122.208129889525)) ;
#79923=CARTESIAN_POINT('Ctrl Pts',(-19.2734003828313,13.3512998246835,122.204528622569)) ;
#79924=CARTESIAN_POINT('Ctrl Pts',(-19.2789378517144,13.3515638273757,122.203905439729)) ;
#79925=CARTESIAN_POINT('Ctrl Pts',(-19.2844813710085,13.3518280106103,122.203320159961)) ;
#79926=CARTESIAN_POINT('Ctrl Pts',(-19.290029704004,13.3520923350148,122.202772972482)) ;
#79927=CARTESIAN_POINT('Ctrl Pts',(-19.360440713544,13.3554467386142,122.19582890067)) ;
#79928=CARTESIAN_POINT('Ctrl Pts',(-19.4313297110453,13.3587503674759,122.19504973569)) ;
#79929=CARTESIAN_POINT('Ctrl Pts',(-19.5018619235022,13.3620953493016,122.200440834737)) ;
#79930=CARTESIAN_POINT('Ctrl Pts',(-19.5670909451669,13.3651888279318,122.205426586697)) ;
#79931=CARTESIAN_POINT('Ctrl Pts',(-19.6318412542396,13.3682908758495,122.215679365529)) ;
#79932=CARTESIAN_POINT('Ctrl Pts',(-19.6954027317278,13.3713529115821,122.231082305476)) ;
#79933=CARTESIAN_POINT('Ctrl Pts',(-19.7007491392792,13.3716104715321,122.232377907744)) ;
#79934=CARTESIAN_POINT('Ctrl Pts',(-19.7060871405538,13.3718677483895,122.233709918135)) ;
#79935=CARTESIAN_POINT('Ctrl Pts',(-19.711416315147,13.3721247132427,122.235078250401)) ;
#79936=CARTESIAN_POINT('Ctrl Pts',(-19.769383977558,13.3749198274948,122.249962173134)) ;
#79937=CARTESIAN_POINT('Ctrl Pts',(-19.826202342528,13.3777373491628,122.269121127388)) ;
#79938=CARTESIAN_POINT('Ctrl Pts',(-19.881325845597,13.3805764700006,122.29236555184)) ;
#79939=CARTESIAN_POINT('Ctrl Pts',(-19.8908402239965,13.3810665054386,122.296377565547)) ;
#79940=CARTESIAN_POINT('Ctrl Pts',(-19.9003041537587,13.3815571843407,122.300511172329)) ;
#79941=CARTESIAN_POINT('Ctrl Pts',(-19.909714882751,13.3820485025508,122.304765249621)) ;
#79942=CARTESIAN_POINT('Ctrl Pts',(-19.9625480806773,13.3848068342658,122.328648256744)) ;
#79943=CARTESIAN_POINT('Ctrl Pts',(-20.0136392374553,13.3875266827007,122.356303461624)) ;
#79944=CARTESIAN_POINT('Ctrl Pts',(-20.0625177211307,13.3902529020074,122.387473933324)) ;
#79945=CARTESIAN_POINT('Ctrl Pts',(-20.0734076217942,13.3908602910916,122.394418570615)) ;
#79946=CARTESIAN_POINT('Ctrl Pts',(-20.0841877897517,13.3914679964118,122.40153751896)) ;
#79947=CARTESIAN_POINT('Ctrl Pts',(-20.094853191974,13.3920765140131,122.408827629049)) ;
#79948=CARTESIAN_POINT('Ctrl Pts',(-20.1447883901869,13.3949255811559,122.442959777532)) ;
#79949=CARTESIAN_POINT('Ctrl Pts',(-20.1921329756688,13.3977924704886,122.480797749689)) ;
#79950=CARTESIAN_POINT('Ctrl Pts',(-20.2364258868668,13.4006366507319,122.521969374432)) ;
#79951=CARTESIAN_POINT('Ctrl Pts',(-20.2440550764245,13.4011265438011,122.529060941029)) ;
#79952=CARTESIAN_POINT('Ctrl Pts',(-20.2515938080061,13.401615763137,122.536251313755)) ;
#79953=CARTESIAN_POINT('Ctrl Pts',(-20.2590398232441,13.402104101619,122.543538468909)) ;
#79954=CARTESIAN_POINT('Ctrl Pts',(-20.3092384544237,13.4053963220306,122.592666116681)) ;
#79955=CARTESIAN_POINT('Ctrl Pts',(-20.3551122685804,13.4087006073066,122.646087327709)) ;
#79956=CARTESIAN_POINT('Ctrl Pts',(-20.3961083195075,13.4120397603772,122.703176251959)) ;
#79957=CARTESIAN_POINT('Ctrl Pts',(-20.4194907060249,13.4139442698597,122.735737322171)) ;
#79958=CARTESIAN_POINT('Ctrl Pts',(-20.4412263130121,13.4158353105015,122.769414004562)) ;
#79959=CARTESIAN_POINT('Ctrl Pts',(-20.4611878719886,13.4177137178806,122.803957082543)) ;
#79960=CARTESIAN_POINT('Ctrl Pts',(-20.4764077561463,13.419145927797,122.830294787226)) ;
#79961=CARTESIAN_POINT('Ctrl Pts',(-20.4905971960194,13.4205707934319,122.857135520827)) ;
#79962=CARTESIAN_POINT('Ctrl Pts',(-20.5037186695672,13.4219886851572,122.884361176354)) ;
#79963=CARTESIAN_POINT('Ctrl Pts',(-20.5144322700877,13.4231463848218,122.906590752641)) ;
#79964=CARTESIAN_POINT('Ctrl Pts',(-20.5245108043189,13.424312442704,122.929244377532)) ;
#79965=CARTESIAN_POINT('Ctrl Pts',(-20.533852008639,13.4254760024545,122.952094174275)) ;
#79966=CARTESIAN_POINT('Ctrl Pts',(-20.5428664550124,13.4265988605586,122.97414467872)) ;
#79967=CARTESIAN_POINT('Ctrl Pts',(-20.5511944078365,13.427719392245,122.996377332141)) ;
#79968=CARTESIAN_POINT('Ctrl Pts',(-20.5587873005049,13.4288278410515,123.018571602254)) ;
#79969=CARTESIAN_POINT('Ctrl Pts',(-20.5635331084435,13.4295206580548,123.032443751895)) ;
#79970=CARTESIAN_POINT('Ctrl Pts',(-20.568102944472,13.4302253268598,123.04663484588)) ;
#79971=CARTESIAN_POINT('Ctrl Pts',(-20.5723778495344,13.4309244835595,123.060799202518)) ;
#79972=CARTESIAN_POINT('Ctrl Pts',(-20.5742105953237,13.4312242274085,123.06687177363)) ;
#79973=CARTESIAN_POINT('Ctrl Pts',(-20.5759897537802,13.4315229581185,123.072939221501)) ;
#79974=CARTESIAN_POINT('Ctrl Pts',(-20.5777087635802,13.4318193074104,123.078973461537)) ;
#79975=CARTESIAN_POINT('Ctrl Pts',(-20.5862099243874,13.4332848679824,123.108815085998)) ;
#79976=CARTESIAN_POINT('Ctrl Pts',(-20.5936629775568,13.4347626950335,123.139331795925)) ;
#79977=CARTESIAN_POINT('Ctrl Pts',(-20.5999462560564,13.4362509313631,123.17030707295)) ;
#79978=CARTESIAN_POINT('Ctrl Pts',(-20.6061951543524,13.4377310245127,123.201112862608)) ;
#79979=CARTESIAN_POINT('Ctrl Pts',(-20.6112868051342,13.4392214133396,123.232371646335)) ;
#79980=CARTESIAN_POINT('Ctrl Pts',(-20.6151500417308,13.4407202709629,123.263852742209)) ;
#79981=CARTESIAN_POINT('Ctrl Pts',(-20.6160279965581,13.4410608996697,123.271007100841)) ;
#79982=CARTESIAN_POINT('Ctrl Pts',(-20.6168427143569,13.4414019657611,123.278172888928)) ;
#79983=CARTESIAN_POINT('Ctrl Pts',(-20.6175937276234,13.4417434477945,123.285347319404)) ;
#79984=CARTESIAN_POINT('Ctrl Pts',(-20.6249761933209,13.4451002185878,123.355872021493)) ;
#79985=CARTESIAN_POINT('Ctrl Pts',(-20.6261691568536,13.4484538465774,123.426893770811)) ;
#79986=CARTESIAN_POINT('Ctrl Pts',(-20.621164396608,13.4517681683501,123.497606568652)) ;
#79987=CARTESIAN_POINT('Ctrl Pts',(-20.6164600480809,13.4548835473062,123.564074816888)) ;
#79988=CARTESIAN_POINT('Ctrl Pts',(-20.6062896907596,13.4580234506368,123.630062366585)) ;
#79989=CARTESIAN_POINT('Ctrl Pts',(-20.5907777971686,13.4611842724295,123.694825471852)) ;
#79990=CARTESIAN_POINT('Ctrl Pts',(-20.5899123609554,13.4613606203155,123.698438721018)) ;
#79991=CARTESIAN_POINT('Ctrl Pts',(-20.5890303112337,13.4615370333149,123.702048161313)) ;
#79992=CARTESIAN_POINT('Ctrl Pts',(-20.5881316743378,13.4617135108015,123.705653664296)) ;
#79993=CARTESIAN_POINT('Ctrl Pts',(-20.5740434312057,13.4644802097312,123.762178388433)) ;
#79994=CARTESIAN_POINT('Ctrl Pts',(-20.5558944562323,13.4672125201831,123.817653148817)) ;
#79995=CARTESIAN_POINT('Ctrl Pts',(-20.5338558989619,13.4699542231989,123.871563619345)) ;
#79996=CARTESIAN_POINT('Ctrl Pts',(-20.5290538725615,13.4705516184868,123.88331028223)) ;
#79997=CARTESIAN_POINT('Ctrl Pts',(-20.5240673663107,13.4711494597049,123.894982741291)) ;
#79998=CARTESIAN_POINT('Ctrl Pts',(-20.5188984612438,13.4717481997614,123.906575782835)) ;
#79999=CARTESIAN_POINT('Ctrl Pts',(-20.4954340221929,13.4744662027781,123.959202831152)) ;
#80000=CARTESIAN_POINT('Ctrl Pts',(-20.468235883307,13.4771958570766,124.010126937028)) ;
#80001=CARTESIAN_POINT('Ctrl Pts',(-20.4375558260374,13.479905711605,124.058883431865)) ;
#80002=CARTESIAN_POINT('Ctrl Pts',(-20.4305098026622,13.4805280604547,124.070080914298)) ;
#80003=CARTESIAN_POINT('Ctrl Pts',(-20.4232803172227,13.4811493649787,124.081164173257)) ;
#80004=CARTESIAN_POINT('Ctrl Pts',(-20.4158707580077,13.4817692441999,124.092127770366)) ;
#80005=CARTESIAN_POINT('Ctrl Pts',(-20.3808596839067,13.4846982493829,124.143932108473)) ;
#80006=CARTESIAN_POINT('Ctrl Pts',(-20.3418719851168,13.4876453239122,124.192992666741)) ;
#80007=CARTESIAN_POINT('Ctrl Pts',(-20.299305823346,13.4906079428639,124.238804928216)) ;
#80008=CARTESIAN_POINT('Ctrl Pts',(-20.2941076490582,13.4909697375153,124.244399515789)) ;
#80009=CARTESIAN_POINT('Ctrl Pts',(-20.2888561590993,13.4913317639848,124.249945699095)) ;
#80010=CARTESIAN_POINT('Ctrl Pts',(-20.2835521217904,13.4916940176739,124.255442590736)) ;
#80011=CARTESIAN_POINT('Ctrl Pts',(-20.2344266246723,13.4950491774371,124.306354286624)) ;
#80012=CARTESIAN_POINT('Ctrl Pts',(-20.1809262171979,13.4983581432627,124.352897140689)) ;
#80013=CARTESIAN_POINT('Ctrl Pts',(-20.1236843419261,13.5016986778291,124.394512406366)) ;
#80014=CARTESIAN_POINT('Ctrl Pts',(-20.0904562899518,13.503637808154,124.418669445322)) ;
#80015=CARTESIAN_POINT('Ctrl Pts',(-20.0560448598183,13.5055781736,124.44110534709)) ;
#80016=CARTESIAN_POINT('Ctrl Pts',(-20.0207051752874,13.5075076020376,124.461687207213)) ;
#80017=CARTESIAN_POINT('Ctrl Pts',(-19.9950132719789,13.5089102939268,124.476650191948)) ;
#80018=CARTESIAN_POINT('Ctrl Pts',(-19.9688313835272,13.5103072053112,124.490634187891)) ;
#80019=CARTESIAN_POINT('Ctrl Pts',(-19.9422641111465,13.5116936591906,124.503604138563)) ;
#80020=CARTESIAN_POINT('Ctrl Pts',(-19.9195299530059,13.512880076121,124.514702790522)) ;
#80021=CARTESIAN_POINT('Ctrl Pts',(-19.8963628780932,13.5140730034568,124.52512850839)) ;
#80022=CARTESIAN_POINT('Ctrl Pts',(-19.8729916778398,13.515263555876,124.534779676322)) ;
#80023=CARTESIAN_POINT('Ctrl Pts',(-19.8496204775865,13.5164541082953,124.544430844253)) ;
#80024=CARTESIAN_POINT('Ctrl Pts',(-19.826045673914,13.5176422857981,124.553307341802)) ;
#80025=CARTESIAN_POINT('Ctrl Pts',(-19.8025139576554,13.5188192030627,124.561357383308)) ;
#80026=CARTESIAN_POINT('Ctrl Pts',(-19.7895816065837,13.5194660027725,124.565781453434)) ;
#80027=CARTESIAN_POINT('Ctrl Pts',(-19.7763375942247,13.520125198213,124.570063774942)) ;
#80028=CARTESIAN_POINT('Ctrl Pts',(-19.7631512999327,13.5207777077975,124.574078752279)) ;
#80029=CARTESIAN_POINT('Ctrl Pts',(-19.7583580644925,13.5210148958957,124.575538201858)) ;
#80030=CARTESIAN_POINT('Ctrl Pts',(-19.7535726125751,13.5212512005702,124.576962802294)) ;
#80031=CARTESIAN_POINT('Ctrl Pts',(-19.7488131806747,13.5214857053212,124.578348155295)) ;
#80032=CARTESIAN_POINT('Ctrl Pts',(-19.7194810128453,13.5229309477061,124.58688602443)) ;
#80033=CARTESIAN_POINT('Ctrl Pts',(-19.689468046598,13.5243872978826,124.594417550275)) ;
#80034=CARTESIAN_POINT('Ctrl Pts',(-19.6589894692077,13.5258535219998,124.600818895649)) ;
#80035=CARTESIAN_POINT('Ctrl Pts',(-19.628689447621,13.5273111563845,124.607182739358)) ;
#80036=CARTESIAN_POINT('Ctrl Pts',(-19.597929815092,13.5287785493577,124.61242936282)) ;
#80037=CARTESIAN_POINT('Ctrl Pts',(-19.5669400142052,13.5302544886269,124.616485450686)) ;
#80038=CARTESIAN_POINT('Ctrl Pts',(-19.5590953627818,13.5306281028082,124.617512194794)) ;
#80039=CARTESIAN_POINT('Ctrl Pts',(-19.5512360288153,13.5310022646201,124.618462903704)) ;
#80040=CARTESIAN_POINT('Ctrl Pts',(-19.5433658496564,13.5313769543985,124.619336906487)) ;
#80041=CARTESIAN_POINT('Ctrl Pts',(-19.4728496206335,13.534734147379,124.627167907427)) ;
#80042=CARTESIAN_POINT('Ctrl Pts',(-19.40179126521,13.5380934253591,124.628806009374)) ;
#80043=CARTESIAN_POINT('Ctrl Pts',(-19.3310038383664,13.5414077514449,124.624236377072)) ;
#80044=CARTESIAN_POINT('Ctrl Pts',(-19.2641668580587,13.5445371143447,124.619921763055)) ;
#80045=CARTESIAN_POINT('Ctrl Pts',(-19.1977803711769,13.5476779798217,124.610082037491)) ;
#80046=CARTESIAN_POINT('Ctrl Pts',(-19.132598939239,13.5508697467509,124.594837974479)) ;
#80047=CARTESIAN_POINT('Ctrl Pts',(-19.1291457887477,13.5510388386412,124.594030381855)) ;
#80048=CARTESIAN_POINT('Ctrl Pts',(-19.1256960182946,13.5512080733925,124.593207633271)) ;
#80049=CARTESIAN_POINT('Ctrl Pts',(-19.1222497395156,13.5513774568627,124.592369750726)) ;
#80050=CARTESIAN_POINT('Ctrl Pts',(-19.0653270435142,13.5541751886781,124.578530320871)) ;
#80051=CARTESIAN_POINT('Ctrl Pts',(-19.009444848784,13.5569465950344,124.560579032738)) ;
#80052=CARTESIAN_POINT('Ctrl Pts',(-18.9551249662201,13.5596834935631,124.538687022647)) ;
#80053=CARTESIAN_POINT('Ctrl Pts',(-18.9436985177004,13.5602592133302,124.534081933047)) ;
#80054=CARTESIAN_POINT('Ctrl Pts',(-18.9323411408641,13.5608334061555,124.529302643614)) ;
#80055=CARTESIAN_POINT('Ctrl Pts',(-18.9210575982544,13.5614059958772,124.524351025318)) ;
#80056=CARTESIAN_POINT('Ctrl Pts',(-18.867195164181,13.5641392754157,124.500714280794)) ;
#80057=CARTESIAN_POINT('Ctrl Pts',(-18.8150850440426,13.5669062015152,124.473176883449)) ;
#80058=CARTESIAN_POINT('Ctrl Pts',(-18.7652166588985,13.5697062433898,124.441999493491)) ;
#80059=CARTESIAN_POINT('Ctrl Pts',(-18.7554793384308,13.5702529806658,124.435911784084)) ;
#80060=CARTESIAN_POINT('Ctrl Pts',(-18.7458274121111,13.5708009805345,124.429685434137)) ;
#80061=CARTESIAN_POINT('Ctrl Pts',(-18.7362644137408,13.5713502390443,124.423322588574)) ;
#80062=CARTESIAN_POINT('Ctrl Pts',(-18.6856315360648,13.5742583791341,124.389633449605)) ;
#80063=CARTESIAN_POINT('Ctrl Pts',(-18.6375717516268,13.5771200435325,124.352166199987)) ;
#80064=CARTESIAN_POINT('Ctrl Pts',(-18.592556707396,13.5799635694306,124.311292316254)) ;
#80065=CARTESIAN_POINT('Ctrl Pts',(-18.5850880158292,13.5804353543251,124.304510707218)) ;
#80066=CARTESIAN_POINT('Ctrl Pts',(-18.5777030672295,13.5809066399041,124.297635411384)) ;
#80067=CARTESIAN_POINT('Ctrl Pts',(-18.5704039303823,13.5813775555924,124.290668234917)) ;
#80068=CARTESIAN_POINT('Ctrl Pts',(-18.5194585604116,13.5846643790162,124.242039829913)) ;
#80069=CARTESIAN_POINT('Ctrl Pts',(-18.4728077112974,13.5879998975297,124.189040152522)) ;
#80070=CARTESIAN_POINT('Ctrl Pts',(-18.4310222353521,13.5913395370313,124.132304274245)) ;
#80071=CARTESIAN_POINT('Ctrl Pts',(-18.4054964725353,13.5933796441231,124.097645662866)) ;
#80072=CARTESIAN_POINT('Ctrl Pts',(-18.3818506872119,13.5954070301464,124.061674949715)) ;
#80073=CARTESIAN_POINT('Ctrl Pts',(-18.3602282781819,13.5974254310589,124.024661623705)) ;
#80074=CARTESIAN_POINT('Ctrl Pts',(-18.3464060730839,13.5987157013218,124.001000717894)) ;
#80075=CARTESIAN_POINT('Ctrl Pts',(-18.3334097938057,13.6000022998613,123.976914292308)) ;
#80076=CARTESIAN_POINT('Ctrl Pts',(-18.3212665887893,13.6012862026144,123.952477029753)) ;
#80077=CARTESIAN_POINT('Ctrl Pts',(-18.3101238971397,13.6024643209503,123.930053223102)) ;
#80078=CARTESIAN_POINT('Ctrl Pts',(-18.2996490228853,13.6036459044671,123.907224022409)) ;
#80079=CARTESIAN_POINT('Ctrl Pts',(-18.2899392691066,13.6048221127595,123.884216358921)) ;
#80080=CARTESIAN_POINT('Ctrl Pts',(-18.2801672790814,13.6060058601504,123.861061224072)) ;
#80081=CARTESIAN_POINT('Ctrl Pts',(-18.2711704023844,13.6071841631893,123.8377258344)) ;
#80082=CARTESIAN_POINT('Ctrl Pts',(-18.2629980370417,13.6083480103872,123.814459176388)) ;
#80083=CARTESIAN_POINT('Ctrl Pts',(-18.2619265327424,13.6085006060219,123.811408612316)) ;
#80084=CARTESIAN_POINT('Ctrl Pts',(-18.2608691312784,13.6086529531512,123.808359248072)) ;
#80085=CARTESIAN_POINT('Ctrl Pts',(-18.259825879779,13.6088050314641,123.80531165987)) ;
#80086=CARTESIAN_POINT('Origin',(-19.4092696390626,-30.19753203383,123.411833654984)) ;
#80087=CARTESIAN_POINT('',(-18.259825879779,12.870840300276,123.80531165987)) ;
#80088=CARTESIAN_POINT('',(-18.259825879779,12.8888247888664,123.80531165987)) ;
#80089=CARTESIAN_POINT('',(-18.259825879779,-30.19753203383,123.80531165987)) ;
#80090=CARTESIAN_POINT('Ctrl Pts',(-18.259825879779,13.2308616644972,123.80531165987)) ;
#80091=CARTESIAN_POINT('Ctrl Pts',(-18.2662155410734,13.229929779781,123.823977395204)) ;
#80092=CARTESIAN_POINT('Ctrl Pts',(-18.2731402046744,13.2289823495695,123.842708806219)) ;
#80093=CARTESIAN_POINT('Ctrl Pts',(-18.2805158878487,13.2280348698646,123.861234217073)) ;
#80094=CARTESIAN_POINT('Ctrl Pts',(-18.2856172109641,13.2273795542814,123.874047146313)) ;
#80095=CARTESIAN_POINT('Ctrl Pts',(-18.2909332321475,13.2267242150223,123.886761815414)) ;
#80096=CARTESIAN_POINT('Ctrl Pts',(-18.2964225629164,13.2260739790644,123.899293685344)) ;
#80097=CARTESIAN_POINT('Ctrl Pts',(-18.3103610748771,13.2244228995324,123.931114616938)) ;
#80098=CARTESIAN_POINT('Ctrl Pts',(-18.3257931498652,13.2227693158545,123.962619901958)) ;
#80099=CARTESIAN_POINT('Ctrl Pts',(-18.342659690849,13.2211109075677,123.993545881482)) ;
#80100=CARTESIAN_POINT('Ctrl Pts',(-18.3595262318327,13.2194524992809,124.024471861005)) ;
#80101=CARTESIAN_POINT('Ctrl Pts',(-18.3778270305652,13.2177892663854,124.054817831129)) ;
#80102=CARTESIAN_POINT('Ctrl Pts',(-18.3974491913048,13.2161188884183,124.084340366909)) ;
#80103=CARTESIAN_POINT('Ctrl Pts',(-18.4365917331541,13.2127867966906,124.143232305857)) ;
#80104=CARTESIAN_POINT('Ctrl Pts',(-18.4807968336201,13.2094316614767,124.198586925243)) ;
#80105=CARTESIAN_POINT('Ctrl Pts',(-18.5295493467101,13.2061226175737,124.249770468418)) ;
#80106=CARTESIAN_POINT('Ctrl Pts',(-18.5738592237391,13.2031151145931,124.296289844759)) ;
#80107=CARTESIAN_POINT('Ctrl Pts',(-18.6218081637929,13.2001058428464,124.339234964246)) ;
#80108=CARTESIAN_POINT('Ctrl Pts',(-18.6728787352241,13.1970492393281,124.378153650032)) ;
#80109=CARTESIAN_POINT('Ctrl Pts',(-18.6776608816052,13.1967630250751,124.381797918094)) ;
#80110=CARTESIAN_POINT('Ctrl Pts',(-18.6824703744847,13.1964763958135,124.385406910975)) ;
#80111=CARTESIAN_POINT('Ctrl Pts',(-18.6873067735839,13.196189314135,124.388980274973)) ;
#80112=CARTESIAN_POINT('Ctrl Pts',(-18.7337853611335,13.1934304121803,124.42332088831)) ;
#80113=CARTESIAN_POINT('Ctrl Pts',(-18.7826889633777,13.1907006475101,124.454321374326)) ;
#80114=CARTESIAN_POINT('Ctrl Pts',(-18.8335667710696,13.1879971448032,124.481699115624)) ;
#80115=CARTESIAN_POINT('Ctrl Pts',(-18.8451091827042,13.1873838137161,124.487910176478)) ;
#80116=CARTESIAN_POINT('Ctrl Pts',(-18.8567530918386,13.1867718342768,124.493934963064)) ;
#80117=CARTESIAN_POINT('Ctrl Pts',(-18.8684930404656,13.1861611729122,124.499770494371)) ;
#80118=CARTESIAN_POINT('Ctrl Pts',(-18.921426430588,13.1834078068394,124.526081891895)) ;
#80119=CARTESIAN_POINT('Ctrl Pts',(-18.9762487783818,13.1806156356083,124.54850969572)) ;
#80120=CARTESIAN_POINT('Ctrl Pts',(-19.0324403858194,13.1778111404927,124.566842577021)) ;
#80121=CARTESIAN_POINT('Ctrl Pts',(-19.0431186301153,13.1772781946431,124.570326424416)) ;
#80122=CARTESIAN_POINT('Ctrl Pts',(-19.0538462651928,13.1767448037479,124.573662534302)) ;
#80123=CARTESIAN_POINT('Ctrl Pts',(-19.0646196442166,13.1762111495361,124.576849653646)) ;
#80124=CARTESIAN_POINT('Ctrl Pts',(-19.1256125949851,13.1731898926963,124.594893371665)) ;
#80125=CARTESIAN_POINT('Ctrl Pts',(-19.1879673326654,13.1702142455434,124.608126440509)) ;
#80126=CARTESIAN_POINT('Ctrl Pts',(-19.2510277607696,13.1672162128466,124.616410511826)) ;
#80127=CARTESIAN_POINT('Ctrl Pts',(-19.2583148370614,13.1668697690681,124.617367794571)) ;
#80128=CARTESIAN_POINT('Ctrl Pts',(-19.2656113243022,13.1665230263658,124.618259047039)) ;
#80129=CARTESIAN_POINT('Ctrl Pts',(-19.2729161992964,13.1661758798175,124.619084099403)) ;
#80130=CARTESIAN_POINT('Ctrl Pts',(-19.3434354710218,13.1628246216797,124.627048929993)) ;
#80131=CARTESIAN_POINT('Ctrl Pts',(-19.4145457118438,13.1594555857011,124.628819748298)) ;
#80132=CARTESIAN_POINT('Ctrl Pts',(-19.4853787873511,13.1561418975459,124.624373672316)) ;
#80133=CARTESIAN_POINT('Ctrl Pts',(-19.5211247735273,13.1544696413275,124.622129955389)) ;
#80134=CARTESIAN_POINT('Ctrl Pts',(-19.5567324960085,13.1527935023082,124.618303626824)) ;
#80135=CARTESIAN_POINT('Ctrl Pts',(-19.5919531539832,13.1511142506408,124.612946734366)) ;
#80136=CARTESIAN_POINT('Ctrl Pts',(-19.6257887200428,13.1495010374305,124.607800507717)) ;
#80137=CARTESIAN_POINT('Ctrl Pts',(-19.659266612977,13.147884951575,124.601242220538)) ;
#80138=CARTESIAN_POINT('Ctrl Pts',(-19.6921789519876,13.1462666758921,124.593361571178)) ;
#80139=CARTESIAN_POINT('Ctrl Pts',(-19.7130866415298,13.14523866006,124.588355358458)) ;
#80140=CARTESIAN_POINT('Ctrl Pts',(-19.7340270137043,13.1442031299505,124.582750069096)) ;
#80141=CARTESIAN_POINT('Ctrl Pts',(-19.7547385735872,13.1431759272749,124.576607071303)) ;
#80142=CARTESIAN_POINT('Ctrl Pts',(-19.7709429874757,13.1423722593042,124.571800881943)) ;
#80143=CARTESIAN_POINT('Ctrl Pts',(-19.7870074624047,13.1415736887748,124.566666606665)) ;
#80144=CARTESIAN_POINT('Ctrl Pts',(-19.8028133768221,13.1407878025743,124.561254910467)) ;
#80145=CARTESIAN_POINT('Ctrl Pts',(-19.8206105815958,13.1399029073845,124.555161427808)) ;
#80146=CARTESIAN_POINT('Ctrl Pts',(-19.8384921936885,13.1390131360211,124.548572668124)) ;
#80147=CARTESIAN_POINT('Ctrl Pts',(-19.8561768921072,13.1381271180561,124.541576901594)) ;
#80148=CARTESIAN_POINT('Ctrl Pts',(-19.8677905613895,13.1375452636541,124.536982731147)) ;
#80149=CARTESIAN_POINT('Ctrl Pts',(-19.8793196061818,13.1369650279592,124.532214063494)) ;
#80150=CARTESIAN_POINT('Ctrl Pts',(-19.8906888197564,13.1363888549909,124.527307307091)) ;
#80151=CARTESIAN_POINT('Ctrl Pts',(-19.9223697790245,13.1347833162944,124.513634351728)) ;
#80152=CARTESIAN_POINT('Ctrl Pts',(-19.9537678031507,13.1331490770808,124.498477050397)) ;
#80153=CARTESIAN_POINT('Ctrl Pts',(-19.9846098515591,13.1314967446217,124.481894184099)) ;
#80154=CARTESIAN_POINT('Ctrl Pts',(-20.0154518999675,13.1298444121627,124.465311317801)) ;
#80155=CARTESIAN_POINT('Ctrl Pts',(-20.045737223135,13.1281739864582,124.447303101419)) ;
#80156=CARTESIAN_POINT('Ctrl Pts',(-20.0752140367108,13.1264960747798,124.427985196501)) ;
#80157=CARTESIAN_POINT('Ctrl Pts',(-20.134546358724,13.1231186949368,124.389101205452)) ;
#80158=CARTESIAN_POINT('Ctrl Pts',(-20.1903651834497,13.119800985813,124.345089512785)) ;
#80159=CARTESIAN_POINT('Ctrl Pts',(-20.2420112365384,13.1164657148701,124.296473314913)) ;
#80160=CARTESIAN_POINT('Ctrl Pts',(-20.289587554447,13.1133932649693,124.251688098093)) ;
#80161=CARTESIAN_POINT('Ctrl Pts',(-20.3334894405665,13.1102924643633,124.203116917199)) ;
#80162=CARTESIAN_POINT('Ctrl Pts',(-20.3732409589605,13.1072237698501,124.151296426528)) ;
#80163=CARTESIAN_POINT('Ctrl Pts',(-20.376451305804,13.1069759409836,124.147111385167)) ;
#80164=CARTESIAN_POINT('Ctrl Pts',(-20.379634604183,13.1067283215206,124.142905169477)) ;
#80165=CARTESIAN_POINT('Ctrl Pts',(-20.382790614312,13.106480943306,124.138678072198)) ;
#80166=CARTESIAN_POINT('Ctrl Pts',(-20.4181815626463,13.1037068870598,124.091276138962)) ;
#80167=CARTESIAN_POINT('Ctrl Pts',(-20.450080551243,13.1009347849525,124.041322143165)) ;
#80168=CARTESIAN_POINT('Ctrl Pts',(-20.4781886737502,13.0981286305586,123.989291872839)) ;
#80169=CARTESIAN_POINT('Ctrl Pts',(-20.4834422395951,13.0976041445537,123.979567123311)) ;
#80170=CARTESIAN_POINT('Ctrl Pts',(-20.488563501437,13.0970784689762,123.969769917912)) ;
#80171=CARTESIAN_POINT('Ctrl Pts',(-20.4935506797433,13.0965513687291,123.959903468882)) ;
#80172=CARTESIAN_POINT('Ctrl Pts',(-20.5196526873711,13.0937926194271,123.908264222791)) ;
#80173=CARTESIAN_POINT('Ctrl Pts',(-20.5420463743133,13.0910584749845,123.854788919448)) ;
#80174=CARTESIAN_POINT('Ctrl Pts',(-20.5605278743063,13.0883504306551,123.799970707929)) ;
#80175=CARTESIAN_POINT('Ctrl Pts',(-20.5646923033328,13.0877402281058,123.787618542179)) ;
#80176=CARTESIAN_POINT('Ctrl Pts',(-20.568658291334,13.0871313507487,123.775198270447)) ;
#80177=CARTESIAN_POINT('Ctrl Pts',(-20.5724238452424,13.0865238156907,123.762715670384)) ;
#80178=CARTESIAN_POINT('Ctrl Pts',(-20.590720052164,13.0835719027974,123.702064770356)) ;
#80179=CARTESIAN_POINT('Ctrl Pts',(-20.6042533504138,13.0805866753739,123.640031126584)) ;
#80180=CARTESIAN_POINT('Ctrl Pts',(-20.6128804632903,13.0775726118262,123.577263035347)) ;
#80181=CARTESIAN_POINT('Ctrl Pts',(-20.6138609883362,13.0772300447541,123.57012905131)) ;
#80182=CARTESIAN_POINT('Ctrl Pts',(-20.614778190337,13.0768871051846,123.562985593044)) ;
#80183=CARTESIAN_POINT('Ctrl Pts',(-20.615631900232,13.0765437996927,123.555833623426)) ;
#80184=CARTESIAN_POINT('Ctrl Pts',(-20.6240384845652,13.0731632290955,123.485407315736)) ;
#80185=CARTESIAN_POINT('Ctrl Pts',(-20.6262623135186,13.069833350483,123.414355351615)) ;
#80186=CARTESIAN_POINT('Ctrl Pts',(-20.6222745808894,13.0665160349233,123.343533529152)) ;
#80187=CARTESIAN_POINT('Ctrl Pts',(-20.6202145429152,13.0648023302542,123.306947414373)) ;
#80188=CARTESIAN_POINT('Ctrl Pts',(-20.6164972921792,13.0630787969676,123.270496808143)) ;
#80189=CARTESIAN_POINT('Ctrl Pts',(-20.6111745725807,13.0613571613528,123.234434593911)) ;
#80190=CARTESIAN_POINT('Ctrl Pts',(-20.6062595643491,13.0597674001297,123.201134684621)) ;
#80191=CARTESIAN_POINT('Ctrl Pts',(-20.5999763082354,13.0581792569958,123.168166269748)) ;
#80192=CARTESIAN_POINT('Ctrl Pts',(-20.5924035112702,13.0566019647332,123.135717490083)) ;
#80193=CARTESIAN_POINT('Ctrl Pts',(-20.5873355715961,13.0555463941068,123.114001807146)) ;
#80194=CARTESIAN_POINT('Ctrl Pts',(-20.5816296818219,13.0544857440984,123.09227307492)) ;
#80195=CARTESIAN_POINT('Ctrl Pts',(-20.5753455905511,13.0534299520535,123.070787072469)) ;
#80196=CARTESIAN_POINT('Ctrl Pts',(-20.5701618703803,13.0525590336846,123.053063360401)) ;
#80197=CARTESIAN_POINT('Ctrl Pts',(-20.5645857062331,13.0516914209316,123.035504758932)) ;
#80198=CARTESIAN_POINT('Ctrl Pts',(-20.5586761597941,13.0508326916541,123.018246884138)) ;
#80199=CARTESIAN_POINT('Ctrl Pts',(-20.5529103591577,13.0499948503975,123.001408795718)) ;
#80200=CARTESIAN_POINT('Ctrl Pts',(-20.546693394412,13.0491462820869,122.984473753146)) ;
#80201=CARTESIAN_POINT('Ctrl Pts',(-20.5401199674319,13.0482990036882,122.967735207664)) ;
#80202=CARTESIAN_POINT('Ctrl Pts',(-20.5361498654645,13.0477872794919,122.957625757517)) ;
#80203=CARTESIAN_POINT('Ctrl Pts',(-20.5320507039911,13.0472760258174,122.947587682286)) ;
#80204=CARTESIAN_POINT('Ctrl Pts',(-20.5278519379966,13.0467678900933,122.937682269247)) ;
#80205=CARTESIAN_POINT('Ctrl Pts',(-20.5150841029079,13.045222723457,122.907561352688)) ;
#80206=CARTESIAN_POINT('Ctrl Pts',(-20.500969811741,13.0436600419622,122.877660814971)) ;
#80207=CARTESIAN_POINT('Ctrl Pts',(-20.4855559912974,13.0420909675042,122.848226004151)) ;
#80208=CARTESIAN_POINT('Ctrl Pts',(-20.4702064941635,13.0405284409401,122.81891402754)) ;
#80209=CARTESIAN_POINT('Ctrl Pts',(-20.4535684798359,13.0389595746585,122.79006450468)) ;
#80210=CARTESIAN_POINT('Ctrl Pts',(-20.4357371405512,13.0373953518966,122.761902609047)) ;
#80211=CARTESIAN_POINT('Ctrl Pts',(-20.4336430548303,13.0372116519234,122.758595318295)) ;
#80212=CARTESIAN_POINT('Ctrl Pts',(-20.4315325643706,13.0370280159926,122.755297485666)) ;
#80213=CARTESIAN_POINT('Ctrl Pts',(-20.4294058654555,13.0368444618938,122.752009454393)) ;
#80214=CARTESIAN_POINT('Ctrl Pts',(-20.3911287352109,13.0335407859017,122.69283022579)) ;
#80215=CARTESIAN_POINT('Ctrl Pts',(-20.3477826778876,13.0302328466101,122.637107690408)) ;
#80216=CARTESIAN_POINT('Ctrl Pts',(-20.2998744795623,13.0268838791217,122.585474826046)) ;
#80217=CARTESIAN_POINT('Ctrl Pts',(-20.2568823878123,13.0238785664078,122.539140275395)) ;
#80218=CARTESIAN_POINT('Ctrl Pts',(-20.2103150811076,13.0208984974685,122.496210972854)) ;
#80219=CARTESIAN_POINT('Ctrl Pts',(-20.160660763911,13.0179372381888,122.457130940217)) ;
#80220=CARTESIAN_POINT('Ctrl Pts',(-20.1546424670006,13.0175783220144,122.452394287838)) ;
#80221=CARTESIAN_POINT('Ctrl Pts',(-20.1485788626903,13.0172196821611,122.447714136001)) ;
#80222=CARTESIAN_POINT('Ctrl Pts',(-20.142470855856,13.0168613071728,122.443091237322)) ;
#80223=CARTESIAN_POINT('Ctrl Pts',(-20.0955166488246,13.0141063637269,122.40755353287)) ;
#80224=CARTESIAN_POINT('Ctrl Pts',(-20.0460100127249,13.0113300555962,122.375458694454)) ;
#80225=CARTESIAN_POINT('Ctrl Pts',(-19.9944195367589,13.0085420966997,122.347105758613)) ;
#80226=CARTESIAN_POINT('Ctrl Pts',(-19.9840590476005,13.0079822139427,122.341411872699)) ;
#80227=CARTESIAN_POINT('Ctrl Pts',(-19.9736146068897,13.0074218613176,122.335868752493)) ;
#80228=CARTESIAN_POINT('Ctrl Pts',(-19.9630901436767,13.0068611174976,122.33047860471)) ;
#80229=CARTESIAN_POINT('Ctrl Pts',(-19.9115657163906,13.0041158939557,122.304090154115)) ;
#80230=CARTESIAN_POINT('Ctrl Pts',(-19.8581843020153,13.0013947918625,122.281404000126)) ;
#80231=CARTESIAN_POINT('Ctrl Pts',(-19.8034385789658,12.9986707661172,122.262626648871)) ;
#80232=CARTESIAN_POINT('Ctrl Pts',(-19.7910897472083,12.9980563156404,122.258391096967)) ;
#80233=CARTESIAN_POINT('Ctrl Pts',(-19.7786715777912,12.9974417164067,122.254354232714)) ;
#80234=CARTESIAN_POINT('Ctrl Pts',(-19.7661898627449,12.9968266580205,122.250518086325)) ;
#80235=CARTESIAN_POINT('Ctrl Pts',(-19.7075298248851,12.9939360818386,122.232489434682)) ;
#80236=CARTESIAN_POINT('Ctrl Pts',(-19.6475485678453,12.9910307279178,122.218923594634)) ;
#80237=CARTESIAN_POINT('Ctrl Pts',(-19.5868449944418,12.9881433223301,122.209954755408)) ;
#80238=CARTESIAN_POINT('Ctrl Pts',(-19.5777701226496,12.9877116700558,122.208613960105)) ;
#80239=CARTESIAN_POINT('Ctrl Pts',(-19.568679128988,12.9872804189036,122.207375809367)) ;
#80240=CARTESIAN_POINT('Ctrl Pts',(-19.5595740378673,12.9868496782118,122.206240654098)) ;
#80241=CARTESIAN_POINT('Ctrl Pts',(-19.4898970413724,12.9835534215054,122.197553842661)) ;
#80242=CARTESIAN_POINT('Ctrl Pts',(-19.4195615991172,12.9802519555717,122.194920530747)) ;
#80243=CARTESIAN_POINT('Ctrl Pts',(-19.3493791105797,12.9769173597985,122.198384430384)) ;
#80244=CARTESIAN_POINT('Ctrl Pts',(-19.3116842828543,12.9751263572873,122.200244881656)) ;
#80245=CARTESIAN_POINT('Ctrl Pts',(-19.2741285272671,12.9733486752165,122.203863529548)) ;
#80246=CARTESIAN_POINT('Ctrl Pts',(-19.2369706410513,12.9715813245093,122.20918701055)) ;
#80247=CARTESIAN_POINT('Ctrl Pts',(-19.2042609075386,12.970025542506,122.213873220199)) ;
#80248=CARTESIAN_POINT('Ctrl Pts',(-19.1718596801468,12.9684777663934,122.219879657425)) ;
#80249=CARTESIAN_POINT('Ctrl Pts',(-19.139934078093,12.9669359571818,122.227137807232)) ;
#80250=CARTESIAN_POINT('Ctrl Pts',(-19.1174728567786,12.96585121905,122.232244270341)) ;
#80251=CARTESIAN_POINT('Ctrl Pts',(-19.0950170794709,12.9647552497427,122.238025766184)) ;
#80252=CARTESIAN_POINT('Ctrl Pts',(-19.0728179318652,12.9636626863374,122.244423639262)) ;
#80253=CARTESIAN_POINT('Ctrl Pts',(-19.0535145082355,12.9627126402082,122.249986954419)) ;
#80254=CARTESIAN_POINT('Ctrl Pts',(-19.0344051671983,12.9617651693813,122.256015449663)) ;
#80255=CARTESIAN_POINT('Ctrl Pts',(-19.0156454794067,12.9608298976992,122.262439937836)) ;
#80256=CARTESIAN_POINT('Ctrl Pts',(-18.9996147016043,12.9600306769079,122.267929876877)) ;
#80257=CARTESIAN_POINT('Ctrl Pts',(-18.9834735656277,12.9592217466141,122.273836898882)) ;
#80258=CARTESIAN_POINT('Ctrl Pts',(-18.9675274205177,12.9584173094524,122.280060838364)) ;
#80259=CARTESIAN_POINT('Ctrl Pts',(-18.958652576749,12.9579695991071,122.283524778404)) ;
#80260=CARTESIAN_POINT('Ctrl Pts',(-18.9498378417739,12.9575232805054,122.287085994564)) ;
#80261=CARTESIAN_POINT('Ctrl Pts',(-18.9411333105159,12.9570808020558,122.290720692799)) ;
#80262=CARTESIAN_POINT('Ctrl Pts',(-18.9115402471301,12.9555764944238,122.303077688491)) ;
#80263=CARTESIAN_POINT('Ctrl Pts',(-18.8821336217213,12.95405373186,122.316737473371)) ;
#80264=CARTESIAN_POINT('Ctrl Pts',(-18.8531578655204,12.9525179515629,122.331655155192)) ;
#80265=CARTESIAN_POINT('Ctrl Pts',(-18.8243115077086,12.9509890296715,122.346506218425)) ;
#80266=CARTESIAN_POINT('Ctrl Pts',(-18.7958927801328,12.9494472060551,122.3626037859)) ;
#80267=CARTESIAN_POINT('Ctrl Pts',(-18.7681258982293,12.9478978453932,122.379854682488)) ;
#80268=CARTESIAN_POINT('Ctrl Pts',(-18.7641464874169,12.9476757987626,122.382326994814)) ;
#80269=CARTESIAN_POINT('Ctrl Pts',(-18.7601804276636,12.9474535973271,122.384822916485)) ;
#80270=CARTESIAN_POINT('Ctrl Pts',(-18.7562283392693,12.9472312568782,122.387342094819)) ;
#80271=CARTESIAN_POINT('Ctrl Pts',(-18.6964137833706,12.943866151171,122.425469666436)) ;
#80272=CARTESIAN_POINT('Ctrl Pts',(-18.6400443839774,12.9405486009369,122.468770151356)) ;
#80273=CARTESIAN_POINT('Ctrl Pts',(-18.5877897308444,12.9372019724685,122.51672659073)) ;
#80274=CARTESIAN_POINT('Ctrl Pts',(-18.5396101659096,12.9341163314023,122.560943138851)) ;
#80275=CARTESIAN_POINT('Ctrl Pts',(-18.4950608892707,12.9310133340656,122.609000108474)) ;
#80276=CARTESIAN_POINT('Ctrl Pts',(-18.4546266679024,12.9279493121563,122.660366627298)) ;
#80277=CARTESIAN_POINT('Ctrl Pts',(-18.4512066913697,12.9276901533876,122.664711271093)) ;
#80278=CARTESIAN_POINT('Ctrl Pts',(-18.4478161310652,12.9274312734485,122.669079570653)) ;
#80279=CARTESIAN_POINT('Ctrl Pts',(-18.4444552679901,12.927172706425,122.673471192872)) ;
#80280=CARTESIAN_POINT('Ctrl Pts',(-18.4082581932642,12.9243878950052,122.720769721275)) ;
#80281=CARTESIAN_POINT('Ctrl Pts',(-18.375571621791,12.9215938819148,122.770694787871)) ;
#80282=CARTESIAN_POINT('Ctrl Pts',(-18.3467042321094,12.9187651732054,122.82276604254)) ;
#80283=CARTESIAN_POINT('Ctrl Pts',(-18.3414903806441,12.9182542691295,122.83217083426)) ;
#80284=CARTESIAN_POINT('Ctrl Pts',(-18.3364009997207,12.9177422332347,122.841645565417)) ;
#80285=CARTESIAN_POINT('Ctrl Pts',(-18.3314377545054,12.917228915314,122.851187309489)) ;
#80286=CARTESIAN_POINT('Ctrl Pts',(-18.3047988596977,12.9144738182958,122.902400075654)) ;
#80287=CARTESIAN_POINT('Ctrl Pts',(-18.2818294855986,12.9117487873613,122.95548336231)) ;
#80288=CARTESIAN_POINT('Ctrl Pts',(-18.262738061945,12.9090471640161,123.009949046226)) ;
#80289=CARTESIAN_POINT('Ctrl Pts',(-18.2583816834394,12.9084306938102,123.022377304013)) ;
#80290=CARTESIAN_POINT('Ctrl Pts',(-18.2542270258558,12.907815442401,123.034877458936)) ;
#80291=CARTESIAN_POINT('Ctrl Pts',(-18.2502762138882,12.9072013306773,123.047443566635)) ;
#80292=CARTESIAN_POINT('Ctrl Pts',(-18.2316189672304,12.9043012600087,123.106785538054)) ;
#80293=CARTESIAN_POINT('Ctrl Pts',(-18.2175379643146,12.9013695518874,123.167515476281)) ;
#80294=CARTESIAN_POINT('Ctrl Pts',(-18.2081770681978,12.8984127829643,123.229015350927)) ;
#80295=CARTESIAN_POINT('Ctrl Pts',(-18.2069304814426,12.898019031241,123.237205264396)) ;
#80296=CARTESIAN_POINT('Ctrl Pts',(-18.2057675283162,12.8976248350859,123.245408813936)) ;
#80297=CARTESIAN_POINT('Ctrl Pts',(-18.2046884809982,12.8972302100307,123.253624522122)) ;
#80298=CARTESIAN_POINT('Ctrl Pts',(-18.1954900615473,12.8938661992751,123.323659940141)) ;
#80299=CARTESIAN_POINT('Ctrl Pts',(-18.1924158000991,12.8905427332555,123.394395417807)) ;
#80300=CARTESIAN_POINT('Ctrl Pts',(-18.1955062488531,12.8872427554171,123.46497806835)) ;
#80301=CARTESIAN_POINT('Ctrl Pts',(-18.1972007151705,12.8854334061153,123.503677925057)) ;
#80302=CARTESIAN_POINT('Ctrl Pts',(-18.2007483633934,12.8836140272436,123.542250460683)) ;
#80303=CARTESIAN_POINT('Ctrl Pts',(-18.2060983810991,12.8817930848426,123.580430274451)) ;
#80304=CARTESIAN_POINT('Ctrl Pts',(-18.2104580346587,12.880309224703,123.611542463261)) ;
#80305=CARTESIAN_POINT('Ctrl Pts',(-18.2160134967859,12.878824326319,123.64239381509)) ;
#80306=CARTESIAN_POINT('Ctrl Pts',(-18.2227126010336,12.8773429707999,123.672847623171)) ;
#80307=CARTESIAN_POINT('Ctrl Pts',(-18.2277179246073,12.8762361566011,123.695601585173)) ;
#80308=CARTESIAN_POINT('Ctrl Pts',(-18.2334066902034,12.8751269962437,123.718322694069)) ;
#80309=CARTESIAN_POINT('Ctrl Pts',(-18.2397173376852,12.8740258444861,123.740761170446)) ;
#80310=CARTESIAN_POINT('Ctrl Pts',(-18.245864571975,12.8729532068744,123.76261860612)) ;
#80311=CARTESIAN_POINT('Ctrl Pts',(-18.2526015019176,12.8718881684698,123.784207516959)) ;
#80312=CARTESIAN_POINT('Ctrl Pts',(-18.259825879779,12.870840300276,123.80531165987)) ;
#80313=CARTESIAN_POINT('Ctrl Pts',(-18.259825879779,12.8888247888663,123.80531165987)) ;
#80314=CARTESIAN_POINT('Ctrl Pts',(-18.2532458294082,12.8897813285136,123.786089752316)) ;
#80315=CARTESIAN_POINT('Ctrl Pts',(-18.247071181349,12.8907544247006,123.766465209361)) ;
#80316=CARTESIAN_POINT('Ctrl Pts',(-18.2414031003154,12.8917312466636,123.746697274626)) ;
#80317=CARTESIAN_POINT('Ctrl Pts',(-18.2371820599301,12.8924586895019,123.731976022344)) ;
#80318=CARTESIAN_POINT('Ctrl Pts',(-18.2332409732336,12.893188198594,123.717175704504)) ;
#80319=CARTESIAN_POINT('Ctrl Pts',(-18.2296035771432,12.8939144748306,123.702408737262)) ;
#80320=CARTESIAN_POINT('Ctrl Pts',(-18.2212772303626,12.8955769904473,123.668605739978)) ;
#80321=CARTESIAN_POINT('Ctrl Pts',(-18.2143391259864,12.8972454835374,123.634164045277)) ;
#80322=CARTESIAN_POINT('Ctrl Pts',(-18.2088966327909,12.8989103111607,123.599318432764)) ;
#80323=CARTESIAN_POINT('Ctrl Pts',(-18.2034541395954,12.900575138784,123.56447282025)) ;
#80324=CARTESIAN_POINT('Ctrl Pts',(-18.199507497113,12.9022363009406,123.529223921072)) ;
#80325=CARTESIAN_POINT('Ctrl Pts',(-18.197112973659,12.9038841546903,123.493822157852)) ;
#80326=CARTESIAN_POINT('Ctrl Pts',(-18.1923664545662,12.9071505955648,123.423647382676)) ;
#80327=CARTESIAN_POINT('Ctrl Pts',(-18.19372501243,12.9104588638225,123.353212635087)) ;
#80328=CARTESIAN_POINT('Ctrl Pts',(-18.2011587472781,12.9138225142835,123.283326965522)) ;
#80329=CARTESIAN_POINT('Ctrl Pts',(-18.2077270055295,12.916794549922,123.221577772801)) ;
#80330=CARTESIAN_POINT('Ctrl Pts',(-18.2190277864584,12.919718658498,123.160388817979)) ;
#80331=CARTESIAN_POINT('Ctrl Pts',(-18.2349430601355,12.9226187056347,123.100380637484)) ;
#80332=CARTESIAN_POINT('Ctrl Pts',(-18.2372015476686,12.9230302424035,123.091865061171)) ;
#80333=CARTESIAN_POINT('Ctrl Pts',(-18.2395528758531,12.9234412946332,123.083373246407)) ;
#80334=CARTESIAN_POINT('Ctrl Pts',(-18.241996623602,12.9238519305238,123.074906951587)) ;
#80335=CARTESIAN_POINT('Ctrl Pts',(-18.2583480343684,12.9265995447674,123.018257952383)) ;
#80336=CARTESIAN_POINT('Ctrl Pts',(-18.2788154430492,12.9293831647335,122.96284209491)) ;
#80337=CARTESIAN_POINT('Ctrl Pts',(-18.3032017711111,12.9321792524141,122.909180924394)) ;
#80338=CARTESIAN_POINT('Ctrl Pts',(-18.3079630592657,12.9327251722065,122.898703894195)) ;
#80339=CARTESIAN_POINT('Ctrl Pts',(-18.3128735896712,12.9332715672717,122.888293694738)) ;
#80340=CARTESIAN_POINT('Ctrl Pts',(-18.31793167961,12.9338182624219,122.877954123308)) ;
#80341=CARTESIAN_POINT('Ctrl Pts',(-18.3435730794007,12.9365896700242,122.825538866186)) ;
#80342=CARTESIAN_POINT('Ctrl Pts',(-18.3729787867492,12.9393311003956,122.775004910072)) ;
#80343=CARTESIAN_POINT('Ctrl Pts',(-18.4058732647575,12.9420751350093,122.726821529459)) ;
#80344=CARTESIAN_POINT('Ctrl Pts',(-18.4128371725788,12.9426560593852,122.716620892714)) ;
#80345=CARTESIAN_POINT('Ctrl Pts',(-18.4199572833244,12.94323710048,122.706525510553)) ;
#80346=CARTESIAN_POINT('Ctrl Pts',(-18.4272307252923,12.9438185674378,122.696539681904)) ;
#80347=CARTESIAN_POINT('Ctrl Pts',(-18.4642301242527,12.9467764418593,122.645742595765)) ;
#80348=CARTESIAN_POINT('Ctrl Pts',(-18.5051425390423,12.9497506721255,122.597862446162)) ;
#80349=CARTESIAN_POINT('Ctrl Pts',(-18.5495449045503,12.9527091008555,122.553393629733)) ;
#80350=CARTESIAN_POINT('Ctrl Pts',(-18.5550400253381,12.9530752282685,122.547890285153)) ;
#80351=CARTESIAN_POINT('Ctrl Pts',(-18.5605885476501,12.9534411136669,122.542439146153)) ;
#80352=CARTESIAN_POINT('Ctrl Pts',(-18.5661896262514,12.9538066960978,122.537041114959)) ;
#80353=CARTESIAN_POINT('Ctrl Pts',(-18.6169576386995,12.9571203245476,122.48811351827)) ;
#80354=CARTESIAN_POINT('Ctrl Pts',(-18.6719101867737,12.9604271439176,122.443678705657)) ;
#80355=CARTESIAN_POINT('Ctrl Pts',(-18.7304180440209,12.9637793859921,122.404259137644)) ;
#80356=CARTESIAN_POINT('Ctrl Pts',(-18.7598230568367,12.965464163487,122.384447560923)) ;
#80357=CARTESIAN_POINT('Ctrl Pts',(-18.7900595549664,12.9671409241981,122.365952648998)) ;
#80358=CARTESIAN_POINT('Ctrl Pts',(-18.8208969866602,12.9688031493527,122.348883271387)) ;
#80359=CARTESIAN_POINT('Ctrl Pts',(-18.851734418354,12.9704653745073,122.331813893776)) ;
#80360=CARTESIAN_POINT('Ctrl Pts',(-18.8831721463384,12.9721130641054,122.316170247903)) ;
#80361=CARTESIAN_POINT('Ctrl Pts',(-18.9149607439661,12.973739699374,122.302011771837)) ;
#80362=CARTESIAN_POINT('Ctrl Pts',(-18.9338084784656,12.9747041454949,122.293617088909)) ;
#80363=CARTESIAN_POINT('Ctrl Pts',(-18.9530441471631,12.9756793751788,122.285629754367)) ;
#80364=CARTESIAN_POINT('Ctrl Pts',(-18.9724168258569,12.976654697032,122.278164604653)) ;
#80365=CARTESIAN_POINT('Ctrl Pts',(-18.9868451849857,12.977381096008,122.272604719893)) ;
#80366=CARTESIAN_POINT('Ctrl Pts',(-19.001349010063,12.9781075461099,122.267333529315)) ;
#80367=CARTESIAN_POINT('Ctrl Pts',(-19.0158180196968,12.9788296304523,122.262380863738)) ;
#80368=CARTESIAN_POINT('Ctrl Pts',(-19.0342731679293,12.9797506453602,122.256063763973)) ;
#80369=CARTESIAN_POINT('Ctrl Pts',(-19.053109171126,12.9806863048851,122.2501174097)) ;
#80370=CARTESIAN_POINT('Ctrl Pts',(-19.0720577385372,12.9816216662129,122.244642997795)) ;
#80371=CARTESIAN_POINT('Ctrl Pts',(-19.0851606201767,12.9822684659684,122.240857457196)) ;
#80372=CARTESIAN_POINT('Ctrl Pts',(-19.0983169045046,12.9829151231355,122.237296577758)) ;
#80373=CARTESIAN_POINT('Ctrl Pts',(-19.1114337586695,12.9835566968411,122.233979808178)) ;
#80374=CARTESIAN_POINT('Ctrl Pts',(-19.1451010559027,12.9852034371626,122.22546658802)) ;
#80375=CARTESIAN_POINT('Ctrl Pts',(-19.1794387949778,12.9868560446172,122.218324534818)) ;
#80376=CARTESIAN_POINT('Ctrl Pts',(-19.21420034137,12.9885147179043,122.212669835824)) ;
#80377=CARTESIAN_POINT('Ctrl Pts',(-19.2489618877623,12.9901733911914,122.207015136831)) ;
#80378=CARTESIAN_POINT('Ctrl Pts',(-19.2841465466228,12.9918381303111,122.202848063812)) ;
#80379=CARTESIAN_POINT('Ctrl Pts',(-19.3194904692908,12.9935091339629,122.200229100371)) ;
#80380=CARTESIAN_POINT('Ctrl Pts',(-19.3902004547269,12.9968521880148,122.194989532921)) ;
#80381=CARTESIAN_POINT('Ctrl Pts',(-19.4612308056923,13.000197572698,122.195951121451)) ;
#80382=CARTESIAN_POINT('Ctrl Pts',(-19.5317526856796,13.0035326050172,122.203097207542)) ;
#80383=CARTESIAN_POINT('Ctrl Pts',(-19.5962898690814,13.0065846165698,122.209636855502)) ;
#80384=CARTESIAN_POINT('Ctrl Pts',(-19.6602229995032,13.0096473642197,122.221341375042)) ;
#80385=CARTESIAN_POINT('Ctrl Pts',(-19.7228608896261,13.0127043920223,122.238076259414)) ;
#80386=CARTESIAN_POINT('Ctrl Pts',(-19.7282510714014,13.0129674586026,122.239516347332)) ;
#80387=CARTESIAN_POINT('Ctrl Pts',(-19.7336316683635,13.0132304828266,122.240993654563)) ;
#80388=CARTESIAN_POINT('Ctrl Pts',(-19.7390022433148,13.0134934542082,122.242508077663)) ;
#80389=CARTESIAN_POINT('Ctrl Pts',(-19.7953263709184,13.0162513774818,122.258390652745)) ;
#80390=CARTESIAN_POINT('Ctrl Pts',(-19.8504639847626,13.0189973645646,122.278336270964)) ;
#80391=CARTESIAN_POINT('Ctrl Pts',(-19.9039010481062,13.0217630898227,122.302155474036)) ;
#80392=CARTESIAN_POINT('Ctrl Pts',(-19.9148591565728,13.0223302451915,122.307039975439)) ;
#80393=CARTESIAN_POINT('Ctrl Pts',(-19.925745816016,13.0228982305888,122.312087205238)) ;
#80394=CARTESIAN_POINT('Ctrl Pts',(-19.9365566901172,13.0234673191557,122.317295276546)) ;
#80395=CARTESIAN_POINT('Ctrl Pts',(-19.9886872531689,13.0262114920266,122.342408850818)) ;
#80396=CARTESIAN_POINT('Ctrl Pts',(-20.038990378096,13.0289466035877,122.371235502409)) ;
#80397=CARTESIAN_POINT('Ctrl Pts',(-20.0870043674368,13.0316624975888,122.403507549976)) ;
#80398=CARTESIAN_POINT('Ctrl Pts',(-20.0978207686876,13.0322743234269,122.410777668966)) ;
#80399=CARTESIAN_POINT('Ctrl Pts',(-20.1085211047223,13.0328851739874,122.418222459547)) ;
#80400=CARTESIAN_POINT('Ctrl Pts',(-20.1191002842362,13.033494933158,122.425838547868)) ;
#80401=CARTESIAN_POINT('Ctrl Pts',(-20.1704527012543,13.0364547664011,122.462807817837)) ;
#80402=CARTESIAN_POINT('Ctrl Pts',(-20.2188726090177,13.0394380498734,122.503762264382)) ;
#80403=CARTESIAN_POINT('Ctrl Pts',(-20.2638534759819,13.0424389658114,122.548275688336)) ;
#80404=CARTESIAN_POINT('Ctrl Pts',(-20.2689325561807,13.0427778186114,122.553301986526)) ;
#80405=CARTESIAN_POINT('Ctrl Pts',(-20.2739678224269,13.0431168962276,122.558373619549)) ;
#80406=CARTESIAN_POINT('Ctrl Pts',(-20.2789585710333,13.0434561902842,122.563489940625)) ;
#80407=CARTESIAN_POINT('Ctrl Pts',(-20.328332389001,13.0468128496365,122.614106055637)) ;
#80408=CARTESIAN_POINT('Ctrl Pts',(-20.3732090024784,13.0501297950685,122.668954533018)) ;
#80409=CARTESIAN_POINT('Ctrl Pts',(-20.413054955581,13.0534545350462,122.727391594305)) ;
#80410=CARTESIAN_POINT('Ctrl Pts',(-20.4333412241692,13.0551472180647,122.757142919809)) ;
#80411=CARTESIAN_POINT('Ctrl Pts',(-20.4522765989244,13.0568444933791,122.78776252857)) ;
#80412=CARTESIAN_POINT('Ctrl Pts',(-20.4697500363502,13.0585351659895,122.819020680216)) ;
#80413=CARTESIAN_POINT('Ctrl Pts',(-20.4865506341453,13.0601607368395,122.849075192149)) ;
#80414=CARTESIAN_POINT('Ctrl Pts',(-20.501999818948,13.0617802036885,122.879719360213)) ;
#80415=CARTESIAN_POINT('Ctrl Pts',(-20.5160412745599,13.063383615616,122.910732424749)) ;
#80416=CARTESIAN_POINT('Ctrl Pts',(-20.5249283323932,13.0643984402128,122.930361080476)) ;
#80417=CARTESIAN_POINT('Ctrl Pts',(-20.5333601781884,13.0654199755197,122.950384604298)) ;
#80418=CARTESIAN_POINT('Ctrl Pts',(-20.5412249340041,13.0664387567713,122.970559243378)) ;
#80419=CARTESIAN_POINT('Ctrl Pts',(-20.5474251735456,13.0672419206518,122.986464072197)) ;
#80420=CARTESIAN_POINT('Ctrl Pts',(-20.5532738640289,13.068043372866,123.002462265936)) ;
#80421=CARTESIAN_POINT('Ctrl Pts',(-20.558737602334,13.0688384759608,123.018426362858)) ;
#80422=CARTESIAN_POINT('Ctrl Pts',(-20.5647703980733,13.0697163903658,123.036053147034)) ;
#80423=CARTESIAN_POINT('Ctrl Pts',(-20.5704708719528,13.0706067410412,123.054045743056)) ;
#80424=CARTESIAN_POINT('Ctrl Pts',(-20.5757361798665,13.0714972686474,123.072125390042)) ;
#80425=CARTESIAN_POINT('Ctrl Pts',(-20.579151634762,13.072074928477,123.083853140787)) ;
#80426=CARTESIAN_POINT('Ctrl Pts',(-20.5823849749415,13.0726526627545,123.095617130514)) ;
#80427=CARTESIAN_POINT('Ctrl Pts',(-20.5854194026214,13.0732271253608,123.107337957534)) ;
#80428=CARTESIAN_POINT('Ctrl Pts',(-20.5941186488215,13.0748740229545,123.140939799685)) ;
#80429=CARTESIAN_POINT('Ctrl Pts',(-20.6014580999589,13.0765340989596,123.175244208016)) ;
#80430=CARTESIAN_POINT('Ctrl Pts',(-20.6073128924853,13.0781972778934,123.209996445795)) ;
#80431=CARTESIAN_POINT('Ctrl Pts',(-20.6131676850117,13.0798604568273,123.244748683574)) ;
#80432=CARTESIAN_POINT('Ctrl Pts',(-20.617537515338,13.0815267386897,123.279948012451)) ;
#80433=CARTESIAN_POINT('Ctrl Pts',(-20.6203564173013,13.083186047998,123.31532090111)) ;
#80434=CARTESIAN_POINT('Ctrl Pts',(-20.6259389565516,13.0864721357949,123.385373191648)) ;
#80435=CARTESIAN_POINT('Ctrl Pts',(-20.6254307588554,13.089790362517,123.455751084173)) ;
#80436=CARTESIAN_POINT('Ctrl Pts',(-20.6188518700433,13.0931166999359,123.525661255243)) ;
#80437=CARTESIAN_POINT('Ctrl Pts',(-20.6129825581758,13.0960842697257,123.588031149073)) ;
#80438=CARTESIAN_POINT('Ctrl Pts',(-20.6022908582607,13.0990174373957,123.649884042373)) ;
#80439=CARTESIAN_POINT('Ctrl Pts',(-20.5868916641318,13.1019732940614,123.710584825956)) ;
#80440=CARTESIAN_POINT('Ctrl Pts',(-20.5849358576223,13.1023487087526,123.718294254558)) ;
#80441=CARTESIAN_POINT('Ctrl Pts',(-20.5829041831187,13.1027244894353,123.725985111667)) ;
#80442=CARTESIAN_POINT('Ctrl Pts',(-20.5807969353277,13.1031007530736,123.733656106331)) ;
#80443=CARTESIAN_POINT('Ctrl Pts',(-20.5653733780598,13.1058547356842,123.789802339353)) ;
#80444=CARTESIAN_POINT('Ctrl Pts',(-20.5459194132871,13.1086131334078,123.844802121024)) ;
#80445=CARTESIAN_POINT('Ctrl Pts',(-20.5226186805511,13.1113469816987,123.898146114111)) ;
#80446=CARTESIAN_POINT('Ctrl Pts',(-20.5175456933214,13.1119421894814,123.909760057706)) ;
#80447=CARTESIAN_POINT('Ctrl Pts',(-20.5122905486546,13.1125362335941,123.921295583843)) ;
#80448=CARTESIAN_POINT('Ctrl Pts',(-20.5068554484329,13.1131288151207,123.932747551088)) ;
#80449=CARTESIAN_POINT('Ctrl Pts',(-20.4816239304041,13.1158797729435,123.985911339469)) ;
#80450=CARTESIAN_POINT('Ctrl Pts',(-20.4525416222922,13.1186438690752,124.037206847902)) ;
#80451=CARTESIAN_POINT('Ctrl Pts',(-20.4198836724748,13.1214376143312,124.086151956349)) ;
#80452=CARTESIAN_POINT('Ctrl Pts',(-20.4134463021852,13.1219883033,124.095799769169)) ;
#80453=CARTESIAN_POINT('Ctrl Pts',(-20.4068701432227,13.1225401442649,124.105356339859)) ;
#80454=CARTESIAN_POINT('Ctrl Pts',(-20.4001575102361,13.1230932636784,124.114818094959)) ;
#80455=CARTESIAN_POINT('Ctrl Pts',(-20.3640599656681,13.1260676930446,124.165699191407)) ;
#80456=CARTESIAN_POINT('Ctrl Pts',(-20.3240715618893,13.1290113327513,124.213752737903)) ;
#80457=CARTESIAN_POINT('Ctrl Pts',(-20.280602485974,13.1319272155956,124.258488818542)) ;
#80458=CARTESIAN_POINT('Ctrl Pts',(-20.2746963362105,13.1323233970283,124.264567116424)) ;
#80459=CARTESIAN_POINT('Ctrl Pts',(-20.2687259912361,13.1327190660499,124.270584221896)) ;
#80460=CARTESIAN_POINT('Ctrl Pts',(-20.2626925378787,13.1331142302675,124.276538952679)) ;
#80461=CARTESIAN_POINT('Ctrl Pts',(-20.2124365464096,13.1364057729999,124.326139220003)) ;
#80462=CARTESIAN_POINT('Ctrl Pts',(-20.1579262026917,13.139733462171,124.371287158225)) ;
#80463=CARTESIAN_POINT('Ctrl Pts',(-20.0997951209569,13.1431024819908,124.411443806463)) ;
#80464=CARTESIAN_POINT('Ctrl Pts',(-20.0695294058607,13.144856548679,124.432351204683)) ;
#80465=CARTESIAN_POINT('Ctrl Pts',(-20.0383513299908,13.1465967018408,124.451853085651)) ;
#80466=CARTESIAN_POINT('Ctrl Pts',(-20.0064937701153,13.1483201646471,124.46983612822)) ;
#80467=CARTESIAN_POINT('Ctrl Pts',(-19.9768591713267,13.1499233674345,124.486564347632)) ;
#80468=CARTESIAN_POINT('Ctrl Pts',(-19.9466372807795,13.1515121278449,124.501978605502)) ;
#80469=CARTESIAN_POINT('Ctrl Pts',(-19.9160303243104,13.1530842107175,124.516025442661)) ;
#80470=CARTESIAN_POINT('Ctrl Pts',(-19.895810249714,13.1541227861468,124.525305296915)) ;
#80471=CARTESIAN_POINT('Ctrl Pts',(-19.8751876241726,13.1551716918063,124.534092711869)) ;
#80472=CARTESIAN_POINT('Ctrl Pts',(-19.8544013312711,13.1562211252396,124.542277670704)) ;
#80473=CARTESIAN_POINT('Ctrl Pts',(-19.8372102335997,13.1570890487667,124.549046959843)) ;
#80474=CARTESIAN_POINT('Ctrl Pts',(-19.8199077540772,13.1579573332887,124.555404985381)) ;
#80475=CARTESIAN_POINT('Ctrl Pts',(-19.8026384890018,13.1588204336388,124.561314774439)) ;
#80476=CARTESIAN_POINT('Ctrl Pts',(-19.7858523723805,13.1596593867193,124.567059223198)) ;
#80477=CARTESIAN_POINT('Ctrl Pts',(-19.7687146880563,13.1605123080096,124.572508646653)) ;
#80478=CARTESIAN_POINT('Ctrl Pts',(-19.7515162067081,13.1613635178667,124.577557971888)) ;
#80479=CARTESIAN_POINT('Ctrl Pts',(-19.7412079405897,13.1618737081301,124.58058438958)) ;
#80480=CARTESIAN_POINT('Ctrl Pts',(-19.7308781843441,13.1623832835692,124.583468017363)) ;
#80481=CARTESIAN_POINT('Ctrl Pts',(-19.7205920882092,13.1628888680262,124.586194855273)) ;
#80482=CARTESIAN_POINT('Ctrl Pts',(-19.6890331133565,13.1644400616915,124.594561120559)) ;
#80483=CARTESIAN_POINT('Ctrl Pts',(-19.6568234814033,13.1659985862561,124.60173391568)) ;
#80484=CARTESIAN_POINT('Ctrl Pts',(-19.6241856364059,13.1675616636008,124.607599940749)) ;
#80485=CARTESIAN_POINT('Ctrl Pts',(-19.5916847617139,13.1691181812238,124.613441348039)) ;
#80486=CARTESIAN_POINT('Ctrl Pts',(-19.5587598541828,13.1706792134942,124.617986708264)) ;
#80487=CARTESIAN_POINT('Ctrl Pts',(-19.5256469814756,13.1722420171226,124.621173231058)) ;
#80488=CARTESIAN_POINT('Ctrl Pts',(-19.5216231627236,13.1724319263039,124.621560451771)) ;
#80489=CARTESIAN_POINT('Ctrl Pts',(-19.5175965817914,13.1726218616423,124.621927668767)) ;
#80490=CARTESIAN_POINT('Ctrl Pts',(-19.5135676720988,13.1728118182152,124.622274821002)) ;
#80491=CARTESIAN_POINT('Ctrl Pts',(-19.4431860182137,13.1761301993118,124.628339277721)) ;
#80492=CARTESIAN_POINT('Ctrl Pts',(-19.3724202623327,13.1794637724057,124.628252168937)) ;
#80493=CARTESIAN_POINT('Ctrl Pts',(-19.3020841165369,13.1827969618019,124.622022549267)) ;
#80494=CARTESIAN_POINT('Ctrl Pts',(-19.2381208971503,13.1858281418898,124.616357374909)) ;
#80495=CARTESIAN_POINT('Ctrl Pts',(-19.1746816194266,13.1888539155085,124.605623438599)) ;
#80496=CARTESIAN_POINT('Ctrl Pts',(-19.1124419072866,13.1918776184193,124.58994196653)) ;
#80497=CARTESIAN_POINT('Ctrl Pts',(-19.1062917947322,13.1921764005407,124.588392428222)) ;
#80498=CARTESIAN_POINT('Ctrl Pts',(-19.1001533868472,13.1924751624437,124.586794622992)) ;
#80499=CARTESIAN_POINT('Ctrl Pts',(-19.0940273309136,13.1927739073465,124.585148695047)) ;
#80500=CARTESIAN_POINT('Ctrl Pts',(-19.0376030709326,13.1955255080902,124.569988816119)) ;
#80501=CARTESIAN_POINT('Ctrl Pts',(-18.982310761406,13.1982673320755,124.550764643093)) ;
#80502=CARTESIAN_POINT('Ctrl Pts',(-18.9286648343349,13.2010292632919,124.527658425169)) ;
#80503=CARTESIAN_POINT('Ctrl Pts',(-18.9172881129165,13.2016149875722,124.522758276757)) ;
#80504=CARTESIAN_POINT('Ctrl Pts',(-18.9059853714614,13.2022016161536,124.517683712586)) ;
#80505=CARTESIAN_POINT('Ctrl Pts',(-18.8947614126757,13.2027894340587,124.512436753774)) ;
#80506=CARTESIAN_POINT('Ctrl Pts',(-18.8425149448965,13.205525670874,124.488012656203)) ;
#80507=CARTESIAN_POINT('Ctrl Pts',(-18.7920410632873,13.2082605174372,124.459879143387)) ;
#80508=CARTESIAN_POINT('Ctrl Pts',(-18.7438008678464,13.2109629922146,124.428296743651)) ;
#80509=CARTESIAN_POINT('Ctrl Pts',(-18.73273725433,13.2115827893817,124.421053500513)) ;
#80510=CARTESIAN_POINT('Ctrl Pts',(-18.721791021334,13.2122008838315,124.413629037106)) ;
#80511=CARTESIAN_POINT('Ctrl Pts',(-18.7109675360248,13.2128169018266,124.406026829864)) ;
#80512=CARTESIAN_POINT('Ctrl Pts',(-18.6588979399802,13.2157804396561,124.369454150288)) ;
#80513=CARTESIAN_POINT('Ctrl Pts',(-18.6097447256124,13.2187668771422,124.328815918986)) ;
#80514=CARTESIAN_POINT('Ctrl Pts',(-18.5640274925586,13.2218051835985,124.284537275842)) ;
#80515=CARTESIAN_POINT('Ctrl Pts',(-18.559277135695,13.2221208859926,124.279936399054)) ;
#80516=CARTESIAN_POINT('Ctrl Pts',(-18.5545638479963,13.2224371484024,124.275296254488)) ;
#80517=CARTESIAN_POINT('Ctrl Pts',(-18.5498881932309,13.2227540033275,124.270617345238)) ;
#80518=CARTESIAN_POINT('Ctrl Pts',(-18.4997504569173,13.2261516854667,124.2204447106)) ;
#80519=CARTESIAN_POINT('Ctrl Pts',(-18.4540891529611,13.2294902857806,124.165960527441)) ;
#80520=CARTESIAN_POINT('Ctrl Pts',(-18.4134553008324,13.2327808911029,124.107821945015)) ;
#80521=CARTESIAN_POINT('Ctrl Pts',(-18.3918974899517,13.2345266829367,124.076977205982)) ;
#80522=CARTESIAN_POINT('Ctrl Pts',(-18.3718010491922,13.2362874613736,124.045163734806)) ;
#80523=CARTESIAN_POINT('Ctrl Pts',(-18.3532841579246,13.2380562906017,124.012616943459)) ;
#80524=CARTESIAN_POINT('Ctrl Pts',(-18.337148907225,13.2395976132042,123.984256316923)) ;
#80525=CARTESIAN_POINT('Ctrl Pts',(-18.3222124155681,13.2411450487989,123.955339566188)) ;
#80526=CARTESIAN_POINT('Ctrl Pts',(-18.3085229193702,13.2426940083626,123.926034544882)) ;
#80527=CARTESIAN_POINT('Ctrl Pts',(-18.298944521022,13.2437777992861,123.905530125755)) ;
#80528=CARTESIAN_POINT('Ctrl Pts',(-18.2898869625498,13.2448654054133,123.884636235243)) ;
#80529=CARTESIAN_POINT('Ctrl Pts',(-18.2814571063029,13.2459424605924,123.863591097685)) ;
#80530=CARTESIAN_POINT('Ctrl Pts',(-18.2737001243048,13.2469335448281,123.844225790803)) ;
#80531=CARTESIAN_POINT('Ctrl Pts',(-18.2664741872634,13.2479156952537,123.824732962847)) ;
#80532=CARTESIAN_POINT('Ctrl Pts',(-18.259825879779,13.2488777185653,123.80531165987)) ;
#80533=CARTESIAN_POINT('Origin',(-19.4092696390626,-30.19753203383,123.411833654984)) ;
#80534=CARTESIAN_POINT('',(-18.259825879779,12.510900730771,123.80531165987)) ;
#80535=CARTESIAN_POINT('',(-18.259825879779,12.5288903030032,123.80531165987)) ;
#80536=CARTESIAN_POINT('',(-18.259825879779,-30.19753203383,123.80531165987)) ;
#80537=CARTESIAN_POINT('Ctrl Pts',(-18.259825879779,12.870840300276,123.80531165987)) ;
#80538=CARTESIAN_POINT('Ctrl Pts',(-18.2652438286331,12.8700544476548,123.821138789776)) ;
#80539=CARTESIAN_POINT('Ctrl Pts',(-18.2710476408713,12.8692618062305,123.837012818616)) ;
#80540=CARTESIAN_POINT('Ctrl Pts',(-18.2771267299168,12.8684744374755,123.852626496755)) ;
#80541=CARTESIAN_POINT('Ctrl Pts',(-18.2797352125343,12.8681365846007,123.859326186085)) ;
#80542=CARTESIAN_POINT('Ctrl Pts',(-18.282393759643,12.867799702525,123.865978162539)) ;
#80543=CARTESIAN_POINT('Ctrl Pts',(-18.285090905704,12.8674647441515,123.872559247446)) ;
#80544=CARTESIAN_POINT('Ctrl Pts',(-18.2970887061201,12.865974738189,123.901834096284)) ;
#80545=CARTESIAN_POINT('Ctrl Pts',(-18.3103663206228,12.8644630347073,123.930961610968)) ;
#80546=CARTESIAN_POINT('Ctrl Pts',(-18.3248839005837,12.862942247799,123.959696289473)) ;
#80547=CARTESIAN_POINT('Ctrl Pts',(-18.3393287989552,12.8614290746398,123.988287109145)) ;
#80548=CARTESIAN_POINT('Ctrl Pts',(-18.3550011089457,12.8599069087778,124.016488416133)) ;
#80549=CARTESIAN_POINT('Ctrl Pts',(-18.3718124892914,12.858388175797,124.044074557231)) ;
#80550=CARTESIAN_POINT('Ctrl Pts',(-18.3749875471227,12.8581013424172,124.049284575179)) ;
#80551=CARTESIAN_POINT('Ctrl Pts',(-18.3782030986378,12.8578146314863,124.0544727119)) ;
#80552=CARTESIAN_POINT('Ctrl Pts',(-18.3814583607703,12.8575281267115,124.059637539119)) ;
#80553=CARTESIAN_POINT('Ctrl Pts',(-18.4190899396721,12.8542160656237,124.11934412959)) ;
#80554=CARTESIAN_POINT('Ctrl Pts',(-18.4618403115692,12.8509002845194,124.175638483707)) ;
#80555=CARTESIAN_POINT('Ctrl Pts',(-18.5092135497178,12.8475541933109,124.227888145884)) ;
#80556=CARTESIAN_POINT('Ctrl Pts',(-18.5523033632248,12.8445106511806,124.275413463701)) ;
#80557=CARTESIAN_POINT('Ctrl Pts',(-18.5991145856276,12.8414987770607,124.319472287255)) ;
#80558=CARTESIAN_POINT('Ctrl Pts',(-18.6491457361005,12.8384804507046,124.359598155391)) ;
#80559=CARTESIAN_POINT('Ctrl Pts',(-18.6544581856012,12.8381599562488,124.363858833911)) ;
#80560=CARTESIAN_POINT('Ctrl Pts',(-18.6598069062294,12.8378393890454,124.368075204618)) ;
#80561=CARTESIAN_POINT('Ctrl Pts',(-18.6651912734813,12.8375187034571,124.372246733799)) ;
#80562=CARTESIAN_POINT('Ctrl Pts',(-18.7120795895278,12.8347260991437,124.40857337526)) ;
#80563=CARTESIAN_POINT('Ctrl Pts',(-18.7615941697354,12.8319149846304,124.44143451251)) ;
#80564=CARTESIAN_POINT('Ctrl Pts',(-18.8132612855669,12.8291247582724,124.470521493135)) ;
#80565=CARTESIAN_POINT('Ctrl Pts',(-18.823061917314,12.8285954858215,124.476038944248)) ;
#80566=CARTESIAN_POINT('Ctrl Pts',(-18.8329399204803,12.8280669649586,124.481420722888)) ;
#80567=CARTESIAN_POINT('Ctrl Pts',(-18.8428919483362,12.8275394645878,124.486664901056)) ;
#80568=CARTESIAN_POINT('Ctrl Pts',(-18.8949996559076,12.824777531496,124.514122832886)) ;
#80569=CARTESIAN_POINT('Ctrl Pts',(-18.9490737869791,12.8220158289773,124.53777063425)) ;
#80570=CARTESIAN_POINT('Ctrl Pts',(-19.0046041253018,12.8192219391128,124.557386673425)) ;
#80571=CARTESIAN_POINT('Ctrl Pts',(-19.0152882478231,12.8186843904047,124.561160829539)) ;
#80572=CARTESIAN_POINT('Ctrl Pts',(-19.0260262156451,12.8181456501742,124.564785878634)) ;
#80573=CARTESIAN_POINT('Ctrl Pts',(-19.0368143068355,12.8176054875281,124.568260445395)) ;
#80574=CARTESIAN_POINT('Ctrl Pts',(-19.0954403516193,12.8146700655968,124.587142386879)) ;
#80575=CARTESIAN_POINT('Ctrl Pts',(-19.1554537398915,12.8117625018629,124.601546016932)) ;
#80576=CARTESIAN_POINT('Ctrl Pts',(-19.2162518026066,12.8088828516118,124.611329386905)) ;
#80577=CARTESIAN_POINT('Ctrl Pts',(-19.2254481721147,12.8084472731315,124.612809228223)) ;
#80578=CARTESIAN_POINT('Ctrl Pts',(-19.2346624728816,12.8080123333077,124.614183453138)) ;
#80579=CARTESIAN_POINT('Ctrl Pts',(-19.243892594155,12.8075780323319,124.61545167126)) ;
#80580=CARTESIAN_POINT('Ctrl Pts',(-19.3137968124457,12.8042888588397,124.625056506757)) ;
#80581=CARTESIAN_POINT('Ctrl Pts',(-19.3844454421074,12.8009600868674,124.62855644456)) ;
#80582=CARTESIAN_POINT('Ctrl Pts',(-19.4549977610507,12.7975966410503,124.625899071238)) ;
#80583=CARTESIAN_POINT('Ctrl Pts',(-19.4946799715306,12.7957048681525,124.624404429403)) ;
#80584=CARTESIAN_POINT('Ctrl Pts',(-19.5342351639706,12.7938301259445,124.620961938844)) ;
#80585=CARTESIAN_POINT('Ctrl Pts',(-19.5733911893916,12.7919703264446,124.615623509071)) ;
#80586=CARTESIAN_POINT('Ctrl Pts',(-19.6041976335048,12.7905071082365,124.611423439308)) ;
#80587=CARTESIAN_POINT('Ctrl Pts',(-19.6347569943669,12.7890531394645,124.606050872099)) ;
#80588=CARTESIAN_POINT('Ctrl Pts',(-19.6649429132893,12.7876074032817,124.599552928605)) ;
#80589=CARTESIAN_POINT('Ctrl Pts',(-19.6888698339983,12.7864614380023,124.594402322485)) ;
#80590=CARTESIAN_POINT('Ctrl Pts',(-19.712749770549,12.7853054287652,124.588500829333)) ;
#80591=CARTESIAN_POINT('Ctrl Pts',(-19.7363390471498,12.7841509014001,124.581906942594)) ;
#80592=CARTESIAN_POINT('Ctrl Pts',(-19.7588770859414,12.7830478246512,124.575606907302)) ;
#80593=CARTESIAN_POINT('Ctrl Pts',(-19.7811494990811,12.7819461006402,124.568675322403)) ;
#80594=CARTESIAN_POINT('Ctrl Pts',(-19.8029573224534,12.7808557819277,124.561205615679)) ;
#80595=CARTESIAN_POINT('Ctrl Pts',(-19.817043721936,12.7801515087554,124.556380683308)) ;
#80596=CARTESIAN_POINT('Ctrl Pts',(-19.8312706523649,12.7794353947332,124.551213688254)) ;
#80597=CARTESIAN_POINT('Ctrl Pts',(-19.8452968087345,12.7787251458483,124.545820517074)) ;
#80598=CARTESIAN_POINT('Ctrl Pts',(-19.8514774803503,12.7784121723573,124.543443998579)) ;
#80599=CARTESIAN_POINT('Ctrl Pts',(-19.8576193910325,12.7781003377312,124.541024208478)) ;
#80600=CARTESIAN_POINT('Ctrl Pts',(-19.863694495186,12.7777911569645,124.53857406263)) ;
#80601=CARTESIAN_POINT('Ctrl Pts',(-19.8925245790538,12.7763239051763,124.526946622428)) ;
#80602=CARTESIAN_POINT('Ctrl Pts',(-19.9212388608835,12.7748458991295,124.514074790318)) ;
#80603=CARTESIAN_POINT('Ctrl Pts',(-19.9495920023153,12.773356568108,124.499996161163)) ;
#80604=CARTESIAN_POINT('Ctrl Pts',(-19.9777932858638,12.7718752138624,124.485992936381)) ;
#80605=CARTESIAN_POINT('Ctrl Pts',(-20.0056366915137,12.7703826556292,124.470795969259)) ;
#80606=CARTESIAN_POINT('Ctrl Pts',(-20.0328967183668,12.7688783318134,124.45449139463)) ;
#80607=CARTESIAN_POINT('Ctrl Pts',(-20.0388064558109,12.7685522074544,124.450956704231)) ;
#80608=CARTESIAN_POINT('Ctrl Pts',(-20.0446888539843,12.768225530131,124.447370136059)) ;
#80609=CARTESIAN_POINT('Ctrl Pts',(-20.0505417560582,12.767898294121,124.443732859388)) ;
#80610=CARTESIAN_POINT('Ctrl Pts',(-20.110801109042,12.7645291910702,124.406284780456)) ;
#80611=CARTESIAN_POINT('Ctrl Pts',(-20.1676603652674,12.7611694127812,124.363632839701)) ;
#80612=CARTESIAN_POINT('Ctrl Pts',(-20.2204695563796,12.7578667843255,124.31626750565)) ;
#80613=CARTESIAN_POINT('Ctrl Pts',(-20.2727611706988,12.7545965245506,124.269366393777)) ;
#80614=CARTESIAN_POINT('Ctrl Pts',(-20.3209020836178,12.7512924797053,124.217997962919)) ;
#80615=CARTESIAN_POINT('Ctrl Pts',(-20.3642974923925,12.7479375921959,124.162811481188)) ;
#80616=CARTESIAN_POINT('Ctrl Pts',(-20.4002454991736,12.7451584613536,124.117095953312)) ;
#80617=CARTESIAN_POINT('Ctrl Pts',(-20.4328852777677,12.742418077025,124.068825008237)) ;
#80618=CARTESIAN_POINT('Ctrl Pts',(-20.461916599482,12.7396961292568,124.018447430631)) ;
#80619=CARTESIAN_POINT('Ctrl Pts',(-20.4682779426553,12.7390996960657,124.007408695897)) ;
#80620=CARTESIAN_POINT('Ctrl Pts',(-20.4744661969473,12.7385041480797,123.996268922871)) ;
#80621=CARTESIAN_POINT('Ctrl Pts',(-20.4804784836014,12.7379092716233,123.985033015998)) ;
#80622=CARTESIAN_POINT('Ctrl Pts',(-20.5079240155246,12.7351937156767,123.933742141411)) ;
#80623=CARTESIAN_POINT('Ctrl Pts',(-20.5316651272719,12.7324521685231,123.88050941552)) ;
#80624=CARTESIAN_POINT('Ctrl Pts',(-20.5514839489327,12.7296938003856,123.825829266571)) ;
#80625=CARTESIAN_POINT('Ctrl Pts',(-20.5557379593736,12.7291017305311,123.814092447474)) ;
#80626=CARTESIAN_POINT('Ctrl Pts',(-20.559811435531,12.7285088856924,123.802289017377)) ;
#80627=CARTESIAN_POINT('Ctrl Pts',(-20.5637025105913,12.7279153565559,123.790423989276)) ;
#80628=CARTESIAN_POINT('Ctrl Pts',(-20.5826652147322,12.7250228609757,123.732601147511)) ;
#80629=CARTESIAN_POINT('Ctrl Pts',(-20.5972647474954,12.7221506683593,123.673397226161)) ;
#80630=CARTESIAN_POINT('Ctrl Pts',(-20.6073590837758,12.7192993883011,123.61339649519)) ;
#80631=CARTESIAN_POINT('Ctrl Pts',(-20.6089743525134,12.7188431340797,123.603795338435)) ;
#80632=CARTESIAN_POINT('Ctrl Pts',(-20.610474368506,12.7183874153358,123.594173804297)) ;
#80633=CARTESIAN_POINT('Ctrl Pts',(-20.6118586700221,12.717932234567,123.584534317116)) ;
#80634=CARTESIAN_POINT('Ctrl Pts',(-20.6218395159693,12.7146503706968,123.515033391598)) ;
#80635=CARTESIAN_POINT('Ctrl Pts',(-20.6257805720531,12.7113409674474,123.444756157452)) ;
#80636=CARTESIAN_POINT('Ctrl Pts',(-20.6236229978934,12.7079998035975,123.374526604962)) ;
#80637=CARTESIAN_POINT('Ctrl Pts',(-20.6223527583993,12.7060327433881,123.333180007059)) ;
#80638=CARTESIAN_POINT('Ctrl Pts',(-20.6189683608956,12.7040831719724,123.291957810843)) ;
#80639=CARTESIAN_POINT('Ctrl Pts',(-20.6135225780402,12.7021457426414,123.251145276285)) ;
#80640=CARTESIAN_POINT('Ctrl Pts',(-20.6096329606307,12.7007619454802,123.221995170753)) ;
#80641=CARTESIAN_POINT('Ctrl Pts',(-20.6046928480253,12.6993843425356,123.193053959686)) ;
#80642=CARTESIAN_POINT('Ctrl Pts',(-20.5987371476557,12.6980109856402,123.164421161188)) ;
#80643=CARTESIAN_POINT('Ctrl Pts',(-20.5935681866693,12.6968190471993,123.139570713856)) ;
#80644=CARTESIAN_POINT('Ctrl Pts',(-20.5875972158044,12.6956183571829,123.114792440979)) ;
#80645=CARTESIAN_POINT('Ctrl Pts',(-20.5808845007879,12.6944212672785,123.090330137322)) ;
#80646=CARTESIAN_POINT('Ctrl Pts',(-20.5741717857715,12.6932241773741,123.065867833665)) ;
#80647=CARTESIAN_POINT('Ctrl Pts',(-20.5667175537136,12.6920306875816,123.041721989206)) ;
#80648=CARTESIAN_POINT('Ctrl Pts',(-20.5586326678525,12.6908531495887,123.018119895845)) ;
#80649=CARTESIAN_POINT('Ctrl Pts',(-20.5541414064836,12.6901990116096,123.005008619822)) ;
#80650=CARTESIAN_POINT('Ctrl Pts',(-20.5493406381397,12.6895333106017,122.991738989093)) ;
#80651=CARTESIAN_POINT('Ctrl Pts',(-20.5443553865511,12.6888739164767,122.978675205992)) ;
#80652=CARTESIAN_POINT('Ctrl Pts',(-20.5424583250474,12.6886229940933,122.973703982459)) ;
#80653=CARTESIAN_POINT('Ctrl Pts',(-20.5405350594797,12.6883729849888,122.968762386795)) ;
#80654=CARTESIAN_POINT('Ctrl Pts',(-20.5385943316674,12.6881248738665,122.963869778362)) ;
#80655=CARTESIAN_POINT('Ctrl Pts',(-20.5272753794957,12.68667780957,122.93533450387)) ;
#80656=CARTESIAN_POINT('Ctrl Pts',(-20.5147339491118,12.6852153862968,122.906884421184)) ;
#80657=CARTESIAN_POINT('Ctrl Pts',(-20.5010042023758,12.6837414307202,122.878765611155)) ;
#80658=CARTESIAN_POINT('Ctrl Pts',(-20.4873540842985,12.6822760236703,122.850809882293)) ;
#80659=CARTESIAN_POINT('Ctrl Pts',(-20.4725295461049,12.6807992176972,122.823182188348)) ;
#80660=CARTESIAN_POINT('Ctrl Pts',(-20.4566134182114,12.6793147732787,122.796108956468)) ;
#80661=CARTESIAN_POINT('Ctrl Pts',(-20.4526682092607,12.6789468167352,122.789398181243)) ;
#80662=CARTESIAN_POINT('Ctrl Pts',(-20.448656161394,12.6785783908704,122.78272137491)) ;
#80663=CARTESIAN_POINT('Ctrl Pts',(-20.444578985311,12.6782095529563,122.776081774408)) ;
#80664=CARTESIAN_POINT('Ctrl Pts',(-20.4075827945685,12.6748627272253,122.715834210506)) ;
#80665=CARTESIAN_POINT('Ctrl Pts',(-20.3654101310523,12.6715220564939,122.658949047217)) ;
#80666=CARTESIAN_POINT('Ctrl Pts',(-20.3185410461941,12.6682155379078,122.606059862746)) ;
#80667=CARTESIAN_POINT('Ctrl Pts',(-20.2747485812569,12.6651260685979,122.556642474642)) ;
#80668=CARTESIAN_POINT('Ctrl Pts',(-20.2269818742819,12.6620310002448,122.510863018777)) ;
#80669=CARTESIAN_POINT('Ctrl Pts',(-20.1757783500652,12.6588878040927,122.469225416084)) ;
#80670=CARTESIAN_POINT('Ctrl Pts',(-20.1723499810233,12.6586773491183,122.466437540245)) ;
#80671=CARTESIAN_POINT('Ctrl Pts',(-20.1689062175314,12.6584666783836,122.463668218323)) ;
#80672=CARTESIAN_POINT('Ctrl Pts',(-20.1654472267241,12.6582557791229,122.460917595596)) ;
#80673=CARTESIAN_POINT('Ctrl Pts',(-20.1196759772228,12.6554650452884,122.424519858182)) ;
#80674=CARTESIAN_POINT('Ctrl Pts',(-20.0713044553254,12.6526971472822,122.391454374463)) ;
#80675=CARTESIAN_POINT('Ctrl Pts',(-20.0207859716826,12.6499642441057,122.362027162804)) ;
#80676=CARTESIAN_POINT('Ctrl Pts',(-20.0100535520215,12.6493836513866,122.355775486938)) ;
#80677=CARTESIAN_POINT('Ctrl Pts',(-19.9992243363149,12.6488046380909,122.349687861134)) ;
#80678=CARTESIAN_POINT('Ctrl Pts',(-19.9883028378967,12.6482273208029,122.343766966648)) ;
#80679=CARTESIAN_POINT('Ctrl Pts',(-19.9365861933381,12.6454935463847,122.315729715362)) ;
#80680=CARTESIAN_POINT('Ctrl Pts',(-19.8828637603558,12.6427273694508,122.291470213793)) ;
#80681=CARTESIAN_POINT('Ctrl Pts',(-19.8276417803091,12.6399265123786,122.271215117736)) ;
#80682=CARTESIAN_POINT('Ctrl Pts',(-19.8168671346936,12.6393800226956,122.267263041376)) ;
#80683=CARTESIAN_POINT('Ctrl Pts',(-19.8060354655735,12.6388322127423,122.26346326699)) ;
#80684=CARTESIAN_POINT('Ctrl Pts',(-19.7951506272147,12.6382830656004,122.259817266617)) ;
#80685=CARTESIAN_POINT('Ctrl Pts',(-19.7373273714089,12.6353658449111,122.240448709612)) ;
#80686=CARTESIAN_POINT('Ctrl Pts',(-19.6780916519949,12.6324929751349,122.225453540607)) ;
#80687=CARTESIAN_POINT('Ctrl Pts',(-19.6180299855097,12.629644765805,122.214977350395)) ;
#80688=CARTESIAN_POINT('Ctrl Pts',(-19.6082535311584,12.6291811524867,122.213272103082)) ;
#80689=CARTESIAN_POINT('Ctrl Pts',(-19.5984552195503,12.6287181925532,122.21168647846)) ;
#80690=CARTESIAN_POINT('Ctrl Pts',(-19.5886376125502,12.6282558010846,122.210220977716)) ;
#80691=CARTESIAN_POINT('Ctrl Pts',(-19.5189112904046,12.6249718178806,122.19981274107)) ;
#80692=CARTESIAN_POINT('Ctrl Pts',(-19.4483672292415,12.6216433959297,122.195489850219)) ;
#80693=CARTESIAN_POINT('Ctrl Pts',(-19.3778572930884,12.6182833583503,122.197313519044)) ;
#80694=CARTESIAN_POINT('Ctrl Pts',(-19.3352166590783,12.6162513875317,122.198416376303)) ;
#80695=CARTESIAN_POINT('Ctrl Pts',(-19.292692077002,12.614235820897,122.201767656007)) ;
#80696=CARTESIAN_POINT('Ctrl Pts',(-19.2505806312853,12.612237690103,122.207315620709)) ;
#80697=CARTESIAN_POINT('Ctrl Pts',(-19.2229315759349,12.6109257800514,122.210958240441)) ;
#80698=CARTESIAN_POINT('Ctrl Pts',(-19.1954604882387,12.6096213862839,122.215546738106)) ;
#80699=CARTESIAN_POINT('Ctrl Pts',(-19.1682482299057,12.6083248007956,122.221054676159)) ;
#80700=CARTESIAN_POINT('Ctrl Pts',(-19.1422661761438,12.6070868310008,122.226313612806)) ;
#80701=CARTESIAN_POINT('Ctrl Pts',(-19.1163797759702,12.6058411342532,122.232443360207)) ;
#80702=CARTESIAN_POINT('Ctrl Pts',(-19.0908463574102,12.6045965813391,122.239377894716)) ;
#80703=CARTESIAN_POINT('Ctrl Pts',(-19.0653129388503,12.603352028425,122.246312429225)) ;
#80704=CARTESIAN_POINT('Ctrl Pts',(-19.0401330527927,12.6021086193443,122.254051484177)) ;
#80705=CARTESIAN_POINT('Ctrl Pts',(-19.015545705886,12.6008752248834,122.262474111356)) ;
#80706=CARTESIAN_POINT('Ctrl Pts',(-19.0036139187657,12.6002766812423,122.266561457375)) ;
#80707=CARTESIAN_POINT('Ctrl Pts',(-18.9915061483425,12.5996650936151,122.270921283469)) ;
#80708=CARTESIAN_POINT('Ctrl Pts',(-18.9796199090638,12.5990611136394,122.275415155664)) ;
#80709=CARTESIAN_POINT('Ctrl Pts',(-18.9761299444542,12.5988837767466,122.276734618831)) ;
#80710=CARTESIAN_POINT('Ctrl Pts',(-18.9726589616602,12.5987070957027,122.278065314125)) ;
#80711=CARTESIAN_POINT('Ctrl Pts',(-18.9692167198068,12.5985315932456,122.279402939956)) ;
#80712=CARTESIAN_POINT('Ctrl Pts',(-18.9410916850274,12.5970976403397,122.29033208864)) ;
#80713=CARTESIAN_POINT('Ctrl Pts',(-18.9130159442305,12.5956536956959,122.302452626089)) ;
#80714=CARTESIAN_POINT('Ctrl Pts',(-18.8852362505225,12.5942025436577,122.31573379467)) ;
#80715=CARTESIAN_POINT('Ctrl Pts',(-18.8576318509199,12.5927605486102,122.328931157051)) ;
#80716=CARTESIAN_POINT('Ctrl Pts',(-18.8303203638607,12.591311436841,122.343274407333)) ;
#80717=CARTESIAN_POINT('Ctrl Pts',(-18.8035290017548,12.5898579403164,122.358684009208)) ;
#80718=CARTESIAN_POINT('Ctrl Pts',(-18.7958378539878,12.5894406768527,122.363107730726)) ;
#80719=CARTESIAN_POINT('Ctrl Pts',(-18.78818944604,12.5890230520307,122.367619028999)) ;
#80720=CARTESIAN_POINT('Ctrl Pts',(-18.7805888210449,12.5886051304848,122.372215299461)) ;
#80721=CARTESIAN_POINT('Ctrl Pts',(-18.7198680009331,12.5852663867599,122.408934557692)) ;
#80722=CARTESIAN_POINT('Ctrl Pts',(-18.6624972427602,12.5819070867189,122.450892105939)) ;
#80723=CARTESIAN_POINT('Ctrl Pts',(-18.6091191273835,12.5785748167538,122.497609910628)) ;
#80724=CARTESIAN_POINT('Ctrl Pts',(-18.5777387961616,12.576615816619,122.525074727899)) ;
#80725=CARTESIAN_POINT('Ctrl Pts',(-18.5478029560891,12.5746631140264,122.554134352609)) ;
#80726=CARTESIAN_POINT('Ctrl Pts',(-18.5195056024907,12.5727088655747,122.584569576646)) ;
#80727=CARTESIAN_POINT('Ctrl Pts',(-18.4999106558522,12.5713556155616,122.605644925225)) ;
#80728=CARTESIAN_POINT('Ctrl Pts',(-18.481100615183,12.5700016242955,122.627379084785)) ;
#80729=CARTESIAN_POINT('Ctrl Pts',(-18.4631281010885,12.5686442874272,122.649690567234)) ;
#80730=CARTESIAN_POINT('Ctrl Pts',(-18.4363506617847,12.5666219768359,122.682932681495)) ;
#80731=CARTESIAN_POINT('Ctrl Pts',(-18.4112434404779,12.5645976075795,122.717694317056)) ;
#80732=CARTESIAN_POINT('Ctrl Pts',(-18.3880097318216,12.5625726742712,122.753749999248)) ;
#80733=CARTESIAN_POINT('Ctrl Pts',(-18.3647956860237,12.5605494546788,122.789775167252)) ;
#80734=CARTESIAN_POINT('Ctrl Pts',(-18.3434523867715,12.5585256719889,122.82709168502)) ;
#80735=CARTESIAN_POINT('Ctrl Pts',(-18.3241416998298,12.5565028170232,122.865442539042)) ;
#80736=CARTESIAN_POINT('Ctrl Pts',(-18.3048298827935,12.5544798436765,122.903795637421)) ;
#80737=CARTESIAN_POINT('Ctrl Pts',(-18.2875512170765,12.5524577981627,122.943182616963)) ;
#80738=CARTESIAN_POINT('Ctrl Pts',(-18.2724213519401,12.5504381715651,122.983322432084)) ;
#80739=CARTESIAN_POINT('Ctrl Pts',(-18.2678973567496,12.5498342811186,122.995324675919)) ;
#80740=CARTESIAN_POINT('Ctrl Pts',(-18.2635651510703,12.5492306069413,123.007394098955)) ;
#80741=CARTESIAN_POINT('Ctrl Pts',(-18.2594269703917,12.5486271888959,123.019522893739)) ;
#80742=CARTESIAN_POINT('Ctrl Pts',(-18.2435244538054,12.5463083279707,123.06613235215)) ;
#80743=CARTESIAN_POINT('Ctrl Pts',(-18.2304408727889,12.543969043762,123.113766337352)) ;
#80744=CARTESIAN_POINT('Ctrl Pts',(-18.2202951051978,12.5416357742674,123.162062852235)) ;
#80745=CARTESIAN_POINT('Ctrl Pts',(-18.215944345221,12.5406352097028,123.182773610892)) ;
#80746=CARTESIAN_POINT('Ctrl Pts',(-18.2121332123063,12.5396357511898,123.203605972904)) ;
#80747=CARTESIAN_POINT('Ctrl Pts',(-18.2088682788955,12.5386394835517,123.224530503399)) ;
#80748=CARTESIAN_POINT('Ctrl Pts',(-18.1979762759186,12.5353158782233,123.29433592353)) ;
#80749=CARTESIAN_POINT('Ctrl Pts',(-18.1931905831683,12.532009642944,123.364997383629)) ;
#80750=CARTESIAN_POINT('Ctrl Pts',(-18.1945771249853,12.5286466831811,123.435666244636)) ;
#80751=CARTESIAN_POINT('Ctrl Pts',(-18.1954453231439,12.5265409295443,123.479916316467)) ;
#80752=CARTESIAN_POINT('Ctrl Pts',(-18.1987345660899,12.524445018058,123.524055666228)) ;
#80753=CARTESIAN_POINT('Ctrl Pts',(-18.2043922934707,12.5223708167657,123.567771072445)) ;
#80754=CARTESIAN_POINT('Ctrl Pts',(-18.2078100782309,12.5211178094909,123.594179175752)) ;
#80755=CARTESIAN_POINT('Ctrl Pts',(-18.2120911794677,12.5198727248409,123.620432721153)) ;
#80756=CARTESIAN_POINT('Ctrl Pts',(-18.217215114198,12.5186381791136,123.64646508049)) ;
#80757=CARTESIAN_POINT('Ctrl Pts',(-18.2221197203024,12.5174564777787,123.671383131799)) ;
#80758=CARTESIAN_POINT('Ctrl Pts',(-18.2278209212937,12.5162682169221,123.69620254406)) ;
#80759=CARTESIAN_POINT('Ctrl Pts',(-18.2342563280413,12.5150802068191,123.720685747429)) ;
#80760=CARTESIAN_POINT('Ctrl Pts',(-18.2407347997116,12.5138842467038,123.745332789279)) ;
#80761=CARTESIAN_POINT('Ctrl Pts',(-18.2479571476,12.5126885407095,123.769638609505)) ;
#80762=CARTESIAN_POINT('Ctrl Pts',(-18.2558095264191,12.511500036749,123.793377446213)) ;
#80763=CARTESIAN_POINT('Ctrl Pts',(-18.2571308068481,12.5113000531442,123.797371861291)) ;
#80764=CARTESIAN_POINT('Ctrl Pts',(-18.2584698156533,12.5111002734513,123.801350270854)) ;
#80765=CARTESIAN_POINT('Ctrl Pts',(-18.259825879779,12.510900730771,123.80531165987)) ;
#80766=CARTESIAN_POINT('Ctrl Pts',(-18.259825879779,12.5288903030032,123.80531165987)) ;
#80767=CARTESIAN_POINT('Ctrl Pts',(-18.2524098048089,12.5299743464015,123.783647523662)) ;
#80768=CARTESIAN_POINT('Ctrl Pts',(-18.2455076163158,12.5310699985716,123.761472531738)) ;
#80769=CARTESIAN_POINT('Ctrl Pts',(-18.2392292933661,12.5321671007081,123.739020888121)) ;
#80770=CARTESIAN_POINT('Ctrl Pts',(-18.2331128960579,12.5332359072362,123.717148299901)) ;
#80771=CARTESIAN_POINT('Ctrl Pts',(-18.227588592158,12.5343060899024,123.695013616499)) ;
#80772=CARTESIAN_POINT('Ctrl Pts',(-18.2227126740053,12.5353682558269,123.672847954897)) ;
#80773=CARTESIAN_POINT('Ctrl Pts',(-18.2144906444783,12.5371593358493,123.635471051005)) ;
#80774=CARTESIAN_POINT('Ctrl Pts',(-18.2079926912785,12.5389655205004,123.597494755401)) ;
#80775=CARTESIAN_POINT('Ctrl Pts',(-18.2033107178565,12.5407863761254,123.559173318512)) ;
#80776=CARTESIAN_POINT('Ctrl Pts',(-18.1994966225247,12.5422697072581,123.527955368222)) ;
#80777=CARTESIAN_POINT('Ctrl Pts',(-18.1968868214949,12.543762774471,123.496508937966)) ;
#80778=CARTESIAN_POINT('Ctrl Pts',(-18.1955062474138,12.5452653433241,123.464978035478)) ;
#80779=CARTESIAN_POINT('Ctrl Pts',(-18.1924157706671,12.5486289108168,123.39439470187)) ;
#80780=CARTESIAN_POINT('Ctrl Pts',(-18.1954901578647,12.5519576978783,123.323659203646)) ;
#80781=CARTESIAN_POINT('Ctrl Pts',(-18.2046884819164,12.5552556142764,123.25362451513)) ;
#80782=CARTESIAN_POINT('Ctrl Pts',(-18.2127932845956,12.5581614655498,123.191915737757)) ;
#80783=CARTESIAN_POINT('Ctrl Pts',(-18.2256359409674,12.561085567277,123.13089343027)) ;
#80784=CARTESIAN_POINT('Ctrl Pts',(-18.2430795069021,12.5640439274076,123.071177711639)) ;
#80785=CARTESIAN_POINT('Ctrl Pts',(-18.2453973836478,12.5644370301813,123.063242770121)) ;
#80786=CARTESIAN_POINT('Ctrl Pts',(-18.2477964241806,12.5648307378462,123.055330881221)) ;
#80787=CARTESIAN_POINT('Ctrl Pts',(-18.2502762395728,12.5652250879601,123.047443484941)) ;
#80788=CARTESIAN_POINT('Ctrl Pts',(-18.2675896731787,12.5679783390837,122.992375711655)) ;
#80789=CARTESIAN_POINT('Ctrl Pts',(-18.2888214169512,12.5707060852376,122.938576593479)) ;
#80790=CARTESIAN_POINT('Ctrl Pts',(-18.3137738281503,12.5734075221599,122.886538667041)) ;
#80791=CARTESIAN_POINT('Ctrl Pts',(-18.3194690820111,12.5740241106306,122.874661289777)) ;
#80792=CARTESIAN_POINT('Ctrl Pts',(-18.3253579683102,12.5746393285058,122.862875580663)) ;
#80793=CARTESIAN_POINT('Ctrl Pts',(-18.3314377858075,12.5752531662224,122.851187249312)) ;
#80794=CARTESIAN_POINT('Ctrl Pts',(-18.3589039783336,12.5780262403996,122.798384026295)) ;
#80795=CARTESIAN_POINT('Ctrl Pts',(-18.3902368225375,12.5808351609625,122.74763471134)) ;
#80796=CARTESIAN_POINT('Ctrl Pts',(-18.4251361962623,12.5836604667693,122.699424178035)) ;
#80797=CARTESIAN_POINT('Ctrl Pts',(-18.431459525935,12.5841723768162,122.690689032866)) ;
#80798=CARTESIAN_POINT('Ctrl Pts',(-18.4378998236653,12.5846848247728,122.682037160603)) ;
#80799=CARTESIAN_POINT('Ctrl Pts',(-18.4444551479089,12.5851976948804,122.673471349781)) ;
#80800=CARTESIAN_POINT('Ctrl Pts',(-18.4842452315836,12.5883107589698,122.621477837839)) ;
#80801=CARTESIAN_POINT('Ctrl Pts',(-18.5282007356626,12.5913740642443,122.572756774188)) ;
#80802=CARTESIAN_POINT('Ctrl Pts',(-18.5758383764271,12.594457279894,122.5278437079)) ;
#80803=CARTESIAN_POINT('Ctrl Pts',(-18.5797969386911,12.59471348698,122.524111550586)) ;
#80804=CARTESIAN_POINT('Ctrl Pts',(-18.5837809041891,12.5949698315505,122.520405668711)) ;
#80805=CARTESIAN_POINT('Ctrl Pts',(-18.58778998298,12.5952263535819,122.516726359333)) ;
#80806=CARTESIAN_POINT('Ctrl Pts',(-18.6400446190422,12.5985698811328,122.468769962743)) ;
#80807=CARTESIAN_POINT('Ctrl Pts',(-18.6964140289307,12.6019299757216,122.425469517297)) ;
#80808=CARTESIAN_POINT('Ctrl Pts',(-18.7562282492783,12.6052545103643,122.387342152182)) ;
#80809=CARTESIAN_POINT('Ctrl Pts',(-18.7837994777867,12.6067869470287,122.369767430153)) ;
#80810=CARTESIAN_POINT('Ctrl Pts',(-18.8120526841263,12.6083230835739,122.353328360479)) ;
#80811=CARTESIAN_POINT('Ctrl Pts',(-18.8407669229486,12.6098552748236,122.338124868648)) ;
#80812=CARTESIAN_POINT('Ctrl Pts',(-18.8696086665945,12.6113942697283,122.322853866111)) ;
#80813=CARTESIAN_POINT('Ctrl Pts',(-18.898914945886,12.6129292842218,122.30882964563)) ;
#80814=CARTESIAN_POINT('Ctrl Pts',(-18.9284433577873,12.6144525708304,122.296104304595)) ;
#80815=CARTESIAN_POINT('Ctrl Pts',(-18.9326689618149,12.6146705576984,122.294283270247)) ;
#80816=CARTESIAN_POINT('Ctrl Pts',(-18.9368990930012,12.6148883043974,122.292488750564)) ;
#80817=CARTESIAN_POINT('Ctrl Pts',(-18.9411330215784,12.615105788223,122.290720813449)) ;
#80818=CARTESIAN_POINT('Ctrl Pts',(-18.956775472796,12.6159092925976,122.284189085392)) ;
#80819=CARTESIAN_POINT('Ctrl Pts',(-18.9727748193308,12.6167226885707,122.277897489621)) ;
#80820=CARTESIAN_POINT('Ctrl Pts',(-18.9888360565228,12.6175313828714,122.271973357072)) ;
#80821=CARTESIAN_POINT('Ctrl Pts',(-18.99777159258,12.6179812932362,122.268677515078)) ;
#80822=CARTESIAN_POINT('Ctrl Pts',(-19.0067259121831,12.6184297483577,122.265494551706)) ;
#80823=CARTESIAN_POINT('Ctrl Pts',(-19.0156457967525,12.6188742353227,122.262439829157)) ;
#80824=CARTESIAN_POINT('Ctrl Pts',(-19.0372180981158,12.6199492051485,122.255052133174)) ;
#80825=CARTESIAN_POINT('Ctrl Pts',(-19.0592532219469,12.621033427544,122.248189030563)) ;
#80826=CARTESIAN_POINT('Ctrl Pts',(-19.0815133831771,12.6221207014324,122.24195257863)) ;
#80827=CARTESIAN_POINT('Ctrl Pts',(-19.1008724951719,12.6230662766579,122.236528890536)) ;
#80828=CARTESIAN_POINT('Ctrl Pts',(-19.1204012977472,12.6240141598346,122.231578502887)) ;
#80829=CARTESIAN_POINT('Ctrl Pts',(-19.1399340122772,12.6249602721053,122.227137822195)) ;
#80830=CARTESIAN_POINT('Ctrl Pts',(-19.1762012395167,12.6267169592603,122.218892620253)) ;
#80831=CARTESIAN_POINT('Ctrl Pts',(-19.2130824695728,12.6284881998387,122.212263669636)) ;
#80832=CARTESIAN_POINT('Ctrl Pts',(-19.2503316275509,12.6302618249869,122.207348451845)) ;
#80833=CARTESIAN_POINT('Ctrl Pts',(-19.2831219408442,12.6318231414685,122.203021601521)) ;
#80834=CARTESIAN_POINT('Ctrl Pts',(-19.3161967553501,12.6333863058065,122.200022166535)) ;
#80835=CARTESIAN_POINT('Ctrl Pts',(-19.3493790843881,12.6349430168755,122.198384431677)) ;
#80836=CARTESIAN_POINT('Ctrl Pts',(-19.4195611623873,12.6382355289092,122.194920550783)) ;
#80837=CARTESIAN_POINT('Ctrl Pts',(-19.4898965900153,12.64154805959,122.197553795608)) ;
#80838=CARTESIAN_POINT('Ctrl Pts',(-19.5595738808095,12.6448737795494,122.206240634518)) ;
#80839=CARTESIAN_POINT('Ctrl Pts',(-19.6205231923216,12.6477829101929,122.213839334822)) ;
#80840=CARTESIAN_POINT('Ctrl Pts',(-19.6808395885297,12.6506640612106,122.226057302673)) ;
#80841=CARTESIAN_POINT('Ctrl Pts',(-19.7399214211662,12.6535589646203,122.242767662375)) ;
#80842=CARTESIAN_POINT('Ctrl Pts',(-19.748705562942,12.6539893717496,122.245252117616)) ;
#80843=CARTESIAN_POINT('Ctrl Pts',(-19.757462435201,12.6544200828757,122.247835785701)) ;
#80844=CARTESIAN_POINT('Ctrl Pts',(-19.7661900808373,12.6548512351516,122.250518153353)) ;
#80845=CARTESIAN_POINT('Ctrl Pts',(-19.8214982695661,12.6575835013827,122.267516654731)) ;
#80846=CARTESIAN_POINT('Ctrl Pts',(-19.8755571439978,12.6603208780004,122.288460053437)) ;
#80847=CARTESIAN_POINT('Ctrl Pts',(-19.9278701708427,12.6630421379963,122.313152907669)) ;
#80848=CARTESIAN_POINT('Ctrl Pts',(-19.9397012183738,12.6636575746915,122.318737412135)) ;
#80849=CARTESIAN_POINT('Ctrl Pts',(-19.9514430490475,12.6642721870574,122.324513497708)) ;
#80850=CARTESIAN_POINT('Ctrl Pts',(-19.9630900591537,12.6648857295504,122.330478561421)) ;
#80851=CARTESIAN_POINT('Ctrl Pts',(-20.0155103716858,12.6676471326004,122.357325838214)) ;
#80852=CARTESIAN_POINT('Ctrl Pts',(-20.0659434995834,12.670415136917,122.387971786902)) ;
#80853=CARTESIAN_POINT('Ctrl Pts',(-20.1139149856316,12.6732053908043,122.422126207481)) ;
#80854=CARTESIAN_POINT('Ctrl Pts',(-20.1235337418823,12.673764864238,122.428974505783)) ;
#80855=CARTESIAN_POINT('Ctrl Pts',(-20.1330536178746,12.6743252321981,122.435963716956)) ;
#80856=CARTESIAN_POINT('Ctrl Pts',(-20.1424709209913,12.6748866208308,122.443091286621)) ;
#80857=CARTESIAN_POINT('Ctrl Pts',(-20.1928674284073,12.6778908807596,122.481234331716)) ;
#80858=CARTESIAN_POINT('Ctrl Pts',(-20.2402378432288,12.6808711487217,122.523277860457)) ;
#80859=CARTESIAN_POINT('Ctrl Pts',(-20.2840898649842,12.6838320550256,122.568782370421)) ;
#80860=CARTESIAN_POINT('Ctrl Pts',(-20.2894033086905,12.6841908209008,122.574296042138)) ;
#80861=CARTESIAN_POINT('Ctrl Pts',(-20.2946651383711,12.6845493025163,122.579860479491)) ;
#80862=CARTESIAN_POINT('Ctrl Pts',(-20.2998745118911,12.6849075081088,122.585474860889)) ;
#80863=CARTESIAN_POINT('Ctrl Pts',(-20.3477823131988,12.6882017319327,122.637107301417)) ;
#80864=CARTESIAN_POINT('Ctrl Pts',(-20.3911284512309,12.6915271808586,122.692829797445)) ;
#80865=CARTESIAN_POINT('Ctrl Pts',(-20.4294058110033,12.6948703138278,122.752009370206)) ;
#80866=CARTESIAN_POINT('Ctrl Pts',(-20.4475133760429,12.6964518230552,122.780004978293)) ;
#80867=CARTESIAN_POINT('Ctrl Pts',(-20.4644420267259,12.6980235182476,122.808712988296)) ;
#80868=CARTESIAN_POINT('Ctrl Pts',(-20.4800910780841,12.6995841135068,122.837910888563)) ;
#80869=CARTESIAN_POINT('Ctrl Pts',(-20.4958052812698,12.7011512060054,122.867230348694)) ;
#80870=CARTESIAN_POINT('Ctrl Pts',(-20.5102290000787,12.7027071059535,122.897043180513)) ;
#80871=CARTESIAN_POINT('Ctrl Pts',(-20.523309439146,12.7042505113249,122.927105669496)) ;
#80872=CARTESIAN_POINT('Ctrl Pts',(-20.524841996152,12.7044313429241,122.930627911974)) ;
#80873=CARTESIAN_POINT('Ctrl Pts',(-20.5263561703865,12.7046120030052,122.934153567087)) ;
#80874=CARTESIAN_POINT('Ctrl Pts',(-20.5278519224255,12.7047924894739,122.937682232513)) ;
#80875=CARTESIAN_POINT('Ctrl Pts',(-20.5348041812293,12.705631390982,122.95408347726)) ;
#80876=CARTESIAN_POINT('Ctrl Pts',(-20.5414808187029,12.7064832685371,122.970849510673)) ;
#80877=CARTESIAN_POINT('Ctrl Pts',(-20.5477576521918,12.7073326882528,122.987698134135)) ;
#80878=CARTESIAN_POINT('Ctrl Pts',(-20.5515482935938,12.7078456611631,122.997873183349)) ;
#80879=CARTESIAN_POINT('Ctrl Pts',(-20.5551940473909,12.7083577376821,123.008077933982)) ;
#80880=CARTESIAN_POINT('Ctrl Pts',(-20.5586762065934,12.7088655184933,123.018247020808)) ;
#80881=CARTESIAN_POINT('Ctrl Pts',(-20.5658397893312,12.7099101375478,123.039167113949)) ;
#80882=CARTESIAN_POINT('Ctrl Pts',(-20.5725121880288,12.7109660365692,123.060529591782)) ;
#80883=CARTESIAN_POINT('Ctrl Pts',(-20.5785924632154,12.7120216609084,123.082091287369)) ;
#80884=CARTESIAN_POINT('Ctrl Pts',(-20.58360867267,12.7128925479371,123.099879623907)) ;
#80885=CARTESIAN_POINT('Ctrl Pts',(-20.5882226913621,12.7137632480116,123.117803051032)) ;
#80886=CARTESIAN_POINT('Ctrl Pts',(-20.5924034687724,12.7146272730841,123.135717307983)) ;
#80887=CARTESIAN_POINT('Ctrl Pts',(-20.6006051681473,12.7163222865232,123.170860855611)) ;
#80888=CARTESIAN_POINT('Ctrl Pts',(-20.6072936634496,12.7180282649194,123.206614212993)) ;
#80889=CARTESIAN_POINT('Ctrl Pts',(-20.6123708257249,12.7197467163026,123.242737733281)) ;
#80890=CARTESIAN_POINT('Ctrl Pts',(-20.6170581982933,12.7213332367715,123.276087937369)) ;
#80891=CARTESIAN_POINT('Ctrl Pts',(-20.6203725208227,12.7229303885638,123.309753023635)) ;
#80892=CARTESIAN_POINT('Ctrl Pts',(-20.6222745883944,12.724539358364,123.34353366244)) ;
#80893=CARTESIAN_POINT('Ctrl Pts',(-20.6262623466444,12.7279126257966,123.414356078574)) ;
#80894=CARTESIAN_POINT('Ctrl Pts',(-20.6240383934404,12.7312613121533,123.485408065895)) ;
#80895=CARTESIAN_POINT('Ctrl Pts',(-20.6156319034181,12.7345698810621,123.555833596735)) ;
#80896=CARTESIAN_POINT('Ctrl Pts',(-20.6081187423961,12.7375268596463,123.618775246799)) ;
#80897=CARTESIAN_POINT('Ctrl Pts',(-20.5956838500786,12.7405056930328,123.681057206444)) ;
#80898=CARTESIAN_POINT('Ctrl Pts',(-20.5784645379807,12.7435210083962,123.742029330954)) ;
#80899=CARTESIAN_POINT('Ctrl Pts',(-20.5765123326015,12.743862863799,123.748941924719)) ;
#80900=CARTESIAN_POINT('Ctrl Pts',(-20.5744986845941,12.7442051881207,123.755837694971)) ;
#80901=CARTESIAN_POINT('Ctrl Pts',(-20.5724238354329,12.7445480026765,123.762715702902)) ;
#80902=CARTESIAN_POINT('Ctrl Pts',(-20.5557105155931,12.7473094416402,123.81811941541)) ;
#80903=CARTESIAN_POINT('Ctrl Pts',(-20.5350449674215,12.7500407281243,123.872293178228)) ;
#80904=CARTESIAN_POINT('Ctrl Pts',(-20.5106204324781,12.7527494963095,123.924739422088)) ;
#80905=CARTESIAN_POINT('Ctrl Pts',(-20.5051200868351,12.7533595042921,123.936550188171)) ;
#80906=CARTESIAN_POINT('Ctrl Pts',(-20.4994293020387,12.753968370283,123.948273423035)) ;
#80907=CARTESIAN_POINT('Ctrl Pts',(-20.4935506230553,12.7545761814695,123.959903581031)) ;
#80908=CARTESIAN_POINT('Ctrl Pts',(-20.4668860643504,12.7573330962648,124.012655743805)) ;
#80909=CARTESIAN_POINT('Ctrl Pts',(-20.4363847262239,12.760127225549,124.063426780408)) ;
#80910=CARTESIAN_POINT('Ctrl Pts',(-20.4023365548253,12.7629283003074,124.111736503173)) ;
#80911=CARTESIAN_POINT('Ctrl Pts',(-20.3959454412135,12.7634540844033,124.12080462384)) ;
#80912=CARTESIAN_POINT('Ctrl Pts',(-20.3894294835363,12.7639801132181,124.129786098529)) ;
#80913=CARTESIAN_POINT('Ctrl Pts',(-20.3827907748379,12.7645061865598,124.138677857193)) ;
#80914=CARTESIAN_POINT('Ctrl Pts',(-20.3436549708646,12.7676074377384,124.191095599836)) ;
#80915=CARTESIAN_POINT('Ctrl Pts',(-20.3003200443191,12.7706663358612,124.240299227947)) ;
#80916=CARTESIAN_POINT('Ctrl Pts',(-20.2532605411037,12.7737563344538,124.285747411231)) ;
#80917=CARTESIAN_POINT('Ctrl Pts',(-20.2495339480594,12.7740010282239,124.289346405528)) ;
#80918=CARTESIAN_POINT('Ctrl Pts',(-20.2457840194963,12.7742459170217,124.292921867039)) ;
#80919=CARTESIAN_POINT('Ctrl Pts',(-20.2420110021608,12.7744910373231,124.29647353554)) ;
#80920=CARTESIAN_POINT('Ctrl Pts',(-20.1903647834785,12.7778463192005,124.345089863483)) ;
#80921=CARTESIAN_POINT('Ctrl Pts',(-20.1345459269395,12.7812066706123,124.389101475417)) ;
#80922=CARTESIAN_POINT('Ctrl Pts',(-20.075214192574,12.7845191703928,124.427985094354)) ;
#80923=CARTESIAN_POINT('Ctrl Pts',(-20.0457376691239,12.7861648491936,124.447302815599)) ;
#80924=CARTESIAN_POINT('Ctrl Pts',(-20.0154524966392,12.7878143806419,124.465310970758)) ;
#80925=CARTESIAN_POINT('Ctrl Pts',(-19.9846105575071,12.7894647330416,124.481893804531)) ;
#80926=CARTESIAN_POINT('Ctrl Pts',(-19.9537686183751,12.7911150854413,124.498476638304)) ;
#80927=CARTESIAN_POINT('Ctrl Pts',(-19.9223706627251,12.7927662587925,124.513633935522)) ;
#80928=CARTESIAN_POINT('Ctrl Pts',(-19.890689853112,12.7944152213991,124.527306861112)) ;
#80929=CARTESIAN_POINT('Ctrl Pts',(-19.8733675535382,12.7953168342243,124.534782885747)) ;
#80930=CARTESIAN_POINT('Ctrl Pts',(-19.8556736911802,12.7962290946323,124.541935886302)) ;
#80931=CARTESIAN_POINT('Ctrl Pts',(-19.837877219646,12.7971348160649,124.548645617426)) ;
#80932=CARTESIAN_POINT('Ctrl Pts',(-19.826205722036,12.7977288172698,124.553046074598)) ;
#80933=CARTESIAN_POINT('Ctrl Pts',(-19.8144905578315,12.7983200059584,124.557256844807)) ;
#80934=CARTESIAN_POINT('Ctrl Pts',(-19.8028118584132,12.7989035340819,124.561255430345)) ;
#80935=CARTESIAN_POINT('Ctrl Pts',(-19.7826198328396,12.7999124319371,124.568168832134)) ;
#80936=CARTESIAN_POINT('Ctrl Pts',(-19.7620048595353,12.8009244496695,124.574628037106)) ;
#80937=CARTESIAN_POINT('Ctrl Pts',(-19.7412166057261,12.8019330346865,124.580532550084)) ;
#80938=CARTESIAN_POINT('Ctrl Pts',(-19.7249347561583,12.8027229822057,124.585157103593)) ;
#80939=CARTESIAN_POINT('Ctrl Pts',(-19.7085470911927,12.8035108239631,124.589442309953)) ;
#80940=CARTESIAN_POINT('Ctrl Pts',(-19.6921799650699,12.8042934117004,124.593361328602)) ;
#80941=CARTESIAN_POINT('Ctrl Pts',(-19.6579132877952,12.8059318594787,124.601566296674)) ;
#80942=CARTESIAN_POINT('Ctrl Pts',(-19.6230334882165,12.8075974503459,124.608337509049)) ;
#80943=CARTESIAN_POINT('Ctrl Pts',(-19.5877754174827,12.8092799940258,124.613574718257)) ;
#80944=CARTESIAN_POINT('Ctrl Pts',(-19.5539179714286,12.8108956987621,124.618603879653)) ;
#80945=CARTESIAN_POINT('Ctrl Pts',(-19.5197123376266,12.812527036165,124.6222186044)) ;
#80946=CARTESIAN_POINT('Ctrl Pts',(-19.4853790432398,12.8141649827786,124.624373656255)) ;
#80947=CARTESIAN_POINT('Ctrl Pts',(-19.4145452746383,12.8175442661676,124.628819790748)) ;
#80948=CARTESIAN_POINT('Ctrl Pts',(-19.343435013163,12.8208579572261,124.627048899914)) ;
#80949=CARTESIAN_POINT('Ctrl Pts',(-19.2729158335981,12.8242010480661,124.619084058099)) ;
#80950=CARTESIAN_POINT('Ctrl Pts',(-19.2097868481366,12.827193793222,124.611953907319)) ;
#80951=CARTESIAN_POINT('Ctrl Pts',(-19.1472852309664,12.8302092116872,124.599875437733)) ;
#80952=CARTESIAN_POINT('Ctrl Pts',(-19.0860661233276,12.8331908220591,124.582980692508)) ;
#80953=CARTESIAN_POINT('Ctrl Pts',(-19.0788994638717,12.8335398664504,124.581002896845)) ;
#80954=CARTESIAN_POINT('Ctrl Pts',(-19.0717503683076,12.8338884475227,124.578959154462)) ;
#80955=CARTESIAN_POINT('Ctrl Pts',(-19.0646198790754,12.8342364746619,124.576849723125)) ;
#80956=CARTESIAN_POINT('Ctrl Pts',(-19.0078934037652,12.8370051981361,124.560068181106)) ;
#80957=CARTESIAN_POINT('Ctrl Pts',(-18.9524364073411,12.8397779519758,124.539151933304)) ;
#80958=CARTESIAN_POINT('Ctrl Pts',(-18.8987731161,12.8425868853042,124.514303244646)) ;
#80959=CARTESIAN_POINT('Ctrl Pts',(-18.8886143406051,12.8431186328434,124.509599242271)) ;
#80960=CARTESIAN_POINT('Ctrl Pts',(-18.8785197895817,12.8436516769365,124.504754453293)) ;
#80961=CARTESIAN_POINT('Ctrl Pts',(-18.8684929416447,12.8441862356861,124.499770445251)) ;
#80962=CARTESIAN_POINT('Ctrl Pts',(-18.816742531374,12.8469451919186,124.474047061129)) ;
#80963=CARTESIAN_POINT('Ctrl Pts',(-18.7668609318805,12.8496745801071,124.444642998157)) ;
#80964=CARTESIAN_POINT('Ctrl Pts',(-18.7193050246574,12.8523779218263,124.411831018458)) ;
#80965=CARTESIAN_POINT('Ctrl Pts',(-18.7085176446678,12.8529911363788,124.404388088359)) ;
#80966=CARTESIAN_POINT('Ctrl Pts',(-18.6978498211941,12.8536030107243,124.396769986417)) ;
#80967=CARTESIAN_POINT('Ctrl Pts',(-18.6873066910414,12.8542135859656,124.388980213986)) ;
#80968=CARTESIAN_POINT('Ctrl Pts',(-18.6357053940623,12.8572019275588,124.350854690087)) ;
#80969=CARTESIAN_POINT('Ctrl Pts',(-18.5871692007383,12.8602368807547,124.308669656888)) ;
#80970=CARTESIAN_POINT('Ctrl Pts',(-18.542217609392,12.8632832123375,124.262872240437)) ;
#80971=CARTESIAN_POINT('Ctrl Pts',(-18.5379626773981,12.8635715655043,124.258537246132)) ;
#80972=CARTESIAN_POINT('Ctrl Pts',(-18.5337398383119,12.8638600206183,124.254169915882)) ;
#80973=CARTESIAN_POINT('Ctrl Pts',(-18.5295495179456,12.8641485477988,124.249770648193)) ;
#80974=CARTESIAN_POINT('Ctrl Pts',(-18.4807966480294,12.8675054577398,124.198586751342)) ;
#80975=CARTESIAN_POINT('Ctrl Pts',(-18.4365915825538,12.8708059686782,124.143232112355)) ;
#80976=CARTESIAN_POINT('Ctrl Pts',(-18.39744901714,12.8741441467103,124.084340104869)) ;
#80977=CARTESIAN_POINT('Ctrl Pts',(-18.377826846205,12.8758175756045,124.054817537164)) ;
#80978=CARTESIAN_POINT('Ctrl Pts',(-18.3595260505841,12.8774935606388,124.02447155287)) ;
#80979=CARTESIAN_POINT('Ctrl Pts',(-18.342659499529,12.8791574474389,123.993545530683)) ;
#80980=CARTESIAN_POINT('Ctrl Pts',(-18.3257929484739,12.8808213342391,123.962619508496)) ;
#80981=CARTESIAN_POINT('Ctrl Pts',(-18.3103608501574,12.882473122805,123.931114152062)) ;
#80982=CARTESIAN_POINT('Ctrl Pts',(-18.2964222918482,12.8840981587624,123.899293066508)) ;
#80983=CARTESIAN_POINT('Ctrl Pts',(-18.2884868930003,12.8850233124389,123.881176917043)) ;
#80984=CARTESIAN_POINT('Ctrl Pts',(-18.2809156414011,12.8859571442745,123.862677592541)) ;
#80985=CARTESIAN_POINT('Ctrl Pts',(-18.273826278364,12.88689064817,123.844053819635)) ;
#80986=CARTESIAN_POINT('Ctrl Pts',(-18.2689213497686,12.8875365129574,123.831168561001)) ;
#80987=CARTESIAN_POINT('Ctrl Pts',(-18.2642461152496,12.8881822207643,123.818224229348)) ;
#80988=CARTESIAN_POINT('Ctrl Pts',(-18.259825879779,12.8888247888663,123.80531165987)) ;
#80989=CARTESIAN_POINT('Origin',(-19.4092696390626,-30.19753203383,123.411833654984)) ;
#80990=CARTESIAN_POINT('',(-20.3451307049827,12.4073898409302,124.186586679355)) ;
#80991=CARTESIAN_POINT('Ctrl Pts',(-20.3451203705583,12.4073818757045,124.186578325469)) ;
#80992=CARTESIAN_POINT('Ctrl Pts',(-20.3351949287717,12.4081071627668,124.198567736058)) ;
#80993=CARTESIAN_POINT('Ctrl Pts',(-20.325040088624,12.4088341710223,124.210365203265)) ;
#80994=CARTESIAN_POINT('Ctrl Pts',(-20.3121345010096,12.409742328298,124.224788326587)) ;
#80995=CARTESIAN_POINT('Ctrl Pts',(-20.309594359267,12.4099203334478,124.227600567204)) ;
#80996=CARTESIAN_POINT('Ctrl Pts',(-20.3050370056896,12.4102384080975,124.232598888577)) ;
#80997=CARTESIAN_POINT('Ctrl Pts',(-20.3030248429629,12.4103784012063,124.234789534253)) ;
#80998=CARTESIAN_POINT('Ctrl Pts',(-20.2989274424902,12.4106625874831,124.23921763062)) ;
#80999=CARTESIAN_POINT('Ctrl Pts',(-20.2968417606344,12.4108067866048,124.241454640298)) ;
#81000=CARTESIAN_POINT('Ctrl Pts',(-20.2923176801424,12.4111185917832,124.246270380385)) ;
#81001=CARTESIAN_POINT('Ctrl Pts',(-20.2898763860514,12.4112862410792,124.248846348195)) ;
#81002=CARTESIAN_POINT('Ctrl Pts',(-20.2831348621503,12.4117475412132,124.255897626483)) ;
#81003=CARTESIAN_POINT('Ctrl Pts',(-20.2788115848992,12.4120415369396,124.260350726086)) ;
#81004=CARTESIAN_POINT('Ctrl Pts',(-20.2545481983232,12.4136813136958,124.284962527665)) ;
#81005=CARTESIAN_POINT('Ctrl Pts',(-20.2339414290011,12.4150371351338,124.304451306211)) ;
#81006=CARTESIAN_POINT('Ctrl Pts',(-20.2030097990134,12.4170051085396,124.331718628332)) ;
#81007=CARTESIAN_POINT('Ctrl Pts',(-20.1932126374959,12.4176189969046,124.340082104741)) ;
#81008=CARTESIAN_POINT('Ctrl Pts',(-20.1763776108473,12.4186569494554,124.353996881931)) ;
#81009=CARTESIAN_POINT('Ctrl Pts',(-20.1694079668242,12.4190819065003,124.359628944506)) ;
#81010=CARTESIAN_POINT('Ctrl Pts',(-20.1621103054176,12.4195219507914,124.365393795902)) ;
#81011=CARTESIAN_POINT('Ctrl Pts',(-20.1618439056668,12.4195380078138,124.365604059489)) ;
#81012=CARTESIAN_POINT('Ctrl Pts',(-20.1613584098179,12.4195672584535,124.36598692086)) ;
#81013=CARTESIAN_POINT('Ctrl Pts',(-20.1611393423655,12.4195804525209,124.366159554839)) ;
#81014=CARTESIAN_POINT('Ctrl Pts',(-20.1607358942941,12.4196047431953,124.366477263027)) ;
#81015=CARTESIAN_POINT('Ctrl Pts',(-20.1605515310391,12.4196158400796,124.366622359314)) ;
#81016=CARTESIAN_POINT('Ctrl Pts',(-20.1602085934314,12.4196364756577,124.36689209486)) ;
#81017=CARTESIAN_POINT('Ctrl Pts',(-20.1600500300406,12.4196460145262,124.367016748055)) ;
#81018=CARTESIAN_POINT('Ctrl Pts',(-20.1597522707092,12.4196639227199,124.367250708948)) ;
#81019=CARTESIAN_POINT('Ctrl Pts',(-20.1596130819206,12.4196722921582,124.367360025719)) ;
#81020=CARTESIAN_POINT('Ctrl Pts',(-20.1593493191757,12.4196881487995,124.36756708782)) ;
#81021=CARTESIAN_POINT('Ctrl Pts',(-20.1592247498602,12.4196956360863,124.367664839319)) ;
#81022=CARTESIAN_POINT('Ctrl Pts',(-20.1589866086921,12.419709946874,124.367851637222)) ;
#81023=CARTESIAN_POINT('Ctrl Pts',(-20.1588730401842,12.4197167704202,124.367940687664)) ;
#81024=CARTESIAN_POINT('Ctrl Pts',(-20.158654058468,12.4197299251898,124.368112330879)) ;
#81025=CARTESIAN_POINT('Ctrl Pts',(-20.1585486475016,12.4197362564463,124.368194926435)) ;
#81026=CARTESIAN_POINT('Ctrl Pts',(-20.1583436622498,12.4197485663735,124.368355489479)) ;
#81027=CARTESIAN_POINT('Ctrl Pts',(-20.1582440894389,12.4197545450679,124.368433458853)) ;
#81028=CARTESIAN_POINT('Ctrl Pts',(-20.1580488011973,12.4197662690306,124.368586327941)) ;
#81029=CARTESIAN_POINT('Ctrl Pts',(-20.1579530866292,12.4197720143179,124.368661228895)) ;
#81030=CARTESIAN_POINT('Ctrl Pts',(-20.1577637300843,12.4197833787939,124.368809363099)) ;
#81031=CARTESIAN_POINT('Ctrl Pts',(-20.1576700887087,12.4197889979836,124.368882596881)) ;
#81032=CARTESIAN_POINT('Ctrl Pts',(-20.1574831628118,12.4198002133178,124.369028741151)) ;
#81033=CARTESIAN_POINT('Ctrl Pts',(-20.1573898782531,12.4198058094711,124.369101651847)) ;
#81034=CARTESIAN_POINT('Ctrl Pts',(-20.1547454393545,12.4199644267504,124.371167908036)) ;
#81035=CARTESIAN_POINT('Ctrl Pts',(-20.1521863335445,12.4201173195669,124.373151065124)) ;
#81036=CARTESIAN_POINT('Ctrl Pts',(-20.1469941620041,12.4204263136892,124.377141578164)) ;
#81037=CARTESIAN_POINT('Ctrl Pts',(-20.1443607566838,12.420582407861,124.379148447169)) ;
#81038=CARTESIAN_POINT('Ctrl Pts',(-20.1381947792298,12.4209464638494,124.383807702979)) ;
#81039=CARTESIAN_POINT('Ctrl Pts',(-20.1346558769511,12.4211543225996,124.386451639636)) ;
#81040=CARTESIAN_POINT('Ctrl Pts',(-20.1233518355119,12.4218149192927,124.394801286129)) ;
#81041=CARTESIAN_POINT('Ctrl Pts',(-20.11553318429,12.422266828683,124.400433955071)) ;
#81042=CARTESIAN_POINT('Ctrl Pts',(-20.0913038663772,12.4236534400491,124.417454947616)) ;
#81043=CARTESIAN_POINT('Ctrl Pts',(-20.0746788275006,12.4245854632615,124.428531977815)) ;
#81044=CARTESIAN_POINT('Ctrl Pts',(-20.0478927348905,12.4260679981706,124.445440629808)) ;
#81045=CARTESIAN_POINT('Ctrl Pts',(-20.0379075500964,12.426616925415,124.451543811609)) ;
#81046=CARTESIAN_POINT('Ctrl Pts',(-20.0221992236386,12.4274748179944,124.460836090356)) ;
#81047=CARTESIAN_POINT('Ctrl Pts',(-20.0165357731909,12.4277829769006,124.464124787248)) ;
#81048=CARTESIAN_POINT('Ctrl Pts',(-20.0042389782745,12.4284495607202,124.471133052563)) ;
#81049=CARTESIAN_POINT('Ctrl Pts',(-19.9975967374022,12.4288080654643,124.474836455182)) ;
#81050=CARTESIAN_POINT('Ctrl Pts',(-19.9898368802709,12.4292250499094,124.4790679765)) ;
#81051=CARTESIAN_POINT('Ctrl Pts',(-19.9887526831407,12.4292832689228,124.479657058085)) ;
#81052=CARTESIAN_POINT('Ctrl Pts',(-19.9862073380042,12.429419850731,124.481035013427)) ;
#81053=CARTESIAN_POINT('Ctrl Pts',(-19.9847454665762,12.4294982186086,124.481822545253)) ;
#81054=CARTESIAN_POINT('Ctrl Pts',(-19.9811436218778,12.4296911198525,124.483753395688)) ;
#81055=CARTESIAN_POINT('Ctrl Pts',(-19.9790018298922,12.4298056648805,124.484893305448)) ;
#81056=CARTESIAN_POINT('Ctrl Pts',(-19.9742495803081,12.4300594602298,124.487404320452)) ;
#81057=CARTESIAN_POINT('Ctrl Pts',(-19.9716375168863,12.4301987190576,124.488772353519)) ;
#81058=CARTESIAN_POINT('Ctrl Pts',(-19.948779499333,12.4314152607861,124.500638094162)) ;
#81059=CARTESIAN_POINT('Ctrl Pts',(-19.9282466598147,12.4324936651641,124.510573318427)) ;
#81060=CARTESIAN_POINT('Ctrl Pts',(-19.8975368281539,12.4340841684697,124.524379876922)) ;
#81061=CARTESIAN_POINT('Ctrl Pts',(-19.8875679291923,12.434597071333,124.528701906152)) ;
#81062=CARTESIAN_POINT('Ctrl Pts',(-19.8701781872394,12.435485743556,124.535965720148)) ;
#81063=CARTESIAN_POINT('Ctrl Pts',(-19.8627838517513,12.4358617211218,124.538969161112)) ;
#81064=CARTESIAN_POINT('Ctrl Pts',(-19.8429676240375,12.4368644695173,124.546791569487)) ;
#81065=CARTESIAN_POINT('Ctrl Pts',(-19.8304951579678,12.4374907082586,124.551479421536)) ;
#81066=CARTESIAN_POINT('Ctrl Pts',(-19.8043563752147,12.4387953648757,124.56081610576)) ;
#81067=CARTESIAN_POINT('Ctrl Pts',(-19.7906792355348,12.4394736846942,124.565428436577)) ;
#81068=CARTESIAN_POINT('Ctrl Pts',(-19.7673082292067,12.4406274616318,124.572848741369)) ;
#81069=CARTESIAN_POINT('Ctrl Pts',(-19.7576556409935,12.4411024651437,124.575781615882)) ;
#81070=CARTESIAN_POINT('Ctrl Pts',(-19.7407866454728,12.4419305084295,124.58067850486)) ;
#81071=CARTESIAN_POINT('Ctrl Pts',(-19.7335865458731,12.4422832824306,124.582696734997)) ;
#81072=CARTESIAN_POINT('Ctrl Pts',(-19.7180098829887,12.4430452937906,124.58690826025)) ;
#81073=CARTESIAN_POINT('Ctrl Pts',(-19.7096275800231,12.4434546271339,124.589078732567)) ;
#81074=CARTESIAN_POINT('Ctrl Pts',(-19.6746699160501,12.4451592349017,124.597732830853)) ;
#81075=CARTESIAN_POINT('Ctrl Pts',(-19.6479027753465,12.446460475465,124.603407554339)) ;
#81076=CARTESIAN_POINT('Ctrl Pts',(-19.6110658098122,12.4482383263109,124.609926018679)) ;
#81077=CARTESIAN_POINT('Ctrl Pts',(-19.6011428731397,12.448715775322,124.611555151746)) ;
#81078=CARTESIAN_POINT('Ctrl Pts',(-19.5837658892678,12.4495488284594,124.614186972862)) ;
#81079=CARTESIAN_POINT('Ctrl Pts',(-19.5763206380909,12.4499047838548,124.615243978531)) ;
#81080=CARTESIAN_POINT('Ctrl Pts',(-19.5647395600847,12.4504569044709,124.616778602469)) ;
#81081=CARTESIAN_POINT('Ctrl Pts',(-19.560610302201,12.4506534566962,124.61730419657)) ;
#81082=CARTESIAN_POINT('Ctrl Pts',(-19.552615905046,12.4510333989522,124.618280042272)) ;
#81083=CARTESIAN_POINT('Ctrl Pts',(-19.5487511443468,12.4512168095026,124.6187329661)) ;
#81084=CARTESIAN_POINT('Ctrl Pts',(-19.5397504720133,12.4516433525712,124.619743973136)) ;
#81085=CARTESIAN_POINT('Ctrl Pts',(-19.5346130399005,12.4518863590588,124.620287881093)) ;
#81086=CARTESIAN_POINT('Ctrl Pts',(-19.5177162133305,12.4526841952608,124.621967865714)) ;
#81087=CARTESIAN_POINT('Ctrl Pts',(-19.505943680787,12.4532378123697,124.622965191915)) ;
#81088=CARTESIAN_POINT('Ctrl Pts',(-19.467090319242,12.4550596706197,124.625686587222)) ;
#81089=CARTESIAN_POINT('Ctrl Pts',(-19.4399663337638,12.4563231749537,124.626675162395)) ;
#81090=CARTESIAN_POINT('Ctrl Pts',(-19.4032873085652,12.4580383616142,124.626782711314)) ;
#81091=CARTESIAN_POINT('Ctrl Pts',(-19.3937426677449,12.4584852406688,124.626698219334)) ;
#81092=CARTESIAN_POINT('Ctrl Pts',(-19.3786396096712,12.4591938194038,124.62638650644)) ;
#81093=CARTESIAN_POINT('Ctrl Pts',(-19.3730800437493,12.4594549633874,124.62623356464)) ;
#81094=CARTESIAN_POINT('Ctrl Pts',(-19.3626132242422,12.4599472966608,124.625873686047)) ;
#81095=CARTESIAN_POINT('Ctrl Pts',(-19.3577057920009,12.4601784139758,124.625675155148)) ;
#81096=CARTESIAN_POINT('Ctrl Pts',(-19.3499109047112,12.460546013042,124.625312455789)) ;
#81097=CARTESIAN_POINT('Ctrl Pts',(-19.3470225932408,12.4606823310212,124.625167724639)) ;
#81098=CARTESIAN_POINT('Ctrl Pts',(-19.3402806110107,12.4610007912081,124.624805751909)) ;
#81099=CARTESIAN_POINT('Ctrl Pts',(-19.3364274075621,12.4611829994012,124.62458045589)) ;
#81100=CARTESIAN_POINT('Ctrl Pts',(-19.3272924955378,12.4616154601858,124.624002646601)) ;
#81101=CARTESIAN_POINT('Ctrl Pts',(-19.3220118953407,12.4618658442989,124.623633969465)) ;
#81102=CARTESIAN_POINT('Ctrl Pts',(-19.3010691538164,12.4628604591191,124.622034203137)) ;
#81103=CARTESIAN_POINT('Ctrl Pts',(-19.2854292205939,12.4636068434062,124.620533889162)) ;
#81104=CARTESIAN_POINT('Ctrl Pts',(-19.2621492949723,12.4647227455979,124.617844090457)) ;
#81105=CARTESIAN_POINT('Ctrl Pts',(-19.2544843531212,12.4650909426616,124.616884309909)) ;
#81106=CARTESIAN_POINT('Ctrl Pts',(-19.2284568809309,12.46634349718,124.613372803311)) ;
#81107=CARTESIAN_POINT('Ctrl Pts',(-19.2101437085806,12.467228586291,124.610473904923)) ;
#81108=CARTESIAN_POINT('Ctrl Pts',(-19.1814321557965,12.4686167418677,124.605252802963)) ;
#81109=CARTESIAN_POINT('Ctrl Pts',(-19.1709857538774,12.4691219684945,124.603210998307)) ;
#81110=CARTESIAN_POINT('Ctrl Pts',(-19.1566241463862,12.469816499792,124.600207493878)) ;
#81111=CARTESIAN_POINT('Ctrl Pts',(-19.1526849468642,12.4700069988917,124.599363200647)) ;
#81112=CARTESIAN_POINT('Ctrl Pts',(-19.1455266584401,12.470353173029,124.597791675751)) ;
#81113=CARTESIAN_POINT('Ctrl Pts',(-19.1423061980073,12.4705089144514,124.597070892028)) ;
#81114=CARTESIAN_POINT('Ctrl Pts',(-19.1359887750859,12.4708144342264,124.595629910688)) ;
#81115=CARTESIAN_POINT('Ctrl Pts',(-19.1328916247853,12.4709642213392,124.594910659636)) ;
#81116=CARTESIAN_POINT('Ctrl Pts',(-19.1297777194605,12.4711148299593,124.594174622459)) ;
#81117=CARTESIAN_POINT('Ctrl Pts',(-19.1297581115696,12.4711157783243,124.594169987205)) ;
#81118=CARTESIAN_POINT('Ctrl Pts',(-19.1297187849672,12.4711176804152,124.594160689468)) ;
#81119=CARTESIAN_POINT('Ctrl Pts',(-19.1296990663627,12.471118634136,124.594156027003)) ;
#81120=CARTESIAN_POINT('Ctrl Pts',(-19.1296595142969,12.4711205471336,124.594146673871)) ;
#81121=CARTESIAN_POINT('Ctrl Pts',(-19.1296396812692,12.4711215063896,124.5941419833)) ;
#81122=CARTESIAN_POINT('Ctrl Pts',(-19.1295998966232,12.4711234306382,124.594132573054)) ;
#81123=CARTESIAN_POINT('Ctrl Pts',(-19.1295799451038,12.4711243956262,124.594127853396)) ;
#81124=CARTESIAN_POINT('Ctrl Pts',(-19.1295399194418,12.4711263315339,124.594118384003)) ;
#81125=CARTESIAN_POINT('Ctrl Pts',(-19.1295198457925,12.4711273024298,124.594113634378)) ;
#81126=CARTESIAN_POINT('Ctrl Pts',(-19.1294795723347,12.4711292503245,124.594104104195)) ;
#81127=CARTESIAN_POINT('Ctrl Pts',(-19.1294593721875,12.4711302273397,124.594099323549)) ;
#81128=CARTESIAN_POINT('Ctrl Pts',(-19.1294188413759,12.4711321876837,124.594089730272)) ;
#81129=CARTESIAN_POINT('Ctrl Pts',(-19.1293985113244,12.471133170983,124.594084917779)) ;
#81130=CARTESIAN_POINT('Ctrl Pts',(-19.1293577174786,12.4711351440512,124.594075260022)) ;
#81131=CARTESIAN_POINT('Ctrl Pts',(-19.1293372525617,12.4711361338745,124.594070414485)) ;
#81132=CARTESIAN_POINT('Ctrl Pts',(-19.1292961847695,12.4711381201946,124.59406068962)) ;
#81133=CARTESIAN_POINT('Ctrl Pts',(-19.1292755817868,12.4711391166967,124.594055810259)) ;
#81134=CARTESIAN_POINT('Ctrl Pts',(-19.1292342324706,12.4711411166354,124.594046016447)) ;
#81135=CARTESIAN_POINT('Ctrl Pts',(-19.1292134873069,12.4711421200155,124.594041102264)) ;
#81136=CARTESIAN_POINT('Ctrl Pts',(-19.1291718507328,12.4711441338501,124.594031238097)) ;
#81137=CARTESIAN_POINT('Ctrl Pts',(-19.1291509578169,12.4711451443775,124.594026287749)) ;
#81138=CARTESIAN_POINT('Ctrl Pts',(-19.1291090203986,12.4711471727652,124.594016349961)) ;
#81139=CARTESIAN_POINT('Ctrl Pts',(-19.1290879772574,12.4711481905597,124.594011362836)) ;
#81140=CARTESIAN_POINT('Ctrl Pts',(-19.1290457353088,12.4711502336789,124.594001350502)) ;
#81141=CARTESIAN_POINT('Ctrl Pts',(-19.1290245359253,12.4711512590314,124.593996325147)) ;
#81142=CARTESIAN_POINT('Ctrl Pts',(-19.1289819772032,12.4711533174743,124.593986235312)) ;
#81143=CARTESIAN_POINT('Ctrl Pts',(-19.1289606179962,12.4711543505582,124.593981170853)) ;
#81144=CARTESIAN_POINT('Ctrl Pts',(-19.1289177351044,12.4711564246825,124.593971001709)) ;
#81145=CARTESIAN_POINT('Ctrl Pts',(-19.1288962111384,12.4711574657365,124.593965896947)) ;
#81146=CARTESIAN_POINT('Ctrl Pts',(-19.1288529937298,12.4711595560428,124.593955645983)) ;
#81147=CARTESIAN_POINT('Ctrl Pts',(-19.1288313007526,12.4711606052726,124.593950499881)) ;
#81148=CARTESIAN_POINT('Ctrl Pts',(-19.1287877406476,12.4711627121565,124.593940165097)) ;
#81149=CARTESIAN_POINT('Ctrl Pts',(-19.1287658735658,12.4711637698085,124.593934976417)) ;
#81150=CARTESIAN_POINT('Ctrl Pts',(-19.1287219607313,12.4711658937555,124.593924555373)) ;
#81151=CARTESIAN_POINT('Ctrl Pts',(-19.1286999147798,12.4711669600602,124.593919322952)) ;
#81152=CARTESIAN_POINT('Ctrl Pts',(-19.1286556388924,12.4711691015696,124.593908813134)) ;
#81153=CARTESIAN_POINT('Ctrl Pts',(-19.1286334095222,12.471170176747,124.593903535861)) ;
#81154=CARTESIAN_POINT('Ctrl Pts',(-19.1285887619197,12.4711723362378,124.593892935148)) ;
#81155=CARTESIAN_POINT('Ctrl Pts',(-19.1285663436896,12.4711734205512,124.593887611698)) ;
#81156=CARTESIAN_POINT('Ctrl Pts',(-19.1285213143905,12.4711755985064,124.593876917652)) ;
#81157=CARTESIAN_POINT('Ctrl Pts',(-19.1284987019365,12.4711766922152,124.593871546716)) ;
#81158=CARTESIAN_POINT('Ctrl Pts',(-19.1284532782461,12.4711788892488,124.593860756253)) ;
#81159=CARTESIAN_POINT('Ctrl Pts',(-19.1284304674776,12.471179992551,124.593855336824)) ;
#81160=CARTESIAN_POINT('Ctrl Pts',(-19.1283846411428,12.4711822090622,124.593844447908)) ;
#81161=CARTESIAN_POINT('Ctrl Pts',(-19.1283616261888,12.4711833222417,124.593838978554)) ;
#81162=CARTESIAN_POINT('Ctrl Pts',(-19.1283153861599,12.4711855587652,124.593827988486)) ;
#81163=CARTESIAN_POINT('Ctrl Pts',(-19.1282921615205,12.4711866820881,124.593822467862)) ;
#81164=CARTESIAN_POINT('Ctrl Pts',(-19.1282454979295,12.4711889391012,124.593811374218)) ;
#81165=CARTESIAN_POINT('Ctrl Pts',(-19.1282220575147,12.4711900728621,124.593805800837)) ;
#81166=CARTESIAN_POINT('Ctrl Pts',(-19.1281749565108,12.4711923510348,124.593794600243)) ;
#81167=CARTESIAN_POINT('Ctrl Pts',(-19.1281512957772,12.4711934954536,124.593788972983)) ;
#81168=CARTESIAN_POINT('Ctrl Pts',(-19.1281037476936,12.4711957952535,124.593777663057)) ;
#81169=CARTESIAN_POINT('Ctrl Pts',(-19.1280798606057,12.4711969506221,124.593771980439)) ;
#81170=CARTESIAN_POINT('Ctrl Pts',(-19.1280318538365,12.4711992726108,124.593760558334)) ;
#81171=CARTESIAN_POINT('Ctrl Pts',(-19.1280077343803,12.4712004392201,124.593754818884)) ;
#81172=CARTESIAN_POINT('Ctrl Pts',(-19.1279592570408,12.4712027839724,124.593743281681)) ;
#81173=CARTESIAN_POINT('Ctrl Pts',(-19.1279348991688,12.471203962115,124.593737483915)) ;
#81174=CARTESIAN_POINT('Ctrl Pts',(-19.1278859382947,12.4712063302582,124.593725828436)) ;
#81175=CARTESIAN_POINT('Ctrl Pts',(-19.127861336301,12.4712075202101,124.593719970948)) ;
#81176=CARTESIAN_POINT('Ctrl Pts',(-19.1278118816013,12.4712099122421,124.593708194647)) ;
#81177=CARTESIAN_POINT('Ctrl Pts',(-19.127787028385,12.4712111143468,124.593702275696)) ;
#81178=CARTESIAN_POINT('Ctrl Pts',(-19.1277370647114,12.4712135310003,124.593690374866)) ;
#81179=CARTESIAN_POINT('Ctrl Pts',(-19.1277119547266,12.4712147455262,124.593684393082)) ;
#81180=CARTESIAN_POINT('Ctrl Pts',(-19.1276614715568,12.4712171873103,124.593672365113)) ;
#81181=CARTESIAN_POINT('Ctrl Pts',(-19.1276360974865,12.4712184146113,124.5936663187)) ;
#81182=CARTESIAN_POINT('Ctrl Pts',(-19.12758507883,12.4712208822996,124.593654159675)) ;
#81183=CARTESIAN_POINT('Ctrl Pts',(-19.1275594350107,12.4712221226497,124.593648047227)) ;
#81184=CARTESIAN_POINT('Ctrl Pts',(-19.1275078705696,12.4712246167403,124.593635754581)) ;
#81185=CARTESIAN_POINT('Ctrl Pts',(-19.1274819490489,12.4712258705243,124.593629574148)) ;
#81186=CARTESIAN_POINT('Ctrl Pts',(-19.127429821882,12.4712283918369,124.593617143726)) ;
#81187=CARTESIAN_POINT('Ctrl Pts',(-19.127403616693,12.4712296593434,124.593610893826)) ;
#81188=CARTESIAN_POINT('Ctrl Pts',(-19.1273509150534,12.4712322084463,124.593598322708)) ;
#81189=CARTESIAN_POINT('Ctrl Pts',(-19.1273244183494,12.4712334900549,124.593592001409)) ;
#81190=CARTESIAN_POINT('Ctrl Pts',(-19.127271125791,12.4712360677437,124.593579285548)) ;
#81191=CARTESIAN_POINT('Ctrl Pts',(-19.1272443309084,12.4712373637769,124.593572891197)) ;
#81192=CARTESIAN_POINT('Ctrl Pts',(-19.1271904355227,12.4712399706277,124.593560027624)) ;
#81193=CARTESIAN_POINT('Ctrl Pts',(-19.1271633338253,12.4712412815032,124.593553558094)) ;
#81194=CARTESIAN_POINT('Ctrl Pts',(-19.1271088168654,12.471243918423,124.593540542201)) ;
#81195=CARTESIAN_POINT('Ctrl Pts',(-19.1270814019424,12.471245244451,124.593533995896)) ;
#81196=CARTESIAN_POINT('Ctrl Pts',(-19.1270262503819,12.47124791207,124.593520824435)) ;
#81197=CARTESIAN_POINT('Ctrl Pts',(-19.1269985137445,12.4712492536611,124.593514199256)) ;
#81198=CARTESIAN_POINT('Ctrl Pts',(-19.1269427109486,12.4712519527842,124.593500868111)) ;
#81199=CARTESIAN_POINT('Ctrl Pts',(-19.1269146446208,12.4712533103244,124.593494162081)) ;
#81200=CARTESIAN_POINT('Ctrl Pts',(-19.1232261266058,12.4714317203986,124.59261270678)) ;
#81201=CARTESIAN_POINT('Ctrl Pts',(-19.1195697518813,12.4716085949165,124.591720952851)) ;
#81202=CARTESIAN_POINT('Ctrl Pts',(-19.1103423316582,12.4720550570206,124.589424996946)) ;
#81203=CARTESIAN_POINT('Ctrl Pts',(-19.1047769876549,12.4723244160121,124.587998239301)) ;
#81204=CARTESIAN_POINT('Ctrl Pts',(-19.0879711285919,12.4731383198285,124.58356253251)) ;
#81205=CARTESIAN_POINT('Ctrl Pts',(-19.0767635106322,12.4736817661215,124.580431520676)) ;
#81206=CARTESIAN_POINT('Ctrl Pts',(-19.0368958163013,12.4756210993441,124.568673913459)) ;
#81207=CARTESIAN_POINT('Ctrl Pts',(-19.0085119642555,12.4770157746918,124.559150060454)) ;
#81208=CARTESIAN_POINT('Ctrl Pts',(-18.9746763427525,12.4787134502845,124.546387936201)) ;
#81209=CARTESIAN_POINT('Ctrl Pts',(-18.9688611373116,12.4790064217359,124.5441432864)) ;
#81210=CARTESIAN_POINT('Ctrl Pts',(-18.9588898776629,12.4795109142169,124.540205978949)) ;
#81211=CARTESIAN_POINT('Ctrl Pts',(-18.9547254475909,12.4797222578357,124.538534861522)) ;
#81212=CARTESIAN_POINT('Ctrl Pts',(-18.9478449624896,12.4800725258619,124.535729480526)) ;
#81213=CARTESIAN_POINT('Ctrl Pts',(-18.9451235967112,12.4802113462035,124.534608347498)) ;
#81214=CARTESIAN_POINT('Ctrl Pts',(-18.9422116026113,12.4803601949877,124.533396284159)) ;
#81215=CARTESIAN_POINT('Ctrl Pts',(-18.9420168913035,12.4803701492635,124.533315179704)) ;
#81216=CARTESIAN_POINT('Ctrl Pts',(-18.9416692924694,12.4803879222542,124.533170285704)) ;
#81217=CARTESIAN_POINT('Ctrl Pts',(-18.9415163966919,12.4803957408314,124.533106515523)) ;
#81218=CARTESIAN_POINT('Ctrl Pts',(-18.9365214095347,12.4806511971551,124.531021993401)) ;
#81219=CARTESIAN_POINT('Ctrl Pts',(-18.9316924566339,12.4808990667659,124.52896993135)) ;
#81220=CARTESIAN_POINT('Ctrl Pts',(-18.9209181544401,12.4814541312749,124.524308767695)) ;
#81221=CARTESIAN_POINT('Ctrl Pts',(-18.9149801246699,12.4817614309349,124.52168316034)) ;
#81222=CARTESIAN_POINT('Ctrl Pts',(-18.8979819526725,12.482645017007,124.514003633592)) ;
#81223=CARTESIAN_POINT('Ctrl Pts',(-18.886976281193,12.4832219170089,124.508831105724)) ;
#81224=CARTESIAN_POINT('Ctrl Pts',(-18.8555607774336,12.4848813326728,124.493486263975)) ;
#81225=CARTESIAN_POINT('Ctrl Pts',(-18.8353570774093,12.4859634097558,124.482903333363)) ;
#81226=CARTESIAN_POINT('Ctrl Pts',(-18.8076378391511,12.4874660048555,124.467374050866)) ;
#81227=CARTESIAN_POINT('Ctrl Pts',(-18.7998613557678,12.4878897221409,124.462903536099)) ;
#81228=CARTESIAN_POINT('Ctrl Pts',(-18.7917291756995,12.4883352844162,124.458107947052)) ;
#81229=CARTESIAN_POINT('Ctrl Pts',(-18.7913234166414,12.4883575224754,124.45786835055)) ;
#81230=CARTESIAN_POINT('Ctrl Pts',(-18.782935937589,12.4888173425152,124.452909048009)) ;
#81231=CARTESIAN_POINT('Ctrl Pts',(-18.7750083563902,12.4892544799009,124.448098343911)) ;
#81232=CARTESIAN_POINT('Ctrl Pts',(-18.750443398737,12.4906176759226,124.432804058551)) ;
#81233=CARTESIAN_POINT('Ctrl Pts',(-18.7340049644258,12.4915423969222,124.422007006939)) ;
#81234=CARTESIAN_POINT('Ctrl Pts',(-18.7064803172295,12.4931172500784,124.402956142816)) ;
#81235=CARTESIAN_POINT('Ctrl Pts',(-18.6952596669294,12.4937670770598,124.394903527791)) ;
#81236=CARTESIAN_POINT('Ctrl Pts',(-18.6837845615061,12.4944411533968,124.386368179618)) ;
#81237=CARTESIAN_POINT('Ctrl Pts',(-18.6833905324445,12.4944643114425,124.386074723732)) ;
#81238=CARTESIAN_POINT('Ctrl Pts',(-18.6826028318842,12.4945106302433,124.385487335101)) ;
#81239=CARTESIAN_POINT('Ctrl Pts',(-18.6822091605129,12.494533790991,124.385193402452)) ;
#81240=CARTESIAN_POINT('Ctrl Pts',(-18.6813842104247,12.4945823500495,124.384576678119)) ;
#81241=CARTESIAN_POINT('Ctrl Pts',(-18.6809529678954,12.4946077486456,124.384253838228)) ;
#81242=CARTESIAN_POINT('Ctrl Pts',(-18.6799932412372,12.4946643051737,124.383534364191)) ;
#81243=CARTESIAN_POINT('Ctrl Pts',(-18.6794648657086,12.4946954639981,124.383137585527)) ;
#81244=CARTESIAN_POINT('Ctrl Pts',(-18.6779865849993,12.4947827010053,124.382025597215)) ;
#81245=CARTESIAN_POINT('Ctrl Pts',(-18.677037405952,12.4948387854086,124.381309424007)) ;
#81246=CARTESIAN_POINT('Ctrl Pts',(-18.6722650589083,12.4951211326779,124.377697592794)) ;
#81247=CARTESIAN_POINT('Ctrl Pts',(-18.6684580193074,12.4953475423961,124.374780715562)) ;
#81248=CARTESIAN_POINT('Ctrl Pts',(-18.6604677729949,12.4958253390172,124.368583319832)) ;
#81249=CARTESIAN_POINT('Ctrl Pts',(-18.6562886328926,12.4960767535579,124.365297739247)) ;
#81250=CARTESIAN_POINT('Ctrl Pts',(-18.6426423991322,12.4969024371642,124.354423587546)) ;
#81251=CARTESIAN_POINT('Ctrl Pts',(-18.6332674052875,12.4974772121036,124.346720620794)) ;
#81252=CARTESIAN_POINT('Ctrl Pts',(-18.6128213228358,12.4987461124564,124.329401614334)) ;
#81253=CARTESIAN_POINT('Ctrl Pts',(-18.6018057200431,12.4994400176587,124.319722911731)) ;
#81254=CARTESIAN_POINT('Ctrl Pts',(-18.5857958141577,12.5004632501538,124.305134119495)) ;
#81255=CARTESIAN_POINT('Ctrl Pts',(-18.5806644593845,12.500793525911,124.300376460262)) ;
#81256=CARTESIAN_POINT('Ctrl Pts',(-18.5713587859075,12.5013967716912,124.29159776347)) ;
#81257=CARTESIAN_POINT('Ctrl Pts',(-18.5671715935793,12.5016698335591,124.287590679762)) ;
#81258=CARTESIAN_POINT('Ctrl Pts',(-18.5618209024629,12.5020209113366,124.28239628705)) ;
#81259=CARTESIAN_POINT('Ctrl Pts',(-18.5606309545955,12.5020991258231,124.28123634692)) ;
#81260=CARTESIAN_POINT('Ctrl Pts',(-18.5543858940395,12.5025103405062,124.275123734655)) ;
#81261=CARTESIAN_POINT('Ctrl Pts',(-18.5493717386309,12.5028430273277,124.270129396785)) ;
#81262=CARTESIAN_POINT('Ctrl Pts',(-18.5284640589082,12.5042413584933,124.248937226405)) ;
#81263=CARTESIAN_POINT('Ctrl Pts',(-18.5129823544157,12.5053039620752,124.232339575367)) ;
#81264=CARTESIAN_POINT('Ctrl Pts',(-18.4863040867395,12.5071951944769,124.202081646359)) ;
#81265=CARTESIAN_POINT('Ctrl Pts',(-18.4749234280842,12.5080231961958,124.18859259609)) ;
#81266=CARTESIAN_POINT('Ctrl Pts',(-18.4589052683812,12.5092228190037,124.168745283165)) ;
#81267=CARTESIAN_POINT('Ctrl Pts',(-18.4540293329917,12.5095927906,124.162582352647)) ;
#81268=CARTESIAN_POINT('Ctrl Pts',(-18.4451010183587,12.5102794371518,124.151069612642)) ;
#81269=CARTESIAN_POINT('Ctrl Pts',(-18.4410325098955,12.5105959926255,124.145732688638)) ;
#81270=CARTESIAN_POINT('Ctrl Pts',(-18.4319243444403,12.5113131107076,124.133577345849)) ;
#81271=CARTESIAN_POINT('Ctrl Pts',(-18.4269114297649,12.5117138190335,124.12673933283)) ;
#81272=CARTESIAN_POINT('Ctrl Pts',(-18.4154053814133,12.5126478019861,124.110694617467)) ;
#81273=CARTESIAN_POINT('Ctrl Pts',(-18.4089679150352,12.5131813155171,124.101448958921)) ;
#81274=CARTESIAN_POINT('Ctrl Pts',(-18.3872211798402,12.5150216325441,124.069270405564)) ;
#81275=CARTESIAN_POINT('Ctrl Pts',(-18.3725644548256,12.5163287249421,124.045906607494)) ;
#81276=CARTESIAN_POINT('Ctrl Pts',(-18.3540578587316,12.5180699633502,124.014046222899)) ;
#81277=CARTESIAN_POINT('Ctrl Pts',(-18.3494923448433,12.5185077432531,124.005975023411)) ;
#81278=CARTESIAN_POINT('Ctrl Pts',(-18.3402562835985,12.5194109507599,123.989201704953)) ;
#81279=CARTESIAN_POINT('Ctrl Pts',(-18.3355985429631,12.5198762912002,123.980493304886)) ;
#81280=CARTESIAN_POINT('Ctrl Pts',(-18.3255776593783,12.5209001906639,123.961195524633)) ;
#81281=CARTESIAN_POINT('Ctrl Pts',(-18.320262483917,12.5214585425504,123.950582378729)) ;
#81282=CARTESIAN_POINT('Ctrl Pts',(-18.3071838860961,12.5228738705007,123.923482857499)) ;
#81283=CARTESIAN_POINT('Ctrl Pts',(-18.2996343075352,12.5237305022439,123.906896621364)) ;
#81284=CARTESIAN_POINT('Ctrl Pts',(-18.290383698556,12.5248379598755,123.885297464845)) ;
#81285=CARTESIAN_POINT('Ctrl Pts',(-18.2883383557618,12.52508678507,123.880434535276)) ;
#81286=CARTESIAN_POINT('Ctrl Pts',(-18.2846466134175,12.5255434556328,123.871494700197)) ;
#81287=CARTESIAN_POINT('Ctrl Pts',(-18.2829905486527,12.5257512314104,123.867421886359)) ;
#81288=CARTESIAN_POINT('Ctrl Pts',(-18.2736868532533,12.5269351294952,123.844180231193)) ;
#81289=CARTESIAN_POINT('Ctrl Pts',(-18.2665099269775,12.5279132636302,123.824837367136)) ;
#81290=CARTESIAN_POINT('Ctrl Pts',(-18.259825879779,12.5288903030032,123.80531165987)) ;
#81291=CARTESIAN_POINT('',(-20.0599602754258,12.4073831970672,124.437819810756)) ;
#81292=CARTESIAN_POINT('Origin',(-19.4092696390626,12.4073831970673,123.411833654984)) ;
#81293=CARTESIAN_POINT('Ctrl Pts',(-18.259825879779,12.510900730771,123.80531165987)) ;
#81294=CARTESIAN_POINT('Ctrl Pts',(-18.2708779448963,12.5092744369586,123.837597396604)) ;
#81295=CARTESIAN_POINT('Ctrl Pts',(-18.2832817189336,12.5076394659094,123.869394206438)) ;
#81296=CARTESIAN_POINT('Ctrl Pts',(-18.2992643795568,12.5057525469584,123.905762369247)) ;
#81297=CARTESIAN_POINT('Ctrl Pts',(-18.3015526664204,12.5054869325776,123.910873092127)) ;
#81298=CARTESIAN_POINT('Ctrl Pts',(-18.3054234465231,12.5050450941351,123.919360385976)) ;
#81299=CARTESIAN_POINT('Ctrl Pts',(-18.3069862945246,12.5048686558078,123.922745807838)) ;
#81300=CARTESIAN_POINT('Ctrl Pts',(-18.3098741739523,12.5045461653814,123.928926563957)) ;
#81301=CARTESIAN_POINT('Ctrl Pts',(-18.3111943424549,12.5044000593755,123.931724132168)) ;
#81302=CARTESIAN_POINT('Ctrl Pts',(-18.3138334545042,12.5041105663035,123.937261774729)) ;
#81303=CARTESIAN_POINT('Ctrl Pts',(-18.3151520294746,12.5039671761994,123.940001999279)) ;
#81304=CARTESIAN_POINT('Ctrl Pts',(-18.3182412047487,12.5036341061789,123.946360622662)) ;
#81305=CARTESIAN_POINT('Ctrl Pts',(-18.3200195422345,12.5034445157386,123.949975225918)) ;
#81306=CARTESIAN_POINT('Ctrl Pts',(-18.3254992350252,12.5028667432464,123.960974658897)) ;
#81307=CARTESIAN_POINT('Ctrl Pts',(-18.3292579646782,12.5024791994803,123.968330658708)) ;
#81308=CARTESIAN_POINT('Ctrl Pts',(-18.336071983817,12.5017914708978,123.981336893299)) ;
#81309=CARTESIAN_POINT('Ctrl Pts',(-18.3390976015429,12.5014910431626,123.987002287794)) ;
#81310=CARTESIAN_POINT('Ctrl Pts',(-18.3426787219295,12.5011409439048,123.993581755835)) ;
#81311=CARTESIAN_POINT('Ctrl Pts',(-18.3431906737507,12.501091022387,123.994519399683)) ;
#81312=CARTESIAN_POINT('Ctrl Pts',(-18.3538246731278,12.5000567097751,124.013934726689)) ;
#81313=CARTESIAN_POINT('Ctrl Pts',(-18.3644243786652,12.4990749671909,124.032146609859)) ;
#81314=CARTESIAN_POINT('Ctrl Pts',(-18.3834785611712,12.4973778425946,124.063009258256)) ;
#81315=CARTESIAN_POINT('Ctrl Pts',(-18.3917067937197,12.4966650314769,124.075793633516)) ;
#81316=CARTESIAN_POINT('Ctrl Pts',(-18.4037481589575,12.4956488473075,124.093752762712)) ;
#81317=CARTESIAN_POINT('Ctrl Pts',(-18.4073658038323,12.495346838339,124.099056923694)) ;
#81318=CARTESIAN_POINT('Ctrl Pts',(-18.4125732647053,12.4949166911301,124.106563536787)) ;
#81319=CARTESIAN_POINT('Ctrl Pts',(-18.414128691141,12.4947887793874,124.108789726105)) ;
#81320=CARTESIAN_POINT('Ctrl Pts',(-18.4194374626593,12.4943541279479,124.116333851243)) ;
#81321=CARTESIAN_POINT('Ctrl Pts',(-18.4232260690798,12.4940471694145,124.121626823271)) ;
#81322=CARTESIAN_POINT('Ctrl Pts',(-18.4321525980218,12.4933313216252,124.133888459256)) ;
#81323=CARTESIAN_POINT('Ctrl Pts',(-18.4373228367532,12.4929222536337,124.140833150909)) ;
#81324=CARTESIAN_POINT('Ctrl Pts',(-18.4565933846306,12.4914175510375,124.166147987438)) ;
#81325=CARTESIAN_POINT('Ctrl Pts',(-18.4711438126358,12.4903196927723,124.184169128002)) ;
#81326=CARTESIAN_POINT('Ctrl Pts',(-18.49881615561,12.4882995824613,124.21650554077)) ;
#81327=CARTESIAN_POINT('Ctrl Pts',(-18.5117833978879,12.4873779827832,124.230943439137)) ;
#81328=CARTESIAN_POINT('Ctrl Pts',(-18.5286842312663,12.4862096697275,124.248877672681)) ;
#81329=CARTESIAN_POINT('Ctrl Pts',(-18.5323022321512,12.4859613973245,124.252667476463)) ;
#81330=CARTESIAN_POINT('Ctrl Pts',(-18.5419511153411,12.4853041266909,124.262644518653)) ;
#81331=CARTESIAN_POINT('Ctrl Pts',(-18.5480236877417,12.4848954183119,124.268791039838)) ;
#81332=CARTESIAN_POINT('Ctrl Pts',(-18.5574998585772,12.4842651971188,124.278180135829)) ;
#81333=CARTESIAN_POINT('Ctrl Pts',(-18.5608575642792,12.4840433228017,124.281468598696)) ;
#81334=CARTESIAN_POINT('Ctrl Pts',(-18.5682245407831,12.4835596122474,124.288600375835)) ;
#81335=CARTESIAN_POINT('Ctrl Pts',(-18.5722412573361,12.4832978462156,124.292435851528)) ;
#81336=CARTESIAN_POINT('Ctrl Pts',(-18.58171967871,12.4826846806696,124.301363144904)) ;
#81337=CARTESIAN_POINT('Ctrl Pts',(-18.5872023114967,12.4823334807318,124.306432425294)) ;
#81338=CARTESIAN_POINT('Ctrl Pts',(-18.6079289068811,12.4810184089763,124.325244936789)) ;
#81339=CARTESIAN_POINT('Ctrl Pts',(-18.6234736251106,12.480057459793,124.338651744565)) ;
#81340=CARTESIAN_POINT('Ctrl Pts',(-18.6603748226619,12.4778267614658,124.368881780136)) ;
#81341=CARTESIAN_POINT('Ctrl Pts',(-18.6819710535665,12.4765580511313,124.385394811009)) ;
#81342=CARTESIAN_POINT('Ctrl Pts',(-18.7128568840371,12.4747820521826,124.407409235582)) ;
#81343=CARTESIAN_POINT('Ctrl Pts',(-18.7216933348196,12.4742781689636,124.41353235549)) ;
#81344=CARTESIAN_POINT('Ctrl Pts',(-18.7359840832137,12.4734693234892,124.423156767871)) ;
#81345=CARTESIAN_POINT('Ctrl Pts',(-18.7413871662192,12.4731648753908,124.426733098517)) ;
#81346=CARTESIAN_POINT('Ctrl Pts',(-18.7470482306654,12.4728472203578,124.430415403002)) ;
#81347=CARTESIAN_POINT('Ctrl Pts',(-18.7472779247224,12.4728343339784,124.430564699607)) ;
#81348=CARTESIAN_POINT('Ctrl Pts',(-18.7477292637262,12.4728090172404,124.430857843953)) ;
#81349=CARTESIAN_POINT('Ctrl Pts',(-18.7479509051141,12.4727965869237,124.431001697082)) ;
#81350=CARTESIAN_POINT('Ctrl Pts',(-18.7483872392515,12.4727721201238,124.431284691159)) ;
#81351=CARTESIAN_POINT('Ctrl Pts',(-18.7486019290304,12.4727600836758,124.431423836606)) ;
#81352=CARTESIAN_POINT('Ctrl Pts',(-18.7490253876303,12.472736346606,124.431698100083)) ;
#81353=CARTESIAN_POINT('Ctrl Pts',(-18.7492341539641,12.4727246460152,124.431833221816)) ;
#81354=CARTESIAN_POINT('Ctrl Pts',(-18.7496467346263,12.4727015260305,124.432100080445)) ;
#81355=CARTESIAN_POINT('Ctrl Pts',(-18.7498505469923,12.4726901066585,124.432231820405)) ;
#81356=CARTESIAN_POINT('Ctrl Pts',(-18.7502541434033,12.4726674970954,124.432492525083)) ;
#81357=CARTESIAN_POINT('Ctrl Pts',(-18.750453926018,12.4726563069143,124.432621492332)) ;
#81358=CARTESIAN_POINT('Ctrl Pts',(-18.750850355263,12.4726341055428,124.432877237574)) ;
#81359=CARTESIAN_POINT('Ctrl Pts',(-18.7510470005906,12.4726230943717,124.433004017378)) ;
#81360=CARTESIAN_POINT('Ctrl Pts',(-18.7514380283173,12.4726012019729,124.433255958167)) ;
#81361=CARTESIAN_POINT('Ctrl Pts',(-18.7516324098492,12.4725903207555,124.433381120493)) ;
#81362=CARTESIAN_POINT('Ctrl Pts',(-18.75201977778,12.472568639572,124.433630390434)) ;
#81363=CARTESIAN_POINT('Ctrl Pts',(-18.7522127636392,12.4725578396122,124.433754498881)) ;
#81364=CARTESIAN_POINT('Ctrl Pts',(-18.7525982166654,12.4725362718256,124.434002227881)) ;
#81365=CARTESIAN_POINT('Ctrl Pts',(-18.7527906836682,12.4725255039984,124.434125848799)) ;
#81366=CARTESIAN_POINT('Ctrl Pts',(-18.7531760000206,12.4725039500395,124.434373182528)) ;
#81367=CARTESIAN_POINT('Ctrl Pts',(-18.7533688493787,12.4724931639124,124.434496895094)) ;
#81368=CARTESIAN_POINT('Ctrl Pts',(-18.7537558726141,12.4724715206736,124.434745015397)) ;
#81369=CARTESIAN_POINT('Ctrl Pts',(-18.7539500469856,12.4724606635546,124.434869422446)) ;
#81370=CARTESIAN_POINT('Ctrl Pts',(-18.7543407243061,12.472438822253,124.435119571591)) ;
#81371=CARTESIAN_POINT('Ctrl Pts',(-18.754537228102,12.4724278380596,124.435245312406)) ;
#81372=CARTESIAN_POINT('Ctrl Pts',(-18.7549336540121,12.4724056818063,124.435498820478)) ;
#81373=CARTESIAN_POINT('Ctrl Pts',(-18.7551335773291,12.472394509734,124.435626585766)) ;
#81374=CARTESIAN_POINT('Ctrl Pts',(-18.7555380464852,12.4723719105972,124.435884903621)) ;
#81375=CARTESIAN_POINT('Ctrl Pts',(-18.7557425941155,12.4723604835081,124.436015453539)) ;
#81376=CARTESIAN_POINT('Ctrl Pts',(-18.7560159732782,12.4723452134236,124.436189819061)) ;
#81377=CARTESIAN_POINT('Ctrl Pts',(-18.7560847700556,12.4723413708497,124.436233688976)) ;
#81378=CARTESIAN_POINT('Ctrl Pts',(-18.7600925339082,12.4721175325591,124.438788767859)) ;
#81379=CARTESIAN_POINT('Ctrl Pts',(-18.764045939796,12.4718973645067,124.441277240356)) ;
#81380=CARTESIAN_POINT('Ctrl Pts',(-18.7719793798138,12.4714567583463,124.44620729276)) ;
#81381=CARTESIAN_POINT('Ctrl Pts',(-18.77595933397,12.4712363241106,124.448648852768)) ;
#81382=CARTESIAN_POINT('Ctrl Pts',(-18.7852393099155,12.4707236865584,124.454268417085)) ;
#81383=CARTESIAN_POINT('Ctrl Pts',(-18.7905496953622,12.4704313438977,124.45742904317)) ;
#81384=CARTESIAN_POINT('Ctrl Pts',(-18.8126117980378,12.4692207609752,124.470333000411)) ;
#81385=CARTESIAN_POINT('Ctrl Pts',(-18.8295711590067,12.4682990129185,124.479715250224)) ;
#81386=CARTESIAN_POINT('Ctrl Pts',(-18.8734329820549,12.4659403416845,124.502627588803)) ;
#81387=CARTESIAN_POINT('Ctrl Pts',(-18.9006275205337,12.4645028407894,124.515570733043)) ;
#81388=CARTESIAN_POINT('Ctrl Pts',(-18.9389095396364,12.4625197033815,124.532075322591)) ;
#81389=CARTESIAN_POINT('Ctrl Pts',(-18.9496093799162,12.46196959824,124.536508036815)) ;
#81390=CARTESIAN_POINT('Ctrl Pts',(-18.9689435129936,12.4609830805354,124.544195746187)) ;
#81391=CARTESIAN_POINT('Ctrl Pts',(-18.9775546023812,12.4605463327404,124.547506641006)) ;
#81392=CARTESIAN_POINT('Ctrl Pts',(-18.9895041541243,12.4599438014985,124.551945596068)) ;
#81393=CARTESIAN_POINT('Ctrl Pts',(-18.9928110353211,12.4597774302085,124.553157680835)) ;
#81394=CARTESIAN_POINT('Ctrl Pts',(-18.996214072409,12.4596065967133,124.554388250743)) ;
#81395=CARTESIAN_POINT('Ctrl Pts',(-18.9963050038545,12.459602032202,124.554421120127)) ;
#81396=CARTESIAN_POINT('Ctrl Pts',(-18.9964908640187,12.4595927030888,124.55448827872)) ;
#81397=CARTESIAN_POINT('Ctrl Pts',(-18.9965857928986,12.4595879385034,124.554522566888)) ;
#81398=CARTESIAN_POINT('Ctrl Pts',(-18.9967798262084,12.4595782003688,124.554592624093)) ;
#81399=CARTESIAN_POINT('Ctrl Pts',(-18.9968789312626,12.4595732268151,124.554628392156)) ;
#81400=CARTESIAN_POINT('Ctrl Pts',(-18.9970815029335,12.4595630614902,124.554701472633)) ;
#81401=CARTESIAN_POINT('Ctrl Pts',(-18.9971849699443,12.4595578697285,124.554738783882)) ;
#81402=CARTESIAN_POINT('Ctrl Pts',(-18.9973964592291,12.4595472583568,124.554815016601)) ;
#81403=CARTESIAN_POINT('Ctrl Pts',(-18.9975044818939,12.4595418387591,124.554853936786)) ;
#81404=CARTESIAN_POINT('Ctrl Pts',(-18.9976716361686,12.4595334530715,124.554914135112)) ;
#81405=CARTESIAN_POINT('Ctrl Pts',(-18.9977307640803,12.4595304868965,124.554935424038)) ;
#81406=CARTESIAN_POINT('Ctrl Pts',(-18.9978625418105,12.4595238764725,124.554982858884)) ;
#81407=CARTESIAN_POINT('Ctrl Pts',(-18.9979351925447,12.4595202322367,124.555009002494)) ;
#81408=CARTESIAN_POINT('Ctrl Pts',(-18.9980970183312,12.4595121152772,124.555067218622)) ;
#81409=CARTESIAN_POINT('Ctrl Pts',(-18.9981861943902,12.4595076425915,124.55509928754)) ;
#81410=CARTESIAN_POINT('Ctrl Pts',(-18.998384692849,12.459497687352,124.555170644045)) ;
#81411=CARTESIAN_POINT('Ctrl Pts',(-18.9984940173644,12.4594922048242,124.555209926471)) ;
#81412=CARTESIAN_POINT('Ctrl Pts',(-18.9987371590971,12.4594800123597,124.555297252653)) ;
#81413=CARTESIAN_POINT('Ctrl Pts',(-18.9988709789515,12.4594733024872,124.555345288541)) ;
#81414=CARTESIAN_POINT('Ctrl Pts',(-18.9991682898217,12.4594583963113,124.555451952146)) ;
#81415=CARTESIAN_POINT('Ctrl Pts',(-18.9993317849728,12.4594502000914,124.555510568293)) ;
#81416=CARTESIAN_POINT('Ctrl Pts',(-18.9996945609775,12.4594320156238,124.555640542663)) ;
#81417=CARTESIAN_POINT('Ctrl Pts',(-18.9998938479544,12.4594220274967,124.555711883881)) ;
#81418=CARTESIAN_POINT('Ctrl Pts',(-19.0002851411589,12.459402418715,124.555851844584)) ;
#81419=CARTESIAN_POINT('Ctrl Pts',(-19.0004771460836,12.4593927980315,124.555920467837)) ;
#81420=CARTESIAN_POINT('Ctrl Pts',(-19.0012197128852,12.4593555953361,124.556185653098)) ;
#81421=CARTESIAN_POINT('Ctrl Pts',(-19.0017703994541,12.4593280158234,124.556381866096)) ;
#81422=CARTESIAN_POINT('Ctrl Pts',(-19.0038154036166,12.4592256346692,124.557108850624)) ;
#81423=CARTESIAN_POINT('Ctrl Pts',(-19.0053106166825,12.4591508512919,124.557637093195)) ;
#81424=CARTESIAN_POINT('Ctrl Pts',(-19.0117012259222,12.4588315326549,124.559880762249)) ;
#81425=CARTESIAN_POINT('Ctrl Pts',(-19.0166065571016,12.4585872025792,124.561567758131)) ;
#81426=CARTESIAN_POINT('Ctrl Pts',(-19.0216270026011,12.4583379011671,124.563258465656)) ;
#81427=CARTESIAN_POINT('Ctrl Pts',(-19.0217314584802,12.4583327145136,124.563293626856)) ;
#81428=CARTESIAN_POINT('Ctrl Pts',(-19.0219415633262,12.4583222826406,124.563364319038)) ;
#81429=CARTESIAN_POINT('Ctrl Pts',(-19.0220472124483,12.4583170374209,124.56339984971)) ;
#81430=CARTESIAN_POINT('Ctrl Pts',(-19.0222598164606,12.4583064828437,124.563471317631)) ;
#81431=CARTESIAN_POINT('Ctrl Pts',(-19.0223667713187,12.4583011734964,124.563507254468)) ;
#81432=CARTESIAN_POINT('Ctrl Pts',(-19.0225821018788,12.4582904849767,124.563579572164)) ;
#81433=CARTESIAN_POINT('Ctrl Pts',(-19.0226904779518,12.4582851057953,124.563615952708)) ;
#81434=CARTESIAN_POINT('Ctrl Pts',(-19.0229087692449,12.4582742717634,124.563689196187)) ;
#81435=CARTESIAN_POINT('Ctrl Pts',(-19.0230186846185,12.4582688169156,124.563726058691)) ;
#81436=CARTESIAN_POINT('Ctrl Pts',(-19.0232401763883,12.458257825533,124.563800305491)) ;
#81437=CARTESIAN_POINT('Ctrl Pts',(-19.023351752842,12.4582522890066,124.563837689277)) ;
#81438=CARTESIAN_POINT('Ctrl Pts',(-19.023576692188,12.458241128077,124.563913019051)) ;
#81439=CARTESIAN_POINT('Ctrl Pts',(-19.0236900554059,12.4582355036699,124.563950964568)) ;
#81440=CARTESIAN_POINT('Ctrl Pts',(-19.0239186981324,12.4582241605729,124.564027459509)) ;
#81441=CARTESIAN_POINT('Ctrl Pts',(-19.0240339776838,12.4582184418942,124.564066008315)) ;
#81442=CARTESIAN_POINT('Ctrl Pts',(-19.0242665875078,12.4582069036251,124.564143752866)) ;
#81443=CARTESIAN_POINT('Ctrl Pts',(-19.0243839179028,12.4582010840432,124.564182947966)) ;
#81444=CARTESIAN_POINT('Ctrl Pts',(-19.0246207686207,12.458189337106,124.564262029517)) ;
#81445=CARTESIAN_POINT('Ctrl Pts',(-19.0247402893849,12.4581834097448,124.564301915371)) ;
#81446=CARTESIAN_POINT('Ctrl Pts',(-19.0249816658408,12.4581714401052,124.564382424547)) ;
#81447=CARTESIAN_POINT('Ctrl Pts',(-19.0251035216686,12.4581653978372,124.564423047106)) ;
#81448=CARTESIAN_POINT('Ctrl Pts',(-19.025349719219,12.4581531909493,124.564505077554)) ;
#81449=CARTESIAN_POINT('Ctrl Pts',(-19.0254740611223,12.4581470263391,124.564546484623)) ;
#81450=CARTESIAN_POINT('Ctrl Pts',(-19.0257253879984,12.4581345670296,124.564630133757)) ;
#81451=CARTESIAN_POINT('Ctrl Pts',(-19.0258523733336,12.4581282723326,124.564672374986)) ;
#81452=CARTESIAN_POINT('Ctrl Pts',(-19.0261091513439,12.4581155447667,124.564757744178)) ;
#81453=CARTESIAN_POINT('Ctrl Pts',(-19.0262389442418,12.4581091119085,124.564800871177)) ;
#81454=CARTESIAN_POINT('Ctrl Pts',(-19.0265015090463,12.4580960995771,124.564888065799)) ;
#81455=CARTESIAN_POINT('Ctrl Pts',(-19.0266342813408,12.4580895201082,124.564932132425)) ;
#81456=CARTESIAN_POINT('Ctrl Pts',(-19.0269029846112,12.4580762057221,124.565021262512)) ;
#81457=CARTESIAN_POINT('Ctrl Pts',(-19.0270389159778,12.4580694708111,124.565066324884)) ;
#81458=CARTESIAN_POINT('Ctrl Pts',(-19.0364123898857,12.4576050873161,124.568171869593)) ;
#81459=CARTESIAN_POINT('Ctrl Pts',(-19.045686391355,12.4571482136245,124.571121288879)) ;
#81460=CARTESIAN_POINT('Ctrl Pts',(-19.0676006511695,12.4560741305134,124.57780186751)) ;
#81461=CARTESIAN_POINT('Ctrl Pts',(-19.0802681764214,12.4554575338223,124.58143940474)) ;
#81462=CARTESIAN_POINT('Ctrl Pts',(-19.1221287196726,12.4534313825446,124.592725955992)) ;
#81463=CARTESIAN_POINT('Ctrl Pts',(-19.1515475027644,12.4520259695632,124.599493465862)) ;
#81464=CARTESIAN_POINT('Ctrl Pts',(-19.1926036909814,12.4500710253046,124.607340598084)) ;
#81465=CARTESIAN_POINT('Ctrl Pts',(-19.2040504531208,12.4495265908159,124.609358630735)) ;
#81466=CARTESIAN_POINT('Ctrl Pts',(-19.2205777903511,12.448739951088,124.61202842498)) ;
#81467=CARTESIAN_POINT('Ctrl Pts',(-19.2256363232185,12.4484991162218,124.612812799154)) ;
#81468=CARTESIAN_POINT('Ctrl Pts',(-19.235307100479,12.4480386298423,124.614249817801)) ;
#81469=CARTESIAN_POINT('Ctrl Pts',(-19.2399184430646,12.4478190270199,124.614907952638)) ;
#81470=CARTESIAN_POINT('Ctrl Pts',(-19.2495396099516,12.4473608353244,124.616224681586)) ;
#81471=CARTESIAN_POINT('Ctrl Pts',(-19.2545499899835,12.4471222192283,124.616878574135)) ;
#81472=CARTESIAN_POINT('Ctrl Pts',(-19.2755098960883,12.44612410801,124.619481124076)) ;
#81473=CARTESIAN_POINT('Ctrl Pts',(-19.2914931641354,12.4453632273878,124.621144523827)) ;
#81474=CARTESIAN_POINT('Ctrl Pts',(-19.3400199729492,12.4430558625448,124.625223573964)) ;
#81475=CARTESIAN_POINT('Ctrl Pts',(-19.3726323283655,12.4415093022874,124.62664571233)) ;
#81476=CARTESIAN_POINT('Ctrl Pts',(-19.4146372795782,12.4395243298544,124.626784260741)) ;
#81477=CARTESIAN_POINT('Ctrl Pts',(-19.4240122513541,12.4390817367332,124.626706669822)) ;
#81478=CARTESIAN_POINT('Ctrl Pts',(-19.4479262366249,12.4379535630246,124.62623189385)) ;
#81479=CARTESIAN_POINT('Ctrl Pts',(-19.4624607378427,12.4372685471284,124.625682131427)) ;
#81480=CARTESIAN_POINT('Ctrl Pts',(-19.505739744189,12.4352276028772,124.623266280612)) ;
#81481=CARTESIAN_POINT('Ctrl Pts',(-19.5344313832049,12.4338729142859,124.620638858866)) ;
#81482=CARTESIAN_POINT('Ctrl Pts',(-19.5732441652108,12.4320281066831,124.615687820181)) ;
#81483=CARTESIAN_POINT('Ctrl Pts',(-19.5834688212528,12.4315409686251,124.614250862273)) ;
#81484=CARTESIAN_POINT('Ctrl Pts',(-19.6033923191214,12.43058891903,124.611191381478)) ;
#81485=CARTESIAN_POINT('Ctrl Pts',(-19.6130922438604,12.4301240908056,124.609581089074)) ;
#81486=CARTESIAN_POINT('Ctrl Pts',(-19.6332590674186,12.4291544519405,124.605981102098)) ;
#81487=CARTESIAN_POINT('Ctrl Pts',(-19.6437214872329,12.4286494617801,124.60397111297)) ;
#81488=CARTESIAN_POINT('Ctrl Pts',(-19.6763822536025,12.4270679706454,124.597249898521)) ;
#81489=CARTESIAN_POINT('Ctrl Pts',(-19.698476044724,12.4259914549365,124.592054178708)) ;
#81490=CARTESIAN_POINT('Ctrl Pts',(-19.7266697639441,12.4246125401667,124.584584682613)) ;
#81491=CARTESIAN_POINT('Ctrl Pts',(-19.7329147663155,12.4243067478347,124.58287662775)) ;
#81492=CARTESIAN_POINT('Ctrl Pts',(-19.7431366683324,12.4238056288648,124.579992846724)) ;
#81493=CARTESIAN_POINT('Ctrl Pts',(-19.7471217202963,12.4236101160344,124.578846534858)) ;
#81494=CARTESIAN_POINT('Ctrl Pts',(-19.7517716917863,12.4233817979331,124.577483142913)) ;
#81495=CARTESIAN_POINT('Ctrl Pts',(-19.7524423820719,12.4233488619146,124.577285864766)) ;
#81496=CARTESIAN_POINT('Ctrl Pts',(-19.7574907149469,12.4231009161189,124.575796202665)) ;
#81497=CARTESIAN_POINT('Ctrl Pts',(-19.7618612202299,12.422886069044,124.574479734891)) ;
#81498=CARTESIAN_POINT('Ctrl Pts',(-19.7722985742821,12.4223724823631,124.571271567179)) ;
#81499=CARTESIAN_POINT('Ctrl Pts',(-19.7783582074024,12.422073901283,124.569356833635)) ;
#81500=CARTESIAN_POINT('Ctrl Pts',(-19.7943685490549,12.4212837423584,124.564159352773)) ;
#81501=CARTESIAN_POINT('Ctrl Pts',(-19.8042922959812,12.4207926806324,124.560795267022)) ;
#81502=CARTESIAN_POINT('Ctrl Pts',(-19.8450857901445,12.4187667234625,124.546375543884)) ;
#81503=CARTESIAN_POINT('Ctrl Pts',(-19.8755450511598,12.4172357058851,124.534200907544)) ;
#81504=CARTESIAN_POINT('Ctrl Pts',(-19.9116559119258,12.4153765671281,124.518043304277)) ;
#81505=CARTESIAN_POINT('Ctrl Pts',(-19.9178140438702,12.4150579857214,124.515225853268)) ;
#81506=CARTESIAN_POINT('Ctrl Pts',(-19.9285034726263,12.4145021708986,124.510226758634)) ;
#81507=CARTESIAN_POINT('Ctrl Pts',(-19.9330453820801,12.414265113429,124.508068189605)) ;
#81508=CARTESIAN_POINT('Ctrl Pts',(-19.9419836110536,12.4137967907583,124.5037520135)) ;
#81509=CARTESIAN_POINT('Ctrl Pts',(-19.9463805474503,12.4135655406944,124.501595899481)) ;
#81510=CARTESIAN_POINT('Ctrl Pts',(-19.9560453773763,12.413055288216,124.496783880251)) ;
#81511=CARTESIAN_POINT('Ctrl Pts',(-19.9613072015799,12.4127762063331,124.494116071267)) ;
#81512=CARTESIAN_POINT('Ctrl Pts',(-19.9984633144749,12.4107963380609,124.474936003137)) ;
#81513=CARTESIAN_POINT('Ctrl Pts',(-20.02963087542,12.4090863940919,124.457055018248)) ;
#81514=CARTESIAN_POINT('Ctrl Pts',(-20.0599602754258,12.4073831970671,124.437819810756)) ;
#81515=CARTESIAN_POINT('Origin',(-19.4092696390626,12.3398872919312,123.411833654984)) ;
#81516=CARTESIAN_POINT('',(-19.4092696390626,12.3998836520522,123.411833654984)) ;
#81517=CARTESIAN_POINT('',(-18.8344050941734,12.0999018514474,123.240115636693)) ;
#81518=CARTESIAN_POINT('',(-19.2942967300848,12.3398872919312,123.377490051326)) ;
#81519=CARTESIAN_POINT('Origin',(-19.4092696390626,12.0999018514474,123.411833654984)) ;
#81520=CARTESIAN_POINT('Origin',(-19.4092696390626,11.9199127710845,123.411833654984)) ;
#81521=CARTESIAN_POINT('',(-18.1240607872049,12.4705811104891,123.027928413015)) ;
#81522=CARTESIAN_POINT('Ctrl Pts',(-20.0599602754274,12.4073831970671,124.437819810754)) ;
#81523=CARTESIAN_POINT('Ctrl Pts',(-20.0004707798595,12.4089443847785,124.479246016639)) ;
#81524=CARTESIAN_POINT('Ctrl Pts',(-19.9375759144554,12.4104965535012,124.515176126025)) ;
#81525=CARTESIAN_POINT('Ctrl Pts',(-19.8055230642977,12.4135619883252,124.575655167027)) ;
#81526=CARTESIAN_POINT('Ctrl Pts',(-19.7366469094468,12.4150958593948,124.600048047181)) ;
#81527=CARTESIAN_POINT('Ctrl Pts',(-19.5229749245386,12.4197782665643,124.655153900126)) ;
#81528=CARTESIAN_POINT('Ctrl Pts',(-19.3738301151842,12.4228609961199,124.665868103026)) ;
#81529=CARTESIAN_POINT('Ctrl Pts',(-19.1462099532735,12.4276127977452,124.64205564411)) ;
#81530=CARTESIAN_POINT('Ctrl Pts',(-19.0660088189675,12.4292659064182,124.625546210781)) ;
#81531=CARTESIAN_POINT('Ctrl Pts',(-18.9099376819915,12.4326333165009,124.577450942515)) ;
#81532=CARTESIAN_POINT('Ctrl Pts',(-18.8339818501442,12.4343499486543,124.545751384892)) ;
#81533=CARTESIAN_POINT('Ctrl Pts',(-18.6883020808879,12.4377451727855,124.467494661077)) ;
#81534=CARTESIAN_POINT('Ctrl Pts',(-18.6190403720584,12.4394104855472,124.420918065797)) ;
#81535=CARTESIAN_POINT('Ctrl Pts',(-18.4905718925471,12.4427709330837,124.315120935469)) ;
#81536=CARTESIAN_POINT('Ctrl Pts',(-18.4314678570159,12.4444740645654,124.25601094446)) ;
#81537=CARTESIAN_POINT('Ctrl Pts',(-18.3246877800231,12.4478688624784,124.126126814797)) ;
#81538=CARTESIAN_POINT('Ctrl Pts',(-18.2775921591984,12.4495305257554,124.055602387271)) ;
#81539=CARTESIAN_POINT('Ctrl Pts',(-18.1975609831306,12.4529109006071,123.90631896517)) ;
#81540=CARTESIAN_POINT('Ctrl Pts',(-18.1646626693663,12.4546483109236,123.827609347576)) ;
#81541=CARTESIAN_POINT('Ctrl Pts',(-18.1149037431104,12.4580007720278,123.665002308302)) ;
#81542=CARTESIAN_POINT('Ctrl Pts',(-18.0980236143064,12.4596416636239,123.58126056863)) ;
#81543=CARTESIAN_POINT('Ctrl Pts',(-18.0801681116067,12.4630480670112,123.410618686017)) ;
#81544=CARTESIAN_POINT('Ctrl Pts',(-18.079700387576,12.4647476001311,123.323794170317)) ;
#81545=CARTESIAN_POINT('Ctrl Pts',(-18.0942444324001,12.4678125093508,123.166790916998)) ;
#81546=CARTESIAN_POINT('Ctrl Pts',(-18.1064133510925,12.4692000007385,123.0966580497)) ;
#81547=CARTESIAN_POINT('Ctrl Pts',(-18.1240607848549,12.4705811104891,123.027928420882)) ;
#81548=CARTESIAN_POINT('',(-20.8811762570041,12.5498512937297,123.700066866625)) ;
#81549=CARTESIAN_POINT('Ctrl Pts',(-20.8811762570041,12.5498512937297,123.700066866625)) ;
#81550=CARTESIAN_POINT('Ctrl Pts',(-20.8239387353199,12.5305321283812,123.791298907814)) ;
#81551=CARTESIAN_POINT('Ctrl Pts',(-20.7477236709935,12.5080679368041,123.891522335765)) ;
#81552=CARTESIAN_POINT('Ctrl Pts',(-20.6010201821559,12.4694919241787,124.025328940159)) ;
#81553=CARTESIAN_POINT('Ctrl Pts',(-20.5520435705854,12.4570505014033,124.063385132327)) ;
#81554=CARTESIAN_POINT('Ctrl Pts',(-20.451686730373,12.4324340735919,124.130565753573)) ;
#81555=CARTESIAN_POINT('Ctrl Pts',(-20.3988578773564,12.4199510743856,124.161083210787)) ;
#81556=CARTESIAN_POINT('Ctrl Pts',(-20.3451307049827,12.4073898409302,124.186586679355)) ;
#81557=CARTESIAN_POINT('Ctrl Pts',(-18.1240607848549,12.4705811104891,123.027928420882)) ;
#81558=CARTESIAN_POINT('Ctrl Pts',(-18.1279098458917,12.4708823427136,123.012937882319)) ;
#81559=CARTESIAN_POINT('Ctrl Pts',(-18.1320193178887,12.471183020255,122.99801403888)) ;
#81560=CARTESIAN_POINT('Ctrl Pts',(-18.161059296499,12.4731748557988,122.899300917852)) ;
#81561=CARTESIAN_POINT('Ctrl Pts',(-18.1939563937343,12.4748348374863,122.817970672594)) ;
#81562=CARTESIAN_POINT('Ctrl Pts',(-18.2750524739676,12.4782125473854,122.662421849023)) ;
#81563=CARTESIAN_POINT('Ctrl Pts',(-18.3233531703796,12.4799263147624,122.588305207079)) ;
#81564=CARTESIAN_POINT('Ctrl Pts',(-18.4340812960901,12.4833084828719,122.450081264731)) ;
#81565=CARTESIAN_POINT('Ctrl Pts',(-18.496341239815,12.4849766794128,122.386340236217)) ;
#81566=CARTESIAN_POINT('Ctrl Pts',(-18.5984276425599,12.4875069623852,122.300239051129)) ;
#81567=CARTESIAN_POINT('Ctrl Pts',(-18.6340836690644,12.488357950932,122.273028142518)) ;
#81568=CARTESIAN_POINT('Ctrl Pts',(-18.7447054878371,12.4908935345292,122.196872452221)) ;
#81569=CARTESIAN_POINT('Ctrl Pts',(-18.8233958024688,12.492561011236,122.153383232491)) ;
#81570=CARTESIAN_POINT('Ctrl Pts',(-18.9877409414025,12.4959478846102,122.082090718853)) ;
#81571=CARTESIAN_POINT('Ctrl Pts',(-19.0732092836722,12.4976141777242,122.054534548675)) ;
#81572=CARTESIAN_POINT('Ctrl Pts',(-19.2511933598784,12.5009671960115,122.015636377078)) ;
#81573=CARTESIAN_POINT('Ctrl Pts',(-19.3435306874433,12.502704565731,122.004769570121)) ;
#81574=CARTESIAN_POINT('Ctrl Pts',(-19.5262352003067,12.5061073744164,122.001418957146)) ;
#81575=CARTESIAN_POINT('Ctrl Pts',(-19.6161591817334,12.507727171673,122.008516660418)) ;
#81576=CARTESIAN_POINT('Ctrl Pts',(-19.7978537234547,12.5110837575643,122.040382303008)) ;
#81577=CARTESIAN_POINT('Ctrl Pts',(-19.8894756330781,12.5128703471317,122.065894447071)) ;
#81578=CARTESIAN_POINT('Ctrl Pts',(-20.0629268598057,12.5162623626902,122.133678007326)) ;
#81579=CARTESIAN_POINT('Ctrl Pts',(-20.1447838037588,12.5178649946103,122.175274708415)) ;
#81580=CARTESIAN_POINT('Ctrl Pts',(-20.3019291037484,12.5212444282736,122.274566651441)) ;
#81581=CARTESIAN_POINT('Ctrl Pts',(-20.3767707100987,12.522982262924,122.332838750037)) ;
#81582=CARTESIAN_POINT('Ctrl Pts',(-20.5138479942751,12.5263554079533,122.463352252629)) ;
#81583=CARTESIAN_POINT('Ctrl Pts',(-20.5758166537567,12.528031334414,122.535122831076)) ;
#81584=CARTESIAN_POINT('Ctrl Pts',(-20.7402840444869,12.5331385715931,122.767564209032)) ;
#81585=CARTESIAN_POINT('Ctrl Pts',(-20.8187421074678,12.5364847742368,122.943199468672)) ;
#81586=CARTESIAN_POINT('Ctrl Pts',(-20.8832644852129,12.5414807225746,123.221724626541)) ;
#81587=CARTESIAN_POINT('Ctrl Pts',(-20.8958426824975,12.5431677444753,123.317292456651)) ;
#81588=CARTESIAN_POINT('Ctrl Pts',(-20.9024557483465,12.5465526000103,123.509223945522)) ;
#81589=CARTESIAN_POINT('Ctrl Pts',(-20.8963747034844,12.5481950593457,123.605216792126)) ;
#81590=CARTESIAN_POINT('Ctrl Pts',(-20.8811762570041,12.5498512937297,123.700066866625)) ;
#81591=CARTESIAN_POINT('',(-19.179323821107,11.9199127710845,123.343146447668)) ;
#81592=CARTESIAN_POINT('Ctrl Pts',(-20.5445227346514,11.9799091312055,123.023213403245)) ;
#81593=CARTESIAN_POINT('Ctrl Pts',(-20.5894944790636,11.9865359820236,123.154537963808)) ;
#81594=CARTESIAN_POINT('Ctrl Pts',(-20.6334264843498,11.9997666085046,123.432369739635)) ;
#81595=CARTESIAN_POINT('Ctrl Pts',(-20.5528870867457,12.0197422297632,123.849423964094)) ;
#81596=CARTESIAN_POINT('Ctrl Pts',(-20.3351947176899,12.0396595646652,124.212660991227)) ;
#81597=CARTESIAN_POINT('Ctrl Pts',(-20.0078997286727,12.0595328413812,124.480006144063)) ;
#81598=CARTESIAN_POINT('Ctrl Pts',(-19.6059596659497,12.0795573315451,124.620366658966)) ;
#81599=CARTESIAN_POINT('Ctrl Pts',(-19.1834847849121,12.0994251726959,124.61509168873)) ;
#81600=CARTESIAN_POINT('Ctrl Pts',(-18.7864895436431,12.1193708235754,124.466037582566)) ;
#81601=CARTESIAN_POINT('Ctrl Pts',(-18.4649120080556,12.1392762241924,124.190860873568)) ;
#81602=CARTESIAN_POINT('Ctrl Pts',(-18.2561386390073,12.1591504520087,123.823451800427)) ;
#81603=CARTESIAN_POINT('Ctrl Pts',(-18.1848458732936,12.1791362428864,123.404512149067)) ;
#81604=CARTESIAN_POINT('Ctrl Pts',(-18.2606755389189,12.1990304855461,122.988387736168)) ;
#81605=CARTESIAN_POINT('Ctrl Pts',(-18.4728668974967,12.2189092016182,122.622775123101)) ;
#81606=CARTESIAN_POINT('Ctrl Pts',(-18.7999576817719,12.2389486514628,122.349782388766)) ;
#81607=CARTESIAN_POINT('Ctrl Pts',(-19.1972059733625,12.2588118130006,122.205994923479)) ;
#81608=CARTESIAN_POINT('Ctrl Pts',(-19.6218869886643,12.2787911810149,122.206159049441)) ;
#81609=CARTESIAN_POINT('Ctrl Pts',(-20.018012005359,12.2986017615377,122.349652549516)) ;
#81610=CARTESIAN_POINT('Ctrl Pts',(-20.3444464973365,12.3185826898233,122.621438196783)) ;
#81611=CARTESIAN_POINT('Ctrl Pts',(-20.5574196739387,12.3384753616927,122.986936030998)) ;
#81612=CARTESIAN_POINT('Ctrl Pts',(-20.6337266981278,12.3584016919798,123.403693608248)) ;
#81613=CARTESIAN_POINT('Ctrl Pts',(-20.5626962923593,12.3783722460721,123.822338681512)) ;
#81614=CARTESIAN_POINT('Ctrl Pts',(-20.3894978118444,12.3949040851597,124.128191080618)) ;
#81615=CARTESIAN_POINT('Ctrl Pts',(-20.1931347282858,12.4082438239873,124.328472259114)) ;
#81616=CARTESIAN_POINT('Ctrl Pts',(-20.0213926648739,12.4182760662059,124.450877135037)) ;
#81617=CARTESIAN_POINT('Ctrl Pts',(-19.8344384158834,12.4281337668493,124.540321523917)) ;
#81618=CARTESIAN_POINT('Ctrl Pts',(-19.6322020198109,12.4381256314886,124.597064382826)) ;
#81619=CARTESIAN_POINT('Ctrl Pts',(-19.4246153604294,12.4480481812487,124.617642782804)) ;
#81620=CARTESIAN_POINT('Ctrl Pts',(-19.1462130895236,12.4613259547422,124.597251052543)) ;
#81621=CARTESIAN_POINT('Ctrl Pts',(-18.8783247008221,12.4746732936828,124.503674838352)) ;
#81622=CARTESIAN_POINT('Ctrl Pts',(-18.6486087635049,12.487880525476,124.347609621771)) ;
#81623=CARTESIAN_POINT('Ctrl Pts',(-18.4978177576768,12.4978676415657,124.201561862873)) ;
#81624=CARTESIAN_POINT('Ctrl Pts',(-18.3749666738686,12.5078185471454,124.032184095878)) ;
#81625=CARTESIAN_POINT('Ctrl Pts',(-18.282681770341,12.5178736491529,123.842034979796)) ;
#81626=CARTESIAN_POINT('Ctrl Pts',(-18.2257950874506,12.527695322474,123.643518287885)) ;
#81627=CARTESIAN_POINT('Ctrl Pts',(-18.203381172838,12.5377537935489,123.433271612789)) ;
#81628=CARTESIAN_POINT('Ctrl Pts',(-18.2179067713694,12.5476784047254,123.225110816846)) ;
#81629=CARTESIAN_POINT('Ctrl Pts',(-18.2846782509593,12.5609557436258,122.95410104125)) ;
#81630=CARTESIAN_POINT('Ctrl Pts',(-18.4211173569722,12.5742546228634,122.706459136274)) ;
#81631=CARTESIAN_POINT('Ctrl Pts',(-18.6137338939602,12.5874934950341,122.50549677162)) ;
#81632=CARTESIAN_POINT('Ctrl Pts',(-18.7832480563762,12.5975001131707,122.380910631003)) ;
#81633=CARTESIAN_POINT('Ctrl Pts',(-18.9724531099051,12.6075310582322,122.287792261205)) ;
#81634=CARTESIAN_POINT('Ctrl Pts',(-19.1713356879387,12.617387231584,122.229594635167)) ;
#81635=CARTESIAN_POINT('Ctrl Pts',(-19.3802129828016,12.6273865025469,122.206224196748)) ;
#81636=CARTESIAN_POINT('Ctrl Pts',(-19.5878656312304,12.6372809543042,122.219099840381)) ;
#81637=CARTESIAN_POINT('Ctrl Pts',(-19.7934896655894,12.6473442701136,122.268715021665)) ;
#81638=CARTESIAN_POINT('Ctrl Pts',(-19.9832142539162,12.6571831268532,122.351202089314)) ;
#81639=CARTESIAN_POINT('Ctrl Pts',(-20.1597894985126,12.6672492486708,122.467780794413)) ;
#81640=CARTESIAN_POINT('Ctrl Pts',(-20.3106265913815,12.677132476395,122.610717001511)) ;
#81641=CARTESIAN_POINT('Ctrl Pts',(-20.4360240786786,12.6871219376738,122.779153363513)) ;
#81642=CARTESIAN_POINT('Ctrl Pts',(-20.5299739101893,12.6970856481003,122.966382455643)) ;
#81643=CARTESIAN_POINT('Ctrl Pts',(-20.5903897211659,12.7070806508312,123.167652541848)) ;
#81644=CARTESIAN_POINT('Ctrl Pts',(-20.6147102751126,12.7171169818415,123.377230943918)) ;
#81645=CARTESIAN_POINT('Ctrl Pts',(-20.6028463796374,12.7269632111838,123.58390229972)) ;
#81646=CARTESIAN_POINT('Ctrl Pts',(-20.5549966972298,12.736948709459,123.788268814636)) ;
#81647=CARTESIAN_POINT('Ctrl Pts',(-20.4729187888963,12.746883612442,123.980370469917)) ;
#81648=CARTESIAN_POINT('Ctrl Pts',(-20.3572021787444,12.7569411155372,124.157299797761)) ;
#81649=CARTESIAN_POINT('Ctrl Pts',(-20.2161112283117,12.7667627719077,124.30808911269)) ;
#81650=CARTESIAN_POINT('Ctrl Pts',(-20.0473094958752,12.7768188345729,124.435340829882)) ;
#81651=CARTESIAN_POINT('Ctrl Pts',(-19.8609443815606,12.7867594992761,124.529924426075)) ;
#81652=CARTESIAN_POINT('Ctrl Pts',(-19.6619130199022,12.7966639032246,124.591112791339)) ;
#81653=CARTESIAN_POINT('Ctrl Pts',(-19.4523192191116,12.8067103882181,124.617049850997)) ;
#81654=CARTESIAN_POINT('Ctrl Pts',(-19.2445050876568,12.8166066160299,124.606538219208)) ;
#81655=CARTESIAN_POINT('Ctrl Pts',(-19.0383681426615,12.8266661995934,124.559383118428)) ;
#81656=CARTESIAN_POINT('Ctrl Pts',(-18.8475319931247,12.8365182092622,124.478858160451)) ;
#81657=CARTESIAN_POINT('Ctrl Pts',(-18.6712600278316,12.8464807407018,124.365762068548)) ;
#81658=CARTESIAN_POINT('Ctrl Pts',(-18.5164450069791,12.8565122889411,124.222542592833)) ;
#81659=CARTESIAN_POINT('Ctrl Pts',(-18.390477483579,12.8664037001542,124.057089548771)) ;
#81660=CARTESIAN_POINT('Ctrl Pts',(-18.2936063772451,12.8764199538622,123.870112758873)) ;
#81661=CARTESIAN_POINT('Ctrl Pts',(-18.2310247387816,12.8864500567069,123.668752580011)) ;
#81662=CARTESIAN_POINT('Ctrl Pts',(-18.204422386425,12.8963065056606,123.46324083498)) ;
#81663=CARTESIAN_POINT('Ctrl Pts',(-18.2137782930825,12.9063055164329,123.253271985163)) ;
#81664=CARTESIAN_POINT('Ctrl Pts',(-18.2587651034631,12.9162007333509,123.050131402828)) ;
#81665=CARTESIAN_POINT('Ctrl Pts',(-18.339668596568,12.9262612487082,122.854741757177)) ;
#81666=CARTESIAN_POINT('Ctrl Pts',(-18.4508077453333,12.9361105420953,122.680014237117)) ;
#81667=CARTESIAN_POINT('Ctrl Pts',(-18.592713145265,12.9461377177753,122.524134235879)) ;
#81668=CARTESIAN_POINT('Ctrl Pts',(-18.7599030550601,12.9561662934024,122.395673635507)) ;
#81669=CARTESIAN_POINT('Ctrl Pts',(-18.9432361554979,12.9660113869483,122.299636177384)) ;
#81670=CARTESIAN_POINT('Ctrl Pts',(-19.143231563781,12.9760026283801,122.235427957992)) ;
#81671=CARTESIAN_POINT('Ctrl Pts',(-19.3523277949078,12.9860384095234,122.207228144837)) ;
#81672=CARTESIAN_POINT('Ctrl Pts',(-19.5592861625854,12.9958906152531,122.215330009686)) ;
#81673=CARTESIAN_POINT('Ctrl Pts',(-19.7640842461694,13.0058527093701,122.259137343665)) ;
#81674=CARTESIAN_POINT('Ctrl Pts',(-19.9592496485709,13.0158752701972,122.338556584842)) ;
#81675=CARTESIAN_POINT('Ctrl Pts',(-20.13609931847,13.0258030418487,122.449432047866)) ;
#81676=CARTESIAN_POINT('Ctrl Pts',(-20.292758411066,13.0358454259736,122.590938523857)) ;
#81677=CARTESIAN_POINT('Ctrl Pts',(-20.4205737272681,13.0457346500442,122.754925408144)) ;
#81678=CARTESIAN_POINT('Ctrl Pts',(-20.5192984833546,13.0557238982115,122.940270443942)) ;
#81679=CARTESIAN_POINT('Ctrl Pts',(-20.5839903547336,13.0656824752535,123.13937958665)) ;
#81680=CARTESIAN_POINT('Ctrl Pts',(-20.6134664474397,13.0755820443448,123.345414260246)) ;
#81681=CARTESIAN_POINT('Ctrl Pts',(-20.606545766267,13.0856299564288,123.556518066984)) ;
#81682=CARTESIAN_POINT('Ctrl Pts',(-20.5638845202153,13.095525310736,123.760161232026)) ;
#81683=CARTESIAN_POINT('Ctrl Pts',(-20.4852609723389,13.1055869612272,123.956508898549)) ;
#81684=CARTESIAN_POINT('Ctrl Pts',(-20.3761562249618,13.1154315766896,124.13238749909)) ;
#81685=CARTESIAN_POINT('Ctrl Pts',(-20.2371197494185,13.125391655591,124.288952093036)) ;
#81686=CARTESIAN_POINT('Ctrl Pts',(-20.0714719776813,13.1354298499494,124.419691976004)) ;
#81687=CARTESIAN_POINT('Ctrl Pts',(-19.8888379913786,13.145303565349,124.518402109954)) ;
#81688=CARTESIAN_POINT('Ctrl Pts',(-19.6879341319038,13.1553752748833,124.585176379889)) ;
#81689=CARTESIAN_POINT('Ctrl Pts',(-19.4834366764819,13.1652077153358,124.615443529714)) ;
#81690=CARTESIAN_POINT('Ctrl Pts',(-19.272605892093,13.1752395362612,124.610216779178)) ;
#81691=CARTESIAN_POINT('Ctrl Pts',(-19.0662333340768,13.1852599061468,124.567919588929)) ;
#81692=CARTESIAN_POINT('Ctrl Pts',(-18.873132979465,13.1951266772805,124.492120670378)) ;
#81693=CARTESIAN_POINT('Ctrl Pts',(-18.6925009208601,13.2051974484699,124.381720145738)) ;
#81694=CARTESIAN_POINT('Ctrl Pts',(-18.537329422245,13.2150406089915,124.244796167475)) ;
#81695=CARTESIAN_POINT('Ctrl Pts',(-18.4059658449901,13.2250208421779,124.08120074674)) ;
#81696=CARTESIAN_POINT('Ctrl Pts',(-18.3049709764517,13.2350393622131,123.896379526624)) ;
#81697=CARTESIAN_POINT('Ctrl Pts',(-18.2380816447624,13.2449226705968,123.699636053287)) ;
#81698=CARTESIAN_POINT('Ctrl Pts',(-18.2058768832933,13.2549909547676,123.490468235174)) ;
#81699=CARTESIAN_POINT('Ctrl Pts',(-18.2101289843034,13.2648210814352,123.283817052542)) ;
#81700=CARTESIAN_POINT('Ctrl Pts',(-18.2508798573275,13.2748876536418,123.076180818645)) ;
#81701=CARTESIAN_POINT('Ctrl Pts',(-18.3258688030346,13.2847778098825,122.882224404602)) ;
#81702=CARTESIAN_POINT('Ctrl Pts',(-18.4340995112208,13.2947703374589,122.702192244666)) ;
#81703=CARTESIAN_POINT('Ctrl Pts',(-18.571661784907,13.3047318273332,122.544287761038)) ;
#81704=CARTESIAN_POINT('Ctrl Pts',(-18.7334033065214,13.3146410492204,122.412979799339)) ;
#81705=CARTESIAN_POINT('Ctrl Pts',(-18.9180669225408,13.3246896290307,122.310402899942)) ;
#81706=CARTESIAN_POINT('Ctrl Pts',(-19.1144428684157,13.3345726035008,122.242506570762)) ;
#81707=CARTESIAN_POINT('Ctrl Pts',(-19.3218592255467,13.3445675146435,122.208921813123)) ;
#81708=CARTESIAN_POINT('Ctrl Pts',(-19.5325087212817,13.3545879012171,122.212159433721)) ;
#81709=CARTESIAN_POINT('Ctrl Pts',(-19.7371141879911,13.3644980050741,122.251364326533)) ;
#81710=CARTESIAN_POINT('Ctrl Pts',(-19.9323647674742,13.374425717284,122.325127289265)) ;
#81711=CARTESIAN_POINT('Ctrl Pts',(-20.1138238775436,13.3844688270513,122.43305489869)) ;
#81712=CARTESIAN_POINT('Ctrl Pts',(-20.2713928547841,13.3943552475068,122.568612065668)) ;
#81713=CARTESIAN_POINT('Ctrl Pts',(-20.4047144716701,13.4043484251125,122.730961914886)) ;
#81714=CARTESIAN_POINT('Ctrl Pts',(-20.5072674311864,13.4142940880164,122.913174188626)) ;
#81715=CARTESIAN_POINT('Ctrl Pts',(-20.5770419820694,13.4242413842216,123.110324466056)) ;
#81716=CARTESIAN_POINT('Ctrl Pts',(-20.6116395125164,13.4342891497995,123.318702120629)) ;
#81717=CARTESIAN_POINT('Ctrl Pts',(-20.609736309306,13.4441373630171,123.525730692802)) ;
#81718=CARTESIAN_POINT('Ctrl Pts',(-20.572167565725,13.4540969358112,123.73171350062)) ;
#81719=CARTESIAN_POINT('Ctrl Pts',(-20.4984960852348,13.4641335568437,123.929428932147)) ;
#81720=CARTESIAN_POINT('Ctrl Pts',(-20.393541247342,13.474014071654,124.108708094483)) ;
#81721=CARTESIAN_POINT('Ctrl Pts',(-20.256803503164,13.4840667229611,124.269810836834)) ;
#81722=CARTESIAN_POINT('Ctrl Pts',(-20.0967179447139,13.4939621212411,124.402720841087)) ;
#81723=CARTESIAN_POINT('Ctrl Pts',(-19.913262767579,13.5040122429472,124.507479244964)) ;
#81724=CARTESIAN_POINT('Ctrl Pts',(-19.717652853567,13.5138965224891,124.577663674712)) ;
#81725=CARTESIAN_POINT('Ctrl Pts',(-19.510645163499,13.523891303781,124.613591990072)) ;
#81726=CARTESIAN_POINT('Ctrl Pts',(-19.301497134244,13.5338391489678,124.612953428536)) ;
#81727=CARTESIAN_POINT('Ctrl Pts',(-19.095840811531,13.5437761123552,124.576354548961)) ;
#81728=CARTESIAN_POINT('Ctrl Pts',(-18.898621765146,13.5537590770924,124.504501861206)) ;
#81729=CARTESIAN_POINT('Ctrl Pts',(-18.7160044603142,13.563802928508,124.398546755933)) ;
#81730=CARTESIAN_POINT('Ctrl Pts',(-18.5576688042803,13.5736311298428,124.265752330225)) ;
#81731=CARTESIAN_POINT('Ctrl Pts',(-18.421408955207,13.5837077024408,124.103605355622)) ;
#81732=CARTESIAN_POINT('Ctrl Pts',(-18.3176011922116,13.5935597824484,123.924323629217)) ;
#81733=CARTESIAN_POINT('Ctrl Pts',(-18.2447623948526,13.6036330674525,123.725509185819)) ;
#81734=CARTESIAN_POINT('Ctrl Pts',(-18.2084518087594,13.613474419163,123.521808388656)) ;
#81735=CARTESIAN_POINT('Ctrl Pts',(-18.2072839710603,13.6234359185595,123.312402282748)) ;
#81736=CARTESIAN_POINT('Ctrl Pts',(-18.2431244045269,13.6334716946895,123.104477458676)) ;
#81737=CARTESIAN_POINT('Ctrl Pts',(-18.3132663380114,13.643360121327,122.908785005835)) ;
#81738=CARTESIAN_POINT('Ctrl Pts',(-18.417302510942,13.6533754434019,122.725719693206)) ;
#81739=CARTESIAN_POINT('Ctrl Pts',(-18.5521194988632,13.6634057923022,122.563574869052)) ;
#81740=CARTESIAN_POINT('Ctrl Pts',(-18.7097686244556,13.6732491679088,122.429528067973)) ;
#81741=CARTESIAN_POINT('Ctrl Pts',(-18.8914413453651,13.683278604806,122.322502836408)) ;
#81742=CARTESIAN_POINT('Ctrl Pts',(-19.0891909781922,13.6933104827389,122.249169480939)) ;
#81743=CARTESIAN_POINT('Ctrl Pts',(-19.2923910474279,13.7031401058444,122.211639192755)) ;
#81744=CARTESIAN_POINT('Ctrl Pts',(-19.5023938465683,13.7131295769975,122.209303796898)) ;
#81745=CARTESIAN_POINT('Ctrl Pts',(-19.7106448780283,13.7231734257599,122.244181273255)) ;
#81746=CARTESIAN_POINT('Ctrl Pts',(-19.9054181998677,13.7329951312916,122.312725993549)) ;
#81747=CARTESIAN_POINT('Ctrl Pts',(-20.0894923668064,13.7430301711194,122.415798371662)) ;
#81748=CARTESIAN_POINT('Ctrl Pts',(-20.2523425461733,13.7530548780108,122.549585334357)) ;
#81749=CARTESIAN_POINT('Ctrl Pts',(-20.3874635188741,13.7629075823516,122.706578430368)) ;
#81750=CARTESIAN_POINT('Ctrl Pts',(-20.495034847891,13.7728957045593,122.886895987857)) ;
#81751=CARTESIAN_POINT('Ctrl Pts',(-20.5692346966723,13.7828241746666,123.08199531323)) ;
#81752=CARTESIAN_POINT('Ctrl Pts',(-20.6090140370944,13.7928131518338,123.288203351907)) ;
#81753=CARTESIAN_POINT('Ctrl Pts',(-20.6120399399708,13.8028509591135,123.499202419839)) ;
#81754=CARTESIAN_POINT('Ctrl Pts',(-20.5793586406497,13.8126972599768,123.703608137573)) ;
#81755=CARTESIAN_POINT('Ctrl Pts',(-20.5108933551934,13.8227230033561,123.902954081901)) ;
#81756=CARTESIAN_POINT('Ctrl Pts',(-20.4083206360127,13.8327538697951,124.087214529611)) ;
#81757=CARTESIAN_POINT('Ctrl Pts',(-20.2782096650615,13.8425912285939,124.247959028834)) ;
#81758=CARTESIAN_POINT('Ctrl Pts',(-20.1200757165618,13.8525831895276,124.386233235836)) ;
#81759=CARTESIAN_POINT('Ctrl Pts',(-19.939381440305,13.8626155520842,124.495031216594)) ;
#81760=CARTESIAN_POINT('Ctrl Pts',(-19.7459291063119,13.8724807126586,124.569766298816)) ;
#81761=CARTESIAN_POINT('Ctrl Pts',(-19.5405428783788,13.8824426172363,124.610756191596)) ;
#81762=CARTESIAN_POINT('Ctrl Pts',(-19.3296341401678,13.892477547312,124.615150409139)) ;
#81763=CARTESIAN_POINT('Ctrl Pts',(-19.1241882630405,13.9023624941656,124.583680284887)) ;
#81764=CARTESIAN_POINT('Ctrl Pts',(-18.9238050412693,13.9124281704771,124.515772547022)) ;
#81765=CARTESIAN_POINT('Ctrl Pts',(-18.7422739018673,13.922267090112,124.416547651095)) ;
#81766=CARTESIAN_POINT('Ctrl Pts',(-18.5769212021709,13.9323305998464,124.284614917872)) ;
#81767=CARTESIAN_POINT('Ctrl Pts',(-18.4394438907327,13.9422242130082,124.12849967911)) ;
#81768=CARTESIAN_POINT('Ctrl Pts',(-18.3301649153485,13.9521682198216,123.950314437566)) ;
#81769=CARTESIAN_POINT('Ctrl Pts',(-18.252931772702,13.9621691741759,123.754727554759)) ;
#81770=CARTESIAN_POINT('Ctrl Pts',(-18.2110520046167,13.9722079318682,123.547897335282)) ;
#81771=CARTESIAN_POINT('Ctrl Pts',(-18.2053814422572,13.9820321160382,123.341422790906)) ;
#81772=CARTESIAN_POINT('Ctrl Pts',(-18.2360559546118,13.9920901816376,123.132225932652)) ;
#81773=CARTESIAN_POINT('Ctrl Pts',(-18.3020120627055,14.0020202284123,122.934144622133)) ;
#81774=CARTESIAN_POINT('Ctrl Pts',(-18.4010833690568,14.0119716707494,122.749875876778)) ;
#81775=CARTESIAN_POINT('Ctrl Pts',(-18.5321101497463,14.0220184679287,122.58421709419)) ;
#81776=CARTESIAN_POINT('Ctrl Pts',(-18.6866603133442,14.0318664086088,122.446457948608)) ;
#81777=CARTESIAN_POINT('Ctrl Pts',(-18.8644655336791,14.0418280399514,122.335821830782)) ;
#81778=CARTESIAN_POINT('Ctrl Pts',(-19.0602066092931,14.0518566993273,122.257452043026)) ;
#81779=CARTESIAN_POINT('Ctrl Pts',(-19.2641111444034,14.0617670022155,122.214707828412)) ;
#81780=CARTESIAN_POINT('Ctrl Pts',(-19.4728544922654,14.0717018967777,122.207453402267)) ;
#81781=CARTESIAN_POINT('Ctrl Pts',(-19.68185738335,14.0817429954446,122.237057210089)) ;
#81782=CARTESIAN_POINT('Ctrl Pts',(-19.8795330772188,14.091630277949,122.301367079773)) ;
#81783=CARTESIAN_POINT('Ctrl Pts',(-20.065123390794,14.1016220184595,122.399728598824)) ;
#81784=CARTESIAN_POINT('Ctrl Pts',(-20.2301072624107,14.1115725676949,122.528359338337)) ;
#81785=CARTESIAN_POINT('Ctrl Pts',(-20.3702567814711,14.1215082453297,122.683224847717)) ;
#81786=CARTESIAN_POINT('Ctrl Pts',(-20.4821496428218,14.1314936631225,122.860862878877)) ;
#81787=CARTESIAN_POINT('Ctrl Pts',(-20.5615945327275,14.141522455993,123.056157709777)) ;
#81788=CARTESIAN_POINT('Ctrl Pts',(-20.6054790276225,14.1514019672209,123.259164195847)) ;
#81789=CARTESIAN_POINT('Ctrl Pts',(-20.6140230839649,14.1613955038939,123.469094160262)) ;
#81790=CARTESIAN_POINT('Ctrl Pts',(-20.5854452308061,14.1714277721577,123.678050018947)) ;
#81791=CARTESIAN_POINT('Ctrl Pts',(-20.5225143012457,14.1812917341636,123.875665243064)) ;
#81792=CARTESIAN_POINT('Ctrl Pts',(-20.4242669170228,14.1913617955085,124.06316684514)) ;
#81793=CARTESIAN_POINT('Ctrl Pts',(-20.2978535530189,14.2012041598572,124.226991191777)) ;
#81794=CARTESIAN_POINT('Ctrl Pts',(-20.1436081129759,14.2111648323597,124.368614423322)) ;
#81795=CARTESIAN_POINT('Ctrl Pts',(-19.9655216612941,14.2212029034275,124.481821948191)) ;
#81796=CARTESIAN_POINT('Ctrl Pts',(-19.773794365022,14.2310765183879,124.561451051005)) ;
#81797=CARTESIAN_POINT('Ctrl Pts',(-19.5671348212395,14.2411487529692,124.607418823694)) ;
#81798=CARTESIAN_POINT('Ctrl Pts',(-19.3607741072514,14.250972771418,124.616812784655)) ;
#81799=CARTESIAN_POINT('Ctrl Pts',(-19.1509484643771,14.261037692394,124.589865490901)) ;
#81800=CARTESIAN_POINT('Ctrl Pts',(-18.8857421831171,14.2742479906888,124.507190925921)) ;
#81801=CARTESIAN_POINT('Ctrl Pts',(-18.6462439305007,14.2875634374207,124.356328829034)) ;
#81802=CARTESIAN_POINT('Ctrl Pts',(-18.4564443867322,14.300853682688,124.151228791517)) ;
#81803=CARTESIAN_POINT('Ctrl Pts',(-18.3421585188713,14.3109044322951,123.973546353508)) ;
#81804=CARTESIAN_POINT('Ctrl Pts',(-18.2619973092775,14.3207170392773,123.783433923944)) ;
#81805=CARTESIAN_POINT('Ctrl Pts',(-18.2145911012313,14.3307881372716,123.577110239697)) ;
#81806=CARTESIAN_POINT('Ctrl Pts',(-18.2041343827819,14.3406777100464,123.369451442456)) ;
#81807=CARTESIAN_POINT('Ctrl Pts',(-18.2378552198279,14.3539478168497,123.092490133588)) ;
#81808=CARTESIAN_POINT('Ctrl Pts',(-18.3698702894281,14.3705645037722,122.76481914799)) ;
#81809=CARTESIAN_POINT('Ctrl Pts',(-18.6050453051043,14.3871385470885,122.502296262875)) ;
#81810=CARTESIAN_POINT('Ctrl Pts',(-18.8388900348431,14.4004351145203,122.349191255889)) ;
#81811=CARTESIAN_POINT('Ctrl Pts',(-19.0327140202685,14.4104651780977,122.266120714729)) ;
#81812=CARTESIAN_POINT('Ctrl Pts',(-19.2351924737432,14.4203590699469,122.218606671375)) ;
#81813=CARTESIAN_POINT('Ctrl Pts',(-19.5133780610374,14.4336118257325,122.202020475397)) ;
#81814=CARTESIAN_POINT('Ctrl Pts',(-19.8616301080899,14.4503399307249,122.274027235168)) ;
#81815=CARTESIAN_POINT('Ctrl Pts',(-20.2206980583628,14.4701707672034,122.495229511939)) ;
#81816=CARTESIAN_POINT('Ctrl Pts',(-20.484680559631,14.4900961590936,122.826481287003)) ;
#81817=CARTESIAN_POINT('Ctrl Pts',(-20.619780680086,14.5100213724456,123.228098196348)) ;
#81818=CARTESIAN_POINT('Ctrl Pts',(-20.6098292278703,14.5299463859307,123.651592133763)) ;
#81819=CARTESIAN_POINT('Ctrl Pts',(-20.4568503086671,14.5498228576307,124.045589431713)) ;
#81820=CARTESIAN_POINT('Ctrl Pts',(-20.1773268323864,14.5698021755395,124.365478490848)) ;
#81821=CARTESIAN_POINT('Ctrl Pts',(-19.8060956324391,14.5897351791155,124.570044599947)) ;
#81822=CARTESIAN_POINT('Ctrl Pts',(-19.3882614992928,14.6096304491432,124.635961690786)) ;
#81823=CARTESIAN_POINT('Ctrl Pts',(-18.9723460744339,14.6295517870491,124.555651059117)) ;
#81824=CARTESIAN_POINT('Ctrl Pts',(-18.6081837802081,14.6495094103152,124.337753576671)) ;
#81825=CARTESIAN_POINT('Ctrl Pts',(-18.3412613988883,14.6693892422725,124.010077128848)) ;
#81826=CARTESIAN_POINT('Ctrl Pts',(-18.201016862601,14.6892710935694,123.611189546996)) ;
#81827=CARTESIAN_POINT('Ctrl Pts',(-18.2061577113468,14.7093421106732,123.184511307658)) ;
#81828=CARTESIAN_POINT('Ctrl Pts',(-18.3545971328961,14.7291493344262,122.790298984124)) ;
#81829=CARTESIAN_POINT('Ctrl Pts',(-18.630222996083,14.749130469995,122.467037934246)) ;
#81830=CARTESIAN_POINT('Ctrl Pts',(-18.9990324357376,14.7690579633343,122.258519647139)) ;
#81831=CARTESIAN_POINT('Ctrl Pts',(-19.4145307497255,14.7888786246921,122.18730127194)) ;
#81832=CARTESIAN_POINT('Ctrl Pts',(-19.8347873100262,14.8089758139139,122.263805837987)) ;
#81833=CARTESIAN_POINT('Ctrl Pts',(-20.1980424116417,14.8287394929222,122.475491393999)) ;
#81834=CARTESIAN_POINT('Ctrl Pts',(-20.4713801712505,14.8487967715953,122.802607740335)) ;
#81835=CARTESIAN_POINT('Ctrl Pts',(-20.6146598483129,14.8685921953427,123.198496247975)) ;
#81836=CARTESIAN_POINT('Ctrl Pts',(-20.6155550087254,14.8885558400703,123.622927778774)) ;
#81837=CARTESIAN_POINT('Ctrl Pts',(-20.470426520549,14.9085393313444,124.022283127792)) ;
#81838=CARTESIAN_POINT('Ctrl Pts',(-20.2007731778919,14.9283468264937,124.345851882021)) ;
#81839=CARTESIAN_POINT('Ctrl Pts',(-19.8340286108545,14.9483294172138,124.560210061234)) ;
#81840=CARTESIAN_POINT('Ctrl Pts',(-19.4180417678935,14.968212071205,124.636132917858)) ;
#81841=CARTESIAN_POINT('Ctrl Pts',(-18.9996611265361,14.9881703160681,124.565621362804)) ;
#81842=CARTESIAN_POINT('Ctrl Pts',(-18.6317275054773,15.0080459031097,124.35759044417)) ;
#81843=CARTESIAN_POINT('Ctrl Pts',(-18.3552455446959,15.0280267912449,124.035054764001)) ;
#81844=CARTESIAN_POINT('Ctrl Pts',(-18.2060499354365,15.0479619323559,123.638243857989)) ;
#81845=CARTESIAN_POINT('Ctrl Pts',(-18.2009208909891,15.067873950367,123.214932035603)) ;
#81846=CARTESIAN_POINT('Ctrl Pts',(-18.3399790656831,15.0877621686106,122.815553113942)) ;
#81847=CARTESIAN_POINT('Ctrl Pts',(-18.5625223680875,15.1043604724575,122.541718610699)) ;
#81848=CARTESIAN_POINT('Ctrl Pts',(-18.7884689621563,15.1176330623603,122.377905248733)) ;
#81849=CARTESIAN_POINT('Ctrl Pts',(-18.9775554066951,15.1276404773112,122.285678430504)) ;
#81850=CARTESIAN_POINT('Ctrl Pts',(-19.1798597516223,15.1376478240438,122.22785769584)) ;
#81851=CARTESIAN_POINT('Ctrl Pts',(-19.457193918436,15.1509141838454,122.19875899803)) ;
#81852=CARTESIAN_POINT('Ctrl Pts',(-19.8041247998046,15.1674288414683,122.253102887633)) ;
#81853=CARTESIAN_POINT('Ctrl Pts',(-20.1135389192194,15.184026274711,122.4226744457)) ;
#81854=CARTESIAN_POINT('Ctrl Pts',(-20.3161544867179,15.197374271856,122.616914600856)) ;
#81855=CARTESIAN_POINT('Ctrl Pts',(-20.4392738849815,15.2072700262076,122.784604378727)) ;
#81856=CARTESIAN_POINT('Ctrl Pts',(-20.5324949089409,15.2172579801389,122.972739458481)) ;
#81857=CARTESIAN_POINT('Ctrl Pts',(-20.5915500229038,15.2272152038437,123.173594433495)) ;
#81858=CARTESIAN_POINT('Ctrl Pts',(-20.61491405898,15.2372507504003,123.383260935523)) ;
#81859=CARTESIAN_POINT('Ctrl Pts',(-20.6018719810459,15.2471378616764,123.590723454185)) ;
#81860=CARTESIAN_POINT('Ctrl Pts',(-20.5528214869393,15.2571292667773,123.79495655389)) ;
#81861=CARTESIAN_POINT('Ctrl Pts',(-20.469375655594,15.2670748879921,123.986671291111)) ;
#81862=CARTESIAN_POINT('Ctrl Pts',(-20.3542146612541,15.2770241362604,124.161292940439)) ;
#81863=CARTESIAN_POINT('Ctrl Pts',(-20.2089133776194,15.287070631429,124.314566336844)) ;
#81864=CARTESIAN_POINT('Ctrl Pts',(-20.042609411081,15.2969219742205,124.438017667828)) ;
#81865=CARTESIAN_POINT('Ctrl Pts',(-19.8554011038652,15.3068937543479,124.532309413521)) ;
#81866=CARTESIAN_POINT('Ctrl Pts',(-19.6541309470983,15.3168889543256,124.592800416461)) ;
#81867=CARTESIAN_POINT('Ctrl Pts',(-19.4446258145735,15.3269229460216,124.617258984874)) ;
#81868=CARTESIAN_POINT('Ctrl Pts',(-19.2377471749459,15.3367783509941,124.605514108099)) ;
#81869=CARTESIAN_POINT('Ctrl Pts',(-19.0330947230129,15.3467776488399,124.55762545372)) ;
#81870=CARTESIAN_POINT('Ctrl Pts',(-18.8417260232628,15.3566727614451,124.475969746375)) ;
#81871=CARTESIAN_POINT('Ctrl Pts',(-18.6645920999811,15.3667334069801,124.360440268439)) ;
#81872=CARTESIAN_POINT('Ctrl Pts',(-18.5133455015667,15.3765822839693,124.219009644722)) ;
#81873=CARTESIAN_POINT('Ctrl Pts',(-18.3862687864151,15.3866109950629,124.050778478714)) ;
#81874=CARTESIAN_POINT('Ctrl Pts',(-18.290833948785,15.396640396319,123.86275858809)) ;
#81875=CARTESIAN_POINT('Ctrl Pts',(-18.2302119049096,15.406480588115,123.66496496262)) ;
#81876=CARTESIAN_POINT('Ctrl Pts',(-18.2040500549491,15.416484017308,123.456316143428)) ;
#81877=CARTESIAN_POINT('Ctrl Pts',(-18.2145657244891,15.4264695297742,123.246616916574)) ;
#81878=CARTESIAN_POINT('Ctrl Pts',(-18.26178793961,15.4365106261582,123.040892392394)) ;
#81879=CARTESIAN_POINT('Ctrl Pts',(-18.3421420875874,15.4463538221092,122.850175898891)) ;
#81880=CARTESIAN_POINT('Ctrl Pts',(-18.4556407659876,15.4563401331636,122.673598929047)) ;
#81881=CARTESIAN_POINT('Ctrl Pts',(-18.5972860767463,15.4662748184213,122.520057465721)) ;
#81882=CARTESIAN_POINT('Ctrl Pts',(-18.7655513631646,15.4763323796383,122.392067434468)) ;
#81883=CARTESIAN_POINT('Ctrl Pts',(-18.9489772344995,15.4861540212469,122.297204603864)) ;
#81884=CARTESIAN_POINT('Ctrl Pts',(-19.1506365335545,15.4962100848379,122.233796786976)) ;
#81885=CARTESIAN_POINT('Ctrl Pts',(-19.3579112056646,15.5061507605997,122.207051934583)) ;
#81886=CARTESIAN_POINT('Ctrl Pts',(-19.5659421426239,15.516055119388,122.216014786074)) ;
#81887=CARTESIAN_POINT('Ctrl Pts',(-19.772129699741,15.5261017739638,122.261734136277)) ;
#81888=CARTESIAN_POINT('Ctrl Pts',(-19.9644276677444,15.5359973686067,122.34119219078)) ;
#81889=CARTESIAN_POINT('Ctrl Pts',(-20.1429244164977,15.5460593152635,122.454662034304)) ;
#81890=CARTESIAN_POINT('Ctrl Pts',(-20.2957651324477,15.5559089391957,122.594383759069)) ;
#81891=CARTESIAN_POINT('Ctrl Pts',(-20.4240143606613,15.5658721782255,122.759973311807)) ;
#81892=CARTESIAN_POINT('Ctrl Pts',(-20.5219183135764,15.5758967530014,122.946614158251)) ;
#81893=CARTESIAN_POINT('Ctrl Pts',(-20.5853737236392,15.5858153156891,123.145237961311)) ;
#81894=CARTESIAN_POINT('Ctrl Pts',(-20.6139543239796,15.5958075024131,123.353364337211)) ;
#81895=CARTESIAN_POINT('Ctrl Pts',(-20.605550036432,15.6058423009973,123.564151643716)) ;
#81896=CARTESIAN_POINT('Ctrl Pts',(-20.5618195347646,15.6156974916709,123.766687362844)) ;
#81897=CARTESIAN_POINT('Ctrl Pts',(-20.482721928661,15.6256968398239,123.96141891483)) ;
#81898=CARTESIAN_POINT('Ctrl Pts',(-20.3723321482436,15.6355919654991,124.137780679672)) ;
#81899=CARTESIAN_POINT('Ctrl Pts',(-20.2306926367424,15.6456525084472,124.294818439706)) ;
#81900=CARTESIAN_POINT('Ctrl Pts',(-20.0674780437418,15.6555017827141,124.422264726541)) ;
#81901=CARTESIAN_POINT('Ctrl Pts',(-19.8815798640716,15.665529007284,124.521651786014)) ;
#81902=CARTESIAN_POINT('Ctrl Pts',(-19.6810377876268,15.6755574064718,124.586740135574)) ;
#81903=CARTESIAN_POINT('Ctrl Pts',(-19.4761222669464,15.6854031568852,124.615862634401)) ;
#81904=CARTESIAN_POINT('Ctrl Pts',(-19.2662142305259,15.695391947286,124.609449912632)) ;
#81905=CARTESIAN_POINT('Ctrl Pts',(-19.0595807224344,15.7054368756857,124.565927885616)) ;
#81906=CARTESIAN_POINT('Ctrl Pts',(-18.8677446564262,15.7152613604747,124.489355654725)) ;
#81907=CARTESIAN_POINT('Ctrl Pts',(-18.6878182095202,15.7253187580159,124.378336126653)) ;
#81908=CARTESIAN_POINT('Ctrl Pts',(-18.5321217513917,15.7352448496021,124.239371234552)) ;
#81909=CARTESIAN_POINT('Ctrl Pts',(-18.4021311728377,15.7451996347466,124.075359055294)) ;
#81910=CARTESIAN_POINT('Ctrl Pts',(-18.3019733000776,15.7552370044043,123.889627359725)) ;
#81911=CARTESIAN_POINT('Ctrl Pts',(-18.2364143023807,15.7651258145259,123.692335431482)) ;
#81912=CARTESIAN_POINT('Ctrl Pts',(-18.2054278152639,15.7751151735769,123.484630912349)) ;
#81913=CARTESIAN_POINT('Ctrl Pts',(-18.2111153581584,15.785073721033,123.275354627164)) ;
#81914=CARTESIAN_POINT('Ctrl Pts',(-18.2523061623846,15.7949732975841,123.071338434884)) ;
#81915=CARTESIAN_POINT('Ctrl Pts',(-18.329490776144,15.8050212094148,122.874729160765)) ;
#81916=CARTESIAN_POINT('Ctrl Pts',(-18.4378567623646,15.8149165572753,122.697113500965)) ;
#81917=CARTESIAN_POINT('Ctrl Pts',(-18.5776691405104,15.8249782338065,122.538410360444)) ;
#81918=CARTESIAN_POINT('Ctrl Pts',(-18.739350169092,15.8348227515557,122.409198097224)) ;
#81919=CARTESIAN_POINT('Ctrl Pts',(-18.9227807641953,15.8447831952704,122.308206346156)) ;
#81920=CARTESIAN_POINT('Ctrl Pts',(-19.1226076900904,15.8548200280887,122.240451395418)) ;
#81921=CARTESIAN_POINT('Ctrl Pts',(-19.3278520560388,15.8646988248355,122.208586052293)) ;
#81922=CARTESIAN_POINT('Ctrl Pts',(-19.5392660873161,15.8747581409638,122.212851544582)) ;
#81923=CARTESIAN_POINT('Ctrl Pts',(-19.7428659929903,15.8846285877171,122.252995254409)) ;
#81924=CARTESIAN_POINT('Ctrl Pts',(-19.9389930726343,15.8946212259751,122.328273341098)) ;
#81925=CARTESIAN_POINT('Ctrl Pts',(-20.1195385569295,15.904653241523,122.437273858021)) ;
#81926=CARTESIAN_POINT('Ctrl Pts',(-20.2761009241912,15.9145190978296,122.573347765819)) ;
#81927=CARTESIAN_POINT('Ctrl Pts',(-20.4093380273943,15.9245883872987,122.737816277399)) ;
#81928=CARTESIAN_POINT('Ctrl Pts',(-20.5097308458922,15.93443194485,122.918789574222)) ;
#81929=CARTESIAN_POINT('Ctrl Pts',(-20.5787544498906,15.9444120716378,123.116917393126)) ;
#81930=CARTESIAN_POINT('Ctrl Pts',(-20.6120581104924,15.9544306202378,123.324883620406)) ;
#81931=CARTESIAN_POINT('Ctrl Pts',(-20.6092324188456,15.964313920761,123.53266749653)) ;
#81932=CARTESIAN_POINT('Ctrl Pts',(-20.5695642742578,15.9743822078091,123.740549105626)) ;
#81933=CARTESIAN_POINT('Ctrl Pts',(-20.4963847976889,15.9842123308277,123.933856076758)) ;
#81934=CARTESIAN_POINT('Ctrl Pts',(-20.3884819599051,15.9942789147531,124.115873458542)) ;
#81935=CARTESIAN_POINT('Ctrl Pts',(-20.2528965388693,16.0041690277675,124.273541553575)) ;
#81936=CARTESIAN_POINT('Ctrl Pts',(-20.0906428375853,16.0141617165302,124.406954216609)) ;
#81937=CARTESIAN_POINT('Ctrl Pts',(-19.9081751563257,16.0241226048859,124.509724874185)) ;
#81938=CARTESIAN_POINT('Ctrl Pts',(-19.7116275426118,16.0340405497659,124.579282843754)) ;
#81939=CARTESIAN_POINT('Ctrl Pts',(-19.5041323834058,16.0440483028621,124.614214939347)) ;
#81940=CARTESIAN_POINT('Ctrl Pts',(-19.29326855203,16.0540793968212,124.612157277847)) ;
#81941=CARTESIAN_POINT('Ctrl Pts',(-19.0896398485272,16.0639273648492,124.574676420677)) ;
#81942=CARTESIAN_POINT('Ctrl Pts',(-18.8913605350658,16.073989320975,124.50102077639)) ;
#81943=CARTESIAN_POINT('Ctrl Pts',(-18.7119475644722,16.0838865325762,124.395627492663)) ;
#81944=CARTESIAN_POINT('Ctrl Pts',(-18.5525797590912,16.0938176992408,124.260752898042)) ;
#81945=CARTESIAN_POINT('Ctrl Pts',(-18.4177343388883,16.103859883445,124.098313844903)) ;
#81946=CARTESIAN_POINT('Ctrl Pts',(-18.3146251501111,16.1137465516981,123.917832423583)) ;
#81947=CARTESIAN_POINT('Ctrl Pts',(-18.2433394533002,16.1237396636764,123.720221174115)) ;
#81948=CARTESIAN_POINT('Ctrl Pts',(-18.2076942572138,16.1336853412922,123.514192350361)) ;
#81949=CARTESIAN_POINT('Ctrl Pts',(-18.2079375236498,16.1436326442772,123.305059089537)) ;
#81950=CARTESIAN_POINT('Ctrl Pts',(-18.2450857238941,16.1536803680239,123.097121717048)) ;
#81951=CARTESIAN_POINT('Ctrl Pts',(-18.3161807940119,16.1635287417865,122.902670785188)) ;
#81952=CARTESIAN_POINT('Ctrl Pts',(-18.4205216585494,16.1734877142322,122.721154060357)) ;
#81953=CARTESIAN_POINT('Ctrl Pts',(-18.5561610324773,16.1835265761133,122.559473799906)) ;
#81954=CARTESIAN_POINT('Ctrl Pts',(-18.7150408954212,16.1934051802851,122.425694987581)) ;
#81955=CARTESIAN_POINT('Ctrl Pts',(-18.8977929392953,16.2034567214885,122.319658585763)) ;
#81956=CARTESIAN_POINT('Ctrl Pts',(-19.0931360052247,16.2133521194688,122.248009860964)) ;
#81957=CARTESIAN_POINT('Ctrl Pts',(-19.3010941183184,16.2234033520141,122.210689224517)) ;
#81958=CARTESIAN_POINT('Ctrl Pts',(-19.5089537512372,16.2332895426384,122.210030667253)) ;
#81959=CARTESIAN_POINT('Ctrl Pts',(-19.7159989180033,16.2432820819541,122.245467035054)) ;
#81960=CARTESIAN_POINT('Ctrl Pts',(-19.912880843383,16.2532305278489,122.316077257933)) ;
#81961=CARTESIAN_POINT('Ctrl Pts',(-20.0944193479257,16.2631673303808,122.419404599673)) ;
#81962=CARTESIAN_POINT('Ctrl Pts',(-20.2562110345139,16.2731503378321,122.553127840936)) ;
#81963=CARTESIAN_POINT('Ctrl Pts',(-20.392826960401,16.2831941792469,122.714098614043)) ;
#81964=CARTESIAN_POINT('Ctrl Pts',(-20.4975783868843,16.2930223778708,122.892232473459)) ;
#81965=CARTESIAN_POINT('Ctrl Pts',(-20.5717018307411,16.303098971313,123.090636621067)) ;
#81966=CARTESIAN_POINT('Ctrl Pts',(-20.6095109727593,16.3129509706546,123.294322600127)) ;
#81967=CARTESIAN_POINT('Ctrl Pts',(-20.6115947138046,16.3230245574784,123.506054671263)) ;
#81968=CARTESIAN_POINT('Ctrl Pts',(-20.5776393567891,16.3328647825759,123.710139991898)) ;
#81969=CARTESIAN_POINT('Ctrl Pts',(-20.5085932982019,16.3428304866046,123.907927939968)) ;
#81970=CARTESIAN_POINT('Ctrl Pts',(-20.4053465774814,16.3528571199112,124.091716983098)) ;
#81971=CARTESIAN_POINT('Ctrl Pts',(-20.2733735919819,16.362771415623,124.253036040026)) ;
#81972=CARTESIAN_POINT('Ctrl Pts',(-20.1144503949313,16.3727597043154,124.390304188214)) ;
#81973=CARTESIAN_POINT('Ctrl Pts',(-19.9330154611805,16.3827984374738,124.498096915543)) ;
#81974=CARTESIAN_POINT('Ctrl Pts',(-19.7395811105255,16.3926417693013,124.571625597567)) ;
#81975=CARTESIAN_POINT('Ctrl Pts',(-19.5326001724498,16.4026694951809,124.611656473864)) ;
#81976=CARTESIAN_POINT('Ctrl Pts',(-19.3217012598712,16.4127018315695,124.614568733438)) ;
#81977=CARTESIAN_POINT('Ctrl Pts',(-19.1176631418604,16.4225313318701,124.581915860113)) ;
#81978=CARTESIAN_POINT('Ctrl Pts',(-18.9189922527592,16.4325208357869,124.513822081444)) ;
#81979=CARTESIAN_POINT('Ctrl Pts',(-18.7344293002481,16.4425646762993,124.411248255595)) ;
#81980=CARTESIAN_POINT('Ctrl Pts',(-18.5738358373638,16.4523863820673,124.281460870642)) ;
#81981=CARTESIAN_POINT('Ctrl Pts',(-18.434881893899,16.4624214291997,124.12271871664)) ;
#81982=CARTESIAN_POINT('Ctrl Pts',(-18.3262087635374,16.4724461066366,123.942138990231)) ;
#81983=CARTESIAN_POINT('Ctrl Pts',(-18.2514329538547,16.482298921491,123.748970510266)) ;
#81984=CARTESIAN_POINT('Ctrl Pts',(-18.2104254283557,16.4922866310986,123.543056577685)) ;
#81985=CARTESIAN_POINT('Ctrl Pts',(-18.2058105603721,16.5022166410927,123.334340206634)) ;
#81986=CARTESIAN_POINT('Ctrl Pts',(-18.2373758713605,16.5122063963118,123.126705719172)) ;
#81987=CARTESIAN_POINT('Ctrl Pts',(-18.3050193572529,16.5222330049947,122.927059272191)) ;
#81988=CARTESIAN_POINT('Ctrl Pts',(-18.4046805568282,16.5321169450166,122.7447319742)) ;
#81989=CARTESIAN_POINT('Ctrl Pts',(-18.5354936535171,16.5421061725551,122.580436407492)) ;
#81990=CARTESIAN_POINT('Ctrl Pts',(-18.6939750843828,16.5521490430788,122.440936928317)) ;
#81991=CARTESIAN_POINT('Ctrl Pts',(-18.8703193515889,16.5619814298342,122.33309621936)) ;
#81992=CARTESIAN_POINT('Ctrl Pts',(-19.0656339220194,16.5719747230058,122.255709958654)) ;
#81993=CARTESIAN_POINT('Ctrl Pts',(-19.2723178782231,16.5820067286542,122.213677942991)) ;
#81994=CARTESIAN_POINT('Ctrl Pts',(-19.4796281167346,16.5918719846232,122.208007210698)) ;
#81995=CARTESIAN_POINT('Ctrl Pts',(-19.6868865943995,16.6018338645307,122.23813162248)) ;
#81996=CARTESIAN_POINT('Ctrl Pts',(-19.887099697081,16.6118687978926,122.304588583073)) ;
#81997=CARTESIAN_POINT('Ctrl Pts',(-20.0701600638373,16.6217537562719,122.403012885151)) ;
#81998=CARTESIAN_POINT('Ctrl Pts',(-20.2362528490299,16.6318193831945,122.534076877196)) ;
#81999=CARTESIAN_POINT('Ctrl Pts',(-20.3740988588356,16.6416584888589,122.688345892466)) ;
#82000=CARTESIAN_POINT('Ctrl Pts',(-20.4857489154389,16.6517213038642,122.868002484053)) ;
#82001=CARTESIAN_POINT('Ctrl Pts',(-20.5630460687322,16.6616175099129,123.061183032358)) ;
#82002=CARTESIAN_POINT('Ctrl Pts',(-20.6063783427559,16.6715583329382,123.265604149292)) ;
#82003=CARTESIAN_POINT('Ctrl Pts',(-20.6136572723222,16.6815629159168,123.475829767627)) ;
#82004=CARTESIAN_POINT('Ctrl Pts',(-20.5840255687026,16.6915838103616,123.68440137035)) ;
#82005=CARTESIAN_POINT('Ctrl Pts',(-20.519713862323,16.701475730951,123.88217222093)) ;
#82006=CARTESIAN_POINT('Ctrl Pts',(-20.4213081374851,16.7114691632964,124.067785900772)) ;
#82007=CARTESIAN_POINT('Ctrl Pts',(-20.2927295608921,16.7214147681962,124.232664555243)) ;
#82008=CARTESIAN_POINT('Ctrl Pts',(-20.1377257127213,16.7313620416778,124.37306033678)) ;
#82009=CARTESIAN_POINT('Ctrl Pts',(-19.9587973051972,16.7414099561541,124.48532564178)) ;
#82010=CARTESIAN_POINT('Ctrl Pts',(-19.7670526137768,16.7512575965015,124.563399289271)) ;
#82011=CARTESIAN_POINT('Ctrl Pts',(-19.5624702723363,16.7612193118781,124.608137597195)) ;
#82012=CARTESIAN_POINT('Ctrl Pts',(-19.351788240765,16.7712479354509,124.616465589517)) ;
#82013=CARTESIAN_POINT('Ctrl Pts',(-19.1453379706875,16.7811582975173,124.588489764781)) ;
#82014=CARTESIAN_POINT('Ctrl Pts',(-18.9462095070637,16.7910929911697,124.52545651433)) ;
#82015=CARTESIAN_POINT('Ctrl Pts',(-18.7591671244395,16.8011348342976,124.42758603691)) ;
#82016=CARTESIAN_POINT('Ctrl Pts',(-18.5944417057161,16.811019339868,124.300871726085)) ;
#82017=CARTESIAN_POINT('Ctrl Pts',(-18.4524057695084,16.8210214436532,124.145859468398)) ;
#82018=CARTESIAN_POINT('Ctrl Pts',(-18.340207999891,16.8309397950682,123.970062273976)) ;
#82019=CARTESIAN_POINT('Ctrl Pts',(-18.2592729248101,16.8409874510891,123.774984976864)) ;
#82020=CARTESIAN_POINT('Ctrl Pts',(-18.2140000295948,16.8508586441173,123.572415400728)) ;
#82021=CARTESIAN_POINT('Ctrl Pts',(-18.2043727844571,16.8609243572608,123.361070125236)) ;
#82022=CARTESIAN_POINT('Ctrl Pts',(-18.230785233552,16.8707768178334,123.15557468565)) ;
#82023=CARTESIAN_POINT('Ctrl Pts',(-18.3149326595085,16.884205280556,122.88617187367)) ;
#82024=CARTESIAN_POINT('Ctrl Pts',(-18.4633057586097,16.8972862280731,122.650748676165)) ;
#82025=CARTESIAN_POINT('Ctrl Pts',(-18.6709271509889,16.9107607263076,122.458191539496)) ;
#82026=CARTESIAN_POINT('Ctrl Pts',(-18.8447722117222,16.9205928299171,122.346294262746)) ;
#82027=CARTESIAN_POINT('Ctrl Pts',(-19.0376048145137,16.9305587330438,122.264442659652)) ;
#82028=CARTESIAN_POINT('Ctrl Pts',(-19.2431084187965,16.940586142354,122.217330844712)) ;
#82029=CARTESIAN_POINT('Ctrl Pts',(-19.451166029566,16.9504971737206,122.206685708904)) ;
#82030=CARTESIAN_POINT('Ctrl Pts',(-19.7276789875147,16.9637414813416,122.240089337459)) ;
#82031=CARTESIAN_POINT('Ctrl Pts',(-20.0569136948359,16.9804419640128,122.372795307525)) ;
#82032=CARTESIAN_POINT('Ctrl Pts',(-20.318335465656,16.9969487931686,122.60717328351)) ;
#82033=CARTESIAN_POINT('Ctrl Pts',(-20.4717078308237,17.0102594214062,122.841129236635)) ;
#82034=CARTESIAN_POINT('Ctrl Pts',(-20.5546945465041,17.0202519849463,123.0341657377)) ;
#82035=CARTESIAN_POINT('Ctrl Pts',(-20.6028174013198,17.0302820679478,123.239432150588)) ;
#82036=CARTESIAN_POINT('Ctrl Pts',(-20.6188287669329,17.0434556719456,123.515992319437)) ;
#82037=CARTESIAN_POINT('Ctrl Pts',(-20.5476980425484,17.060093377177,123.862375167711)) ;
#82038=CARTESIAN_POINT('Ctrl Pts',(-20.3266354431392,17.0799751397444,124.222885241376)) ;
#82039=CARTESIAN_POINT('Ctrl Pts',(-20.0488094967542,17.0966714919609,124.443797368873)) ;
#82040=CARTESIAN_POINT('Ctrl Pts',(-19.7952426665839,17.10982851975,124.554332583483)) ;
#82041=CARTESIAN_POINT('Ctrl Pts',(-19.5219785942262,17.1232058743935,124.620786207619)) ;
#82042=CARTESIAN_POINT('Ctrl Pts',(-19.1705568147902,17.1397367086523,124.612580143332)) ;
#82043=CARTESIAN_POINT('Ctrl Pts',(-18.7748002339287,17.1597013983954,124.459120979636)) ;
#82044=CARTESIAN_POINT('Ctrl Pts',(-18.4561699434069,17.1796178918191,124.18016633333)) ;
#82045=CARTESIAN_POINT('Ctrl Pts',(-18.251376561792,17.1995076111686,123.810101526073)) ;
#82046=CARTESIAN_POINT('Ctrl Pts',(-18.1851276822054,17.2195143408165,123.389957438637)) ;
#82047=CARTESIAN_POINT('Ctrl Pts',(-18.265260003141,17.2393523944634,122.975738571344)) ;
#82048=CARTESIAN_POINT('Ctrl Pts',(-18.4831733622697,17.259345732677,122.610816790265)) ;
#82049=CARTESIAN_POINT('Ctrl Pts',(-18.8110017559419,17.2792285320836,122.343752288443)) ;
#82050=CARTESIAN_POINT('Ctrl Pts',(-19.2100490249569,17.2991207130023,122.203910324025)) ;
#82051=CARTESIAN_POINT('Ctrl Pts',(-19.6333306351389,17.3190228914974,122.207929474009)) ;
#82052=CARTESIAN_POINT('Ctrl Pts',(-20.0320400933982,17.3390602027011,122.357765014815)) ;
#82053=CARTESIAN_POINT('Ctrl Pts',(-20.3526643050806,17.358872644242,122.6313021622)) ;
#82054=CARTESIAN_POINT('Ctrl Pts',(-20.56304176731,17.3789378849769,123.002232875681)) ;
#82055=CARTESIAN_POINT('Ctrl Pts',(-20.6335141765675,17.3986950898327,123.41657822951)) ;
#82056=CARTESIAN_POINT('Ctrl Pts',(-20.5580063907539,17.4187283624784,123.83557538103)) ;
#82057=CARTESIAN_POINT('Ctrl Pts',(-20.3461519216991,17.4385412709322,124.199927820861)) ;
#82058=CARTESIAN_POINT('Ctrl Pts',(-20.0203445224272,17.4585374170597,124.472800756352)) ;
#82059=CARTESIAN_POINT('Ctrl Pts',(-19.6233800168032,17.4783991702822,124.617465592322)) ;
#82060=CARTESIAN_POINT('Ctrl Pts',(-19.1967646853301,17.4984676874103,124.617721492029)) ;
#82061=CARTESIAN_POINT('Ctrl Pts',(-18.8003376642784,17.5182985604071,124.473776925844)) ;
#82062=CARTESIAN_POINT('Ctrl Pts',(-18.4747560307729,17.5382204712238,124.202953891927)) ;
#82063=CARTESIAN_POINT('Ctrl Pts',(-18.2610777332137,17.5581499146591,123.836937868401)) ;
#82064=CARTESIAN_POINT('Ctrl Pts',(-18.1850738365675,17.5780595847755,123.420547828184)) ;
#82065=CARTESIAN_POINT('Ctrl Pts',(-18.2548694891289,17.5979329420383,123.003739230976)) ;
#82066=CARTESIAN_POINT('Ctrl Pts',(-18.4639624788878,17.6179244766563,122.633712881794)) ;
#82067=CARTESIAN_POINT('Ctrl Pts',(-18.7847202419542,17.637790094067,122.35877951611)) ;
#82068=CARTESIAN_POINT('Ctrl Pts',(-19.1821148442675,17.6577710238952,122.208575263194)) ;
#82069=CARTESIAN_POINT('Ctrl Pts',(-19.6060391285895,17.6777094859784,122.203480332858)) ;
#82070=CARTESIAN_POINT('Ctrl Pts',(-20.0055817549243,17.6976016792001,122.342419869265)) ;
#82071=CARTESIAN_POINT('Ctrl Pts',(-20.3347847387671,17.7175723942355,122.610483331917)) ;
#82072=CARTESIAN_POINT('Ctrl Pts',(-20.5517123532575,17.7373820659016,122.97165207797)) ;
#82073=CARTESIAN_POINT('Ctrl Pts',(-20.6333779860565,17.7573752825927,123.388684203349)) ;
#82074=CARTESIAN_POINT('Ctrl Pts',(-20.5685930951932,17.7772261947891,123.805942343805)) ;
#82075=CARTESIAN_POINT('Ctrl Pts',(-20.362939595394,17.7973008011081,124.179847955856)) ;
#82076=CARTESIAN_POINT('Ctrl Pts',(-20.098611386588,17.8138174329915,124.411232739304)) ;
#82077=CARTESIAN_POINT('Ctrl Pts',(-19.8472361889034,17.8271561406856,124.5354219874)) ;
#82078=CARTESIAN_POINT('Ctrl Pts',(-19.6486955377895,17.8369985149939,124.59379753129)) ;
#82079=CARTESIAN_POINT('Ctrl Pts',(-19.4386609397151,17.8470535349766,124.617501312887)) ;
#82080=CARTESIAN_POINT('Ctrl Pts',(-19.1610336754665,17.8602856916342,124.600234915123)) ;
#82081=CARTESIAN_POINT('Ctrl Pts',(-18.8258947387444,17.8769006589793,124.488350086626)) ;
#82082=CARTESIAN_POINT('Ctrl Pts',(-18.5495768294908,17.8934952459905,124.269022287686)) ;
#82083=CARTESIAN_POINT('Ctrl Pts',(-18.3833597966674,17.9067288143459,124.045859206005)) ;
#82084=CARTESIAN_POINT('Ctrl Pts',(-18.2885301550365,17.9167724321545,123.857229906636)) ;
#82085=CARTESIAN_POINT('Ctrl Pts',(-18.2287562614033,17.9266593563894,123.658135422975)) ;
#82086=CARTESIAN_POINT('Ctrl Pts',(-18.2038373016727,17.9366500108362,123.449600406301)) ;
#82087=CARTESIAN_POINT('Ctrl Pts',(-18.2155183704076,17.9466117692902,123.240489064376)) ;
#82088=CARTESIAN_POINT('Ctrl Pts',(-18.2792425265462,17.9599516343574,122.96736967854)) ;
#82089=CARTESIAN_POINT('Ctrl Pts',(-18.4130348686305,17.9732604172707,122.718034036451)) ;
#82090=CARTESIAN_POINT('Ctrl Pts',(-18.6026066029756,17.9864561747147,122.515468776243)) ;
#82091=CARTESIAN_POINT('Ctrl Pts',(-18.7697372859476,17.9964180583912,122.389261077873)) ;
#82092=CARTESIAN_POINT('Ctrl Pts',(-18.9579188488401,18.0064611679059,122.293522046831)) ;
#82093=CARTESIAN_POINT('Ctrl Pts',(-19.1559639974618,18.0163134179051,122.232844543332)) ;
#82094=CARTESIAN_POINT('Ctrl Pts',(-19.3639322401646,18.0262849548556,122.206660737817)) ;
#82095=CARTESIAN_POINT('Ctrl Pts',(-19.573840915156,18.0362802203331,122.217029724111)) ;
#82096=CARTESIAN_POINT('Ctrl Pts',(-19.779447227666,18.0463141932067,122.264110388096)) ;
#82097=CARTESIAN_POINT('Ctrl Pts',(-19.9704605148367,18.0561696079691,122.34442663518)) ;
#82098=CARTESIAN_POINT('Ctrl Pts',(-20.1472770470841,18.0661688854779,122.458056104505)) ;
#82099=CARTESIAN_POINT('Ctrl Pts',(-20.3002748716103,18.0760640696409,122.599059938975)) ;
#82100=CARTESIAN_POINT('Ctrl Pts',(-20.4285143260641,18.0861244492817,122.767212166188)) ;
#82101=CARTESIAN_POINT('Ctrl Pts',(-20.5237126864081,18.0959743182898,122.951130297099)) ;
#82102=CARTESIAN_POINT('Ctrl Pts',(-20.5871207089532,18.1060058794977,123.152253484728)) ;
#82103=CARTESIAN_POINT('Ctrl Pts',(-20.6141694641062,18.11601632838,123.360978666179)) ;
#82104=CARTESIAN_POINT('Ctrl Pts',(-20.604896382514,18.125923067797,123.569036040792)) ;
#82105=CARTESIAN_POINT('Ctrl Pts',(-20.5598938047864,18.1358610838654,123.773047836236)) ;
#82106=CARTESIAN_POINT('Ctrl Pts',(-20.4797271671721,18.1458663303166,123.967538007628)) ;
#82107=CARTESIAN_POINT('Ctrl Pts',(-20.366397809523,18.1559003913728,124.145444996922)) ;
#82108=CARTESIAN_POINT('Ctrl Pts',(-20.2268317398703,18.165745472431,124.298300989317)) ;
#82109=CARTESIAN_POINT('Ctrl Pts',(-20.060776723632,18.1757312783845,124.426689933067)) ;
#82110=CARTESIAN_POINT('Ctrl Pts',(-19.8759066270791,18.1856660989387,124.523963672816)) ;
#82111=CARTESIAN_POINT('Ctrl Pts',(-19.6745058024379,18.1957236240709,124.588245907448)) ;
#82112=CARTESIAN_POINT('Ctrl Pts',(-19.4699075166441,18.2055452747222,124.616238143895)) ;
#82113=CARTESIAN_POINT('Ctrl Pts',(-19.2586565390616,18.215601338227,124.608486330295)) ;
#82114=CARTESIAN_POINT('Ctrl Pts',(-19.0543868823573,18.2255420052909,124.564306968047)) ;
#82115=CARTESIAN_POINT('Ctrl Pts',(-18.8613551751565,18.2354463989569,124.486226473999)) ;
#82116=CARTESIAN_POINT('Ctrl Pts',(-18.6823712516307,18.2454929227199,124.374127325452)) ;
#82117=CARTESIAN_POINT('Ctrl Pts',(-18.5277423264652,18.2553890057363,124.234883369432)) ;
#82118=CARTESIAN_POINT('Ctrl Pts',(-18.3975181426355,18.2654557049663,124.068106618512)) ;
#82119=CARTESIAN_POINT('Ctrl Pts',(-18.3003841373162,18.2752793153674,123.885816193792)) ;
#82120=CARTESIAN_POINT('Ctrl Pts',(-18.2345287994309,18.2853351755449,123.68495762991)) ;
#82121=CARTESIAN_POINT('Ctrl Pts',(-18.2051746041223,18.2952683218498,123.478179409818)) ;
#82122=CARTESIAN_POINT('Ctrl Pts',(-18.2117492807388,18.3052135776204,123.269226631086)) ;
#82123=CARTESIAN_POINT('Ctrl Pts',(-18.2545138769522,18.3151968760589,123.063722386448)) ;
#82124=CARTESIAN_POINT('Ctrl Pts',(-18.3329825492014,18.3252340562055,122.867858860331)) ;
#82125=CARTESIAN_POINT('Ctrl Pts',(-18.4419876978032,18.335088608915,122.69165785752)) ;
#82126=CARTESIAN_POINT('Ctrl Pts',(-18.5817046998285,18.3450881273623,122.534632662835)) ;
#82127=CARTESIAN_POINT('Ctrl Pts',(-18.7447605670421,18.3549832098244,122.405396558866)) ;
#82128=CARTESIAN_POINT('Ctrl Pts',(-18.9307947270975,18.3650437553305,122.304828639192)) ;
#82129=CARTESIAN_POINT('Ctrl Pts',(-19.1272549383344,18.3748930625785,122.239367983502)) ;
#82130=CARTESIAN_POINT('Ctrl Pts',(-19.335695185128,18.3849201526658,122.207938380251)) ;
#82131=CARTESIAN_POINT('Ctrl Pts',(-19.5464637126567,18.3949490568028,122.213739548366)) ;
#82132=CARTESIAN_POINT('Ctrl Pts',(-19.7492771311671,18.4047929219021,122.254862772888)) ;
#82133=CARTESIAN_POINT('Ctrl Pts',(-19.9450396765661,18.4147887486105,122.331265523239)) ;
#82134=CARTESIAN_POINT('Ctrl Pts',(-20.1248922159333,18.4248139652595,122.441153309289)) ;
#82135=CARTESIAN_POINT('Ctrl Pts',(-20.2809828268305,18.4347037974171,122.578506486257)) ;
#82136=CARTESIAN_POINT('Ctrl Pts',(-20.4123979974566,18.4446946535018,122.742346656916)) ;
#82137=CARTESIAN_POINT('Ctrl Pts',(-20.512875040643,18.4546397480947,122.925697224082)) ;
#82138=CARTESIAN_POINT('Ctrl Pts',(-20.5804101851488,18.4645916518628,123.123726283587)) ;
#82139=CARTESIAN_POINT('Ctrl Pts',(-20.612623320595,18.4746280513322,123.332244177723)) ;
#82140=CARTESIAN_POINT('Ctrl Pts',(-20.608359655852,18.4845171214209,123.540106555575)) ;
#82141=CARTESIAN_POINT('Ctrl Pts',(-20.5680335601972,18.4945064107918,123.746199638526)) ;
#82142=CARTESIAN_POINT('Ctrl Pts',(-20.4926226085068,18.5044649770015,123.941500179011)) ;
#82143=CARTESIAN_POINT('Ctrl Pts',(-20.3855172625548,18.5143645482183,124.119959380232)) ;
#82144=CARTESIAN_POINT('Ctrl Pts',(-20.2469737641147,18.5244124626325,124.279390783866)) ;
#82145=CARTESIAN_POINT('Ctrl Pts',(-20.0854054590516,18.5343078054931,124.410487000382)) ;
#82146=CARTESIAN_POINT('Ctrl Pts',(-19.9005352475718,18.5443694994405,124.513234875)) ;
#82147=CARTESIAN_POINT('Ctrl Pts',(-19.7049300850852,18.5542139525247,124.580875665388)) ;
#82148=CARTESIAN_POINT('Ctrl Pts',(-19.498273946928,18.5641746374831,124.614633531059)) ;
#82149=CARTESIAN_POINT('Ctrl Pts',(-19.2873015921753,18.5742105699917,124.611621178761)) ;
#82150=CARTESIAN_POINT('Ctrl Pts',(-19.0830712792715,18.5840991856797,124.572810355091)) ;
#82151=CARTESIAN_POINT('Ctrl Pts',(-18.8860431848826,18.5941135948222,124.498576084643)) ;
#82152=CARTESIAN_POINT('Ctrl Pts',(-18.7048498408381,18.60414740378,124.390593284749)) ;
#82153=CARTESIAN_POINT('Ctrl Pts',(-18.5479907947063,18.6139778580362,124.255995839856)) ;
#82154=CARTESIAN_POINT('Ctrl Pts',(-18.4135763365836,18.6240555256144,124.092282621306)) ;
#82155=CARTESIAN_POINT('Ctrl Pts',(-18.3118234906073,18.6339073937366,123.911832218199)) ;
#82156=CARTESIAN_POINT('Ctrl Pts',(-18.2412636801989,18.643980431302,123.712204324392)) ;
#82157=CARTESIAN_POINT('Ctrl Pts',(-18.2072562008697,18.6538229846528,123.508079026734)) ;
#82158=CARTESIAN_POINT('Ctrl Pts',(-18.2085295969781,18.6638033801463,123.298272657034)) ;
#82159=CARTESIAN_POINT('Ctrl Pts',(-18.2467612461067,18.6738218581241,123.091156421006)) ;
#82160=CARTESIAN_POINT('Ctrl Pts',(-18.3189753825504,18.6837051724301,122.896304492424)) ;
#82161=CARTESIAN_POINT('Ctrl Pts',(-18.4259403191284,18.6937734749689,122.713693094242)) ;
#82162=CARTESIAN_POINT('Ctrl Pts',(-18.559602694153,18.7036035222423,122.556032920979)) ;
#82163=CARTESIAN_POINT('Ctrl Pts',(-18.7222140012075,18.7136703936578,122.420633660617)) ;
#82164=CARTESIAN_POINT('Ctrl Pts',(-18.902732128757,18.7235594324569,122.317446999546)) ;
#82165=CARTESIAN_POINT('Ctrl Pts',(-19.1003669108627,18.733556130591,122.246036925525)) ;
#82166=CARTESIAN_POINT('Ctrl Pts',(-19.3065324036651,18.7435085563029,122.210267846884)) ;
#82167=CARTESIAN_POINT('Ctrl Pts',(-19.515513806108,18.7534498585359,122.210548414054)) ;
#82168=CARTESIAN_POINT('Ctrl Pts',(-19.7222190007818,18.7634330976198,122.247050242627)) ;
#82169=CARTESIAN_POINT('Ctrl Pts',(-19.9203917966261,18.7734718991884,122.319582333041)) ;
#82170=CARTESIAN_POINT('Ctrl Pts',(-20.0997259540497,18.78332000531,122.423079562139)) ;
#82171=CARTESIAN_POINT('Ctrl Pts',(-20.2618814355052,18.7933802008854,122.558833866396)) ;
#82172=CARTESIAN_POINT('Ctrl Pts',(-20.3956744733974,18.8032778841968,122.718208717392)) ;
#82173=CARTESIAN_POINT('Ctrl Pts',(-20.500699852914,18.8132089245708,122.898646703033)) ;
#82174=CARTESIAN_POINT('Ctrl Pts',(-20.5733935792951,18.8232511422274,123.096852695664)) ;
#82175=CARTESIAN_POINT('Ctrl Pts',(-20.6101416824105,18.8331378029614,123.301436586852)) ;
#82176=CARTESIAN_POINT('Ctrl Pts',(-20.6111685252256,18.8431309115638,123.511509895884)) ;
#82177=CARTESIAN_POINT('Ctrl Pts',(-20.5757926368399,18.8530766102021,123.717585377804)) ;
#82178=CARTESIAN_POINT('Ctrl Pts',(-20.5055613870211,18.8630238324731,123.914572351637)) ;
#82179=CARTESIAN_POINT('Ctrl Pts',(-20.4009471133785,18.8730718580533,124.098082373486)) ;
#82180=CARTESIAN_POINT('Ctrl Pts',(-20.2688858623514,18.8829191051962,124.257508865836)) ;
#82181=CARTESIAN_POINT('Ctrl Pts',(-20.1097243653322,18.8928822822869,124.393663555677)) ;
#82182=CARTESIAN_POINT('Ctrl Pts',(-19.9279708858338,18.9029120033203,124.500552461279)) ;
#82183=CARTESIAN_POINT('Ctrl Pts',(-19.7329558262972,18.9128164708532,124.573584982313)) ;
#82184=CARTESIAN_POINT('Ctrl Pts',(-19.5257968131938,18.922840956683,124.612170961109)) ;
#82185=CARTESIAN_POINT('Ctrl Pts',(-19.3175695516905,18.9327447918069,124.614349948157)) ;
#82186=CARTESIAN_POINT('Ctrl Pts',(-19.1091146460019,18.9427959825169,124.579889389743)) ;
#82187=CARTESIAN_POINT('Ctrl Pts',(-18.9130619745761,18.9526804251752,124.510943593051)) ;
#82188=CARTESIAN_POINT('Ctrl Pts',(-18.729812387142,18.962673433027,124.408243899049)) ;
#82189=CARTESIAN_POINT('Ctrl Pts',(-18.5679260209722,18.9726217527433,124.275805077291)) ;
#82190=CARTESIAN_POINT('Ctrl Pts',(-18.43144613634,18.9825585914528,124.117671370071)) ;
#82191=CARTESIAN_POINT('Ctrl Pts',(-18.3237491330142,18.9925415803724,123.937505527869)) ;
#82192=CARTESIAN_POINT('Ctrl Pts',(-18.2488966397258,19.0025854597365,123.74009037589)) ;
#82193=CARTESIAN_POINT('Ctrl Pts',(-18.209813065763,19.0124135250949,123.537170735293)) ;
#82194=CARTESIAN_POINT('Ctrl Pts',(-18.2063851574917,19.0224906136498,123.325393194983)) ;
#82195=CARTESIAN_POINT('Ctrl Pts',(-18.2389095766539,19.0323407658061,123.120827998228)) ;
#82196=CARTESIAN_POINT('Ctrl Pts',(-18.3079229039894,19.0424212462584,122.920512664248)) ;
#82197=CARTESIAN_POINT('Ctrl Pts',(-18.4078474700848,19.0522357440273,122.739938974569)) ;
#82198=CARTESIAN_POINT('Ctrl Pts',(-18.5406432867953,19.0623040400474,122.575174067644)) ;
#82199=CARTESIAN_POINT('Ctrl Pts',(-18.6974620235744,19.0722028725302,122.438290128418)) ;
#82200=CARTESIAN_POINT('Ctrl Pts',(-18.8783200381135,19.0822557525447,122.329027971715)) ;
#82201=CARTESIAN_POINT('Ctrl Pts',(-19.0718217296824,19.0921255680409,122.254003566536)) ;
#82202=CARTESIAN_POINT('Ctrl Pts',(-19.2795065095552,19.1021982491237,122.212846725004)) ;
#82203=CARTESIAN_POINT('Ctrl Pts',(-19.486188422999,19.1120307276946,122.208399680051)) ;
#82204=CARTESIAN_POINT('Ctrl Pts',(-19.6946842168501,19.1220613616807,122.239936675267)) ;
#82205=CARTESIAN_POINT('Ctrl Pts',(-19.8943771096132,19.1320929188999,122.307793559759)) ;
#82206=CARTESIAN_POINT('Ctrl Pts',(-20.0757189797169,19.1419226277716,122.406859095438)) ;
#82207=CARTESIAN_POINT('Ctrl Pts',(-20.2401349998331,19.1519120765737,122.537526739617)) ;
#82208=CARTESIAN_POINT('Ctrl Pts',(-20.3797167257988,19.1619559289737,122.695962343136)) ;
#82209=CARTESIAN_POINT('Ctrl Pts',(-20.4876019773481,19.1717776423058,122.872018751571)) ;
#82210=CARTESIAN_POINT('Ctrl Pts',(-20.5654043920265,19.1818126472945,123.068115049024)) ;
#82211=CARTESIAN_POINT('Ctrl Pts',(-20.6073616916099,19.1918374857421,123.274657345158)) ;
#82212=CARTESIAN_POINT('Ctrl Pts',(-20.6131682474204,19.2016896986973,123.48170036684)) ;
#82213=CARTESIAN_POINT('Ctrl Pts',(-20.5828695009904,19.2116796548911,123.689507417309)) ;
#82214=CARTESIAN_POINT('Ctrl Pts',(-20.5173663448206,19.2216077651743,123.887689668796)) ;
#82215=CARTESIAN_POINT('Ctrl Pts',(-20.418139793369,19.2315963652539,124.072765163294)) ;
#82216=CARTESIAN_POINT('Ctrl Pts',(-20.2875636494693,19.2416229571814,124.238246501146)) ;
#82217=CARTESIAN_POINT('Ctrl Pts',(-20.1326099243232,19.2515080852456,124.376719379815)) ;
#82218=CARTESIAN_POINT('Ctrl Pts',(-19.9543134180587,19.2614992027191,124.487770824645)) ;
#82219=CARTESIAN_POINT('Ctrl Pts',(-19.7583197917987,19.2715398185709,124.566149257661)) ;
#82220=CARTESIAN_POINT('Ctrl Pts',(-19.5560396568112,19.2813728094246,124.608747665679)) ;
#82221=CARTESIAN_POINT('Ctrl Pts',(-19.3460913751893,19.2913659408749,124.616289970547)) ;
#82222=CARTESIAN_POINT('Ctrl Pts',(-19.1372600744288,19.3013979893103,124.586714092898)) ;
#82223=CARTESIAN_POINT('Ctrl Pts',(-18.9400108934153,19.3112632358527,124.522664185443)) ;
#82224=CARTESIAN_POINT('Ctrl Pts',(-18.7547919716297,19.3212251106795,124.42490173768)) ;
#82225=CARTESIAN_POINT('Ctrl Pts',(-18.5883738308643,19.3312600737908,124.295260107016)) ;
#82226=CARTESIAN_POINT('Ctrl Pts',(-18.4488190485599,19.3411449182532,124.141239793615)) ;
#82227=CARTESIAN_POINT('Ctrl Pts',(-18.3361799509214,19.3512109710939,123.962131077529)) ;
#82228=CARTESIAN_POINT('Ctrl Pts',(-18.2579205679467,19.3610484870029,123.770652745803)) ;
#82229=CARTESIAN_POINT('Ctrl Pts',(-18.2128628982536,19.3711172351118,123.563864379788)) ;
#82230=CARTESIAN_POINT('Ctrl Pts',(-18.2046274737914,19.3809977521428,123.356276336326)) ;
#82231=CARTESIAN_POINT('Ctrl Pts',(-18.2324438381508,19.3909889390772,123.148111150481)) ;
#82232=CARTESIAN_POINT('Ctrl Pts',(-18.295726868169,19.4009420053522,122.948631988173)) ;
#82233=CARTESIAN_POINT('Ctrl Pts',(-18.3935294192508,19.4109778428848,122.7617040229)) ;
#82234=CARTESIAN_POINT('Ctrl Pts',(-18.52033969625,19.4208679690962,122.596912733029)) ;
#82235=CARTESIAN_POINT('Ctrl Pts',(-18.6751751290804,19.4308601510042,122.454963151658)) ;
#82236=CARTESIAN_POINT('Ctrl Pts',(-18.8515331266452,19.4408060909428,122.342630531984)) ;
#82237=CARTESIAN_POINT('Ctrl Pts',(-19.0445885211167,19.4507532747068,122.262219660309)) ;
#82238=CARTESIAN_POINT('Ctrl Pts',(-19.2507744026111,19.4608012130143,122.216323259587)) ;
#82239=CARTESIAN_POINT('Ctrl Pts',(-19.4575916167922,19.4706488477546,122.206936574078)) ;
#82240=CARTESIAN_POINT('Ctrl Pts',(-19.665347647943,19.4806105617284,122.233259207866)) ;
#82241=CARTESIAN_POINT('Ctrl Pts',(-19.8666638852989,19.4906391965192,122.295933848434)) ;
#82242=CARTESIAN_POINT('Ctrl Pts',(-20.0518399911396,19.5005495151164,122.391400478421)) ;
#82243=CARTESIAN_POINT('Ctrl Pts',(-20.2183835123299,19.5104843714279,122.517455349615)) ;
#82244=CARTESIAN_POINT('Ctrl Pts',(-20.3618707138859,19.5205256073886,122.672277289521)) ;
#82245=CARTESIAN_POINT('Ctrl Pts',(-20.4746969570894,19.5304123789686,122.846864648244)) ;
#82246=CARTESIAN_POINT('Ctrl Pts',(-20.5566359414748,19.5404125576748,123.040441264708)) ;
#82247=CARTESIAN_POINT('Ctrl Pts',(-20.6035192091407,19.5503298358844,123.243629797779)) ;
#82248=CARTESIAN_POINT('Ctrl Pts',(-20.6144848722906,19.560377082298,123.454540489081)) ;
#82249=CARTESIAN_POINT('Ctrl Pts',(-20.5893212879762,19.5702509712793,123.660622657951)) ;
#82250=CARTESIAN_POINT('Ctrl Pts',(-20.5277315386694,19.5803129888599,123.862966123418)) ;
#82251=CARTESIAN_POINT('Ctrl Pts',(-20.4337174008764,19.5901840505942,124.047986023597)) ;
#82252=CARTESIAN_POINT('Ctrl Pts',(-20.3079299585367,19.6001781139545,124.216278196079)) ;
#82253=CARTESIAN_POINT('Ctrl Pts',(-20.1539324806393,19.6102102719879,124.36037634443)) ;
#82254=CARTESIAN_POINT('Ctrl Pts',(-19.9804428606357,19.620074148228,124.474010290571)) ;
#82255=CARTESIAN_POINT('Ctrl Pts',(-19.7859181324196,19.6301446628663,124.557511621058)) ;
#82256=CARTESIAN_POINT('Ctrl Pts',(-19.5845187702975,19.6399852998073,124.604891310649)) ;
#82257=CARTESIAN_POINT('Ctrl Pts',(-19.3753708163134,19.6499524286475,124.617420938823)) ;
#82258=CARTESIAN_POINT('Ctrl Pts',(-19.1662428926851,19.659966401772,124.593109655886)) ;
#82259=CARTESIAN_POINT('Ctrl Pts',(-18.8985886193499,19.6732511356353,124.513253218145)) ;
#82260=CARTESIAN_POINT('Ctrl Pts',(-18.6588872460886,19.68647640035,124.36624963569)) ;
#82261=CARTESIAN_POINT('Ctrl Pts',(-18.4660700314843,19.6997869229049,124.163476334807)) ;
#82262=CARTESIAN_POINT('Ctrl Pts',(-18.3496595586421,19.7098155678071,123.987691638222)) ;
#82263=CARTESIAN_POINT('Ctrl Pts',(-18.2666103147507,19.719696600161,123.797282030804)) ;
#82264=CARTESIAN_POINT('Ctrl Pts',(-18.2169671329577,19.7296775728411,123.593407967415)) ;
#82265=CARTESIAN_POINT('Ctrl Pts',(-18.2036560520165,19.7396587004271,123.384012355789)) ;
#82266=CARTESIAN_POINT('Ctrl Pts',(-18.2339327364672,19.7529018906885,123.107170942939)) ;
#82267=CARTESIAN_POINT('Ctrl Pts',(-18.3623905339946,19.7695698860493,122.776996583947)) ;
#82268=CARTESIAN_POINT('Ctrl Pts',(-18.5937075192732,19.7860903860613,122.512484152482)) ;
#82269=CARTESIAN_POINT('Ctrl Pts',(-18.8258990467803,19.7994034023773,122.356364032903)) ;
#82270=CARTESIAN_POINT('Ctrl Pts',(-19.0164084560592,19.8093199606103,122.271584830569)) ;
#82271=CARTESIAN_POINT('Ctrl Pts',(-19.2209351105263,19.8193476289132,122.220706890432)) ;
#82272=CARTESIAN_POINT('Ctrl Pts',(-19.4974375044467,19.8325282186578,122.200845480391)) ;
#82273=CARTESIAN_POINT('Ctrl Pts',(-19.8469032671938,19.8492763577772,122.268339890241)) ;
#82274=CARTESIAN_POINT('Ctrl Pts',(-20.2084084237355,19.8690711002878,122.484283560404)) ;
#82275=CARTESIAN_POINT('Ctrl Pts',(-20.4779908187138,19.8891154930966,122.814197860746)) ;
#82276=CARTESIAN_POINT('Ctrl Pts',(-20.6171058432914,19.9089546753953,123.212554236894)) ;
#82277=CARTESIAN_POINT('Ctrl Pts',(-20.6129557723522,19.9288799990882,123.636097670843)) ;
#82278=CARTESIAN_POINT('Ctrl Pts',(-20.464422658849,19.9488036371397,124.032909206255)) ;
#82279=CARTESIAN_POINT('Ctrl Pts',(-20.18955447349,19.9687285106052,124.355231228581)) ;
#82280=CARTESIAN_POINT('Ctrl Pts',(-19.8222578423576,19.9886071176841,124.564437264234)) ;
#82281=CARTESIAN_POINT('Ctrl Pts',(-19.403615042977,20.0085845605161,124.636299305193)) ;
#82282=CARTESIAN_POINT('Ctrl Pts',(-18.9865389485054,20.0285164086008,124.560857289686)) ;
#82283=CARTESIAN_POINT('Ctrl Pts',(-18.6207630528678,20.0484116769434,124.348399240722)) ;
#82284=CARTESIAN_POINT('Ctrl Pts',(-18.3486870871748,20.0683341753555,124.023705533677)) ;
#82285=CARTESIAN_POINT('Ctrl Pts',(-18.203574404514,20.0882936572315,123.624866923908)) ;
#82286=CARTESIAN_POINT('Ctrl Pts',(-18.2031996447165,20.1081714096908,123.202277453472)) ;
#82287=CARTESIAN_POINT('Ctrl Pts',(-18.346002051333,20.1280532004254,122.804297838567)) ;
#82288=CARTESIAN_POINT('Ctrl Pts',(-18.6192053764453,20.1481265392764,122.476459381856)) ;
#82289=CARTESIAN_POINT('Ctrl Pts',(-18.98301587099,20.1679310065122,122.264237767861)) ;
#82290=CARTESIAN_POINT('Ctrl Pts',(-19.4008364759886,20.18791434692,122.18732233124)) ;
#82291=CARTESIAN_POINT('Ctrl Pts',(-19.8183361021273,20.207829311518,122.258043575574)) ;
#82292=CARTESIAN_POINT('Ctrl Pts',(-20.1864344857312,20.2276978462343,122.465512799918)) ;
#82293=CARTESIAN_POINT('Ctrl Pts',(-20.4635252494409,20.2477502304461,122.789401507206)) ;
#82294=CARTESIAN_POINT('Ctrl Pts',(-20.6120084813329,20.2675241942353,123.182939564041)) ;
#82295=CARTESIAN_POINT('Ctrl Pts',(-20.6176872102052,20.2875785732566,123.609141239229)) ;
#82296=CARTESIAN_POINT('Ctrl Pts',(-20.4791319362288,20.3073753108299,124.00674845248)) ;
#82297=CARTESIAN_POINT('Ctrl Pts',(-20.2119684125399,20.3273431231813,124.336599903747)) ;
#82298=CARTESIAN_POINT('Ctrl Pts',(-19.8479480817942,20.3473020992464,124.554908135789)) ;
#82299=CARTESIAN_POINT('Ctrl Pts',(-19.4327659312794,20.3671970175238,124.635876929889)) ;
#82300=CARTESIAN_POINT('Ctrl Pts',(-19.0147876905116,20.3870933299741,124.570821089718)) ;
#82301=CARTESIAN_POINT('Ctrl Pts',(-18.6435959691219,20.4070012633482,124.367296800333)) ;
#82302=CARTESIAN_POINT('Ctrl Pts',(-18.3636276837222,20.4269511536367,124.048670511752)) ;
#82303=CARTESIAN_POINT('Ctrl Pts',(-18.2093280562878,20.446828384138,123.655155581433)) ;
#82304=CARTESIAN_POINT('Ctrl Pts',(-18.198304793453,20.466811053009,123.230434093372)) ;
#82305=CARTESIAN_POINT('Ctrl Pts',(-18.3328373858692,20.4867439395894,122.828470917943)) ;
#82306=CARTESIAN_POINT('Ctrl Pts',(-18.5959298066078,20.5066566856073,122.496768356092)) ;
#82307=CARTESIAN_POINT('Ctrl Pts',(-18.895676555151,20.5232264069491,122.311681507848)) ;
#82308=CARTESIAN_POINT('Ctrl Pts',(-19.1634853018324,20.5365264182541,122.231185644961)) ;
#82309=CARTESIAN_POINT('Ctrl Pts',(-19.4404546522305,20.549796606004,122.198099948954)) ;
#82310=CARTESIAN_POINT('Ctrl Pts',(-19.7904975982779,20.5664239883694,122.248239271014)) ;
#82311=CARTESIAN_POINT('Ctrl Pts',(-20.1021496586214,20.5830462781146,122.414851991892)) ;
#82312=CARTESIAN_POINT('Ctrl Pts',(-20.305538571328,20.5962914925091,122.60507349097)) ;
#82313=CARTESIAN_POINT('Ctrl Pts',(-20.4311937815454,20.6062034574698,122.77131708526)) ;
#82314=CARTESIAN_POINT('Ctrl Pts',(-20.5272486919017,20.6162620806342,122.959681415796)) ;
#82315=CARTESIAN_POINT('Ctrl Pts',(-20.5881005962991,20.62610219475,123.157431298094)) ;
#82316=CARTESIAN_POINT('Ctrl Pts',(-20.6144821793486,20.6361679797077,123.367363458734)) ;
#82317=CARTESIAN_POINT('Ctrl Pts',(-20.6041090188649,20.6460512974956,123.574910030849)) ;
#82318=CARTESIAN_POINT('Ctrl Pts',(-20.5578169159025,20.6560407353541,123.779732824598)) ;
#82319=CARTESIAN_POINT('Ctrl Pts',(-20.4767917351146,20.6660044494069,123.972907172998)) ;
#82320=CARTESIAN_POINT('Ctrl Pts',(-20.363282775576,20.6759994610661,124.149756048535)) ;
#82321=CARTESIAN_POINT('Ctrl Pts',(-20.2199777436041,20.6860357527603,124.304604665341)) ;
#82322=CARTESIAN_POINT('Ctrl Pts',(-20.0553288276782,20.6958821304538,124.430086219133)) ;
#82323=CARTESIAN_POINT('Ctrl Pts',(-19.8690272051789,20.7058670746045,124.526746885253)) ;
#82324=CARTESIAN_POINT('Ctrl Pts',(-19.6697103598208,20.7158040457344,124.589424857213)) ;
#82325=CARTESIAN_POINT('Ctrl Pts',(-19.4602253401753,20.7258538303662,124.616732469471)) ;
#82326=CARTESIAN_POINT('Ctrl Pts',(-19.253324082945,20.7357042924436,124.607595743279)) ;
#82327=CARTESIAN_POINT('Ctrl Pts',(-19.0485802151792,20.7456763059641,124.562661428666)) ;
#82328=CARTESIAN_POINT('Ctrl Pts',(-18.8542534350798,20.7556714530835,124.482625689863)) ;
#82329=CARTESIAN_POINT('Ctrl Pts',(-18.6762666846949,20.7657054228196,124.36943917364)) ;
#82330=CARTESIAN_POINT('Ctrl Pts',(-18.5231567953254,20.7755609684902,124.229814819193)) ;
#82331=CARTESIAN_POINT('Ctrl Pts',(-18.394575811181,20.7855597255034,124.063565093148)) ;
#82332=CARTESIAN_POINT('Ctrl Pts',(-18.2976014743614,20.7954568607406,123.87944119294)) ;
#82333=CARTESIAN_POINT('Ctrl Pts',(-18.2330490484476,20.8055099565802,123.678215684589)) ;
#82334=CARTESIAN_POINT('Ctrl Pts',(-18.2048744104078,20.8153934653108,123.472337923428)) ;
#82335=CARTESIAN_POINT('Ctrl Pts',(-18.2124727925747,20.8253883379569,123.262357979921)) ;
#82336=CARTESIAN_POINT('Ctrl Pts',(-18.2568500096631,20.8354082995926,123.056422212533)) ;
#82337=CARTESIAN_POINT('Ctrl Pts',(-18.3352337461589,20.8453136633924,122.863498944733)) ;
#82338=CARTESIAN_POINT('Ctrl Pts',(-18.4459506865734,20.855254251,122.686271481203)) ;
#82339=CARTESIAN_POINT('Ctrl Pts',(-18.5865697971061,20.8652570691006,122.529879035352)) ;
#82340=CARTESIAN_POINT('Ctrl Pts',(-18.7529194184332,20.8752917808248,122.400158067132)) ;
#82341=CARTESIAN_POINT('Ctrl Pts',(-18.9355983712862,20.8851366875621,122.302840177009)) ;
#82342=CARTESIAN_POINT('Ctrl Pts',(-19.1350505907235,20.8951225401311,122.237440608609)) ;
#82343=CARTESIAN_POINT('Ctrl Pts',(-19.3418166620123,20.9050573485441,122.20766040024)) ;
#82344=CARTESIAN_POINT('Ctrl Pts',(-19.5531166794157,20.9151148756252,122.214501576206)) ;
#82345=CARTESIAN_POINT('Ctrl Pts',(-19.755282382907,20.9249365306223,122.256609777774)) ;
#82346=CARTESIAN_POINT('Ctrl Pts',(-19.9517518328601,20.9349925747953,122.334626535932)) ;
#82347=CARTESIAN_POINT('Ctrl Pts',(-20.1294511445661,20.9449333148405,122.444634048167)) ;
#82348=CARTESIAN_POINT('Ctrl Pts',(-20.2852058392503,20.9548374359133,122.582819935686)) ;
#82349=CARTESIAN_POINT('Ctrl Pts',(-20.4163627073902,20.9648849770676,122.748380027201)) ;
#82350=CARTESIAN_POINT('Ctrl Pts',(-20.5154483160002,20.974783728668,122.931410768418)) ;
#82351=CARTESIAN_POINT('Ctrl Pts',(-20.5823152000268,20.9848322076338,123.131775211427)) ;
#82352=CARTESIAN_POINT('Ctrl Pts',(-20.6129012298034,20.9947197047175,123.337400837279)) ;
#82353=CARTESIAN_POINT('Ctrl Pts',(-20.6076505386233,21.0047127950156,123.547403033291)) ;
#82354=CARTESIAN_POINT('Ctrl Pts',(-20.5661097269182,21.0146649650759,123.752476419101)) ;
#82355=CARTESIAN_POINT('Ctrl Pts',(-20.489974800567,21.0246033849904,123.947032286064)) ;
#82356=CARTESIAN_POINT('Ctrl Pts',(-20.3808873584294,21.034588515076,124.126405174509)) ;
#82357=CARTESIAN_POINT('Ctrl Pts',(-20.2413837740045,21.0446252044901,124.284693816363)) ;
#82358=CARTESIAN_POINT('Ctrl Pts',(-20.0796866049328,21.0544798884826,124.414245633382)) ;
#82359=CARTESIAN_POINT('Ctrl Pts',(-19.8954680695033,21.0644793725304,124.515444105572)) ;
#82360=CARTESIAN_POINT('Ctrl Pts',(-19.6985589416017,21.0743744613073,124.582645268236)) ;
#82361=CARTESIAN_POINT('Ctrl Pts',(-19.4895929842184,21.0844350159535,124.615139996336)) ;
#82362=CARTESIAN_POINT('Ctrl Pts',(-19.2825548193412,21.0942842803264,124.611063574309)) ;
#82363=CARTESIAN_POINT('Ctrl Pts',(-19.0756156897001,21.1043115327742,124.570906278873)) ;
#82364=CARTESIAN_POINT('Ctrl Pts',(-18.8789572087526,21.1143398303444,124.494897176349)) ;
#82365=CARTESIAN_POINT('Ctrl Pts',(-18.7015724696845,21.1241859593504,124.388226917804)) ;
#82366=CARTESIAN_POINT('Ctrl Pts',(-18.5427085112095,21.1341798647124,124.250730179564)) ;
#82367=CARTESIAN_POINT('Ctrl Pts',(-18.4100202913512,21.1442039623955,124.0870024506)) ;
#82368=CARTESIAN_POINT('Ctrl Pts',(-18.3089182683856,21.1540937902495,123.905319990407)) ;
#82369=CARTESIAN_POINT('Ctrl Pts',(-18.2399098881066,21.1640857716799,123.706924554748)) ;
#82370=CARTESIAN_POINT('Ctrl Pts',(-18.2065962274029,21.1740327764458,123.500477641717)) ;
#82371=CARTESIAN_POINT('Ctrl Pts',(-18.2092510439381,21.1839824278356,123.291312971923)) ;
#82372=CARTESIAN_POINT('Ctrl Pts',(-18.2486917570198,21.194019430813,123.084028422543)) ;
#82373=CARTESIAN_POINT('Ctrl Pts',(-18.3222881608881,21.203908339248,122.889587468432)) ;
#82374=CARTESIAN_POINT('Ctrl Pts',(-18.429273753743,21.2138976717255,122.708880714178)) ;
#82375=CARTESIAN_POINT('Ctrl Pts',(-18.5657078725449,21.2238562271626,122.550089089031)) ;
#82376=CARTESIAN_POINT('Ctrl Pts',(-18.7263705845267,21.2337557983631,122.417776071601)) ;
#82377=CARTESIAN_POINT('Ctrl Pts',(-18.9102889857896,21.2438037236151,122.313916744243)) ;
#82378=CARTESIAN_POINT('Ctrl Pts',(-19.1064181843842,21.2536990231411,122.244464755994)) ;
#82379=CARTESIAN_POINT('Ctrl Pts',(-19.3150200723039,21.263760879589,122.209527188093)) ;
#82380=CARTESIAN_POINT('Ctrl Pts',(-19.5219709540585,21.2736047260057,122.21125922334)) ;
#82381=CARTESIAN_POINT('Ctrl Pts',(-19.7280504821707,21.2835676751337,122.248639614342)) ;
#82382=CARTESIAN_POINT('Ctrl Pts',(-19.9258060478764,21.2936017115617,122.322083795872)) ;
#82383=CARTESIAN_POINT('Ctrl Pts',(-20.1052484653061,21.3034891385198,122.426997625945)) ;
#82384=CARTESIAN_POINT('Ctrl Pts',(-20.2660567351159,21.3135035728562,122.562908279566)) ;
#82385=CARTESIAN_POINT('Ctrl Pts',(-20.4006745778762,21.3235385174911,122.725323864246)) ;
#82386=CARTESIAN_POINT('Ctrl Pts',(-20.5034505638933,21.3333708675221,122.904698004707)) ;
#82387=CARTESIAN_POINT('Ctrl Pts',(-20.5752878328286,21.3434463066393,123.103919084727)) ;
#82388=CARTESIAN_POINT('Ctrl Pts',(-20.6107746375596,21.3532987718739,123.308030795076)) ;
#82389=CARTESIAN_POINT('Ctrl Pts',(-20.6104406096869,21.3633716494508,123.51975852017)) ;
#82390=CARTESIAN_POINT('Ctrl Pts',(-20.5741595231419,21.3732142456433,123.723492699423)) ;
#82391=CARTESIAN_POINT('Ctrl Pts',(-20.502730586389,21.3831946297586,123.920769607282)) ;
#82392=CARTESIAN_POINT('Ctrl Pts',(-20.3973760350854,21.3932131104074,124.103140698037)) ;
#82393=CARTESIAN_POINT('Ctrl Pts',(-20.2641044764514,21.4030964254077,124.262579989455)) ;
#82394=CARTESIAN_POINT('Ctrl Pts',(-20.1021843288943,21.4131647224982,124.398852256054)) ;
#82395=CARTESIAN_POINT('Ctrl Pts',(-19.9234578599345,21.4229947908705,124.502677758348)) ;
#82396=CARTESIAN_POINT('Ctrl Pts',(-19.7249073454882,21.4330615833389,124.575830411415)) ;
#82397=CARTESIAN_POINT('Ctrl Pts',(-19.5202525728482,21.4429509168274,124.612656973868)) ;
#82398=CARTESIAN_POINT('Ctrl Pts',(-19.310016393334,21.4529530482435,124.613728175413)) ;
#82399=CARTESIAN_POINT('Ctrl Pts',(-19.1043135048021,21.4628769178645,124.578676680394)) ;
#82400=CARTESIAN_POINT('Ctrl Pts',(-18.9055379557793,21.4729204333817,124.507558457858)) ;
#82401=CARTESIAN_POINT('Ctrl Pts',(-18.7248962511209,21.48280264627,124.404861344333)) ;
#82402=CARTESIAN_POINT('Ctrl Pts',(-18.5618819358323,21.4928707234894,124.26991318281)) ;
#82403=CARTESIAN_POINT('Ctrl Pts',(-18.4277131737804,21.5027092282236,124.112452199386)) ;
#82404=CARTESIAN_POINT('Ctrl Pts',(-18.3203059133888,21.512771996653,123.930225116019)) ;
#82405=CARTESIAN_POINT('Ctrl Pts',(-18.2475914284263,21.5226689899357,123.735266065714)) ;
#82406=CARTESIAN_POINT('Ctrl Pts',(-18.2090196028703,21.5326002175705,123.530079755485)) ;
#82407=CARTESIAN_POINT('Ctrl Pts',(-18.2068659043944,21.5426423762126,123.318975217952)) ;
#82408=CARTESIAN_POINT('Ctrl Pts',(-18.2407188945203,21.5525290857437,123.11389200301)) ;
#82409=CARTESIAN_POINT('Ctrl Pts',(-18.3100668942293,21.5625220581723,122.915594081842)) ;
#82410=CARTESIAN_POINT('Ctrl Pts',(-18.4123921025152,21.5724682527089,122.73324535457)) ;
#82411=CARTESIAN_POINT('Ctrl Pts',(-18.5444723633924,21.5824136275604,122.571139711593)) ;
#82412=CARTESIAN_POINT('Ctrl Pts',(-18.7046180543727,21.5924685469203,122.433199194873)) ;
#82413=CARTESIAN_POINT('Ctrl Pts',(-18.8819052439076,21.6022900663638,122.32730254651)) ;
#82414=CARTESIAN_POINT('Ctrl Pts',(-19.0795341491452,21.6123558351307,122.251751647162)) ;
#82415=CARTESIAN_POINT('Ctrl Pts',(-19.2839834267402,21.6222577567857,122.212371550904)) ;
#82416=CARTESIAN_POINT('Ctrl Pts',(-19.4950721221416,21.6323008156068,122.208856215622)) ;
#82417=CARTESIAN_POINT('Ctrl Pts',(-19.7007257257666,21.6422068096495,122.241706225376)) ;
#82418=CARTESIAN_POINT('Ctrl Pts',(-19.8983768302514,21.6521445827313,122.309400724326)) ;
#82419=CARTESIAN_POINT('Ctrl Pts',(-20.0830478955549,21.6621849464636,122.411625303527)) ;
#82420=CARTESIAN_POINT('Ctrl Pts',(-20.2447725573388,21.6720722901871,122.542225508942)) ;
#82421=CARTESIAN_POINT('Ctrl Pts',(-20.3830581794245,21.6820645207558,122.700338520228)) ;
#82422=CARTESIAN_POINT('Ctrl Pts',(-20.491278690877,21.6920130485394,122.879326392428)) ;
#82423=CARTESIAN_POINT('Ctrl Pts',(-20.5669519629379,21.7019498322627,123.074021956924)) ;
#82424=CARTESIAN_POINT('Ctrl Pts',(-20.608129406161,21.7119328330596,123.279844256603)) ;
#82425=CARTESIAN_POINT('Ctrl Pts',(-20.6125825117782,21.7219767199004,123.490926869864)) ;
#82426=CARTESIAN_POINT('Ctrl Pts',(-20.5814885190451,21.7318047434749,123.695222689568)) ;
#82427=CARTESIAN_POINT('Ctrl Pts',(-20.5138274657763,21.7418819916886,123.895933180593)) ;
#82428=CARTESIAN_POINT('Ctrl Pts',(-20.4147141986854,21.7517315469939,124.077802382472)) ;
#82429=CARTESIAN_POINT('Ctrl Pts',(-20.2825949519492,21.7618142551916,124.24349248853)) ;
#82430=CARTESIAN_POINT('Ctrl Pts',(-20.1280211029921,21.771626848118,124.380174263147)) ;
#82431=CARTESIAN_POINT('Ctrl Pts',(-19.9477576074203,21.781694040376,124.490980583927)) ;
#82432=CARTESIAN_POINT('Ctrl Pts',(-19.754162533042,21.7915928698386,124.567467527028)) ;
#82433=CARTESIAN_POINT('Ctrl Pts',(-19.5471445495349,21.8016468610288,124.60990198465)) ;
#82434=CARTESIAN_POINT('Ctrl Pts',(-19.3396514700833,21.811518585812,124.615828020924)) ;
#82435=CARTESIAN_POINT('Ctrl Pts',(-19.1302180432198,21.8215890279422,124.585090725879)) ;
#82436=CARTESIAN_POINT('Ctrl Pts',(-18.9339576769579,21.8314221063725,124.520098546332)) ;
#82437=CARTESIAN_POINT('Ctrl Pts',(-18.7480491234729,21.8414525798739,124.420590536606)) ;
#82438=CARTESIAN_POINT('Ctrl Pts',(-18.5825887690176,21.8514841791725,124.289804551159)) ;
#82439=CARTESIAN_POINT('Ctrl Pts',(-18.444868573602,21.8613138802107,124.135752800917)) ;
#82440=CARTESIAN_POINT('Ctrl Pts',(-18.333675525086,21.8713033182672,123.957587871481)) ;
#82441=CARTESIAN_POINT('Ctrl Pts',(-18.2551799356059,21.8813472214833,123.761568593398)) ;
#82442=CARTESIAN_POINT('Ctrl Pts',(-18.2124473458304,21.8911687422968,123.559558751751)) ;
#82443=CARTESIAN_POINT('Ctrl Pts',(-18.2047822894588,21.9012044665439,123.348720043273)) ;
#82444=CARTESIAN_POINT('Ctrl Pts',(-18.2343460999651,21.9112266204764,123.140091270568)) ;
#82445=CARTESIAN_POINT('Ctrl Pts',(-18.2983110659554,21.9210888522337,122.942886802025)) ;
#82446=CARTESIAN_POINT('Ctrl Pts',(-18.3959903010469,21.9310479226916,122.757690814069)) ;
#82447=CARTESIAN_POINT('Ctrl Pts',(-18.5255720615345,21.9410830950677,122.591216505646)) ;
#82448=CARTESIAN_POINT('Ctrl Pts',(-18.67949002609,21.950963480226,122.451700734787)) ;
#82449=CARTESIAN_POINT('Ctrl Pts',(-18.858352008295,21.9610201948199,122.339007613317)) ;
#82450=CARTESIAN_POINT('Ctrl Pts',(-19.0506455514497,21.970899463392,122.260495049301)) ;
#82451=CARTESIAN_POINT('Ctrl Pts',(-19.2558150150403,21.9808904208777,122.215517103777)) ;
#82452=CARTESIAN_POINT('Ctrl Pts',(-19.4667419989655,21.9909310795129,122.207269166707)) ;
#82453=CARTESIAN_POINT('Ctrl Pts',(-19.6716113086595,22.0007640592209,122.234836706723)) ;
#82454=CARTESIAN_POINT('Ctrl Pts',(-19.8719733239983,22.0107571924706,122.298006116924)) ;
#82455=CARTESIAN_POINT('Ctrl Pts',(-20.0588577669836,22.0207892448539,122.395778372292)) ;
#82456=CARTESIAN_POINT('Ctrl Pts',(-20.2232889178433,22.0306544738052,122.522158713069)) ;
#82457=CARTESIAN_POINT('Ctrl Pts',(-20.3650985185716,22.0406164150485,122.67628155435)) ;
#82458=CARTESIAN_POINT('Ctrl Pts',(-20.4785231195851,22.0506511300852,122.854145179665)) ;
#82459=CARTESIAN_POINT('Ctrl Pts',(-20.5584654837704,22.0605369004293,123.046012221598)) ;
#82460=CARTESIAN_POINT('Ctrl Pts',(-20.6046775906511,22.070599497818,123.252424729211)) ;
#82461=CARTESIAN_POINT('Ctrl Pts',(-20.6142383738852,22.0804499096533,123.4593067714)) ;
#82462=CARTESIAN_POINT('Ctrl Pts',(-20.5877974801273,22.0904770789392,123.668438866555)) ;
#82463=CARTESIAN_POINT('Ctrl Pts',(-20.5249128796181,22.1005045596534,123.86966118125)) ;
#82464=CARTESIAN_POINT('Ctrl Pts',(-20.4301887585523,22.1103476122327,124.053631108362)) ;
#82465=CARTESIAN_POINT('Ctrl Pts',(-20.3034636441155,22.1203415156713,124.22121369691)) ;
#82466=CARTESIAN_POINT('Ctrl Pts',(-20.1487862388261,22.1303686384477,124.364442189682)) ;
#82467=CARTESIAN_POINT('Ctrl Pts',(-19.9741429312409,22.1402593433397,124.477302554671)) ;
#82468=CARTESIAN_POINT('Ctrl Pts',(-19.7807209988621,22.1502513701901,124.55922910085)) ;
#82469=CARTESIAN_POINT('Ctrl Pts',(-19.5769360895709,22.1601973516786,124.606050630884)) ;
#82470=CARTESIAN_POINT('Ctrl Pts',(-19.3681010795256,22.1701445243005,124.617200647158)) ;
#82471=CARTESIAN_POINT('Ctrl Pts',(-19.1584464253659,22.1801924656267,124.591432575702)) ;
#82472=CARTESIAN_POINT('Ctrl Pts',(-18.9604177789619,22.1900400994344,124.531049438807)) ;
#82473=CARTESIAN_POINT('Ctrl Pts',(-18.7734573964872,22.2000018141195,124.436702699596)) ;
#82474=CARTESIAN_POINT('Ctrl Pts',(-18.6047340277275,22.210030446998,124.310256642053)) ;
#82475=CARTESIAN_POINT('Ctrl Pts',(-18.4621942277681,22.2199407725331,124.158312602361)) ;
#82476=CARTESIAN_POINT('Ctrl Pts',(-18.3474585546691,22.2298756030049,123.983782776444)) ;
#82477=CARTESIAN_POINT('Ctrl Pts',(-18.2640502980382,22.2399169353868,123.78985928878)) ;
#82478=CARTESIAN_POINT('Ctrl Pts',(-18.2162240860105,22.2498098088257,123.58745557848)) ;
#82479=CARTESIAN_POINT('Ctrl Pts',(-18.2036438426885,22.2597789746436,123.378240631757)) ;
#82480=CARTESIAN_POINT('Ctrl Pts',(-18.2280682146378,22.2698077083601,123.168844828151)) ;
#82481=CARTESIAN_POINT('Ctrl Pts',(-18.3069945528939,22.2830002271312,122.902886750421)) ;
#82482=CARTESIAN_POINT('Ctrl Pts',(-18.4552999005184,22.2963600951739,122.66069779592)) ;
#82483=CARTESIAN_POINT('Ctrl Pts',(-18.6570215898245,22.3095854323228,122.469325661276)) ;
#82484=CARTESIAN_POINT('Ctrl Pts',(-18.8316797652282,22.3195666581634,122.353021542224)) ;
#82485=CARTESIAN_POINT('Ctrl Pts',(-19.025082549416,22.3296022251463,122.26873651452)) ;
#82486=CARTESIAN_POINT('Ctrl Pts',(-19.22658820499,22.3394653031084,122.219744511049)) ;
#82487=CARTESIAN_POINT('Ctrl Pts',(-19.437838742601,22.3495356019095,122.206163829392)) ;
#82488=CARTESIAN_POINT('Ctrl Pts',(-19.6435055191939,22.3593779004773,122.228957325514)) ;
#82489=CARTESIAN_POINT('Ctrl Pts',(-19.8446819369498,22.3693385986471,122.287067922869)) ;
#82490=CARTESIAN_POINT('Ctrl Pts',(-20.0339845517462,22.3793766328265,122.380317508446)) ;
#82491=CARTESIAN_POINT('Ctrl Pts',(-20.2016926105113,22.389250369673,122.502684369457)) ;
#82492=CARTESIAN_POINT('Ctrl Pts',(-20.3484344011402,22.3993221535983,122.655289347127)) ;
#82493=CARTESIAN_POINT('Ctrl Pts',(-20.4637741168611,22.4091542747995,122.826843880767)) ;
#82494=CARTESIAN_POINT('Ctrl Pts',(-20.5497920261545,22.4191872988249,123.019422041315)) ;
#82495=CARTESIAN_POINT('Ctrl Pts',(-20.6004603771645,22.4292031790216,123.223814284378)) ;
#82496=CARTESIAN_POINT('Ctrl Pts',(-20.6150640004931,22.4390866981158,123.431083471758)) ;
#82497=CARTESIAN_POINT('Ctrl Pts',(-20.5934940797132,22.4490771104794,123.639987608933)) ;
#82498=CARTESIAN_POINT('Ctrl Pts',(-20.517218240559,22.4623402736829,123.908212352652)) ;
#82499=CARTESIAN_POINT('Ctrl Pts',(-20.3727555418363,22.4756178439341,124.150777416786)) ;
#82500=CARTESIAN_POINT('Ctrl Pts',(-20.1718123791193,22.4889481464407,124.346093847646)) ;
#82501=CARTESIAN_POINT('Ctrl Pts',(-19.9998410836339,22.4988468282571,124.463290434871)) ;
#82502=CARTESIAN_POINT('Ctrl Pts',(-19.8085085382788,22.5088363433046,124.549850694843)) ;
#82503=CARTESIAN_POINT('Ctrl Pts',(-19.6058755849689,22.5187843950796,124.601655303795)) ;
#82504=CARTESIAN_POINT('Ctrl Pts',(-19.3975125848243,22.5287257983581,124.61774036324)) ;
#82505=CARTESIAN_POINT('Ctrl Pts',(-19.1194367253564,22.5420124631391,124.590882659697)) ;
#82506=CARTESIAN_POINT('Ctrl Pts',(-18.788660398813,22.5586228847939,124.46721791432)) ;
#82507=CARTESIAN_POINT('Ctrl Pts',(-18.4662722077278,22.5785341470447,124.192767698316)) ;
#82508=CARTESIAN_POINT('Ctrl Pts',(-18.2564052347418,22.5984782762096,123.824248386877)) ;
#82509=CARTESIAN_POINT('Ctrl Pts',(-18.1850298158601,22.6184014388147,123.406724093783)) ;
#82510=CARTESIAN_POINT('Ctrl Pts',(-18.2596165922756,22.6382915612213,122.990368848326)) ;
#82511=CARTESIAN_POINT('Ctrl Pts',(-18.4732461365668,22.6582965148214,122.622623863024)) ;
#82512=CARTESIAN_POINT('Ctrl Pts',(-18.7967224378562,22.678134771837,122.351774793471)) ;
#82513=CARTESIAN_POINT('Ctrl Pts',(-19.1960527549602,22.6981290726235,122.206072274783)) ;
#82514=CARTESIAN_POINT('Ctrl Pts',(-19.6188774272319,22.718014314668,122.205770397816)) ;
#82515=CARTESIAN_POINT('Ctrl Pts',(-20.0166123098937,22.7378892611439,122.348576418114)) ;
#82516=CARTESIAN_POINT('Ctrl Pts',(-20.3441438839441,22.757922331085,122.620968086443)) ;
#82517=CARTESIAN_POINT('Ctrl Pts',(-20.5570158705556,22.7778108379854,122.986324841109)) ;
#82518=CARTESIAN_POINT('Ctrl Pts',(-20.6337660265927,22.7976656977667,123.401523678932)) ;
#82519=CARTESIAN_POINT('Ctrl Pts',(-20.5628771685772,22.8177165315544,123.821821293036)) ;
#82520=CARTESIAN_POINT('Ctrl Pts',(-20.3561026233615,22.8374824734436,124.18784828046)) ;
#82521=CARTESIAN_POINT('Ctrl Pts',(-20.0335851048464,22.857495204903,124.465242814785)) ;
#82522=CARTESIAN_POINT('Ctrl Pts',(-19.6377262813745,22.8773880398465,124.61457533021)) ;
#82523=CARTESIAN_POINT('Ctrl Pts',(-19.2145951458485,22.8972950631861,124.620562118106)) ;
#82524=CARTESIAN_POINT('Ctrl Pts',(-18.8143052784339,22.9172103280868,124.48212442822)) ;
#82525=CARTESIAN_POINT('Ctrl Pts',(-18.4838083763501,22.9372420202465,124.213504451096)) ;
#82526=CARTESIAN_POINT('Ctrl Pts',(-18.2668145194159,22.9570850668195,123.851613055632)) ;
#82527=CARTESIAN_POINT('Ctrl Pts',(-18.1851080185163,22.9770016147193,123.436153668619)) ;
#82528=CARTESIAN_POINT('Ctrl Pts',(-18.2502202177031,22.9969338577106,123.017334018235)) ;
#82529=CARTESIAN_POINT('Ctrl Pts',(-18.4538258820045,23.0168376925199,122.646347008578)) ;
#82530=CARTESIAN_POINT('Ctrl Pts',(-18.7714168386275,23.0367380927074,122.366744945612)) ;
#82531=CARTESIAN_POINT('Ctrl Pts',(-19.1662858522202,23.0566877690867,122.211749727135)) ;
#82532=CARTESIAN_POINT('Ctrl Pts',(-19.5899723211097,23.0766202933071,122.200906811496)) ;
#82533=CARTESIAN_POINT('Ctrl Pts',(-19.9918128358523,23.0965403022933,122.334876915876)) ;
#82534=CARTESIAN_POINT('Ctrl Pts',(-20.3243318262341,23.1164972084694,122.598424755681)) ;
#82535=CARTESIAN_POINT('Ctrl Pts',(-20.5465556585454,23.1363830479709,122.95823999004)) ;
#82536=CARTESIAN_POINT('Ctrl Pts',(-20.6329370108439,23.1563542201068,123.373906265248)) ;
#82537=CARTESIAN_POINT('Ctrl Pts',(-20.573322927364,23.1761684170912,123.791036823515)) ;
#82538=CARTESIAN_POINT('Ctrl Pts',(-20.3738396316099,23.1961496030594,124.166064107875)) ;
#82539=CARTESIAN_POINT('Ctrl Pts',(-20.1119254262802,23.2127251084487,124.401936038304)) ;
#82540=CARTESIAN_POINT('Ctrl Pts',(-19.8627907757275,23.2260345563123,124.529374358132)) ;
#82541=CARTESIAN_POINT('Ctrl Pts',(-19.5941634496156,23.2394022540889,124.611788229656)) ;
#82542=CARTESIAN_POINT('Ctrl Pts',(-19.2437165005351,23.2558928257548,124.624712070297)) ;
#82543=CARTESIAN_POINT('Ctrl Pts',(-18.84025681319,23.2758130980876,124.49601281634)) ;
#82544=CARTESIAN_POINT('Ctrl Pts',(-18.5605856338908,23.2924301338086,124.280092561327)) ;
#82545=CARTESIAN_POINT('Ctrl Pts',(-18.3909771122857,23.3057209840897,124.057986573605)) ;
#82546=CARTESIAN_POINT('Ctrl Pts',(-18.2945642892611,23.3156900292442,123.871929208905)) ;
#82547=CARTESIAN_POINT('Ctrl Pts',(-18.2319237623496,23.3255934198777,123.673347940635)) ;
#82548=CARTESIAN_POINT('Ctrl Pts',(-18.2044109627458,23.3356512059904,123.463725251977)) ;
#82549=CARTESIAN_POINT('Ctrl Pts',(-18.2133455814225,23.3455032426402,123.256767963458)) ;
#82550=CARTESIAN_POINT('Ctrl Pts',(-18.2735481031819,23.3588683667834,122.982370270208)) ;
#82551=CARTESIAN_POINT('Ctrl Pts',(-18.4029731145721,23.3720944297464,122.732648890195)) ;
#82552=CARTESIAN_POINT('Ctrl Pts',(-18.5911585972298,23.3853980780287,122.525747425895)) ;
#82553=CARTESIAN_POINT('Ctrl Pts',(-18.7572840249593,23.3953896091917,122.397160356993)) ;
#82554=CARTESIAN_POINT('Ctrl Pts',(-18.9442034218826,23.405429056991,122.299171365096)) ;
#82555=CARTESIAN_POINT('Ctrl Pts',(-19.1413113103794,23.4152728325048,122.236069997522)) ;
#82556=CARTESIAN_POINT('Ctrl Pts',(-19.3492334705242,23.4252584738925,122.207338845479)) ;
#82557=CARTESIAN_POINT('Ctrl Pts',(-19.5580294441203,23.4351952582543,122.214996284707)) ;
#82558=CARTESIAN_POINT('Ctrl Pts',(-19.7645715963343,23.4452450927216,122.259384713795)) ;
#82559=CARTESIAN_POINT('Ctrl Pts',(-19.9564788390194,23.4550955422248,122.33725097854)) ;
#82560=CARTESIAN_POINT('Ctrl Pts',(-20.1343708523743,23.4650675562069,122.448127375331)) ;
#82561=CARTESIAN_POINT('Ctrl Pts',(-20.290697050754,23.475062714054,122.588593746515)) ;
#82562=CARTESIAN_POINT('Ctrl Pts',(-20.4205292525816,23.4850966404177,122.75482783176)) ;
#82563=CARTESIAN_POINT('Ctrl Pts',(-20.5180699407723,23.4949523488501,122.937651926998)) ;
#82564=CARTESIAN_POINT('Ctrl Pts',(-20.5835848064832,23.5049504981887,123.137338609662)) ;
#82565=CARTESIAN_POINT('Ctrl Pts',(-20.6133315592433,23.5148499013623,123.343349263886)) ;
#82566=CARTESIAN_POINT('Ctrl Pts',(-20.6068042976346,23.5249010982508,123.554533941708)) ;
#82567=CARTESIAN_POINT('Ctrl Pts',(-20.5644542845727,23.5347834220636,123.757945272623)) ;
#82568=CARTESIAN_POINT('Ctrl Pts',(-20.4869988626981,23.5447783177202,123.953265935445)) ;
#82569=CARTESIAN_POINT('Ctrl Pts',(-20.3762451240115,23.5547994171028,124.132491954)) ;
#82570=CARTESIAN_POINT('Ctrl Pts',(-20.2377780768666,23.5647066849648,124.288078659894)) ;
#82571=CARTESIAN_POINT('Ctrl Pts',(-20.0741559214403,23.5746450287901,124.417986713011)) ;
#82572=CARTESIAN_POINT('Ctrl Pts',(-19.8892906509235,23.5846484480906,124.518297171664)) ;
#82573=CARTESIAN_POINT('Ctrl Pts',(-19.6891176969412,23.5946829987977,124.584849929833)) ;
#82574=CARTESIAN_POINT('Ctrl Pts',(-19.4844008635135,23.6045279484033,124.615406104231)) ;
#82575=CARTESIAN_POINT('Ctrl Pts',(-19.2745631998316,23.6145137905162,124.61026978037)) ;
#82576=CARTESIAN_POINT('Ctrl Pts',(-19.0697563432002,23.6244485978853,124.56912101187)) ;
#82577=CARTESIAN_POINT('Ctrl Pts',(-18.8729354133231,23.6345061395986,124.491945311398)) ;
#82578=CARTESIAN_POINT('Ctrl Pts',(-18.6965271286141,23.6443277371107,124.384596044604)) ;
#82579=CARTESIAN_POINT('Ctrl Pts',(-18.5375052095962,23.6543839965912,124.245310916362)) ;
#82580=CARTESIAN_POINT('Ctrl Pts',(-18.4068828190707,23.6643239328916,124.082183811168)) ;
#82581=CARTESIAN_POINT('Ctrl Pts',(-18.3063569600864,23.674231053636,123.89977336365)) ;
#82582=CARTESIAN_POINT('Ctrl Pts',(-18.2381821022871,23.6842739595613,123.699954793719)) ;
#82583=CARTESIAN_POINT('Ctrl Pts',(-18.2061315885862,23.6941817406604,123.494134504047)) ;
#82584=CARTESIAN_POINT('Ctrl Pts',(-18.2099782470609,23.7041921096629,123.283713238738)) ;
#82585=CARTESIAN_POINT('Ctrl Pts',(-18.2508047879774,23.7142229482317,123.076824775959)) ;
#82586=CARTESIAN_POINT('Ctrl Pts',(-18.3252380545856,23.7240757878714,122.883518206758)) ;
#82587=CARTESIAN_POINT('Ctrl Pts',(-18.4332307035632,23.7340637890363,122.703457541296)) ;
#82588=CARTESIAN_POINT('Ctrl Pts',(-18.5700431604149,23.7439926080155,122.545803259153)) ;
#82589=CARTESIAN_POINT('Ctrl Pts',(-18.7328941586295,23.7539803107378,122.413240963306)) ;
#82590=CARTESIAN_POINT('Ctrl Pts',(-18.9173305893805,23.7640163105405,122.310793634948)) ;
#82591=CARTESIAN_POINT('Ctrl Pts',(-19.1130661829979,23.7738711803419,122.242836707875)) ;
#82592=CARTESIAN_POINT('Ctrl Pts',(-19.3205318093657,23.7838706107654,122.209140766422)) ;
#82593=CARTESIAN_POINT('Ctrl Pts',(-19.528576529855,23.7937657282307,122.211727967725)) ;
#82594=CARTESIAN_POINT('Ctrl Pts',(-19.7363643552713,23.8038262217477,122.251054379042)) ;
#82595=CARTESIAN_POINT('Ctrl Pts',(-19.9300969389221,23.8136757019489,122.324201642346)) ;
#82596=CARTESIAN_POINT('Ctrl Pts',(-20.1116481535929,23.8237021522127,122.431297541146)) ;
#82597=CARTESIAN_POINT('Ctrl Pts',(-20.2715506779212,23.8337334426908,122.568801980816)) ;
#82598=CARTESIAN_POINT('Ctrl Pts',(-20.4029659176429,23.8435748303426,122.728604738249)) ;
#82599=CARTESIAN_POINT('Ctrl Pts',(-20.5066563597952,23.8535782312338,122.911544076918)) ;
#82600=CARTESIAN_POINT('Ctrl Pts',(-20.5768109022022,23.863562614025,123.109415512319)) ;
#82601=CARTESIAN_POINT('Ctrl Pts',(-20.6115256239944,23.8736017040384,123.31757326113)) ;
#82602=CARTESIAN_POINT('Ctrl Pts',(-20.6098969878997,23.8834475129475,123.524571599926)) ;
#82603=CARTESIAN_POINT('Ctrl Pts',(-20.5722509348656,23.8934319357665,123.731041364494)) ;
#82604=CARTESIAN_POINT('Ctrl Pts',(-20.4997173978823,23.9033715610077,123.927042140903)) ;
#82605=CARTESIAN_POINT('Ctrl Pts',(-20.3931719092889,23.9134112505264,124.109223158577)) ;
#82606=CARTESIAN_POINT('Ctrl Pts',(-20.2587341754022,23.923299438945,124.267797397072)) ;
#82607=CARTESIAN_POINT('Ctrl Pts',(-20.0974322378108,23.933288964947,124.402272331516)) ;
#82608=CARTESIAN_POINT('Ctrl Pts',(-19.915715878204,23.9432474663022,124.506233907612)) ;
#82609=CARTESIAN_POINT('Ctrl Pts',(-19.7200317103862,23.9531470603059,124.577135525943)) ;
#82610=CARTESIAN_POINT('Ctrl Pts',(-19.5119585755635,23.9631949484272,124.613440422247)) ;
#82611=CARTESIAN_POINT('Ctrl Pts',(-19.3038930888951,23.9730903736727,124.613234238601)) ;
#82612=CARTESIAN_POINT('Ctrl Pts',(-19.0956394147176,23.9831517643733,124.576334613564)) ;
#82613=CARTESIAN_POINT('Ctrl Pts',(-18.9011714992526,23.9929973480599,124.505414746921)) ;
#82614=CARTESIAN_POINT('Ctrl Pts',(-18.7195046967717,24.0029603213691,124.401196093712)) ;
#82615=CARTESIAN_POINT('Ctrl Pts',(-18.5578392061729,24.0129859881949,124.265939513218)) ;
#82616=CARTESIAN_POINT('Ctrl Pts',(-18.4235465432553,24.0229004660612,124.106543727124)) ;
#82617=CARTESIAN_POINT('Ctrl Pts',(-18.3178150664723,24.0328889807362,123.925094508878)) ;
#82618=CARTESIAN_POINT('Ctrl Pts',(-18.2452273820998,24.0429330916517,123.72682449614)) ;
#82619=CARTESIAN_POINT('Ctrl Pts',(-18.2084622185153,24.0527612292462,123.523473719363)) ;
#82620=CARTESIAN_POINT('Ctrl Pts',(-18.2074439800112,24.0628377973052,123.311677825631)) ;
#82621=CARTESIAN_POINT('Ctrl Pts',(-18.2423298172474,24.0726899592093,123.107467672833)) ;
#82622=CARTESIAN_POINT('Ctrl Pts',(-18.3135158921644,24.0827629211662,122.908064117061)) ;
#82623=CARTESIAN_POINT('Ctrl Pts',(-18.4159003186132,24.0926054831691,122.728227437951)) ;
#82624=CARTESIAN_POINT('Ctrl Pts',(-18.5492445179135,24.1025859196629,122.566240438821)) ;
#82625=CARTESIAN_POINT('Ctrl Pts',(-18.7095634324068,24.1126042249873,122.429654343682)) ;
#82626=CARTESIAN_POINT('Ctrl Pts',(-18.8885295576989,24.1224881889067,122.324026226446)) ;
#82627=CARTESIAN_POINT('Ctrl Pts',(-19.0866747117363,24.1325540656453,122.249802038306)) ;
#82628=CARTESIAN_POINT('Ctrl Pts',(-19.2900277987292,24.1423931665062,122.211839217238)) ;
#82629=CARTESIAN_POINT('Ctrl Pts',(-19.5009280452446,24.1524262493719,122.209188900034)) ;
#82630=CARTESIAN_POINT('Ctrl Pts',(-19.7087891088746,24.1624479346474,122.243680922594)) ;
#82631=CARTESIAN_POINT('Ctrl Pts',(-19.9045118842529,24.1723146297458,122.312331343585)) ;
#82632=CARTESIAN_POINT('Ctrl Pts',(-20.0873424230859,24.1822745194804,122.414410683436)) ;
#82633=CARTESIAN_POINT('Ctrl Pts',(-20.2506734219996,24.1923095073059,122.547919076296)) ;
#82634=CARTESIAN_POINT('Ctrl Pts',(-20.3865972542028,24.2021962113802,122.70520302407)) ;
#82635=CARTESIAN_POINT('Ctrl Pts',(-20.4949915148063,24.2122613556131,122.886893116054)) ;
#82636=CARTESIAN_POINT('Ctrl Pts',(-20.5687253538472,24.2221006463416,123.080191844963)) ;
#82637=CARTESIAN_POINT('Ctrl Pts',(-20.608936234929,24.2321632037801,123.28785666925)) ;
#82638=CARTESIAN_POINT('Ctrl Pts',(-20.6121978969833,24.2420602550322,123.495909815713)) ;
#82639=CARTESIAN_POINT('Ctrl Pts',(-20.5798621410768,24.2519914617804,123.702170633504)) ;
#82640=CARTESIAN_POINT('Ctrl Pts',(-20.5112278003848,24.2620336459993,123.901818282665)) ;
#82641=CARTESIAN_POINT('Ctrl Pts',(-20.4106814466933,24.2719202741102,124.083739096484)) ;
#82642=CARTESIAN_POINT('Ctrl Pts',(-20.2789510205555,24.2819135466426,124.247385519698)) ;
#82643=CARTESIAN_POINT('Ctrl Pts',(-20.1215139965701,24.291858622184,124.384961385471)) ;
#82644=CARTESIAN_POINT('Ctrl Pts',(-19.9427040338153,24.3018081729123,124.493512747479)) ;
#82645=CARTESIAN_POINT('Ctrl Pts',(-19.7459483455522,24.3118475077603,124.569858328381)) ;
#82646=CARTESIAN_POINT('Ctrl Pts',(-19.5420958305893,24.3217336467042,124.610447517326)) ;
#82647=CARTESIAN_POINT('Ctrl Pts',(-19.3319860419115,24.3317317596779,124.615343457489)) ;
#82648=CARTESIAN_POINT('Ctrl Pts',(-19.1257788093217,24.3416515220303,124.584048457345)) ;
#82649=CARTESIAN_POINT('Ctrl Pts',(-18.9257658349345,24.351690917643,124.516694244747)) ;
#82650=CARTESIAN_POINT('Ctrl Pts',(-18.7429093393127,24.3616001034313,124.416883437135)) ;
#82651=CARTESIAN_POINT('Ctrl Pts',(-18.5793682381325,24.3715352875888,124.286955899813)) ;
#82652=CARTESIAN_POINT('Ctrl Pts',(-18.4395549919539,24.3815763449747,124.128807119473)) ;
#82653=CARTESIAN_POINT('Ctrl Pts',(-18.3308792199516,24.391463503008,123.951607976595)) ;
#82654=CARTESIAN_POINT('Ctrl Pts',(-18.2534953332544,24.4014557826839,123.756326943082)) ;
#82655=CARTESIAN_POINT('Ctrl Pts',(-18.2114309361531,24.4114042997289,123.551439509569)) ;
#82656=CARTESIAN_POINT('Ctrl Pts',(-18.2052935477801,24.4213410772993,123.342645056263)) ;
#82657=CARTESIAN_POINT('Ctrl Pts',(-18.2353874902954,24.4313241134463,123.134912265281)) ;
#82658=CARTESIAN_POINT('Ctrl Pts',(-18.3018447177131,24.44136786504,122.934516737873)) ;
#82659=CARTESIAN_POINT('Ctrl Pts',(-18.3995391049124,24.4511963942526,122.75241027329)) ;
#82660=CARTESIAN_POINT('Ctrl Pts',(-18.5304447148588,24.4612717551613,122.585941029605)) ;
#82661=CARTESIAN_POINT('Ctrl Pts',(-18.6848541226501,24.4711283540485,122.447684982794)) ;
#82662=CARTESIAN_POINT('Ctrl Pts',(-18.864422486662,24.4811913480664,122.335908343508)) ;
#82663=CARTESIAN_POINT('Ctrl Pts',(-19.0571387654209,24.4910692823558,122.258444824587)) ;
#82664=CARTESIAN_POINT('Ctrl Pts',(-19.2627623039169,24.5010699299139,122.214785947123)) ;
#82665=CARTESIAN_POINT('Ctrl Pts',(-19.4711725797811,24.5109877763519,122.207393835235)) ;
#82666=CARTESIAN_POINT('Ctrl Pts',(-19.6803970457402,24.5210388933576,122.236738188576)) ;
#82667=CARTESIAN_POINT('Ctrl Pts',(-19.8778824426931,24.5309096286682,122.30059393333)) ;
#82668=CARTESIAN_POINT('Ctrl Pts',(-20.0649514483934,24.5409803359112,122.399666053777)) ;
#82669=CARTESIAN_POINT('Ctrl Pts',(-20.2281337107902,24.5508133433631,122.5266026047)) ;
#82670=CARTESIAN_POINT('Ctrl Pts',(-20.370009757199,24.5608438356654,122.682600129859)) ;
#82671=CARTESIAN_POINT('Ctrl Pts',(-20.4821469112332,24.5708754307388,122.861226309303)) ;
#82672=CARTESIAN_POINT('Ctrl Pts',(-20.5603565453377,24.580705129877,123.05249064484)) ;
#82673=CARTESIAN_POINT('Ctrl Pts',(-20.6054976015341,24.5906945797586,123.257597896419)) ;
#82674=CARTESIAN_POINT('Ctrl Pts',(-20.6138517558197,24.6007384375743,123.468583732253)) ;
#82675=CARTESIAN_POINT('Ctrl Pts',(-20.5864978778444,24.6105601281645,123.67324702507)) ;
#82676=CARTESIAN_POINT('Ctrl Pts',(-20.5231546982953,24.6205952187049,123.874478649542)) ;
#82677=CARTESIAN_POINT('Ctrl Pts',(-20.4254304035954,24.6306197376876,124.061214681155)) ;
#82678=CARTESIAN_POINT('Ctrl Pts',(-20.2991788046576,24.6404795830978,124.22559646436)) ;
#82679=CARTESIAN_POINT('Ctrl Pts',(-20.145129895565,24.6504393594134,124.367416560908)) ;
#82680=CARTESIAN_POINT('Ctrl Pts',(-19.9674334411512,24.6604675567281,124.480860594718)) ;
#82681=CARTESIAN_POINT('Ctrl Pts',(-19.7751577797198,24.6703750990184,124.560990106468)) ;
#82682=CARTESIAN_POINT('Ctrl Pts',(-19.5693703328522,24.6804077495822,124.607155032494)) ;
#82683=CARTESIAN_POINT('Ctrl Pts',(-19.3617967555664,24.6902917060089,124.61680553169)) ;
#82684=CARTESIAN_POINT('Ctrl Pts',(-19.1534319522652,24.7002814073707,124.590503034334)) ;
#82685=CARTESIAN_POINT('Ctrl Pts',(-18.9519051623861,24.7103224026468,124.527673623599)) ;
#82686=CARTESIAN_POINT('Ctrl Pts',(-18.7680835662665,24.7201552919151,124.43311943108)) ;
#82687=CARTESIAN_POINT('Ctrl Pts',(-18.6004240956916,24.7301484502826,124.306526655359)) ;
#82688=CARTESIAN_POINT('Ctrl Pts',(-18.4570479654996,24.7401804926347,124.15183839261)) ;
#82689=CARTESIAN_POINT('Ctrl Pts',(-18.3444058754051,24.7500457365931,123.977707914406)) ;
#82690=CARTESIAN_POINT('Ctrl Pts',(-18.2623662492347,24.7600076278391,123.785008651907)) ;
#82691=CARTESIAN_POINT('Ctrl Pts',(-18.2150227218341,24.7700425278576,123.57943498646)) ;
#82692=CARTESIAN_POINT('Ctrl Pts',(-18.2039108265899,24.7799276082722,123.371890119944)) ;
#82693=CARTESIAN_POINT('Ctrl Pts',(-18.2294765748112,24.789992780397,123.161866623619)) ;
#82694=CARTESIAN_POINT('Ctrl Pts',(-18.2896850160126,24.7998400151205,122.963774156201)) ;
#82695=CARTESIAN_POINT('Ctrl Pts',(-18.3846631838683,24.8098708264382,122.775510299179)) ;
#82696=CARTESIAN_POINT('Ctrl Pts',(-18.5109890530779,24.8198804423517,122.607182357342)) ;
#82697=CARTESIAN_POINT('Ctrl Pts',(-18.6629344097243,24.8297912217554,122.46464599339)) ;
#82698=CARTESIAN_POINT('Ctrl Pts',(-18.8373840507773,24.8397204875445,122.349990527342)) ;
#82699=CARTESIAN_POINT('Ctrl Pts',(-19.0313351917403,24.8497631808571,122.266594739761)) ;
#82700=CARTESIAN_POINT('Ctrl Pts',(-19.2336139838106,24.8596497135518,122.218758538381)) ;
#82701=CARTESIAN_POINT('Ctrl Pts',(-19.443319684323,24.8696428586551,122.206287816751)) ;
#82702=CARTESIAN_POINT('Ctrl Pts',(-19.6510167260348,24.8795885393292,122.230384480415)) ;
#82703=CARTESIAN_POINT('Ctrl Pts',(-19.851538316644,24.8895357969559,122.289780441045)) ;
#82704=CARTESIAN_POINT('Ctrl Pts',(-20.0404730206876,24.8995836990774,122.384240048737)) ;
#82705=CARTESIAN_POINT('Ctrl Pts',(-20.2068658067481,24.9094314046991,122.507427675113)) ;
#82706=CARTESIAN_POINT('Ctrl Pts',(-20.3514609472444,24.9193928713332,122.658908390859)) ;
#82707=CARTESIAN_POINT('Ctrl Pts',(-20.4681229399216,24.9294224246014,122.834556316667)) ;
#82708=CARTESIAN_POINT('Ctrl Pts',(-20.5515899926402,24.9393293166288,123.025376823584)) ;
#82709=CARTESIAN_POINT('Ctrl Pts',(-20.6012474613026,24.9492769607418,123.2285093331)) ;
#82710=CARTESIAN_POINT('Ctrl Pts',(-20.6150856722324,24.9592770037707,123.438313378773)) ;
#82711=CARTESIAN_POINT('Ctrl Pts',(-20.5918280692934,24.9693157697647,123.648058183156)) ;
#82712=CARTESIAN_POINT('Ctrl Pts',(-20.5341801448491,24.9791408317869,123.846419031211)) ;
#82713=CARTESIAN_POINT('Ctrl Pts',(-20.4411614002517,24.9891953791133,124.036215807253)) ;
#82714=CARTESIAN_POINT('Ctrl Pts',(-20.317675914931,24.9991386225625,124.204890724799)) ;
#82715=CARTESIAN_POINT('Ctrl Pts',(-20.1678533868408,25.0090407941704,124.349428618332)) ;
#82716=CARTESIAN_POINT('Ctrl Pts',(-19.992519998126,25.0190936297806,124.46741219479)) ;
#82717=CARTESIAN_POINT('Ctrl Pts',(-19.8028366542702,25.0289666874661,124.551709330501)) ;
#82718=CARTESIAN_POINT('Ctrl Pts',(-19.5990412584524,25.0389619489918,124.602912199608)) ;
#82719=CARTESIAN_POINT('Ctrl Pts',(-19.3887859636416,25.0489873184123,124.617620931804)) ;
#82720=CARTESIAN_POINT('Ctrl Pts',(-19.1819727421528,25.0588771509389,124.596169235394)) ;
#82721=CARTESIAN_POINT('Ctrl Pts',(-18.91306138402,25.0721751217483,124.519808852697)) ;
#82722=CARTESIAN_POINT('Ctrl Pts',(-18.6717643622118,25.0853735168574,124.37640217607)) ;
#82723=CARTESIAN_POINT('Ctrl Pts',(-18.4752738616247,25.0987689591369,124.174746619851)) ;
#82724=CARTESIAN_POINT('Ctrl Pts',(-18.3582246189825,25.1086447973759,124.003215132547)) ;
#82725=CARTESIAN_POINT('Ctrl Pts',(-18.2710748662201,25.1187061999736,123.810519405556)) ;
#82726=CARTESIAN_POINT('Ctrl Pts',(-18.2196533575529,25.1285712569087,123.609567294506)) ;
#82727=CARTESIAN_POINT('Ctrl Pts',(-18.203298763142,25.1385833528575,123.399749571812)) ;
#82728=CARTESIAN_POINT('Ctrl Pts',(-18.2303147257671,25.151860662003,123.121871212669)) ;
#82729=CARTESIAN_POINT('Ctrl Pts',(-18.353792179079,25.1684596875103,122.791296798162)) ;
#82730=CARTESIAN_POINT('Ctrl Pts',(-18.5827030592161,25.1850587355433,122.522606055033)) ;
#82731=CARTESIAN_POINT('Ctrl Pts',(-18.8116926955832,25.1983021475742,122.364286012288)) ;
#82732=CARTESIAN_POINT('Ctrl Pts',(-19.0034239801853,25.2083395752627,122.276149971483)) ;
#82733=CARTESIAN_POINT('Ctrl Pts',(-19.2048452374266,25.2182438772183,122.223388078408)) ;
#82734=CARTESIAN_POINT('Ctrl Pts',(-19.4827947851968,25.2315107171934,122.199905674607)) ;
#82735=CARTESIAN_POINT('Ctrl Pts',(-19.8307375228141,25.2481369152834,122.262279578136)) ;
#82736=CARTESIAN_POINT('Ctrl Pts',(-20.1971584545413,25.2680560306668,122.474694751445)) ;
#82737=CARTESIAN_POINT('Ctrl Pts',(-20.4241107571781,25.284662453801,122.745253295824)) ;
#82738=CARTESIAN_POINT('Ctrl Pts',(-20.5421825344432,25.2979586742967,122.998571370006)) ;
#82739=CARTESIAN_POINT('Ctrl Pts',(-20.6149656243915,25.3112275066382,123.267944727549)) ;
#82740=CARTESIAN_POINT('Ctrl Pts',(-20.6152703491861,25.3279187546713,123.62274741247)) ;
#82741=CARTESIAN_POINT('Ctrl Pts',(-20.4723050652647,25.3477284863441,124.019012656486)) ;
#82742=CARTESIAN_POINT('Ctrl Pts',(-20.2011038052829,25.3677060936726,124.345923721756)) ;
#82743=CARTESIAN_POINT('Ctrl Pts',(-19.8352019120776,25.3876324027305,124.559424851809)) ;
#82744=CARTESIAN_POINT('Ctrl Pts',(-19.4208025912353,25.4074492628952,124.636316300838)) ;
#82745=CARTESIAN_POINT('Ctrl Pts',(-18.9994694110562,25.4275490784892,124.56558046184)) ;
#82746=CARTESIAN_POINT('Ctrl Pts',(-18.6335309608518,25.4473060423717,124.358919220961)) ;
#82747=CARTESIAN_POINT('Ctrl Pts',(-18.3557823809738,25.4673429684412,124.036055619481)) ;
#82748=CARTESIAN_POINT('Ctrl Pts',(-18.2066757307838,25.4872125508227,123.640645139258)) ;
#82749=CARTESIAN_POINT('Ctrl Pts',(-18.2003787294005,25.5071171225759,123.217548778513)) ;
#82750=CARTESIAN_POINT('Ctrl Pts',(-18.3392640178439,25.5270697247744,122.816604069234)) ;
#82751=CARTESIAN_POINT('Ctrl Pts',(-18.6060642919708,25.5469792157446,122.488044084388)) ;
#82752=CARTESIAN_POINT('Ctrl Pts',(-18.9674597166613,25.5668305844441,122.269771258974)) ;
#82753=CARTESIAN_POINT('Ctrl Pts',(-19.3863524336457,25.5869107805801,122.187636260904)) ;
#82754=CARTESIAN_POINT('Ctrl Pts',(-19.8024618699774,25.6067117241555,122.252489134257)) ;
#82755=CARTESIAN_POINT('Ctrl Pts',(-20.1751760188317,25.626695700665,122.456396660156)) ;
#82756=CARTESIAN_POINT('Ctrl Pts',(-20.4545282376597,25.6466116636406,122.774650868096)) ;
#82757=CARTESIAN_POINT('Ctrl Pts',(-20.6092750951516,25.6664820984625,123.167879992123)) ;
#82758=CARTESIAN_POINT('Ctrl Pts',(-20.619928125435,25.6865323836956,123.5939462739)) ;
#82759=CARTESIAN_POINT('Ctrl Pts',(-20.486892040256,25.7063063524549,123.992971139945)) ;
#82760=CARTESIAN_POINT('Ctrl Pts',(-20.2223888179771,25.7263628105744,124.3272695752)) ;
#82761=CARTESIAN_POINT('Ctrl Pts',(-19.8640907327752,25.7461576935654,124.548347804245)) ;
#82762=CARTESIAN_POINT('Ctrl Pts',(-19.4487334488014,25.7661243488678,124.635759281327)) ;
#82763=CARTESIAN_POINT('Ctrl Pts',(-19.0285707776427,25.7860833189443,124.57548876472)) ;
#82764=CARTESIAN_POINT('Ctrl Pts',(-18.6553224410746,25.8059794065344,124.376406038216)) ;
#82765=CARTESIAN_POINT('Ctrl Pts',(-18.3720204939912,25.825877576446,124.062217957459)) ;
#82766=CARTESIAN_POINT('Ctrl Pts',(-18.2124360297774,25.8457834118131,123.670170482707)) ;
#82767=CARTESIAN_POINT('Ctrl Pts',(-18.1961936546643,25.865733336751,123.246330110804)) ;
#82768=CARTESIAN_POINT('Ctrl Pts',(-18.3247479467419,25.8856125266614,122.843621262067)) ;
#82769=CARTESIAN_POINT('Ctrl Pts',(-18.5841089761526,25.905593850942,122.507162548675)) ;
#82770=CARTESIAN_POINT('Ctrl Pts',(-18.9420162535925,25.9255236351503,122.280112542374)) ;
#82771=CARTESIAN_POINT('Ctrl Pts',(-19.355512500182,25.9454436245411,122.188825953052)) ;
#82772=CARTESIAN_POINT('Ctrl Pts',(-19.7742961210267,25.9652988198951,122.243020652397)) ;
#82773=CARTESIAN_POINT('Ctrl Pts',(-20.1526865313049,25.9853448215545,122.439009324516)) ;
#82774=CARTESIAN_POINT('Ctrl Pts',(-20.390612650393,26.0018445687643,122.696940363315)) ;
#82775=CARTESIAN_POINT('Ctrl Pts',(-20.5216824453276,26.0152331732124,122.946016191372)) ;
#82776=CARTESIAN_POINT('Ctrl Pts',(-20.5849012114667,26.0250950015473,123.143472116702)) ;
#82777=CARTESIAN_POINT('Ctrl Pts',(-20.6138255653156,26.0350611443048,123.351002200631)) ;
#82778=CARTESIAN_POINT('Ctrl Pts',(-20.6032059167686,26.0484228904298,123.631608353229)) ;
#82779=CARTESIAN_POINT('Ctrl Pts',(-20.5008843919957,26.0648772193849,123.966371529301)) ;
#82780=CARTESIAN_POINT('Ctrl Pts',(-20.2867255145907,26.0816444644332,124.251158212897)) ;
#82781=CARTESIAN_POINT('Ctrl Pts',(-20.0681057939674,26.0948310297072,124.421840339604)) ;
#82782=CARTESIAN_POINT('Ctrl Pts',(-19.8829958353414,26.1048204884518,124.520903003192)) ;
#82783=CARTESIAN_POINT('Ctrl Pts',(-19.6841239965598,26.1147742609329,124.586158608731)) ;
#82784=CARTESIAN_POINT('Ctrl Pts',(-19.4750313009823,26.1248220774656,124.615997658308)) ;
#82785=CARTESIAN_POINT('Ctrl Pts',(-19.268213655038,26.1346636105881,124.609461722499)) ;
#82786=CARTESIAN_POINT('Ctrl Pts',(-19.0626573797531,26.1446498528078,124.566942370509)) ;
#82787=CARTESIAN_POINT('Ctrl Pts',(-18.8684723237742,26.1545864762327,124.489834641604)) ;
#82788=CARTESIAN_POINT('Ctrl Pts',(-18.6887022886735,26.1646363536156,124.378870956204)) ;
#82789=CARTESIAN_POINT('Ctrl Pts',(-18.5339300885659,26.1744867923932,124.241258963112)) ;
#82790=CARTESIAN_POINT('Ctrl Pts',(-18.4034137260128,26.1844588063619,124.077232557393)) ;
#82791=CARTESIAN_POINT('Ctrl Pts',(-18.3031245373039,26.1944539749881,123.892541814178)) ;
#82792=CARTESIAN_POINT('Ctrl Pts',(-18.2364238757988,26.2044878582493,123.692438349081)) ;
#82793=CARTESIAN_POINT('Ctrl Pts',(-18.2057140200122,26.2143437283126,123.487510340136)) ;
#82794=CARTESIAN_POINT('Ctrl Pts',(-18.2107938710183,26.2243412742298,123.277414606972)) ;
#82795=CARTESIAN_POINT('Ctrl Pts',(-18.2518456721577,26.234249401129,123.073191376682)) ;
#82796=CARTESIAN_POINT('Ctrl Pts',(-18.3281770957647,26.2442597726512,122.8770614784)) ;
#82797=CARTESIAN_POINT('Ctrl Pts',(-18.4380159389114,26.2542902153986,122.697063925177)) ;
#82798=CARTESIAN_POINT('Ctrl Pts',(-18.5745552026189,26.2641381679519,122.541414211324)) ;
#82799=CARTESIAN_POINT('Ctrl Pts',(-18.7394363077977,26.2742008369729,122.408905152099)) ;
#82800=CARTESIAN_POINT('Ctrl Pts',(-18.921826397574,26.2840952124368,122.30885227749)) ;
#82801=CARTESIAN_POINT('Ctrl Pts',(-19.1195394226765,26.2940370107549,122.241151657766)) ;
#82802=CARTESIAN_POINT('Ctrl Pts',(-19.3273054139925,26.3040395044822,122.208523084326)) ;
#82803=CARTESIAN_POINT('Ctrl Pts',(-19.5382116556896,26.3140743029892,122.212809760869)) ;
#82804=CARTESIAN_POINT('Ctrl Pts',(-19.7413463318015,26.3239191869685,122.252542608404)) ;
#82805=CARTESIAN_POINT('Ctrl Pts',(-19.9373601105037,26.3339050437866,122.327621631711)) ;
#82806=CARTESIAN_POINT('Ctrl Pts',(-20.1165785345523,26.3438398579613,122.434952365593)) ;
#82807=CARTESIAN_POINT('Ctrl Pts',(-20.2762122406521,26.3538973577467,122.57355737854)) ;
#82808=CARTESIAN_POINT('Ctrl Pts',(-20.4065114699198,26.363719116165,122.733766867349)) ;
#82809=CARTESIAN_POINT('Ctrl Pts',(-20.5097347077751,26.373774773949,122.91823428775)) ;
#82810=CARTESIAN_POINT('Ctrl Pts',(-20.5782258754457,26.383716956129,123.11572137009)) ;
#82811=CARTESIAN_POINT('Ctrl Pts',(-20.611887127279,26.3936221648237,123.321218154667)) ;
#82812=CARTESIAN_POINT('Ctrl Pts',(-20.6092537918309,26.4036639557861,123.532308255734)) ;
#82813=CARTESIAN_POINT('Ctrl Pts',(-20.5705521085007,26.4135717302584,123.736982032277)) ;
#82814=CARTESIAN_POINT('Ctrl Pts',(-20.4964939722591,26.423583230486,123.934001629512)) ;
#82815=CARTESIAN_POINT('Ctrl Pts',(-20.3887491018075,26.4336159908787,124.115324540984)) ;
#82816=CARTESIAN_POINT('Ctrl Pts',(-20.2539283340151,26.4434665600136,124.272523602686)) ;
#82817=CARTESIAN_POINT('Ctrl Pts',(-20.0918867892734,26.4534551695435,124.406059625645)) ;
#82818=CARTESIAN_POINT('Ctrl Pts',(-19.9101964278376,26.4633838255676,124.508820930747)) ;
#82819=CARTESIAN_POINT('Ctrl Pts',(-19.7123664532002,26.4733715717454,124.579225540424)) ;
#82820=CARTESIAN_POINT('Ctrl Pts',(-19.5042772626285,26.4834075606811,124.614026057559)) ;
#82821=CARTESIAN_POINT('Ctrl Pts',(-19.2970856363154,26.4932624304947,124.612543958121)) ;
#82822=CARTESIAN_POINT('Ctrl Pts',(-19.0903087732055,26.5032618717365,124.574850514142)) ;
#82823=CARTESIAN_POINT('Ctrl Pts',(-18.8951319150959,26.5131569459166,124.502774164513)) ;
#82824=CARTESIAN_POINT('Ctrl Pts',(-18.7124927509316,26.5232176017563,124.396160185279)) ;
#82825=CARTESIAN_POINT('Ctrl Pts',(-18.5544270389059,26.5330664759519,124.262395151652)) ;
#82826=CARTESIAN_POINT('Ctrl Pts',(-18.4191734787532,26.5430951879151,124.100664920014)) ;
#82827=CARTESIAN_POINT('Ctrl Pts',(-18.3145428642339,26.5531245884982,123.917602937838)) ;
#82828=CARTESIAN_POINT('Ctrl Pts',(-18.2441983040916,26.5629647821151,123.723055464282)) ;
#82829=CARTESIAN_POINT('Ctrl Pts',(-18.2077335903667,26.5729682046903,123.515958814128)) ;
#82830=CARTESIAN_POINT('Ctrl Pts',(-18.207849921292,26.5829537417834,123.305996098969)) ;
#82831=CARTESIAN_POINT('Ctrl Pts',(-18.2448224488325,26.5929947462702,123.098185943807)) ;
#82832=CARTESIAN_POINT('Ctrl Pts',(-18.3156375537416,26.6028382852114,122.90372091966)) ;
#82833=CARTESIAN_POINT('Ctrl Pts',(-18.420226223306,26.6128233162022,122.721750391998)) ;
#82834=CARTESIAN_POINT('Ctrl Pts',(-18.5541826435393,26.6227627787242,122.561338902929)) ;
#82835=CARTESIAN_POINT('Ctrl Pts',(-18.7155638287665,26.632802510948,122.425330530865)) ;
#82836=CARTESIAN_POINT('Ctrl Pts',(-18.8953261605119,26.6426906912652,122.320904791171)) ;
#82837=CARTESIAN_POINT('Ctrl Pts',(-19.0923360261154,26.6526802069677,122.248179866433)) ;
#82838=CARTESIAN_POINT('Ctrl Pts',(-19.2983696770575,26.6626387576224,122.211042571254)) ;
#82839=CARTESIAN_POINT('Ctrl Pts',(-19.5064961437083,26.6725381647274,122.209729675331)) ;
#82840=CARTESIAN_POINT('Ctrl Pts',(-19.71472754712,26.6825867511437,122.245179243824)) ;
#82841=CARTESIAN_POINT('Ctrl Pts',(-19.9106882517753,26.6924795701081,122.314976938035)) ;
#82842=CARTESIAN_POINT('Ctrl Pts',(-20.0947008341311,26.7025506876379,122.419616599627)) ;
#82843=CARTESIAN_POINT('Ctrl Pts',(-20.2538532375806,26.712366381604,122.551030478766)) ;
#82844=CARTESIAN_POINT('Ctrl Pts',(-20.3913677952363,26.7224327591013,122.711830832678)) ;
#82845=CARTESIAN_POINT('Ctrl Pts',(-20.4970805265388,26.7323317451832,122.891149607162)) ;
#82846=CARTESIAN_POINT('Ctrl Pts',(-20.5712377391384,26.7423859251767,123.089035348672)) ;
#82847=CARTESIAN_POINT('Ctrl Pts',(-20.6094217290172,26.7522567381094,123.293057137242)) ;
#82848=CARTESIAN_POINT('Ctrl Pts',(-20.6116385923756,26.7623306389632,123.504781122853)) ;
#82849=CARTESIAN_POINT('Ctrl Pts',(-20.578165667762,26.7721507943498,123.708548577239)) ;
#82850=CARTESIAN_POINT('Ctrl Pts',(-20.5082435307415,26.7822295013021,123.908510180151)) ;
#82851=CARTESIAN_POINT('Ctrl Pts',(-20.4070109643156,26.7920810898409,124.089251320675)) ;
#82852=CARTESIAN_POINT('Ctrl Pts',(-20.2731855773229,26.8021542063659,124.253326774915)) ;
#82853=CARTESIAN_POINT('Ctrl Pts',(-20.1165101097309,26.8119967234617,124.388517173998)) ;
#82854=CARTESIAN_POINT('Ctrl Pts',(-19.9366356777944,26.8219771850156,124.496525247979)) ;
#82855=CARTESIAN_POINT('Ctrl Pts',(-19.7398462584671,26.8319954350064,124.57156869515)) ;
#82856=CARTESIAN_POINT('Ctrl Pts',(-19.5358433260639,26.8418795952002,124.61119618925)) ;
#82857=CARTESIAN_POINT('Ctrl Pts',(-19.3242969450418,26.8519447421752,124.614819303363)) ;
#82858=CARTESIAN_POINT('Ctrl Pts',(-19.1199162618972,26.861786565816,124.582500420025)) ;
#82859=CARTESIAN_POINT('Ctrl Pts',(-18.9203548754396,26.8718160382768,124.514444221525)) ;
#82860=CARTESIAN_POINT('Ctrl Pts',(-18.7359669740694,26.8818428935388,124.412277169318)) ;
#82861=CARTESIAN_POINT('Ctrl Pts',(-18.5748099018744,26.8916861436494,124.282461811643)) ;
#82862=CARTESIAN_POINT('Ctrl Pts',(-18.4355916287619,26.9017345832325,124.123583549416)) ;
#82863=CARTESIAN_POINT('Ctrl Pts',(-18.3274329259316,26.9116840774804,123.944547242474)) ;
#82864=CARTESIAN_POINT('Ctrl Pts',(-18.2517329022827,26.9215919332064,123.750483492684)) ;
#82865=CARTESIAN_POINT('Ctrl Pts',(-18.210480034894,26.9316514098564,123.543086574013)) ;
#82866=CARTESIAN_POINT('Ctrl Pts',(-18.2056838568797,26.9414922192651,123.33623203913)) ;
#82867=CARTESIAN_POINT('Ctrl Pts',(-18.2373097308937,26.9515543695659,123.127093653458)) ;
#82868=CARTESIAN_POINT('Ctrl Pts',(-18.3038768892104,26.9614515306884,122.929948768524)) ;
#82869=CARTESIAN_POINT('Ctrl Pts',(-18.403389671936,26.9713827050925,122.746410731173)) ;
#82870=CARTESIAN_POINT('Ctrl Pts',(-18.5348933081084,26.9814249088175,122.581254032342)) ;
#82871=CARTESIAN_POINT('Ctrl Pts',(-18.6905332850335,26.9913114912479,122.443483739432)) ;
#82872=CARTESIAN_POINT('Ctrl Pts',(-18.8694457274301,27.0013049269963,122.333371768838)) ;
#82873=CARTESIAN_POINT('Ctrl Pts',(-19.0638389728186,27.0112493953544,122.256431782156)) ;
#82874=CARTESIAN_POINT('Ctrl Pts',(-19.2687173761859,27.0212012116,122.213994239668)) ;
#82875=CARTESIAN_POINT('Ctrl Pts',(-19.4796376595632,27.0312386477145,122.207914896292)) ;
#82876=CARTESIAN_POINT('Ctrl Pts',(-19.6852953955237,27.0411236068908,122.237889880641)) ;
#82877=CARTESIAN_POINT('Ctrl Pts',(-19.8849208638732,27.0511217251028,122.303615150814)) ;
#82878=CARTESIAN_POINT('Ctrl Pts',(-20.0687824125727,27.0610426576147,122.402131159829)) ;
#82879=CARTESIAN_POINT('Ctrl Pts',(-20.2347433918381,27.0710839578368,122.532576220351)) ;
#82880=CARTESIAN_POINT('Ctrl Pts',(-20.3736041394949,27.0809908762268,122.687807501135)) ;
#82881=CARTESIAN_POINT('Ctrl Pts',(-20.4842302839769,27.0909266679358,122.864990331019)) ;
#82882=CARTESIAN_POINT('Ctrl Pts',(-20.5630380544402,27.1009675625137,123.060813866335)) ;
#82883=CARTESIAN_POINT('Ctrl Pts',(-20.6061312160508,27.1108547642276,123.264168808546)) ;
#82884=CARTESIAN_POINT('Ctrl Pts',(-20.6136841214982,27.1208470319892,123.474087454112)) ;
#82885=CARTESIAN_POINT('Ctrl Pts',(-20.5847396470279,27.130795553011,123.681235938774)) ;
#82886=CARTESIAN_POINT('Ctrl Pts',(-20.5206329047438,27.1407323265887,123.880040230082)) ;
#82887=CARTESIAN_POINT('Ctrl Pts',(-20.4227398930541,27.1507153747297,124.065715829988)) ;
#82888=CARTESIAN_POINT('Ctrl Pts',(-20.2930387357381,27.1607590823398,124.232307363465)) ;
#82889=CARTESIAN_POINT('Ctrl Pts',(-20.1400188875306,27.1705877754931,124.371201746397)) ;
#82890=CARTESIAN_POINT('Ctrl Pts',(-19.9609581955699,27.1806625246225,124.484270421944)) ;
#82891=CARTESIAN_POINT('Ctrl Pts',(-19.7689924114484,27.1905278504181,124.562839081487)) ;
#82892=CARTESIAN_POINT('Ctrl Pts',(-19.5632221468659,27.200550024775,124.608103782849)) ;
#82893=CARTESIAN_POINT('Ctrl Pts',(-19.352593328768,27.2105760779819,124.616438890928)) ;
#82894=CARTESIAN_POINT('Ctrl Pts',(-19.1472929985065,27.2204297748282,124.58889990198)) ;
#82895=CARTESIAN_POINT('Ctrl Pts',(-18.94756230638,27.2303891795812,124.526053160044)) ;
#82896=CARTESIAN_POINT('Ctrl Pts',(-18.7604972958979,27.2404274252861,124.428392109811)) ;
#82897=CARTESIAN_POINT('Ctrl Pts',(-18.5957070248986,27.2503016094481,124.302108734558)) ;
#82898=CARTESIAN_POINT('Ctrl Pts',(-18.4526111915143,27.260371392586,124.146135557906)) ;
#82899=CARTESIAN_POINT('Ctrl Pts',(-18.3413269156734,27.2702046476068,123.971898769522)) ;
#82900=CARTESIAN_POINT('Ctrl Pts',(-18.2598539322131,27.2802350737385,123.777409894901)) ;
#82901=CARTESIAN_POINT('Ctrl Pts',(-18.2139770900648,27.2902666859255,123.571552166036)) ;
#82902=CARTESIAN_POINT('Ctrl Pts',(-18.204301463541,27.3000963827801,123.36514186041)) ;
#82903=CARTESIAN_POINT('Ctrl Pts',(-18.2304203551583,27.3100858246826,123.156756796633)) ;
#82904=CARTESIAN_POINT('Ctrl Pts',(-18.2931717693521,27.3201297166982,122.955144101719)) ;
#82905=CARTESIAN_POINT('Ctrl Pts',(-18.387455169837,27.3299512784675,122.771448979149)) ;
#82906=CARTESIAN_POINT('Ctrl Pts',(-18.5145023629227,27.3399868500917,122.603007681867)) ;
#82907=CARTESIAN_POINT('Ctrl Pts',(-18.6691989465435,27.3500161243735,122.459740103133)) ;
#82908=CARTESIAN_POINT('Ctrl Pts',(-18.8426716693766,27.3598499614921,122.347266608957)) ;
#82909=CARTESIAN_POINT('Ctrl Pts',(-19.0371543589241,27.3699023575803,122.264600969507)) ;
#82910=CARTESIAN_POINT('Ctrl Pts',(-19.2407489259686,27.3798391245308,122.217766395529)) ;
#82911=CARTESIAN_POINT('Ctrl Pts',(-19.4492892687206,27.3897733595101,122.206457881068)) ;
#82912=CARTESIAN_POINT('Ctrl Pts',(-19.6584787766812,27.3997971228369,122.231885053703)) ;
#82913=CARTESIAN_POINT('Ctrl Pts',(-19.8573566517877,27.4096834642215,122.292260660859)) ;
#82914=CARTESIAN_POINT('Ctrl Pts',(-20.0448842456016,27.4196725129885,122.386795149275)) ;
#82915=CARTESIAN_POINT('Ctrl Pts',(-20.2137587561122,27.4297137336859,122.513457846421)) ;
#82916=CARTESIAN_POINT('Ctrl Pts',(-20.3553226212523,27.4395463738638,122.664084462041)) ;
#82917=CARTESIAN_POINT('Ctrl Pts',(-20.4709452089178,27.4495403031717,122.839511285258)) ;
#82918=CARTESIAN_POINT('Ctrl Pts',(-20.5542369544809,27.4595695108523,123.033209537113)) ;
#82919=CARTESIAN_POINT('Ctrl Pts',(-20.6022223083643,27.4694453225564,123.235220662099)) ;
#82920=CARTESIAN_POINT('Ctrl Pts',(-20.6147833777703,27.4794445495278,123.44503211102)) ;
#82921=CARTESIAN_POINT('Ctrl Pts',(-20.5911307346589,27.4893540306835,123.652044209463)) ;
#82922=CARTESIAN_POINT('Ctrl Pts',(-20.5310228627754,27.4994072609844,123.854644058628)) ;
#82923=CARTESIAN_POINT('Ctrl Pts',(-20.4384382046183,27.5092778775354,124.040371920306)) ;
#82924=CARTESIAN_POINT('Ctrl Pts',(-20.3135085837969,27.5192995392675,124.210019678146)) ;
#82925=CARTESIAN_POINT('Ctrl Pts',(-20.160659918999,27.5293223524486,124.355074881809)) ;
#82926=CARTESIAN_POINT('Ctrl Pts',(-19.9878844387266,27.5391895169085,124.469859474152)) ;
#82927=CARTESIAN_POINT('Ctrl Pts',(-19.7955494051919,27.5491829591284,124.554411461735)) ;
#82928=CARTESIAN_POINT('Ctrl Pts',(-19.5905834066282,27.5592146327288,124.604073130056)) ;
#82929=CARTESIAN_POINT('Ctrl Pts',(-19.3835855603672,27.5690810678418,124.617490990063)) ;
#82930=CARTESIAN_POINT('Ctrl Pts',(-19.174870131399,27.5790685183749,124.59482811783)) ;
#82931=CARTESIAN_POINT('Ctrl Pts',(-18.974033313999,27.5890134482028,124.536610658265)) ;
#82932=CARTESIAN_POINT('Ctrl Pts',(-18.784566926627,27.5990583432579,124.443394511315)) ;
#82933=CARTESIAN_POINT('Ctrl Pts',(-18.6171298669107,27.6089204049438,124.321093519021)) ;
#82934=CARTESIAN_POINT('Ctrl Pts',(-18.4713021073392,27.6189121277306,124.169926560183)) ;
#82935=CARTESIAN_POINT('Ctrl Pts',(-18.3546885614246,27.6288443419706,123.996714392999)) ;
#82936=CARTESIAN_POINT('Ctrl Pts',(-18.2694196513225,27.6387836605363,123.805941878918)) ;
#82937=CARTESIAN_POINT('Ctrl Pts',(-18.218224017845,27.6488278353122,123.601084916452)) ;
#82938=CARTESIAN_POINT('Ctrl Pts',(-18.2035200669392,27.6586983893772,123.394096892666)) ;
#82939=CARTESIAN_POINT('Ctrl Pts',(-18.2245812237522,27.6686633717313,123.185662506194)) ;
#82940=CARTESIAN_POINT('Ctrl Pts',(-18.2821983595158,27.6786940746212,122.982815613202)) ;
#82941=CARTESIAN_POINT('Ctrl Pts',(-18.3726338777417,27.6885864146464,122.795512202132)) ;
#82942=CARTESIAN_POINT('Ctrl Pts',(-18.4961446567781,27.6986396478063,122.62404318365)) ;
#82943=CARTESIAN_POINT('Ctrl Pts',(-18.6449200835009,27.7085208922831,122.479010016898)) ;
#82944=CARTESIAN_POINT('Ctrl Pts',(-18.8191075113425,27.7185540131541,122.360127402557)) ;
#82945=CARTESIAN_POINT('Ctrl Pts',(-19.008374966413,27.7284352234292,122.274409098091)) ;
#82946=CARTESIAN_POINT('Ctrl Pts',(-19.2132499111456,27.7384972991985,122.221874642393)) ;
#82947=CARTESIAN_POINT('Ctrl Pts',(-19.4198941418905,27.7483543575803,122.205962713999)) ;
#82948=CARTESIAN_POINT('Ctrl Pts',(-19.6290171196823,27.7583489128693,122.226026761165)) ;
#82949=CARTESIAN_POINT('Ctrl Pts',(-19.830168372801,27.7682748004048,122.281656744792)) ;
#82950=CARTESIAN_POINT('Ctrl Pts',(-20.0204729078967,27.7782998204,122.372190057432)) ;
#82951=CARTESIAN_POINT('Ctrl Pts',(-20.1900415778749,27.7881971975037,122.492787694309)) ;
#82952=CARTESIAN_POINT('Ctrl Pts',(-20.3377913724602,27.7981874345846,122.642064148753)) ;
#82953=CARTESIAN_POINT('Ctrl Pts',(-20.4575937503346,27.8082240473934,122.815752536172)) ;
#82954=CARTESIAN_POINT('Ctrl Pts',(-20.544094957431,27.8180739308114,123.003904294989)) ;
#82955=CARTESIAN_POINT('Ctrl Pts',(-20.5978342516824,27.8280775477138,123.20720838406)) ;
#82956=CARTESIAN_POINT('Ctrl Pts',(-20.6153219996542,27.838066959479,123.416522180099)) ;
#82957=CARTESIAN_POINT('Ctrl Pts',(-20.5960192166938,27.8480857208238,123.626239400183)) ;
#82958=CARTESIAN_POINT('Ctrl Pts',(-20.5232688311072,27.8613043962049,123.89449979669)) ;
#82959=CARTESIAN_POINT('Ctrl Pts',(-20.3813539781269,27.8746147034496,124.139307969047)) ;
#82960=CARTESIAN_POINT('Ctrl Pts',(-20.184222532259,27.8878523696756,124.335730450596)) ;
#82961=CARTESIAN_POINT('Ctrl Pts',(-20.0135550690303,27.8977720650863,124.45559246094)) ;
#82962=CARTESIAN_POINT('Ctrl Pts',(-19.8220508423892,27.9078249320848,124.544956156346)) ;
#82963=CARTESIAN_POINT('Ctrl Pts',(-19.6219767232522,27.9176803404141,124.598870292212)) ;
#82964=CARTESIAN_POINT('Ctrl Pts',(-19.4118115423759,27.9277189720907,124.617912531858)) ;
#82965=CARTESIAN_POINT('Ctrl Pts',(-19.1331436916363,27.9410211543577,124.594057320696)) ;
#82966=CARTESIAN_POINT('Ctrl Pts',(-18.8021121159466,27.9575661674406,124.475054043175)) ;
#82967=CARTESIAN_POINT('Ctrl Pts',(-18.5297401860013,27.9742181835168,124.248816186926)) ;
#82968=CARTESIAN_POINT('Ctrl Pts',(-18.3691043653144,27.987441274422,124.021959245793)) ;
#82969=CARTESIAN_POINT('Ctrl Pts',(-18.279074783477,27.9974022339814,123.832881356621)) ;
#82970=CARTESIAN_POINT('Ctrl Pts',(-18.2231429975512,28.0074270307325,123.629695199133)) ;
#82971=CARTESIAN_POINT('Ctrl Pts',(-18.1966274923705,28.0206514781283,123.352901461679)) ;
#82972=CARTESIAN_POINT('Ctrl Pts',(-18.2547427005857,28.0372852628274,123.004090417878)) ;
#82973=CARTESIAN_POINT('Ctrl Pts',(-18.4626541562344,28.0571879295523,122.635456474346)) ;
#82974=CARTESIAN_POINT('Ctrl Pts',(-18.7834264089108,28.0770881573342,122.35955622577)) ;
#82975=CARTESIAN_POINT('Ctrl Pts',(-19.179357615155,28.0970056448657,122.20926617617)) ;
#82976=CARTESIAN_POINT('Ctrl Pts',(-19.6030850730905,28.1169351706826,122.202842194496)) ;
#82977=CARTESIAN_POINT('Ctrl Pts',(-20.0042033525094,28.1368974385688,122.341703258092)) ;
#82978=CARTESIAN_POINT('Ctrl Pts',(-20.3326268321142,28.156787633521,122.608069857982)) ;
#82979=CARTESIAN_POINT('Ctrl Pts',(-20.5514322742889,28.1766778782673,122.9700984434)) ;
#82980=CARTESIAN_POINT('Ctrl Pts',(-20.6334273789311,28.1967522508298,123.388925899664)) ;
#82981=CARTESIAN_POINT('Ctrl Pts',(-20.5686426235298,28.2165376281901,123.804655209976)) ;
#82982=CARTESIAN_POINT('Ctrl Pts',(-20.3652778683003,28.2364995022572,124.177163703848)) ;
#82983=CARTESIAN_POINT('Ctrl Pts',(-20.0460051045629,28.2564794777477,124.457438441996)) ;
#82984=CARTESIAN_POINT('Ctrl Pts',(-19.653857904935,28.2762919076256,124.611414371596)) ;
#82985=CARTESIAN_POINT('Ctrl Pts',(-19.2292624618467,28.2962720157159,124.622968506333)) ;
#82986=CARTESIAN_POINT('Ctrl Pts',(-18.8278348153005,28.3161663993132,124.489281226312)) ;
#82987=CARTESIAN_POINT('Ctrl Pts',(-18.4954922096611,28.3360933272904,124.226621143619)) ;
#82988=CARTESIAN_POINT('Ctrl Pts',(-18.2725085979326,28.3559881845916,123.867030766251)) ;
#82989=CARTESIAN_POINT('Ctrl Pts',(-18.1854382364504,28.3760273781953,123.44997732498)) ;
#82990=CARTESIAN_POINT('Ctrl Pts',(-18.2454140746476,28.395867346106,123.032367008361)) ;
#82991=CARTESIAN_POINT('Ctrl Pts',(-18.4440437795509,28.4157821630701,122.658441102044)) ;
#82992=CARTESIAN_POINT('Ctrl Pts',(-18.7589841342305,28.4357244084664,122.374569023093)) ;
#82993=CARTESIAN_POINT('Ctrl Pts',(-19.1503541669098,28.4555964565809,122.215058285885)) ;
#82994=CARTESIAN_POINT('Ctrl Pts',(-19.5753981818252,28.475607521535,122.198881824646)) ;
#82995=CARTESIAN_POINT('Ctrl Pts',(-19.9769247208087,28.4954190458386,122.326892941792)) ;
#82996=CARTESIAN_POINT('Ctrl Pts',(-20.3149985662992,28.515514257802,122.587908802987)) ;
#82997=CARTESIAN_POINT('Ctrl Pts',(-20.5402449088348,28.5352949817218,122.943300074454)) ;
#82998=CARTESIAN_POINT('Ctrl Pts',(-20.6325412092939,28.5552860573646,123.358060870925)) ;
#82999=CARTESIAN_POINT('Ctrl Pts',(-20.5777380109827,28.5751679964076,123.777357890785)) ;
#83000=CARTESIAN_POINT('Ctrl Pts',(-20.3829565395105,28.5951206009108,124.154169126176)) ;
#83001=CARTESIAN_POINT('Ctrl Pts',(-20.0720353336252,28.6150194696415,124.441191742656)) ;
#83002=CARTESIAN_POINT('Ctrl Pts',(-19.6822522085535,28.6349128694511,124.605274921211)) ;
#83003=CARTESIAN_POINT('Ctrl Pts',(-19.2594120114922,28.6548220002911,124.627173959621)) ;
#83004=CARTESIAN_POINT('Ctrl Pts',(-18.8522721728086,28.6748541000547,124.502181189478)) ;
#83005=CARTESIAN_POINT('Ctrl Pts',(-18.5715057730066,28.6913861732241,124.290597833785)) ;
#83006=CARTESIAN_POINT('Ctrl Pts',(-18.3986990200904,28.7047215138301,124.069861172508)) ;
#83007=CARTESIAN_POINT('Ctrl Pts',(-18.3010384496953,28.7145640723698,123.887414318719)) ;
#83008=CARTESIAN_POINT('Ctrl Pts',(-18.2349738172095,28.7246159792197,123.686701717407)) ;
#83009=CARTESIAN_POINT('Ctrl Pts',(-18.1952065179791,28.7378644936106,123.411043235738)) ;
#83010=CARTESIAN_POINT('Ctrl Pts',(-18.2364118977493,28.7544636685583,123.060489190664)) ;
#83011=CARTESIAN_POINT('Ctrl Pts',(-18.3945321166907,28.7710524543534,122.745246203248)) ;
#83012=CARTESIAN_POINT('Ctrl Pts',(-18.5797842873954,28.7843282706954,122.536445736904)) ;
#83013=CARTESIAN_POINT('Ctrl Pts',(-18.7438859265167,28.7943021214892,122.405910579741)) ;
#83014=CARTESIAN_POINT('Ctrl Pts',(-18.9292775365355,28.8043311535816,122.305499209113)) ;
#83015=CARTESIAN_POINT('Ctrl Pts',(-19.1264646932159,28.8142212790835,122.239514293344)) ;
#83016=CARTESIAN_POINT('Ctrl Pts',(-19.3341633145433,28.824213757355,122.208177518519)) ;
#83017=CARTESIAN_POINT('Ctrl Pts',(-19.5433408860057,28.8341649724524,122.213247360527)) ;
#83018=CARTESIAN_POINT('Ctrl Pts',(-19.7503772801932,28.8442134742074,122.255121662075)) ;
#83019=CARTESIAN_POINT('Ctrl Pts',(-19.9430718587328,28.8540548238242,122.330508467652)) ;
#83020=CARTESIAN_POINT('Ctrl Pts',(-20.1225389719754,28.8640411148444,122.43938139671)) ;
#83021=CARTESIAN_POINT('Ctrl Pts',(-20.2797113936261,28.873977726573,122.577040956257)) ;
#83022=CARTESIAN_POINT('Ctrl Pts',(-20.4119681738559,28.8840276019406,122.741778191217)) ;
#83023=CARTESIAN_POINT('Ctrl Pts',(-20.5117487555868,28.893878060476,122.923259385367)) ;
#83024=CARTESIAN_POINT('Ctrl Pts',(-20.5798319599895,28.9038499974288,123.121510222702)) ;
#83025=CARTESIAN_POINT('Ctrl Pts',(-20.6125111693682,28.9138454543609,123.329122115711)) ;
#83026=CARTESIAN_POINT('Ctrl Pts',(-20.6083934061051,28.923878261414,123.539989200486)) ;
#83027=CARTESIAN_POINT('Ctrl Pts',(-20.5686973010357,28.9337381480039,123.74344956962)) ;
#83028=CARTESIAN_POINT('Ctrl Pts',(-20.493679373233,28.9437272285692,123.939575692006)) ;
#83029=CARTESIAN_POINT('Ctrl Pts',(-20.3863550998014,28.9536587077783,124.118678011433)) ;
#83030=CARTESIAN_POINT('Ctrl Pts',(-20.249070224389,28.9636445672243,124.27752143985)) ;
#83031=CARTESIAN_POINT('Ctrl Pts',(-20.0852249936528,28.9736827178714,124.410502587285)) ;
#83032=CARTESIAN_POINT('Ctrl Pts',(-19.904447217627,28.9835308083759,124.511458793351)) ;
#83033=CARTESIAN_POINT('Ctrl Pts',(-19.7047579448723,28.9935917168938,124.581118061351)) ;
#83034=CARTESIAN_POINT('Ctrl Pts',(-19.4993889431451,29.0034865640518,124.614351432211)) ;
#83035=CARTESIAN_POINT('Ctrl Pts',(-19.2904222945581,29.0134282360969,124.611964719731)) ;
#83036=CARTESIAN_POINT('Ctrl Pts',(-19.0837191063688,29.0234307632223,124.573165462231)) ;
#83037=CARTESIAN_POINT('Ctrl Pts',(-18.8864144001065,29.0334655544098,124.498528920258)) ;
#83038=CARTESIAN_POINT('Ctrl Pts',(-18.7082976445877,29.0433104342689,124.393092631481)) ;
#83039=CARTESIAN_POINT('Ctrl Pts',(-18.5487226744575,29.0532963148874,124.256732103658)) ;
#83040=CARTESIAN_POINT('Ctrl Pts',(-18.4157694205225,29.0632310379806,124.095604648302)) ;
#83041=CARTESIAN_POINT('Ctrl Pts',(-18.3117412163871,29.0732888782918,123.91155389501)) ;
#83042=CARTESIAN_POINT('Ctrl Pts',(-18.2425809972532,29.0831093656883,123.716996801485)) ;
#83043=CARTESIAN_POINT('Ctrl Pts',(-18.2070771108362,29.0931697670334,123.508522429768)) ;
#83044=CARTESIAN_POINT('Ctrl Pts',(-18.2085773475788,29.1031007325863,123.299723943504)) ;
#83045=CARTESIAN_POINT('Ctrl Pts',(-18.2458733773094,29.1130395949228,123.094155479002)) ;
#83046=CARTESIAN_POINT('Ctrl Pts',(-18.3185218478309,29.123025325849,122.897169941289)) ;
#83047=CARTESIAN_POINT('Ctrl Pts',(-18.4248524145763,29.1330497112764,122.715235116205)) ;
#83048=CARTESIAN_POINT('Ctrl Pts',(-18.559295617884,29.1429529956297,122.55622987037)) ;
#83049=CARTESIAN_POINT('Ctrl Pts',(-18.7218419122943,29.1530130002077,122.420962440277)) ;
#83050=CARTESIAN_POINT('Ctrl Pts',(-18.9014185037897,29.1628562692768,122.318086410997)) ;
#83051=CARTESIAN_POINT('Ctrl Pts',(-19.0988343275783,29.1728468348845,122.246460342704)) ;
#83052=CARTESIAN_POINT('Ctrl Pts',(-19.3044348738419,29.1827749666633,122.210453577453)) ;
#83053=CARTESIAN_POINT('Ctrl Pts',(-19.5144210476911,29.1927628537442,122.210327948367)) ;
#83054=CARTESIAN_POINT('Ctrl Pts',(-19.722154657313,29.2027988033129,122.247189650964)) ;
#83055=CARTESIAN_POINT('Ctrl Pts',(-19.9168982115564,29.2126536896917,122.317939837635)) ;
#83056=CARTESIAN_POINT('Ctrl Pts',(-20.099129259896,29.2226531040396,122.422673271606)) ;
#83057=CARTESIAN_POINT('Ctrl Pts',(-20.2589220492417,29.2325482692301,122.555925374151)) ;
#83058=CARTESIAN_POINT('Ctrl Pts',(-20.3953335945201,29.242608587922,122.717517992467)) ;
#83059=CARTESIAN_POINT('Ctrl Pts',(-20.4995231362164,29.2524587196981,122.896499773068)) ;
#83060=CARTESIAN_POINT('Ctrl Pts',(-20.5728206243323,29.2624892901484,123.094215207785)) ;
#83061=CARTESIAN_POINT('Ctrl Pts',(-20.6101551347691,29.2725034408212,123.301419340689)) ;
#83062=CARTESIAN_POINT('Ctrl Pts',(-20.611271903258,29.2823963743666,123.509400284579)) ;
#83063=CARTESIAN_POINT('Ctrl Pts',(-20.5761577667123,29.2923858883568,123.716434470495)) ;
#83064=CARTESIAN_POINT('Ctrl Pts',(-20.505994801406,29.3023396590093,123.91361267384)) ;
#83065=CARTESIAN_POINT('Ctrl Pts',(-20.4015456777071,29.3123874276698,124.097194226307)) ;
#83066=CARTESIAN_POINT('Ctrl Pts',(-20.2697350753662,29.3222291541096,124.256700948655)) ;
#83067=CARTESIAN_POINT('Ctrl Pts',(-20.1102649351783,29.3322146709324,124.393174759304)) ;
#83068=CARTESIAN_POINT('Ctrl Pts',(-19.9303421124139,29.342154002628,124.499490590629)) ;
#83069=CARTESIAN_POINT('Ctrl Pts',(-19.7327438419793,29.3521937723255,124.573634332047)) ;
#83070=CARTESIAN_POINT('Ctrl Pts',(-19.5283969336439,29.3620819335743,124.611863917295)) ;
#83071=CARTESIAN_POINT('Ctrl Pts',(-19.318408138685,29.3720714880767,124.61444751305)) ;
#83072=CARTESIAN_POINT('Ctrl Pts',(-19.1118302786596,29.3820299026003,124.580478870266)) ;
#83073=CARTESIAN_POINT('Ctrl Pts',(-18.9152650511162,29.3919298154297,124.512040426744)) ;
#83074=CARTESIAN_POINT('Ctrl Pts',(-18.7309320391737,29.4019765150796,124.408967908519)) ;
#83075=CARTESIAN_POINT('Ctrl Pts',(-18.5695640054962,29.4118763753852,124.277476281909)) ;
#83076=CARTESIAN_POINT('Ctrl Pts',(-18.4313828878791,29.4219277795906,124.117644015429)) ;
#83077=CARTESIAN_POINT('Ctrl Pts',(-18.3247938273524,29.4318088165118,123.939309433569)) ;
#83078=CARTESIAN_POINT('Ctrl Pts',(-18.2496549022467,29.4418086486893,123.743005208198)) ;
#83079=CARTESIAN_POINT('Ctrl Pts',(-18.2098863976418,29.4517266516742,123.538288197709)) ;
#83080=CARTESIAN_POINT('Ctrl Pts',(-18.2062893419363,29.4617779575487,123.327044356571)) ;
#83081=CARTESIAN_POINT('Ctrl Pts',(-18.2385895959843,29.4716477809403,123.122034250536)) ;
#83082=CARTESIAN_POINT('Ctrl Pts',(-18.3073743398675,29.4817219469906,122.921775475891)) ;
#83083=CARTESIAN_POINT('Ctrl Pts',(-18.4071229866679,29.4915420311322,122.740968826247)) ;
#83084=CARTESIAN_POINT('Ctrl Pts',(-18.5399452984231,29.5016207578681,122.575947041892)) ;
#83085=CARTESIAN_POINT('Ctrl Pts',(-18.6958378157169,29.5114723385176,122.439518093478)) ;
#83086=CARTESIAN_POINT('Ctrl Pts',(-18.8768647521978,29.521545466816,122.329703299433)) ;
#83087=CARTESIAN_POINT('Ctrl Pts',(-19.0697539979625,29.5313879447074,122.254755395135)) ;
#83088=CARTESIAN_POINT('Ctrl Pts',(-19.2754083676275,29.5413685513055,122.213189334731)) ;
#83089=CARTESIAN_POINT('Ctrl Pts',(-19.485955652892,29.5513862603243,122.2083402379)) ;
#83090=CARTESIAN_POINT('Ctrl Pts',(-19.6914902361341,29.5612724393617,122.239308647118)) ;
#83091=CARTESIAN_POINT('Ctrl Pts',(-19.8919142714091,29.571330051934,122.306617589253)) ;
#83092=CARTESIAN_POINT('Ctrl Pts',(-20.0742975260261,29.5812064453062,122.405879060446)) ;
#83093=CARTESIAN_POINT('Ctrl Pts',(-20.2389379421708,29.5912014734566,122.536433084805)) ;
#83094=CARTESIAN_POINT('Ctrl Pts',(-20.3785081408678,29.6012222203026,122.694246134392)) ;
#83095=CARTESIAN_POINT('Ctrl Pts',(-20.4874550855457,29.611124288969,122.871631043243)) ;
#83096=CARTESIAN_POINT('Ctrl Pts',(-20.5649217226117,29.6211150287887,123.066861318861)) ;
#83097=CARTESIAN_POINT('Ctrl Pts',(-20.6070427364269,29.631078224999,123.272029797791)) ;
#83098=CARTESIAN_POINT('Ctrl Pts',(-20.6133815262534,29.6409824092991,123.4801692879)) ;
#83099=CARTESIAN_POINT('Ctrl Pts',(-20.5828416910867,29.65104286969,123.68942921765)) ;
#83100=CARTESIAN_POINT('Ctrl Pts',(-20.5181178762266,29.6608834155608,123.885951528494)) ;
#83101=CARTESIAN_POINT('Ctrl Pts',(-20.4183117865064,29.6709456362725,124.072440578358)) ;
#83102=CARTESIAN_POINT('Ctrl Pts',(-20.2895938023547,29.6808427792891,124.235930311958)) ;
#83103=CARTESIAN_POINT('Ctrl Pts',(-20.1343856079396,29.6907739557063,124.375570798608)) ;
#83104=CARTESIAN_POINT('Ctrl Pts',(-19.9551846882219,29.7008161694849,124.487181192015)) ;
#83105=CARTESIAN_POINT('Ctrl Pts',(-19.7624071612754,29.7107027096876,124.564908201709)) ;
#83106=CARTESIAN_POINT('Ctrl Pts',(-19.5569567804311,29.720696304293,124.608773536135)) ;
#83107=CARTESIAN_POINT('Ctrl Pts',(-19.3480261376384,29.7306401794506,124.616231476392)) ;
#83108=CARTESIAN_POINT('Ctrl Pts',(-19.1406146531479,29.7406007155654,124.587525948238)) ;
#83109=CARTESIAN_POINT('Ctrl Pts',(-18.9405437604366,29.7505973188881,124.523120293792)) ;
#83110=CARTESIAN_POINT('Ctrl Pts',(-18.7541801252713,29.7606304018426,124.424343499834)) ;
#83111=CARTESIAN_POINT('Ctrl Pts',(-18.59065350497,29.7704815705442,124.297265216123)) ;
#83112=CARTESIAN_POINT('Ctrl Pts',(-18.4496497380777,29.7804440612431,124.142406990805)) ;
#83113=CARTESIAN_POINT('Ctrl Pts',(-18.337145412894,29.7904724896608,123.964090322171)) ;
#83114=CARTESIAN_POINT('Ctrl Pts',(-18.25819728872,29.8003828570254,123.771290917072)) ;
#83115=CARTESIAN_POINT('Ctrl Pts',(-18.2132772363488,29.8103177246405,123.567310255916)) ;
#83116=CARTESIAN_POINT('Ctrl Pts',(-18.2045597770297,29.8203588666195,123.356400641158)) ;
#83117=CARTESIAN_POINT('Ctrl Pts',(-18.2320230342371,29.8302460028227,123.150352695314)) ;
#83118=CARTESIAN_POINT('Ctrl Pts',(-18.2951719204759,29.8402382852261,122.950015139329)) ;
#83119=CARTESIAN_POINT('Ctrl Pts',(-18.3917862051207,29.8501868131913,122.764504981868)) ;
#83120=CARTESIAN_POINT('Ctrl Pts',(-18.5187400573616,29.8601235443534,122.598627788548)) ;
#83121=CARTESIAN_POINT('Ctrl Pts',(-18.673140853215,29.8701067552134,122.456430324054)) ;
#83122=CARTESIAN_POINT('Ctrl Pts',(-18.8511109701876,29.8801498543633,122.342866858803)) ;
#83123=CARTESIAN_POINT('Ctrl Pts',(-19.0418427105954,29.8899808186382,122.263194741687)) ;
#83124=CARTESIAN_POINT('Ctrl Pts',(-19.2483822765628,29.9000536710241,122.216595398939)) ;
#83125=CARTESIAN_POINT('Ctrl Pts',(-19.455549423982,29.9099177987359,122.20680736902)) ;
#83126=CARTESIAN_POINT('Ctrl Pts',(-19.6646004829869,29.9199400008708,122.233040555836)) ;
#83127=CARTESIAN_POINT('Ctrl Pts',(-19.8658934126634,29.9299671938392,122.295687403736)) ;
#83128=CARTESIAN_POINT('Ctrl Pts',(-20.0501683092842,29.9398227878062,122.390377344587)) ;
#83129=CARTESIAN_POINT('Ctrl Pts',(-20.2172985731652,29.9497799596715,122.516433231891)) ;
#83130=CARTESIAN_POINT('Ctrl Pts',(-20.3608933907705,29.9598188036699,122.671082973157)) ;
#83131=CARTESIAN_POINT('Ctrl Pts',(-20.4739034023993,29.9696928275454,122.84524049053)) ;
#83132=CARTESIAN_POINT('Ctrl Pts',(-20.5565361429159,29.9797626535358,123.040115256471)) ;
#83133=CARTESIAN_POINT('Ctrl Pts',(-20.6030779857184,29.9895958974331,123.241551209471)) ;
#83134=CARTESIAN_POINT('Ctrl Pts',(-20.6147495281195,29.9996263252062,123.452092287856)) ;
#83135=CARTESIAN_POINT('Ctrl Pts',(-20.5890726629342,30.0096579419513,123.661431338415)) ;
#83136=CARTESIAN_POINT('Ctrl Pts',(-20.5290983151318,30.019487618932,123.859172845459)) ;
#83137=CARTESIAN_POINT('Ctrl Pts',(-20.434731970837,30.0294771357719,124.046795693821)) ;
#83138=CARTESIAN_POINT('Ctrl Pts',(-20.3081181710845,30.0395207479117,124.215767057646)) ;
#83139=CARTESIAN_POINT('Ctrl Pts',(-20.1577705279338,30.049343354247,124.35732849996)) ;
#83140=CARTESIAN_POINT('Ctrl Pts',(-19.9816087128904,30.0593815841462,124.473517351811)) ;
#83141=CARTESIAN_POINT('Ctrl Pts',(-19.7882588039469,30.0693926189382,124.556686176543)) ;
#83142=CARTESIAN_POINT('Ctrl Pts',(-19.5858185488893,30.0792903499053,124.604791885319)) ;
#83143=CARTESIAN_POINT('Ctrl Pts',(-19.3761865187044,30.0892799777558,124.617404592443)) ;
#83144=CARTESIAN_POINT('Ctrl Pts',(-19.1682644783533,30.0992357682018,124.593435202836)) ;
#83145=CARTESIAN_POINT('Ctrl Pts',(-18.9681109878404,30.1091631667638,124.53427778847)) ;
#83146=CARTESIAN_POINT('Ctrl Pts',(-18.7794620901044,30.1191887618737,124.440297304535)) ;
#83147=CARTESIAN_POINT('Ctrl Pts',(-18.6122766484749,30.1290746125433,124.316833188977)) ;
#83148=CARTESIAN_POINT('Ctrl Pts',(-18.4672078423433,30.1390637923875,124.164980782603)) ;
#83149=CARTESIAN_POINT('Ctrl Pts',(-18.3504739201255,30.149104979491,123.989097076407)) ;
#83150=CARTESIAN_POINT('Ctrl Pts',(-18.2674956317655,30.158937622967,123.799773764769)) ;
#83151=CARTESIAN_POINT('Ctrl Pts',(-18.2172642412709,30.1689315726765,123.595763800434)) ;
#83152=CARTESIAN_POINT('Ctrl Pts',(-18.203613049275,30.178960695453,123.385360236912)) ;
#83153=CARTESIAN_POINT('Ctrl Pts',(-18.2260199316159,30.1888368263717,123.178935369056)) ;
#83154=CARTESIAN_POINT('Ctrl Pts',(-18.2843970102494,30.1988348613887,122.977040722259)) ;
#83155=CARTESIAN_POINT('Ctrl Pts',(-18.3760423177623,30.2087487911474,122.789820231878)) ;
#83156=CARTESIAN_POINT('Ctrl Pts',(-18.5003433721555,30.2187919788852,122.619168159099)) ;
#83157=CARTESIAN_POINT('Ctrl Pts',(-18.6502274233987,30.2286918210256,122.474753642193)) ;
#83158=CARTESIAN_POINT('Ctrl Pts',(-18.8242469442218,30.2386830878336,122.357118257708)) ;
#83159=CARTESIAN_POINT('Ctrl Pts',(-19.0169820154261,30.2487151899655,122.271468240282)) ;
#83160=CARTESIAN_POINT('Ctrl Pts',(-19.2182167060322,30.2585820709203,122.221158082751)) ;
#83161=CARTESIAN_POINT('Ctrl Pts',(-19.4277225488607,30.2685738622084,122.205867869769)) ;
#83162=CARTESIAN_POINT('Ctrl Pts',(-19.6374978256527,30.27860597812,122.227678696559)) ;
#83163=CARTESIAN_POINT('Ctrl Pts',(-19.8370434526668,30.28847229492,122.284323901951)) ;
#83164=CARTESIAN_POINT('Ctrl Pts',(-20.0261335233839,30.2984597763936,122.375543048429)) ;
#83165=CARTESIAN_POINT('Ctrl Pts',(-20.1958972985317,30.3084047007725,122.49762869755)) ;
#83166=CARTESIAN_POINT('Ctrl Pts',(-20.3432317615189,30.3184495866832,122.648887741277)) ;
#83167=CARTESIAN_POINT('Ctrl Pts',(-20.4600715018246,30.3283116903958,122.820180920246)) ;
#83168=CARTESIAN_POINT('Ctrl Pts',(-20.5468880473964,30.3383032542202,123.011437808103)) ;
#83169=CARTESIAN_POINT('Ctrl Pts',(-20.5987893919799,30.3482360622831,123.21370328218)) ;
#83170=CARTESIAN_POINT('Ctrl Pts',(-20.6153024482951,30.3581731645195,123.421971743177)) ;
#83171=CARTESIAN_POINT('Ctrl Pts',(-20.5948955461052,30.3682256107899,123.63230200216)) ;
#83172=CARTESIAN_POINT('Ctrl Pts',(-20.5397174330207,30.3780717263715,123.831827122385)) ;
#83173=CARTESIAN_POINT('Ctrl Pts',(-20.4492191425848,30.3881197460864,124.022684679915)) ;
#83174=CARTESIAN_POINT('Ctrl Pts',(-20.3279940543757,30.3980616977153,124.192964425444)) ;
#83175=CARTESIAN_POINT('Ctrl Pts',(-20.1794618084049,30.4080004787144,124.33992376818)) ;
#83176=CARTESIAN_POINT('Ctrl Pts',(-20.0060825101838,30.4180265274405,124.45976448913)) ;
#83177=CARTESIAN_POINT('Ctrl Pts',(-19.8172623615967,30.4279133878487,124.546716314081)) ;
#83178=CARTESIAN_POINT('Ctrl Pts',(-19.6133595978461,30.4379446629805,124.600410230691)) ;
#83179=CARTESIAN_POINT('Ctrl Pts',(-19.4062767925641,30.4478276402809,124.617843638863)) ;
#83180=CARTESIAN_POINT('Ctrl Pts',(-19.1957688211311,30.4578844936881,124.598739097093)) ;
#83181=CARTESIAN_POINT('Ctrl Pts',(-18.9283787606756,30.471052734764,124.526647165086)) ;
#83182=CARTESIAN_POINT('Ctrl Pts',(-18.6818039728824,30.4844537639905,124.384038008386)) ;
#83183=CARTESIAN_POINT('Ctrl Pts',(-18.4857400799911,30.4976666807214,124.187208677308)) ;
#83184=CARTESIAN_POINT('Ctrl Pts',(-18.3657914541072,30.5075950751746,124.016432968705)) ;
#83185=CARTESIAN_POINT('Ctrl Pts',(-18.2766768590663,30.5175765753027,123.826421058636)) ;
#83186=CARTESIAN_POINT('Ctrl Pts',(-18.2218764268591,30.5276171185728,123.622585952812)) ;
#83187=CARTESIAN_POINT('Ctrl Pts',(-18.2033813661449,30.5374664503559,123.416346888214)) ;
#83188=CARTESIAN_POINT('Ctrl Pts',(-18.2206996447847,30.5474618548276,123.206928595446)) ;
#83189=CARTESIAN_POINT('Ctrl Pts',(-18.2745929041492,30.5574781822762,123.003367309086)) ;
#83190=CARTESIAN_POINT('Ctrl Pts',(-18.3909391811523,30.5707018394427,122.750841186866)) ;
#83191=CARTESIAN_POINT('Ctrl Pts',(-18.5712709267288,30.5839961308321,122.53321318112)) ;
#83192=CARTESIAN_POINT('Ctrl Pts',(-18.7990626847824,30.5972804817636,122.371616533633)) ;
#83193=CARTESIAN_POINT('Ctrl Pts',(-18.9884333508581,30.6072528628254,122.281709437163)) ;
#83194=CARTESIAN_POINT('Ctrl Pts',(-19.1891893065226,30.617161242451,122.226046310469)) ;
#83195=CARTESIAN_POINT('Ctrl Pts',(-19.3995715448735,30.627215241199,122.205891863364)) ;
#83196=CARTESIAN_POINT('Ctrl Pts',(-19.606289331107,30.6370774383153,122.2220960198)) ;
#83197=CARTESIAN_POINT('Ctrl Pts',(-19.8780883135872,30.6504245646895,122.291836907067)) ;
#83198=CARTESIAN_POINT('Ctrl Pts',(-20.1845056854532,30.6669615303309,122.46430462257)) ;
#83199=CARTESIAN_POINT('Ctrl Pts',(-20.4154425969608,30.6835961345048,122.732190513853)) ;
#83200=CARTESIAN_POINT('Ctrl Pts',(-20.5367455747761,30.6968859277475,122.983880923607)) ;
#83201=CARTESIAN_POINT('Ctrl Pts',(-20.5937491354777,30.7068385590069,123.185188446597)) ;
#83202=CARTESIAN_POINT('Ctrl Pts',(-20.6151760975103,30.7167905263116,123.393329160038)) ;
#83203=CARTESIAN_POINT('Ctrl Pts',(-20.5948114579857,30.7301577847754,123.67359407567)) ;
#83204=CARTESIAN_POINT('Ctrl Pts',(-20.4800577195779,30.7466745967245,124.005597255658)) ;
#83205=CARTESIAN_POINT('Ctrl Pts',(-20.2120200993978,30.7667004917309,124.336309570418)) ;
#83206=CARTESIAN_POINT('Ctrl Pts',(-19.8510357660558,30.7865112218611,124.553553066115)) ;
#83207=CARTESIAN_POINT('Ctrl Pts',(-19.4344068486954,30.8064884379909,124.636126295085)) ;
#83208=CARTESIAN_POINT('Ctrl Pts',(-19.0157737449017,30.8264153133862,124.570966815067)) ;
#83209=CARTESIAN_POINT('Ctrl Pts',(-18.645743049627,30.8462367748625,124.36909313754)) ;
#83210=CARTESIAN_POINT('Ctrl Pts',(-18.3635487087384,30.8663110926718,124.048939440631)) ;
#83211=CARTESIAN_POINT('Ctrl Pts',(-18.2096219039696,30.8861590616797,123.655865535498)) ;
#83212=CARTESIAN_POINT('Ctrl Pts',(-18.19815035681,30.9061060957429,123.231985121454)) ;
#83213=CARTESIAN_POINT('Ctrl Pts',(-18.3318134073363,30.926002046715,122.830579249658)) ;
#83214=CARTESIAN_POINT('Ctrl Pts',(-18.5938414916461,30.9458975263333,122.498499904225)) ;
#83215=CARTESIAN_POINT('Ctrl Pts',(-18.9545566345522,30.9658536372981,122.274979619949)) ;
#83216=CARTESIAN_POINT('Ctrl Pts',(-19.3687579852179,30.9857581853381,122.188333585932)) ;
#83217=CARTESIAN_POINT('Ctrl Pts',(-19.7873089672698,31.0056323096572,122.247107307915)) ;
#83218=CARTESIAN_POINT('Ctrl Pts',(-20.1636515298828,31.0256868396562,122.447450777236)) ;
#83219=CARTESIAN_POINT('Ctrl Pts',(-20.4457199868758,31.0454943534162,122.760325250148)) ;
#83220=CARTESIAN_POINT('Ctrl Pts',(-20.6062681401233,31.0654777091839,123.153662164199)) ;
#83221=CARTESIAN_POINT('Ctrl Pts',(-20.6222628204701,31.0853960117678,123.576872257537)) ;
#83222=CARTESIAN_POINT('Ctrl Pts',(-20.4942581378236,31.1052642272136,123.979554943358)) ;
#83223=CARTESIAN_POINT('Ctrl Pts',(-20.2337562023119,31.1253145440099,124.31687445342)) ;
#83224=CARTESIAN_POINT('Ctrl Pts',(-19.8787616566699,31.1450906058923,124.542563564278)) ;
#83225=CARTESIAN_POINT('Ctrl Pts',(-19.4626826896039,31.1651452115848,124.635079575042)) ;
#83226=CARTESIAN_POINT('Ctrl Pts',(-19.0452264784568,31.1849389007407,124.580607517285)) ;
#83227=CARTESIAN_POINT('Ctrl Pts',(-18.6678122022123,31.2049055923351,124.38638898605)) ;
#83228=CARTESIAN_POINT('Ctrl Pts',(-18.3797967673245,31.224865638086,124.07456737004)) ;
#83229=CARTESIAN_POINT('Ctrl Pts',(-18.2157691109868,31.2447638982363,123.684593743109)) ;
#83230=CARTESIAN_POINT('Ctrl Pts',(-18.1941556982586,31.2646588137855,123.262145187816)) ;
#83231=CARTESIAN_POINT('Ctrl Pts',(-18.3177211897733,31.2845689941991,122.857238651777)) ;
#83232=CARTESIAN_POINT('Ctrl Pts',(-18.5722267264253,31.3045047933133,122.518239434528)) ;
#83233=CARTESIAN_POINT('Ctrl Pts',(-18.9271454738372,31.3244426549675,122.286400969285)) ;
#83234=CARTESIAN_POINT('Ctrl Pts',(-19.3394522016131,31.3443617016051,122.189424102426)) ;
#83235=CARTESIAN_POINT('Ctrl Pts',(-19.7607105158001,31.3643105996593,122.238978385728)) ;
#83236=CARTESIAN_POINT('Ctrl Pts',(-20.1390295029159,31.3842164271023,122.428816602022)) ;
#83237=CARTESIAN_POINT('Ctrl Pts',(-20.3815087264455,31.4007991224676,122.684686241664)) ;
#83238=CARTESIAN_POINT('Ctrl Pts',(-20.5148524186569,31.4140733361913,122.929906786892)) ;
#83239=CARTESIAN_POINT('Ctrl Pts',(-20.5818785542684,31.4241200553906,123.130173426279)) ;
#83240=CARTESIAN_POINT('Ctrl Pts',(-20.6127165674891,31.4339640900363,123.334840458635)) ;
#83241=CARTESIAN_POINT('Ctrl Pts',(-20.6063535951271,31.4472984749408,123.615037152783)) ;
#83242=CARTESIAN_POINT('Ctrl Pts',(-20.5072194117263,31.4638856922406,123.953619575348)) ;
#83243=CARTESIAN_POINT('Ctrl Pts',(-20.2982546759496,31.4805189042785,124.238841010089)) ;
#83244=CARTESIAN_POINT('Ctrl Pts',(-20.0804678238985,31.4938013465506,124.413704853419)) ;
#83245=CARTESIAN_POINT('Ctrl Pts',(-19.8981272815586,31.5037072344649,124.514266935638)) ;
#83246=CARTESIAN_POINT('Ctrl Pts',(-19.6995097079086,31.51369565257,124.582464166109)) ;
#83247=CARTESIAN_POINT('Ctrl Pts',(-19.4913126461785,31.5237190798087,124.615029422142)) ;
#83248=CARTESIAN_POINT('Ctrl Pts',(-19.2831319092561,31.5336235109258,124.611113980468)) ;
#83249=CARTESIAN_POINT('Ctrl Pts',(-19.0093614799214,31.5468866635362,124.558272298217)) ;
#83250=CARTESIAN_POINT('Ctrl Pts',(-18.7546008901196,31.5602115614401,124.434360421277)) ;
#83251=CARTESIAN_POINT('Ctrl Pts',(-18.5439610209561,31.5734673050557,124.251809963666)) ;
#83252=CARTESIAN_POINT('Ctrl Pts',(-18.4117282371194,31.583426678503,124.089512292891)) ;
#83253=CARTESIAN_POINT('Ctrl Pts',(-18.3095841784395,31.5933705024299,123.907084613389)) ;
#83254=CARTESIAN_POINT('Ctrl Pts',(-18.2401310523998,31.6034184465772,123.707606289012)) ;
#83255=CARTESIAN_POINT('Ctrl Pts',(-18.2068457694298,31.6132694177954,123.503187635857)) ;
#83256=CARTESIAN_POINT('Ctrl Pts',(-18.2090524602005,31.6232412352375,123.293584248886)) ;
#83257=CARTESIAN_POINT('Ctrl Pts',(-18.2477548018564,31.6332366575296,123.087014130891)) ;
#83258=CARTESIAN_POINT('Ctrl Pts',(-18.3222090746577,31.6432697226533,122.889672426475)) ;
#83259=CARTESIAN_POINT('Ctrl Pts',(-18.4278263368555,31.6531350553185,122.71118449622)) ;
#83260=CARTESIAN_POINT('Ctrl Pts',(-18.5636713658397,31.6630955979161,122.551819036529)) ;
#83261=CARTESIAN_POINT('Ctrl Pts',(-18.7265249362776,31.6731292834178,122.417766698447)) ;
#83262=CARTESIAN_POINT('Ctrl Pts',(-18.9073121335119,31.683014115408,122.31523335348)) ;
#83263=CARTESIAN_POINT('Ctrl Pts',(-19.1067295419793,31.6930815421679,122.244429551725)) ;
#83264=CARTESIAN_POINT('Ctrl Pts',(-19.3107004385562,31.7029200313267,122.209912169596)) ;
#83265=CARTESIAN_POINT('Ctrl Pts',(-19.5222334995631,31.7129835125168,122.211086087581)) ;
#83266=CARTESIAN_POINT('Ctrl Pts',(-19.7268674082678,31.722877670332,122.248520772617)) ;
#83267=CARTESIAN_POINT('Ctrl Pts',(-19.9229838785611,31.7328195270763,122.320715616212)) ;
#83268=CARTESIAN_POINT('Ctrl Pts',(-20.1047748415662,31.7428220047477,122.426467352772)) ;
#83269=CARTESIAN_POINT('Ctrl Pts',(-20.2657146991617,31.752856809052,122.562842382034)) ;
#83270=CARTESIAN_POINT('Ctrl Pts',(-20.3982636528338,31.7627016858976,122.721817853387)) ;
#83271=CARTESIAN_POINT('Ctrl Pts',(-20.5029887507993,31.7726875654532,122.90372683207)) ;
#83272=CARTESIAN_POINT('Ctrl Pts',(-20.5743391712646,31.7826222958117,123.100063805189)) ;
#83273=CARTESIAN_POINT('Ctrl Pts',(-20.6107539154827,31.7926801081246,123.308316175894)) ;
#83274=CARTESIAN_POINT('Ctrl Pts',(-20.6108179024331,31.8025007002489,123.514810057198)) ;
#83275=CARTESIAN_POINT('Ctrl Pts',(-20.5744003087098,31.8125672858587,123.723241387401)) ;
#83276=CARTESIAN_POINT('Ctrl Pts',(-20.5034740802056,31.8224668664405,123.918955059192)) ;
#83277=CARTESIAN_POINT('Ctrl Pts',(-20.3981618181735,31.8325184661188,124.102114219325)) ;
#83278=CARTESIAN_POINT('Ctrl Pts',(-20.2651091877199,31.8423926525358,124.261505376368)) ;
#83279=CARTESIAN_POINT('Ctrl Pts',(-20.1036202264451,31.8524491284167,124.397897467732)) ;
#83280=CARTESIAN_POINT('Ctrl Pts',(-19.9238419317425,31.8623420597193,124.502558097825)) ;
#83281=CARTESIAN_POINT('Ctrl Pts',(-19.7253582983379,31.8724048384319,124.575658467282)) ;
#83282=CARTESIAN_POINT('Ctrl Pts',(-19.5217145643937,31.8822473640131,124.612477743301)) ;
#83283=CARTESIAN_POINT('Ctrl Pts',(-19.3117088879781,31.8922381294379,124.613893835916)) ;
#83284=CARTESIAN_POINT('Ctrl Pts',(-19.1059168167146,31.902166205436,124.579001618329)) ;
#83285=CARTESIAN_POINT('Ctrl Pts',(-18.9080017658777,31.912154115823,124.508830983756)) ;
#83286=CARTESIAN_POINT('Ctrl Pts',(-18.7245905230028,31.9221900279479,124.404561296605)) ;
#83287=CARTESIAN_POINT('Ctrl Pts',(-18.5647630481987,31.9320450407956,124.27270294668)) ;
#83288=CARTESIAN_POINT('Ctrl Pts',(-18.4281031647553,31.9420439867119,124.113022558058)) ;
#83289=CARTESIAN_POINT('Ctrl Pts',(-18.3221272962083,31.9519408991599,123.933932731515)) ;
#83290=CARTESIAN_POINT('Ctrl Pts',(-18.2476926054129,31.9619946972534,123.736138061524)) ;
#83291=CARTESIAN_POINT('Ctrl Pts',(-18.2093337802235,31.97187561808,123.53195900041)) ;
#83292=CARTESIAN_POINT('Ctrl Pts',(-18.2066019695323,31.9818801440778,123.321674466972)) ;
#83293=CARTESIAN_POINT('Ctrl Pts',(-18.2404263440032,31.9918641076953,123.114487622753)) ;
#83294=CARTESIAN_POINT('Ctrl Pts',(-18.3102693041505,32.0019037482466,122.915329879683)) ;
#83295=CARTESIAN_POINT('Ctrl Pts',(-18.4114038214133,32.0117477738613,122.734771545471)) ;
#83296=CARTESIAN_POINT('Ctrl Pts',(-18.5438394915442,32.0217387796786,122.571741129883)) ;
#83297=CARTESIAN_POINT('Ctrl Pts',(-18.703628596721,32.0317765712108,122.433903138758)) ;
#83298=CARTESIAN_POINT('Ctrl Pts',(-18.8812503335969,32.0416209709992,122.327667862756)) ;
#83299=CARTESIAN_POINT('Ctrl Pts',(-19.0771971927256,32.0516057715559,122.25246020401)) ;
#83300=CARTESIAN_POINT('Ctrl Pts',(-19.2823298265578,32.0615452949671,122.212499589025)) ;
#83301=CARTESIAN_POINT('Ctrl Pts',(-19.4933471363301,32.0715850140681,122.208776391678)) ;
#83302=CARTESIAN_POINT('Ctrl Pts',(-19.6987028420245,32.0814731859874,122.24115319859)) ;
#83303=CARTESIAN_POINT('Ctrl Pts',(-19.8974425339761,32.0914627484044,122.309009013835)) ;
#83304=CARTESIAN_POINT('Ctrl Pts',(-20.0807345462606,32.1014211205991,122.410164937541)) ;
#83305=CARTESIAN_POINT('Ctrl Pts',(-20.2430472168791,32.1113211948298,122.540457107242)) ;
#83306=CARTESIAN_POINT('Ctrl Pts',(-20.3822631435707,32.1213672912034,122.699266977795)) ;
#83307=CARTESIAN_POINT('Ctrl Pts',(-20.4903109590882,32.1312758752005,122.877375105401)) ;
#83308=CARTESIAN_POINT('Ctrl Pts',(-20.5669294967305,32.1412864537914,123.073389780507)) ;
#83309=CARTESIAN_POINT('Ctrl Pts',(-20.608008918276,32.1513156119042,123.28020159049)) ;
#83310=CARTESIAN_POINT('Ctrl Pts',(-20.6127724602431,32.1611684937423,123.487271842967)) ;
#83311=CARTESIAN_POINT('Ctrl Pts',(-20.581806621185,32.1711280548933,123.694357054793)) ;
#83312=CARTESIAN_POINT('Ctrl Pts',(-20.5144687727705,32.1811664894824,123.894350918024)) ;
#83313=CARTESIAN_POINT('Ctrl Pts',(-20.4154130490164,32.1910397617095,124.07679460432)) ;
#83314=CARTESIAN_POINT('Ctrl Pts',(-20.2835620235085,32.201113003703,124.242457441947)) ;
#83315=CARTESIAN_POINT('Ctrl Pts',(-20.1290461275997,32.2109333352361,124.379450085929)) ;
#83316=CARTESIAN_POINT('Ctrl Pts',(-19.9486477293024,32.2210119964629,124.490491077014)) ;
#83317=CARTESIAN_POINT('Ctrl Pts',(-19.7560810791827,32.2308635917571,124.566868126149)) ;
#83318=CARTESIAN_POINT('Ctrl Pts',(-19.5487382565785,32.2409367269859,124.609752347802)) ;
#83319=CARTESIAN_POINT('Ctrl Pts',(-19.3418894082037,32.2507791625109,124.6158111822)) ;
#83320=CARTESIAN_POINT('Ctrl Pts',(-19.1341823402658,32.2607599316443,124.58613825041)) ;
#83321=CARTESIAN_POINT('Ctrl Pts',(-18.9341677743458,32.2707770328882,124.520238624712)) ;
#83322=CARTESIAN_POINT('Ctrl Pts',(-18.7508181441457,32.2806654804901,124.42222827271)) ;
#83323=CARTESIAN_POINT('Ctrl Pts',(-18.5845185824704,32.2907211946709,124.291738453968)) ;
#83324=CARTESIAN_POINT('Ctrl Pts',(-18.4458907267504,32.3005964010847,124.137177696302)) ;
#83325=CARTESIAN_POINT('Ctrl Pts',(-18.3344556829309,32.3105914535575,123.959039398453)) ;
#83326=CARTESIAN_POINT('Ctrl Pts',(-18.2557440839217,32.3206133375196,123.763594375523)) ;
#83327=CARTESIAN_POINT('Ctrl Pts',(-18.2124503446323,32.3305173100489,123.559934275682)) ;
#83328=CARTESIAN_POINT('Ctrl Pts',(-18.2048119906324,32.3405058067098,123.350081945316)) ;
#83329=CARTESIAN_POINT('Ctrl Pts',(-18.2337946180017,32.3504696039577,123.142637274561)) ;
#83330=CARTESIAN_POINT('Ctrl Pts',(-18.2974931064922,32.3603736272658,122.944386171069)) ;
#83331=CARTESIAN_POINT('Ctrl Pts',(-18.396316975891,32.3704341305874,122.757419493341)) ;
#83332=CARTESIAN_POINT('Ctrl Pts',(-18.5230894394292,32.3802746657273,122.593899248481)) ;
#83333=CARTESIAN_POINT('Ctrl Pts',(-18.6795618066723,32.3903368864319,122.451576307416)) ;
#83334=CARTESIAN_POINT('Ctrl Pts',(-18.8555799493967,32.4002340402081,122.3406038363)) ;
#83335=CARTESIAN_POINT('Ctrl Pts',(-19.0485759608522,32.4101651735936,122.260971581326)) ;
#83336=CARTESIAN_POINT('Ctrl Pts',(-19.254802198742,32.4202075487393,122.215784881501)) ;
#83337=CARTESIAN_POINT('Ctrl Pts',(-19.462464619885,32.4300934865054,122.207066667792)) ;
#83338=CARTESIAN_POINT('Ctrl Pts',(-19.6707916883363,32.4400893294903,122.234516696651)) ;
#83339=CARTESIAN_POINT('Ctrl Pts',(-19.8701274150094,32.4500313073689,122.297413048005)) ;
#83340=CARTESIAN_POINT('Ctrl Pts',(-20.0559495921236,32.4599906818499,122.393870351229)) ;
#83341=CARTESIAN_POINT('Ctrl Pts',(-20.2229152131252,32.4699872976837,122.521538033646)) ;
#83342=CARTESIAN_POINT('Ctrl Pts',(-20.3654870895935,32.4800215162572,122.677008263768)) ;
#83343=CARTESIAN_POINT('Ctrl Pts',(-20.4770646801134,32.4898745834678,122.851527873814)) ;
#83344=CARTESIAN_POINT('Ctrl Pts',(-20.5580731805413,32.4998348413454,123.044611536658)) ;
#83345=CARTESIAN_POINT('Ctrl Pts',(-20.6044060160116,32.509863868051,123.250311165375)) ;
#83346=CARTESIAN_POINT('Ctrl Pts',(-20.6142619776741,32.5197740750854,123.458412229653)) ;
#83347=CARTESIAN_POINT('Ctrl Pts',(-20.5883124061432,32.529708985733,123.665662879571)) ;
#83348=CARTESIAN_POINT('Ctrl Pts',(-20.5259286930374,32.5397501159122,123.867323656511)) ;
#83349=CARTESIAN_POINT('Ctrl Pts',(-20.4310789052782,32.5496372562822,124.052292593451)) ;
#83350=CARTESIAN_POINT('Ctrl Pts',(-20.3045135514618,32.5596295338181,124.219935537952)) ;
#83351=CARTESIAN_POINT('Ctrl Pts',(-20.1513762341763,32.5695780770865,124.362403871637)) ;
#83352=CARTESIAN_POINT('Ctrl Pts',(-19.9762223695005,32.5795147519037,124.476218556103)) ;
#83353=CARTESIAN_POINT('Ctrl Pts',(-19.7831272891508,32.58949817284,124.55852326293)) ;
#83354=CARTESIAN_POINT('Ctrl Pts',(-19.5774219840255,32.5995404880293,124.605989529416)) ;
#83355=CARTESIAN_POINT('Ctrl Pts',(-19.3708457610076,32.6093808054685,124.617131308199)) ;
#83356=CARTESIAN_POINT('Ctrl Pts',(-19.1614606709902,32.619410509526,124.59224704481)) ;
#83357=CARTESIAN_POINT('Ctrl Pts',(-18.9599202826958,32.6294314662485,124.530895291569)) ;
#83358=CARTESIAN_POINT('Ctrl Pts',(-18.7747348077778,32.6392980085521,124.437418884862)) ;
#83359=CARTESIAN_POINT('Ctrl Pts',(-18.6051744829553,32.6493691084972,124.310654926759)) ;
#83360=CARTESIAN_POINT('Ctrl Pts',(-18.4634825803537,32.6592111826748,124.159861045774)) ;
#83361=CARTESIAN_POINT('Ctrl Pts',(-18.348119531362,32.6691719772618,123.985101878547)) ;
#83362=CARTESIAN_POINT('Ctrl Pts',(-18.2645928499221,32.6792098501627,123.79131595217)) ;
#83363=CARTESIAN_POINT('Ctrl Pts',(-18.2163931534487,32.6890841357068,123.589374685025)) ;
#83364=CARTESIAN_POINT('Ctrl Pts',(-18.2037592125035,32.6991538861207,123.378082408074)) ;
#83365=CARTESIAN_POINT('Ctrl Pts',(-18.2273293206378,32.7089871706553,123.172687254376)) ;
#83366=CARTESIAN_POINT('Ctrl Pts',(-18.2868043404784,32.7190175114554,122.970385348413)) ;
#83367=CARTESIAN_POINT('Ctrl Pts',(-18.3810784993133,32.729049435455,122.781715068891)) ;
#83368=CARTESIAN_POINT('Ctrl Pts',(-18.5037608242304,32.7388779703909,122.615463889597)) ;
#83369=CARTESIAN_POINT('Ctrl Pts',(-18.6555715412042,32.7488717481556,122.470222039496)) ;
#83370=CARTESIAN_POINT('Ctrl Pts',(-18.8311254092731,32.7588994586411,122.353490726389)) ;
#83371=CARTESIAN_POINT('Ctrl Pts',(-19.0214892252655,32.7687878694751,122.269952805632)) ;
#83372=CARTESIAN_POINT('Ctrl Pts',(-19.2251690251725,32.7787647200106,122.219945127882)) ;
#83373=CARTESIAN_POINT('Ctrl Pts',(-19.4347962363997,32.7887565165611,122.206021141314)) ;
#83374=CARTESIAN_POINT('Ctrl Pts',(-19.644506274362,32.7987925226548,122.229058211083)) ;
#83375=CARTESIAN_POINT('Ctrl Pts',(-19.8434117086824,32.8086432569176,122.286768454023)) ;
#83376=CARTESIAN_POINT('Ctrl Pts',(-20.0320459418187,32.8186345154458,122.379097172002)) ;
#83377=CARTESIAN_POINT('Ctrl Pts',(-20.200655836678,32.828552410349,122.501801185391)) ;
#83378=CARTESIAN_POINT('Ctrl Pts',(-20.3470163616419,32.838580552012,122.653517385148)) ;
#83379=CARTESIAN_POINT('Ctrl Pts',(-20.4632160383456,32.8484657201279,122.825818799276)) ;
#83380=CARTESIAN_POINT('Ctrl Pts',(-20.5490902337959,32.8584550836339,123.017471264473)) ;
#83381=CARTESIAN_POINT('Ctrl Pts',(-20.6002153354156,32.8684962186439,123.222283159047)) ;
#83382=CARTESIAN_POINT('Ctrl Pts',(-20.6150344431865,32.878328886832,123.428460757677)) ;
#83383=CARTESIAN_POINT('Ctrl Pts',(-20.594080101708,32.8883227897865,123.637515478041)) ;
#83384=CARTESIAN_POINT('Ctrl Pts',(-20.5365126192868,32.898352074871,123.840353459571)) ;
#83385=CARTESIAN_POINT('Ctrl Pts',(-20.4463103933135,32.9082276033129,124.027361177366)) ;
#83386=CARTESIAN_POINT('Ctrl Pts',(-20.3236864945423,32.9182278859289,124.198101789634)) ;
#83387=CARTESIAN_POINT('Ctrl Pts',(-20.1746881491512,32.928139901986,124.343816675066)) ;
#83388=CARTESIAN_POINT('Ctrl Pts',(-20.0004586807909,32.938181977325,124.463012680177)) ;
#83389=CARTESIAN_POINT('Ctrl Pts',(-19.8108772925301,32.9480818099811,124.548917300338)) ;
#83390=CARTESIAN_POINT('Ctrl Pts',(-19.6075007747243,32.9580742105591,124.601531936566)) ;
#83391=CARTESIAN_POINT('Ctrl Pts',(-19.3971732333432,32.9681082323185,124.617729269528)) ;
#83392=CARTESIAN_POINT('Ctrl Pts',(-19.190754436079,32.9779728431597,124.597773976657)) ;
#83393=CARTESIAN_POINT('Ctrl Pts',(-18.9882033469982,32.9879652426208,124.542054828575)) ;
#83394=CARTESIAN_POINT('Ctrl Pts',(-18.7978335009767,32.9979971959537,124.451283463694)) ;
#83395=CARTESIAN_POINT('Ctrl Pts',(-18.6287589942609,33.0078635548954,124.331111742769)) ;
#83396=CARTESIAN_POINT('Ctrl Pts',(-18.4811111557562,33.0178510303812,124.181860134254)) ;
#83397=CARTESIAN_POINT('Ctrl Pts',(-18.362006088434,33.0277959365697,124.009992202084)) ;
#83398=CARTESIAN_POINT('Ctrl Pts',(-18.2738031023012,33.0378409012299,123.818139922867)) ;
#83399=CARTESIAN_POINT('Ctrl Pts',(-18.221036924655,33.0477027081348,123.617622978503)) ;
#83400=CARTESIAN_POINT('Ctrl Pts',(-18.2032624857334,33.0576953804405,123.408320496302)) ;
#83401=CARTESIAN_POINT('Ctrl Pts',(-18.2220069147815,33.0676240513859,123.200418237419)) ;
#83402=CARTESIAN_POINT('Ctrl Pts',(-18.276358079909,33.0775765936112,122.998381929429)) ;
#83403=CARTESIAN_POINT('Ctrl Pts',(-18.3653128439867,33.0875779496071,122.807841826037)) ;
#83404=CARTESIAN_POINT('Ctrl Pts',(-18.486547387057,33.0976065618818,122.635363535432)) ;
#83405=CARTESIAN_POINT('Ctrl Pts',(-18.6332437344153,33.1074708964313,122.488761354518)) ;
#83406=CARTESIAN_POINT('Ctrl Pts',(-18.8051496261247,33.1174632205079,122.368071521827)) ;
#83407=CARTESIAN_POINT('Ctrl Pts',(-18.9941648077372,33.1273907128737,122.279502904876)) ;
#83408=CARTESIAN_POINT('Ctrl Pts',(-19.1976621955604,33.1374180714246,122.224574414037)) ;
#83409=CARTESIAN_POINT('Ctrl Pts',(-19.4046917063012,33.1473044894757,122.205852145858)) ;
#83410=CARTESIAN_POINT('Ctrl Pts',(-19.6148150213246,33.1573362242111,122.22350700037)) ;
#83411=CARTESIAN_POINT('Ctrl Pts',(-19.8157514821659,33.1672178054543,122.276392579727)) ;
#83412=CARTESIAN_POINT('Ctrl Pts',(-20.0078549838356,33.1772797834867,122.364875755103)) ;
#83413=CARTESIAN_POINT('Ctrl Pts',(-20.1782306268323,33.1871368618484,122.482889582793)) ;
#83414=CARTESIAN_POINT('Ctrl Pts',(-20.3278335578549,33.1971314349544,122.630382150663)) ;
#83415=CARTESIAN_POINT('Ctrl Pts',(-20.4488150867353,33.207057231242,122.800439196544)) ;
#83416=CARTESIAN_POINT('Ctrl Pts',(-20.5393606634792,33.2170825984117,122.99074466967)) ;
#83417=CARTESIAN_POINT('Ctrl Pts',(-20.5948558871472,33.2269786780656,123.191261925233)) ;
#83418=CARTESIAN_POINT('Ctrl Pts',(-20.6153122230026,33.2369737577711,123.400394982972)) ;
#83419=CARTESIAN_POINT('Ctrl Pts',(-20.5987384029199,33.246998845587,123.610498671386)) ;
#83420=CARTESIAN_POINT('Ctrl Pts',(-20.5297765324198,33.2601826679542,123.878959486108)) ;
#83421=CARTESIAN_POINT('Ctrl Pts',(-20.3913922331434,33.2735047861002,124.126130635834)) ;
#83422=CARTESIAN_POINT('Ctrl Pts',(-20.1945244288533,33.2868839957278,124.327020121736)) ;
#83423=CARTESIAN_POINT('Ctrl Pts',(-20.0266226406426,33.296722232972,124.44783147606)) ;
#83424=CARTESIAN_POINT('Ctrl Pts',(-19.8359283407029,33.3067951562307,124.539857196587)) ;
#83425=CARTESIAN_POINT('Ctrl Pts',(-19.6364751988179,33.3166517976858,124.596128291563)) ;
#83426=CARTESIAN_POINT('Ctrl Pts',(-19.4276788871458,33.3266371731919,124.617742250002)) ;
#83427=CARTESIAN_POINT('Ctrl Pts',(-19.1491574137072,33.3399212046523,124.597574248406)) ;
#83428=CARTESIAN_POINT('Ctrl Pts',(-18.8168324643961,33.3564399965226,124.483616296897)) ;
#83429=CARTESIAN_POINT('Ctrl Pts',(-18.5395293026587,33.3732257135293,124.258981067428)) ;
#83430=CARTESIAN_POINT('Ctrl Pts',(-18.3774838638889,33.3863388620383,124.035935686859)) ;
#83431=CARTESIAN_POINT('Ctrl Pts',(-18.2842424548978,33.3963744111184,123.846700489471)) ;
#83432=CARTESIAN_POINT('Ctrl Pts',(-18.2259657627014,33.4063904672979,123.644335418821)) ;
#83433=CARTESIAN_POINT('Ctrl Pts',(-18.1960980312473,33.4195685031639,123.368929020654)) ;
#83434=CARTESIAN_POINT('Ctrl Pts',(-18.2490090481057,33.436170380351,123.019870932776)) ;
#83435=CARTESIAN_POINT('Ctrl Pts',(-18.4541281933962,33.4562335249669,122.645836797817)) ;
#83436=CARTESIAN_POINT('Ctrl Pts',(-18.7702598882601,33.4760344150506,122.367699543622)) ;
#83437=CARTESIAN_POINT('Ctrl Pts',(-19.1646435491626,33.4959775403293,122.212088086197)) ;
#83438=CARTESIAN_POINT('Ctrl Pts',(-19.5875673811207,33.5158755854489,122.200707738123)) ;
#83439=CARTESIAN_POINT('Ctrl Pts',(-19.9891371716541,33.5357613450756,122.333269289904)) ;
#83440=CARTESIAN_POINT('Ctrl Pts',(-20.3238757207542,33.5558265202555,122.597734115346)) ;
#83441=CARTESIAN_POINT('Ctrl Pts',(-20.5455361210312,33.5756531633583,122.956408577687)) ;
#83442=CARTESIAN_POINT('Ctrl Pts',(-20.6329532916303,33.5955618728067,123.370482994529)) ;
#83443=CARTESIAN_POINT('Ctrl Pts',(-20.5737633532293,33.6155137098385,123.79068321241)) ;
#83444=CARTESIAN_POINT('Ctrl Pts',(-20.3736428975741,33.6355221845416,124.166059601071)) ;
#83445=CARTESIAN_POINT('Ctrl Pts',(-20.0610026955118,33.6553236433031,124.448078246282)) ;
#83446=CARTESIAN_POINT('Ctrl Pts',(-19.6682568612891,33.675280531539,124.608739923763)) ;
#83447=CARTESIAN_POINT('Ctrl Pts',(-19.2436659702764,33.6952643689531,124.624794639191)) ;
#83448=CARTESIAN_POINT('Ctrl Pts',(-18.8423052598593,33.7150728081741,124.496925818226)) ;
#83449=CARTESIAN_POINT('Ctrl Pts',(-18.5055647293173,33.7350585175543,124.237926514824)) ;
#83450=CARTESIAN_POINT('Ctrl Pts',(-18.2784679586642,33.7549280405696,123.881468060406)) ;
#83451=CARTESIAN_POINT('Ctrl Pts',(-18.1861872054109,33.7749487796868,123.466060026539)) ;
#83452=CARTESIAN_POINT('Ctrl Pts',(-18.2401103433978,33.7947528446637,123.048276947068)) ;
#83453=CARTESIAN_POINT('Ctrl Pts',(-18.4356215903281,33.8148148083945,122.66928309307)) ;
#83454=CARTESIAN_POINT('Ctrl Pts',(-18.7455984770616,33.834647988683,122.383215119623)) ;
#83455=CARTESIAN_POINT('Ctrl Pts',(-19.1356568043022,33.854567186009,122.21836038993)) ;
#83456=CARTESIAN_POINT('Ctrl Pts',(-19.5590432936728,33.8745052111223,122.196755239328)) ;
#83457=CARTESIAN_POINT('Ctrl Pts',(-19.9633828074082,33.8943832571784,122.319991705251)) ;
#83458=CARTESIAN_POINT('Ctrl Pts',(-20.3031557179913,33.9143679914665,122.575085856202)) ;
#83459=CARTESIAN_POINT('Ctrl Pts',(-20.534784691646,33.934278808145,122.92960459951)) ;
#83460=CARTESIAN_POINT('Ctrl Pts',(-20.6316400568924,33.9542777836637,123.343555560692)) ;
#83461=CARTESIAN_POINT('Ctrl Pts',(-20.58241644095,33.9740827043089,123.761861352156)) ;
#83462=CARTESIAN_POINT('Ctrl Pts',(-20.392337806412,33.9940666646001,124.141776573077)) ;
#83463=CARTESIAN_POINT('Ctrl Pts',(-20.0852720969054,34.0139528683241,124.43258612421)) ;
#83464=CARTESIAN_POINT('Ctrl Pts',(-19.6964740781402,34.0339020466473,124.602080252954)) ;
#83465=CARTESIAN_POINT('Ctrl Pts',(-19.2741491940426,34.0538038458868,124.628564557594)) ;
#83466=CARTESIAN_POINT('Ctrl Pts',(-18.8683285859551,34.0736824509392,124.510329663157)) ;
#83467=CARTESIAN_POINT('Ctrl Pts',(-18.5246879272809,34.0937148106649,124.258609949435)) ;
#83468=CARTESIAN_POINT('Ctrl Pts',(-18.3288959796527,34.110296536621,123.965412149913)) ;
#83469=CARTESIAN_POINT('Ctrl Pts',(-18.2390051118599,34.1234907069189,123.702986280917)) ;
#83470=CARTESIAN_POINT('Ctrl Pts',(-18.195215620379,34.1368028850121,123.426625345839)) ;
#83471=CARTESIAN_POINT('Ctrl Pts',(-18.2318570276994,34.1533690646054,123.076205474803)) ;
#83472=CARTESIAN_POINT('Ctrl Pts',(-18.3860722304639,34.1699972594656,122.758154636996)) ;
#83473=CARTESIAN_POINT('Ctrl Pts',(-18.5689207833389,34.1832858411753,122.546840480982)) ;
#83474=CARTESIAN_POINT('Ctrl Pts',(-18.7313513303073,34.1932540892789,122.414464338576)) ;
#83475=CARTESIAN_POINT('Ctrl Pts',(-18.9132140631746,34.2031688455351,122.312607045933)) ;
#83476=CARTESIAN_POINT('Ctrl Pts',(-19.1118792711937,34.2131819961863,122.242971316891)) ;
#83477=CARTESIAN_POINT('Ctrl Pts',(-19.3196579103368,34.2231947033883,122.209223879779)) ;
#83478=CARTESIAN_POINT('Ctrl Pts',(-19.597538352536,34.2364139920796,122.212437336866)) ;
#83479=CARTESIAN_POINT('Ctrl Pts',(-19.9378288626282,34.2530326730776,122.307523642033)) ;
#83480=CARTESIAN_POINT('Ctrl Pts',(-20.2246132922364,34.2695975808511,122.512032295996)) ;
#83481=CARTESIAN_POINT('Ctrl Pts',(-20.4036556912666,34.2829960524619,122.729519755814)) ;
#83482=CARTESIAN_POINT('Ctrl Pts',(-20.5055966706641,34.2928373079489,122.909568823664)) ;
#83483=CARTESIAN_POINT('Ctrl Pts',(-20.5761690059698,34.3028236235371,123.107261401867)) ;
#83484=CARTESIAN_POINT('Ctrl Pts',(-20.6112776484593,34.3127602311235,123.313223850994)) ;
#83485=CARTESIAN_POINT('Ctrl Pts',(-20.609973583627,34.3228100984918,123.524478235219)) ;
#83486=CARTESIAN_POINT('Ctrl Pts',(-20.5729077524679,34.3326605931666,123.728238360151)) ;
#83487=CARTESIAN_POINT('Ctrl Pts',(-20.5006686189369,34.3426323935611,123.925008528361)) ;
#83488=CARTESIAN_POINT('Ctrl Pts',(-20.3950540866116,34.3526283605869,124.106728445384)) ;
#83489=CARTESIAN_POINT('Ctrl Pts',(-20.2587448397583,34.3626658199681,124.267788317343)) ;
#83490=CARTESIAN_POINT('Ctrl Pts',(-20.099944331439,34.3725065208688,124.400411921082)) ;
#83491=CARTESIAN_POINT('Ctrl Pts',(-19.916925180984,34.3825545421362,124.505877187115)) ;
#83492=CARTESIAN_POINT('Ctrl Pts',(-19.7202373549352,34.3925019352189,124.576929496361)) ;
#83493=CARTESIAN_POINT('Ctrl Pts',(-19.5150731826552,34.4024120812653,124.613246050668)) ;
#83494=CARTESIAN_POINT('Ctrl Pts',(-19.3036249159796,34.4124709951149,124.613150609061)) ;
#83495=CARTESIAN_POINT('Ctrl Pts',(-19.0998219309053,34.4223117654042,124.577418246397)) ;
#83496=CARTESIAN_POINT('Ctrl Pts',(-18.9008963305154,34.4323746349828,124.505500646163)) ;
#83497=CARTESIAN_POINT('Ctrl Pts',(-18.7205944587309,34.4422689581133,124.401729144062)) ;
#83498=CARTESIAN_POINT('Ctrl Pts',(-18.5599579928676,34.4522107652078,124.268052326554)) ;
#83499=CARTESIAN_POINT('Ctrl Pts',(-18.4240523663219,34.4622132761631,124.107549499809)) ;
#83500=CARTESIAN_POINT('Ctrl Pts',(-18.3180449884681,34.4722479969815,123.925171280476)) ;
#83501=CARTESIAN_POINT('Ctrl Pts',(-18.2463591450484,34.4820931744872,123.73099253113)) ;
#83502=CARTESIAN_POINT('Ctrl Pts',(-18.2085560221446,34.4920779348883,123.524543622521)) ;
#83503=CARTESIAN_POINT('Ctrl Pts',(-18.2070790887704,34.5020168412047,123.315570311663)) ;
#83504=CARTESIAN_POINT('Ctrl Pts',(-18.2423345282347,34.5120590688404,123.107437291874)) ;
#83505=CARTESIAN_POINT('Ctrl Pts',(-18.3119591424953,34.5219442804248,122.911604455747)) ;
#83506=CARTESIAN_POINT('Ctrl Pts',(-18.4154468238259,34.5319432106267,122.728669490148)) ;
#83507=CARTESIAN_POINT('Ctrl Pts',(-18.5479551281842,34.5418606335371,122.567652774081)) ;
#83508=CARTESIAN_POINT('Ctrl Pts',(-18.7084701842232,34.5519085656159,122.430380022431)) ;
#83509=CARTESIAN_POINT('Ctrl Pts',(-18.8872472231273,34.5617859414253,122.324675785033)) ;
#83510=CARTESIAN_POINT('Ctrl Pts',(-19.0850314861629,34.5718398345932,122.250237672887)) ;
#83511=CARTESIAN_POINT('Ctrl Pts',(-19.2894839508418,34.5817334578465,122.211783907264)) ;
#83512=CARTESIAN_POINT('Ctrl Pts',(-19.5009836238309,34.5917960514695,122.20934143813)) ;
#83513=CARTESIAN_POINT('Ctrl Pts',(-19.7052052787397,34.6016386254585,122.242811571831)) ;
#83514=CARTESIAN_POINT('Ctrl Pts',(-19.9035702129768,34.6116293823415,122.311773012743)) ;
#83515=CARTESIAN_POINT('Ctrl Pts',(-20.0858114401487,34.6215574440994,122.413537172417)) ;
#83516=CARTESIAN_POINT('Ctrl Pts',(-20.2488208163427,34.6315454199886,122.545909746572)) ;
#83517=CARTESIAN_POINT('Ctrl Pts',(-20.3867503190561,34.641581084345,122.705552977548)) ;
#83518=CARTESIAN_POINT('Ctrl Pts',(-20.4932169413994,34.6514370227647,122.883323165584)) ;
#83519=CARTESIAN_POINT('Ctrl Pts',(-20.5685573101781,34.6614325141616,123.079465842186)) ;
#83520=CARTESIAN_POINT('Ctrl Pts',(-20.6084203324499,34.671342319115,123.283961991978)) ;
#83521=CARTESIAN_POINT('Ctrl Pts',(-20.612551190647,34.6813545413818,123.494414786544)) ;
#83522=CARTESIAN_POINT('Ctrl Pts',(-20.5796204241671,34.6913824220746,123.70264640733)) ;
#83523=CARTESIAN_POINT('Ctrl Pts',(-20.5125423139285,34.7012388180572,123.898699508043)) ;
#83524=CARTESIAN_POINT('Ctrl Pts',(-20.4111153015867,34.7112636152372,124.083444109091)) ;
#83525=CARTESIAN_POINT('Ctrl Pts',(-20.2786642763012,34.721294545221,124.247549925688)) ;
#83526=CARTESIAN_POINT('Ctrl Pts',(-20.1229410884498,34.7311391477296,124.383860215577)) ;
#83527=CARTESIAN_POINT('Ctrl Pts',(-19.9435694586071,34.7411299989537,124.493149983065)) ;
#83528=CARTESIAN_POINT('Ctrl Pts',(-19.746860411412,34.751167831965,124.5695515535)) ;
#83529=CARTESIAN_POINT('Ctrl Pts',(-19.543924430635,34.7610122204304,124.610202433286)) ;
#83530=CARTESIAN_POINT('Ctrl Pts',(-19.3341067512897,34.7709970248,124.61548205464)) ;
#83531=CARTESIAN_POINT('Ctrl Pts',(-19.1274314289972,34.7809365442828,124.58447308467)) ;
#83532=CARTESIAN_POINT('Ctrl Pts',(-18.9273406268735,34.7909762752842,124.517347067221)) ;
#83533=CARTESIAN_POINT('Ctrl Pts',(-18.7446690785949,34.8008644035305,124.418099723713)) ;
#83534=CARTESIAN_POINT('Ctrl Pts',(-18.5801062236572,34.810854128739,124.287630585747)) ;
#83535=CARTESIAN_POINT('Ctrl Pts',(-18.4412525822457,34.8208118934405,124.130968222616)) ;
#83536=CARTESIAN_POINT('Ctrl Pts',(-18.3318983026168,34.8307142348525,123.953816542597)) ;
#83537=CARTESIAN_POINT('Ctrl Pts',(-18.2538875050456,34.8407584305589,123.757605403826)) ;
#83538=CARTESIAN_POINT('Ctrl Pts',(-18.2116860598952,34.8506658313181,123.553629678819)) ;
#83539=CARTESIAN_POINT('Ctrl Pts',(-18.2051086185152,34.8606764311925,123.343275057012)) ;
#83540=CARTESIAN_POINT('Ctrl Pts',(-18.2356186127828,34.8707067271047,123.134619193214)) ;
#83541=CARTESIAN_POINT('Ctrl Pts',(-18.3004560794895,34.8805615067544,122.937861249696)) ;
#83542=CARTESIAN_POINT('Ctrl Pts',(-18.3989387378507,34.8905188349719,122.753132034152)) ;
#83543=CARTESIAN_POINT('Ctrl Pts',(-18.5293404007521,34.9005578678788,122.587203276214)) ;
#83544=CARTESIAN_POINT('Ctrl Pts',(-18.683750583713,34.9104309797681,122.448444456777)) ;
#83545=CARTESIAN_POINT('Ctrl Pts',(-18.8634484884761,34.9205042647952,122.336472021751)) ;
#83546=CARTESIAN_POINT('Ctrl Pts',(-19.0549066208828,34.9303245845319,122.259103627693)) ;
#83547=CARTESIAN_POINT('Ctrl Pts',(-19.2620674122068,34.9404032499104,122.214853274735)) ;
#83548=CARTESIAN_POINT('Ctrl Pts',(-19.4690914445195,34.9502548403942,122.20734023343)) ;
#83549=CARTESIAN_POINT('Ctrl Pts',(-19.678827834024,34.9603279907131,122.236334586812)) ;
#83550=CARTESIAN_POINT('Ctrl Pts',(-19.8757733045073,34.9701703706881,122.299862342837)) ;
#83551=CARTESIAN_POINT('Ctrl Pts',(-20.0615624802536,34.9801513469312,122.397356517618)) ;
#83552=CARTESIAN_POINT('Ctrl Pts',(-20.2279932750896,34.9901676752865,122.526380482302)) ;
#83553=CARTESIAN_POINT('Ctrl Pts',(-20.3680015083541,35.0000654722776,122.680305185456)) ;
#83554=CARTESIAN_POINT('Ctrl Pts',(-20.4807624809088,35.0100780290097,122.858068616556)) ;
#83555=CARTESIAN_POINT('Ctrl Pts',(-20.5606293993348,35.0201100638562,123.053255739191)) ;
#83556=CARTESIAN_POINT('Ctrl Pts',(-20.6050415900168,35.0299494646716,123.255303485779)) ;
#83557=CARTESIAN_POINT('Ctrl Pts',(-20.6140547299555,35.0400152503232,123.466701668536)) ;
#83558=CARTESIAN_POINT('Ctrl Pts',(-20.5866072578228,35.0499057054378,123.672832352002)) ;
#83559=CARTESIAN_POINT('Ctrl Pts',(-20.5235800737394,35.0598978240735,123.873208904789)) ;
#83560=CARTESIAN_POINT('Ctrl Pts',(-20.4268258300591,35.0698606508366,124.058965811028)) ;
#83561=CARTESIAN_POINT('Ctrl Pts',(-20.3004423219117,35.0797649341095,124.224463820885)) ;
#83562=CARTESIAN_POINT('Ctrl Pts',(-20.1447351796746,35.0898253680566,124.367564128807)) ;
#83563=CARTESIAN_POINT('Ctrl Pts',(-19.9705404840006,35.0996659207298,124.479217042603)) ;
#83564=CARTESIAN_POINT('Ctrl Pts',(-19.775454299902,35.1097281406755,124.560953485022)) ;
#83565=CARTESIAN_POINT('Ctrl Pts',(-19.5724444891805,35.119625279954,124.606605440931)) ;
#83566=CARTESIAN_POINT('Ctrl Pts',(-19.3639245804483,35.1295564720891,124.617042217637)) ;
#83567=CARTESIAN_POINT('Ctrl Pts',(-19.1544758293092,35.1395986267342,124.590591188997)) ;
#83568=CARTESIAN_POINT('Ctrl Pts',(-18.9558504881667,35.1494853877535,124.52929739217)) ;
#83569=CARTESIAN_POINT('Ctrl Pts',(-18.7686967842373,35.1594846894707,124.433626676918)) ;
#83570=CARTESIAN_POINT('Ctrl Pts',(-18.6021840039089,35.1694054876375,124.307986902434)) ;
#83571=CARTESIAN_POINT('Ctrl Pts',(-18.4584119398437,35.1794395412342,124.153654272285)) ;
#83572=CARTESIAN_POINT('Ctrl Pts',(-18.3447544017699,35.1893626588006,123.978681426512)) ;
#83573=CARTESIAN_POINT('Ctrl Pts',(-18.2621745123595,35.1994187822997,123.784088489185)) ;
#83574=CARTESIAN_POINT('Ctrl Pts',(-18.2155383684478,35.2092642239545,123.582420316723)) ;
#83575=CARTESIAN_POINT('Ctrl Pts',(-18.2038107386585,35.2192265250787,123.373323341411)) ;
#83576=CARTESIAN_POINT('Ctrl Pts',(-18.2290111975994,35.2292550043538,123.16399026275)) ;
#83577=CARTESIAN_POINT('Ctrl Pts',(-18.2893801566425,35.2391653578635,122.964592181347)) ;
#83578=CARTESIAN_POINT('Ctrl Pts',(-18.3832066496104,35.2491002300407,122.777983945553)) ;
#83579=CARTESIAN_POINT('Ctrl Pts',(-18.5094937587254,35.2591413676264,122.608837914047)) ;
#83580=CARTESIAN_POINT('Ctrl Pts',(-18.6607872589449,35.2690285168409,122.46628852353)) ;
#83581=CARTESIAN_POINT('Ctrl Pts',(-18.8361660023692,35.279020751592,122.350681667072)) ;
#83582=CARTESIAN_POINT('Ctrl Pts',(-19.0281614512113,35.288969457155,122.267692165554)) ;
#83583=CARTESIAN_POINT('Ctrl Pts',(-19.2312959711642,35.2989055255787,122.219071218612)) ;
#83584=CARTESIAN_POINT('Ctrl Pts',(-19.4408495262732,35.3088912097945,122.206154757803)) ;
#83585=CARTESIAN_POINT('Ctrl Pts',(-19.6505366990128,35.3189316363631,122.230278771778)) ;
#83586=CARTESIAN_POINT('Ctrl Pts',(-19.8489056511922,35.3287707498269,122.288911025244)) ;
#83587=CARTESIAN_POINT('Ctrl Pts',(-20.0378790782979,35.3388004840027,122.382455871339)) ;
#83588=CARTESIAN_POINT('Ctrl Pts',(-20.2072811529409,35.3488225835086,122.507735654977)) ;
#83589=CARTESIAN_POINT('Ctrl Pts',(-20.3505219702096,35.358691023402,122.657836946013)) ;
#83590=CARTESIAN_POINT('Ctrl Pts',(-20.4678365484085,35.3687598880876,122.83401133288)) ;
#83591=CARTESIAN_POINT('Ctrl Pts',(-20.5508879121588,35.3786025611862,123.023544397002)) ;
#83592=CARTESIAN_POINT('Ctrl Pts',(-20.6010962703193,35.3885631953487,123.226835535581)) ;
#83593=CARTESIAN_POINT('Ctrl Pts',(-20.6149388902107,35.3986011110268,123.437402313412)) ;
#83594=CARTESIAN_POINT('Ctrl Pts',(-20.5927617522168,35.4084753858862,123.643828081637)) ;
#83595=CARTESIAN_POINT('Ctrl Pts',(-20.5339407377704,35.4185451362614,123.847160643849)) ;
#83596=CARTESIAN_POINT('Ctrl Pts',(-20.4429777575099,35.4283784316359,124.03281763608)) ;
#83597=CARTESIAN_POINT('Ctrl Pts',(-20.3192176499442,35.4384087291155,124.203541031282)) ;
#83598=CARTESIAN_POINT('Ctrl Pts',(-20.16722456801,35.4484408155569,124.349771846987)) ;
#83599=CARTESIAN_POINT('Ctrl Pts',(-19.9959822051023,35.4582687440459,124.465363734723)) ;
#83600=CARTESIAN_POINT('Ctrl Pts',(-19.8042655640966,35.4682647851566,124.551422946889)) ;
#83601=CARTESIAN_POINT('Ctrl Pts',(-19.5998043217573,35.4782905972579,124.602646565029)) ;
#83602=CARTESIAN_POINT('Ctrl Pts',(-19.392483122797,35.4881778321527,124.617652844569)) ;
#83603=CARTESIAN_POINT('Ctrl Pts',(-19.1838143097851,35.4981546983637,124.596588858927)) ;
#83604=CARTESIAN_POINT('Ctrl Pts',(-18.9815944245208,35.5081476422355,124.539544119741)) ;
#83605=CARTESIAN_POINT('Ctrl Pts',(-18.7916564256267,35.5181855649069,124.447621093285)) ;
#83606=CARTESIAN_POINT('Ctrl Pts',(-18.623585679529,35.5280340291686,124.326680948825)) ;
#83607=CARTESIAN_POINT('Ctrl Pts',(-18.4767269345962,35.5380258959126,124.176530851777)) ;
#83608=CARTESIAN_POINT('Ctrl Pts',(-18.3589196028122,35.5479436279538,124.004467615478)) ;
#83609=CARTESIAN_POINT('Ctrl Pts',(-18.2717855237114,35.557971812849,123.812511474511)) ;
#83610=CARTESIAN_POINT('Ctrl Pts',(-18.2199640326758,35.5678569708979,123.611253900228)) ;
#83611=CARTESIAN_POINT('Ctrl Pts',(-18.2031956371269,35.5778463314396,123.401912404642)) ;
#83612=CARTESIAN_POINT('Ctrl Pts',(-18.2235772732531,35.5878874883739,123.19180201946)) ;
#83613=CARTESIAN_POINT('Ctrl Pts',(-18.2786256492768,35.5977200718291,122.992558401148)) ;
#83614=CARTESIAN_POINT('Ctrl Pts',(-18.368354397371,35.6077142917911,122.802574694399)) ;
#83615=CARTESIAN_POINT('Ctrl Pts',(-18.4904752636947,35.6177423935784,122.630717576888)) ;
#83616=CARTESIAN_POINT('Ctrl Pts',(-18.6381538687161,35.6276223382014,122.484653315381)) ;
#83617=CARTESIAN_POINT('Ctrl Pts',(-18.8106615035911,35.6376126647585,122.364871615126)) ;
#83618=CARTESIAN_POINT('Ctrl Pts',(-19.0004190126746,35.6475535964128,122.277289203109)) ;
#83619=CARTESIAN_POINT('Ctrl Pts',(-19.203373565365,35.6575407149157,122.223445031076)) ;
#83620=CARTESIAN_POINT('Ctrl Pts',(-19.4135608775624,35.6675740478129,122.205909966889)) ;
#83621=CARTESIAN_POINT('Ctrl Pts',(-19.6201740270743,35.6774401522576,122.224414930449)) ;
#83622=CARTESIAN_POINT('Ctrl Pts',(-19.8244618404045,35.6875062661379,122.279549955093)) ;
#83623=CARTESIAN_POINT('Ctrl Pts',(-20.0121134212357,35.6973622779064,122.367450472132)) ;
#83624=CARTESIAN_POINT('Ctrl Pts',(-20.1843772744917,35.7073569815377,122.487755292346)) ;
#83625=CARTESIAN_POINT('Ctrl Pts',(-20.3333683513366,35.7173883172625,122.637013317977)) ;
#83626=CARTESIAN_POINT('Ctrl Pts',(-20.4524676775641,35.7272548424662,122.806847353514)) ;
#83627=CARTESIAN_POINT('Ctrl Pts',(-20.5416380597562,35.737242270512,122.996911535405)) ;
#83628=CARTESIAN_POINT('Ctrl Pts',(-20.5963428018029,35.7471872001984,123.198733454628)) ;
#83629=CARTESIAN_POINT('Ctrl Pts',(-20.6152390420274,35.7572321183069,123.409042028494)) ;
#83630=CARTESIAN_POINT('Ctrl Pts',(-20.5978399960011,35.7670940879208,123.615657169133)) ;
#83631=CARTESIAN_POINT('Ctrl Pts',(-20.5445360900848,35.7770861559421,123.818824883138)) ;
#83632=CARTESIAN_POINT('Ctrl Pts',(-20.4572545323624,35.7870170813166,124.008498783823)) ;
#83633=CARTESIAN_POINT('Ctrl Pts',(-20.3384335820411,35.7969677095401,124.180653507785)) ;
#83634=CARTESIAN_POINT('Ctrl Pts',(-20.1908529728622,35.8069679485992,124.330416617571)) ;
#83635=CARTESIAN_POINT('Ctrl Pts',(-20.0188759857956,35.8169964039684,124.452357630872)) ;
#83636=CARTESIAN_POINT('Ctrl Pts',(-19.8315424729774,35.8268624385517,124.541414625509)) ;
#83637=CARTESIAN_POINT('Ctrl Pts',(-19.6291530298496,35.8368547602991,124.597623082846)) ;
#83638=CARTESIAN_POINT('Ctrl Pts',(-19.4213005157174,35.8467870499761,124.61775207134)) ;
#83639=CARTESIAN_POINT('Ctrl Pts',(-19.211666492633,35.8567886949468,124.601579008395)) ;
#83640=CARTESIAN_POINT('Ctrl Pts',(-18.9405973697482,35.8701013283629,124.531802097679)) ;
#83641=CARTESIAN_POINT('Ctrl Pts',(-18.6953541163112,35.8833330777444,124.393908284791)) ;
#83642=CARTESIAN_POINT('Ctrl Pts',(-18.4950059200478,35.8966563425615,124.19822486619)) ;
#83643=CARTESIAN_POINT('Ctrl Pts',(-18.3736554135811,35.9065320487792,124.029742314884)) ;
#83644=CARTESIAN_POINT('Ctrl Pts',(-18.2821355538352,35.9165216398792,123.840747272205)) ;
#83645=CARTESIAN_POINT('Ctrl Pts',(-18.2250326647968,35.9264487363346,123.639986046386)) ;
#83646=CARTESIAN_POINT('Ctrl Pts',(-18.2034246484447,35.9364738848392,123.430355376024)) ;
#83647=CARTESIAN_POINT('Ctrl Pts',(-18.218222177825,35.9463695389859,123.222826192878)) ;
#83648=CARTESIAN_POINT('Ctrl Pts',(-18.2690819771899,35.9563730733641,123.018783675102)) ;
#83649=CARTESIAN_POINT('Ctrl Pts',(-18.3544809763552,35.9663582118041,122.826985698645)) ;
#83650=CARTESIAN_POINT('Ctrl Pts',(-18.4726337060775,35.9763941363995,122.652198310176)) ;
#83651=CARTESIAN_POINT('Ctrl Pts',(-18.6164712051897,35.9862454118272,122.503192825929)) ;
#83652=CARTESIAN_POINT('Ctrl Pts',(-18.7860469770092,35.9962376729885,122.379193148442)) ;
#83653=CARTESIAN_POINT('Ctrl Pts',(-18.9756946417762,36.0062775570061,122.286567052607)) ;
#83654=CARTESIAN_POINT('Ctrl Pts',(-19.1742898211919,36.0161123315086,122.228953645098)) ;
#83655=CARTESIAN_POINT('Ctrl Pts',(-19.3848548302103,36.0261887125289,122.206080564844)) ;
#83656=CARTESIAN_POINT('Ctrl Pts',(-19.5914291862838,36.0360349856795,122.219742059449)) ;
#83657=CARTESIAN_POINT('Ctrl Pts',(-19.8644347267717,36.0493995069647,122.286166574249)) ;
#83658=CARTESIAN_POINT('Ctrl Pts',(-20.1107389390427,36.0626057513992,122.421071137189)) ;
#83659=CARTESIAN_POINT('Ctrl Pts',(-20.3128956661837,36.0758707060764,122.613085888176)) ;
#83660=CARTESIAN_POINT('Ctrl Pts',(-20.4382108216345,36.0859029866281,122.782748260018)) ;
#83661=CARTESIAN_POINT('Ctrl Pts',(-20.5310088524388,36.095811720146,122.969242493688)) ;
#83662=CARTESIAN_POINT('Ctrl Pts',(-20.5907141654176,36.1057492710135,123.169457023205)) ;
#83663=CARTESIAN_POINT('Ctrl Pts',(-20.6147942216351,36.1157791186074,123.378913624605)) ;
#83664=CARTESIAN_POINT('Ctrl Pts',(-20.5984716755817,36.1290142585278,123.656761647636)) ;
#83665=CARTESIAN_POINT('Ctrl Pts',(-20.4868793174588,36.145682722899,123.993019408595)) ;
#83666=CARTESIAN_POINT('Ctrl Pts',(-20.225147237261,36.1655537347729,124.324870584311)) ;
#83667=CARTESIAN_POINT('Ctrl Pts',(-19.9231598859888,36.1822608191559,124.511857502732)) ;
#83668=CARTESIAN_POINT('Ctrl Pts',(-19.6579098007615,36.1954381004665,124.59178022723)) ;
#83669=CARTESIAN_POINT('Ctrl Pts',(-19.3810457926493,36.2087055609806,124.625650251506)) ;
#83670=CARTESIAN_POINT('Ctrl Pts',(-19.031245809974,36.2253194516678,124.576426839473)) ;
#83671=CARTESIAN_POINT('Ctrl Pts',(-18.656546623084,36.2452682510952,124.377542791956)) ;
#83672=CARTESIAN_POINT('Ctrl Pts',(-18.3727286129065,36.265189362626,124.063195119709)) ;
#83673=CARTESIAN_POINT('Ctrl Pts',(-18.2127928763886,36.2850558107989,123.672157333383)) ;
#83674=CARTESIAN_POINT('Ctrl Pts',(-18.1960230951589,36.305082157416,123.246720338443)) ;
#83675=CARTESIAN_POINT('Ctrl Pts',(-18.3244917453936,36.3249442018056,122.844336519412)) ;
#83676=CARTESIAN_POINT('Ctrl Pts',(-18.5830321625222,36.3448895044867,122.508241908739)) ;
#83677=CARTESIAN_POINT('Ctrl Pts',(-18.9399427386742,36.3647848115456,122.281138173914)) ;
#83678=CARTESIAN_POINT('Ctrl Pts',(-19.3527183542738,36.3846780817132,122.188728150166)) ;
#83679=CARTESIAN_POINT('Ctrl Pts',(-19.7737310767519,36.4046436743936,122.243004278236)) ;
#83680=CARTESIAN_POINT('Ctrl Pts',(-20.1494256309747,36.4245189980784,122.436570970355)) ;
#83681=CARTESIAN_POINT('Ctrl Pts',(-20.4382669875534,36.4444940606534,122.747982616058)) ;
#83682=CARTESIAN_POINT('Ctrl Pts',(-20.6027131203733,36.4644464702845,123.139055928244)) ;
#83683=CARTESIAN_POINT('Ctrl Pts',(-20.6245287326153,36.4842825245207,123.560259041129)) ;
#83684=CARTESIAN_POINT('Ctrl Pts',(-20.5008694423809,36.5042604359382,123.966645206898)) ;
#83685=CARTESIAN_POINT('Ctrl Pts',(-20.2463345705319,36.5241784854417,124.305097676142)) ;
#83686=CARTESIAN_POINT('Ctrl Pts',(-19.8929822057688,36.5440466292098,124.536788634087)) ;
#83687=CARTESIAN_POINT('Ctrl Pts',(-19.4780342144417,36.5640974857971,124.63420462861)) ;
#83688=CARTESIAN_POINT('Ctrl Pts',(-19.0601853486315,36.583877922253,124.585267888838)) ;
#83689=CARTESIAN_POINT('Ctrl Pts',(-18.679261467487,36.6039079779308,124.395005365554)) ;
#83690=CARTESIAN_POINT('Ctrl Pts',(-18.3887179656958,36.6237890831056,124.087851983068)) ;
#83691=CARTESIAN_POINT('Ctrl Pts',(-18.2193877468624,36.6436695454733,123.700582763927)) ;
#83692=CARTESIAN_POINT('Ctrl Pts',(-18.19234690507,36.6636546926177,123.276492035899)) ;
#83693=CARTESIAN_POINT('Ctrl Pts',(-18.3111820310243,36.6835452711541,122.870593167855)) ;
#83694=CARTESIAN_POINT('Ctrl Pts',(-18.5608264774921,36.7034392910285,122.52912278026)) ;
#83695=CARTESIAN_POINT('Ctrl Pts',(-18.9123819271041,36.7233607357549,122.292957389509)) ;
#83696=CARTESIAN_POINT('Ctrl Pts',(-19.3229430451525,36.7432588738103,122.190279959009)) ;
#83697=CARTESIAN_POINT('Ctrl Pts',(-19.7472711559483,36.7633296290264,122.23504109074)) ;
#83698=CARTESIAN_POINT('Ctrl Pts',(-20.1256424620349,36.7831151790776,122.419154427526)) ;
#83699=CARTESIAN_POINT('Ctrl Pts',(-20.4220170617102,36.803098253955,122.723507791332)) ;
#83700=CARTESIAN_POINT('Ctrl Pts',(-20.5955264961768,36.8230073366009,123.109641754048)) ;
#83701=CARTESIAN_POINT('Ctrl Pts',(-20.6279926914676,36.8428658957237,123.530692354676)) ;
#83702=CARTESIAN_POINT('Ctrl Pts',(-20.5133249107813,36.8629093395624,123.941072173113)) ;
#83703=CARTESIAN_POINT('Ctrl Pts',(-20.3093891442203,36.8794094042916,124.226640227204)) ;
#83704=CARTESIAN_POINT('Ctrl Pts',(-20.0922744150235,36.8927991441405,124.405775148074)) ;
#83705=CARTESIAN_POINT('Ctrl Pts',(-19.9119759265063,36.9026560453489,124.507969785609)) ;
#83706=CARTESIAN_POINT('Ctrl Pts',(-19.7142026391897,36.9126475711954,124.578640987021)) ;
#83707=CARTESIAN_POINT('Ctrl Pts',(-19.5084997100281,36.9225722516463,124.613748997365)) ;
#83708=CARTESIAN_POINT('Ctrl Pts',(-19.2980712246021,36.9325828416907,124.612675113319)) ;
#83709=CARTESIAN_POINT('Ctrl Pts',(-19.0237190251931,36.9458421023944,124.563191736342)) ;
#83710=CARTESIAN_POINT('Ctrl Pts',(-18.767004640469,36.9591931775447,124.442157944638)) ;
#83711=CARTESIAN_POINT('Ctrl Pts',(-18.554897868614,36.9723994867795,124.262901619475)) ;
#83712=CARTESIAN_POINT('Ctrl Pts',(-18.4202072573084,36.9823863203698,124.101894877221)) ;
#83713=CARTESIAN_POINT('Ctrl Pts',(-18.3157478310431,36.9923390478658,123.920555058414)) ;
#83714=CARTESIAN_POINT('Ctrl Pts',(-18.2438653347165,37.0023871447074,123.721943582903)) ;
#83715=CARTESIAN_POINT('Ctrl Pts',(-18.2080589055082,37.0122286015793,123.518146563826)) ;
#83716=CARTESIAN_POINT('Ctrl Pts',(-18.2077355256996,37.0222148684928,123.308238341924)) ;
#83717=CARTESIAN_POINT('Ctrl Pts',(-18.2435931027669,37.0321514693932,123.102404826661)) ;
#83718=CARTESIAN_POINT('Ctrl Pts',(-18.3155367162439,37.0422014121802,122.903771955819)) ;
#83719=CARTESIAN_POINT('Ctrl Pts',(-18.4186658037517,37.052051611866,122.724179687361)) ;
#83720=CARTESIAN_POINT('Ctrl Pts',(-18.5526159351476,37.0620245167981,122.562916724889)) ;
#83721=CARTESIAN_POINT('Ctrl Pts',(-18.7130217569356,37.0720228912777,122.427035007619)) ;
#83722=CARTESIAN_POINT('Ctrl Pts',(-18.8950290315818,37.0820430651477,122.320985383453)) ;
#83723=CARTESIAN_POINT('Ctrl Pts',(-19.0902841551798,37.0919441090897,122.248841936887)) ;
#83724=CARTESIAN_POINT('Ctrl Pts',(-19.296849422935,37.101932912814,122.211043584546)) ;
#83725=CARTESIAN_POINT('Ctrl Pts',(-19.5063417583613,37.1118983796458,122.209838368908)) ;
#83726=CARTESIAN_POINT('Ctrl Pts',(-19.7116920048539,37.1218019419188,122.244315913118)) ;
#83727=CARTESIAN_POINT('Ctrl Pts',(-19.9109467756604,37.1318626197968,122.315177850177)) ;
#83728=CARTESIAN_POINT('Ctrl Pts',(-20.0910226055792,37.1417029177462,122.417070024375)) ;
#83729=CARTESIAN_POINT('Ctrl Pts',(-20.2544023733536,37.1517659126557,122.551425194411)) ;
#83730=CARTESIAN_POINT('Ctrl Pts',(-20.3895668547775,37.1616602068028,122.709563454073)) ;
#83731=CARTESIAN_POINT('Ctrl Pts',(-20.496191309324,37.1716020044997,122.889298737266)) ;
#83732=CARTESIAN_POINT('Ctrl Pts',(-20.5705305806763,37.1816045820288,123.086035719177)) ;
#83733=CARTESIAN_POINT('Ctrl Pts',(-20.6093785758496,37.1916390459499,123.293373240593)) ;
#83734=CARTESIAN_POINT('Ctrl Pts',(-20.6119178344459,37.2014851844709,123.500360820734)) ;
#83735=CARTESIAN_POINT('Ctrl Pts',(-20.5784854248412,37.2114663577079,123.707499064364)) ;
#83736=CARTESIAN_POINT('Ctrl Pts',(-20.5097396929773,37.2214186516652,123.905117967548)) ;
#83737=CARTESIAN_POINT('Ctrl Pts',(-20.4074820202486,37.2314174467998,124.088793919153)) ;
#83738=CARTESIAN_POINT('Ctrl Pts',(-20.2740542843056,37.2414565550606,124.252304030072)) ;
#83739=CARTESIAN_POINT('Ctrl Pts',(-20.1179432203303,37.2512814964997,124.387573712776)) ;
#83740=CARTESIAN_POINT('Ctrl Pts',(-19.9367725786366,37.2613361835741,124.496449030684)) ;
#83741=CARTESIAN_POINT('Ctrl Pts',(-19.7414996689974,37.2712789885143,124.571043200501)) ;
#83742=CARTESIAN_POINT('Ctrl Pts',(-19.5371698877541,37.2811827745108,124.611070181106)) ;
#83743=CARTESIAN_POINT('Ctrl Pts',(-19.3260077883793,37.2912295910756,124.61493909619)) ;
#83744=CARTESIAN_POINT('Ctrl Pts',(-19.1204430941798,37.3011251105543,124.582756712364)) ;
#83745=CARTESIAN_POINT('Ctrl Pts',(-18.9203358363099,37.3111871958787,124.514257554786)) ;
#83746=CARTESIAN_POINT('Ctrl Pts',(-18.7390960612812,37.3210299068366,124.41436004309)) ;
#83747=CARTESIAN_POINT('Ctrl Pts',(-18.5752583699515,37.3310206241427,124.282977391372)) ;
#83748=CARTESIAN_POINT('Ctrl Pts',(-18.4375935777154,37.3409487072392,124.126081569931)) ;
#83749=CARTESIAN_POINT('Ctrl Pts',(-18.3282968872261,37.350936637351,123.946781561077)) ;
#83750=CARTESIAN_POINT('Ctrl Pts',(-18.2517622204331,37.3609724634783,123.750174847478)) ;
#83751=CARTESIAN_POINT('Ctrl Pts',(-18.2109407997604,37.3708278005919,123.547034393052)) ;
#83752=CARTESIAN_POINT('Ctrl Pts',(-18.2056086311467,37.3808255354421,123.336940852331)) ;
#83753=CARTESIAN_POINT('Ctrl Pts',(-18.2364910721176,37.3907334394265,123.130938228114)) ;
#83754=CARTESIAN_POINT('Ctrl Pts',(-18.303026933122,37.400744513975,122.931261324963)) ;
#83755=CARTESIAN_POINT('Ctrl Pts',(-18.4037673378414,37.4107723695106,122.746069528211)) ;
#83756=CARTESIAN_POINT('Ctrl Pts',(-18.5326081128245,37.4206299634158,122.583754393451)) ;
#83757=CARTESIAN_POINT('Ctrl Pts',(-18.6900546247519,37.4306566502539,122.44359153337)) ;
#83758=CARTESIAN_POINT('Ctrl Pts',(-18.8697607051448,37.4406853194077,122.333319595354)) ;
#83759=CARTESIAN_POINT('Ctrl Pts',(-19.0621377283289,37.4505305276891,122.256989623599)) ;
#83760=CARTESIAN_POINT('Ctrl Pts',(-19.2677422232173,37.4605212166522,122.214048076628)) ;
#83761=CARTESIAN_POINT('Ctrl Pts',(-19.4786785246119,37.4705590929345,122.207898022641)) ;
#83762=CARTESIAN_POINT('Ctrl Pts',(-19.6835147870489,37.4804034705767,122.237521469835)) ;
#83763=CARTESIAN_POINT('Ctrl Pts',(-19.882996095527,37.4903882749681,122.302778964749)) ;
#83764=CARTESIAN_POINT('Ctrl Pts',(-20.0673693745768,37.5003278051867,122.401180197241)) ;
#83765=CARTESIAN_POINT('Ctrl Pts',(-20.2334482168437,37.5103674932236,122.531409815803)) ;
#83766=CARTESIAN_POINT('Ctrl Pts',(-20.3723615434971,37.5202557825919,122.686081229765)) ;
#83767=CARTESIAN_POINT('Ctrl Pts',(-20.4837564567188,37.5302449062767,122.864096075934)) ;
#83768=CARTESIAN_POINT('Ctrl Pts',(-20.5621702921538,37.5402049159513,123.058246148547)) ;
#83769=CARTESIAN_POINT('Ctrl Pts',(-20.6059089803281,37.5501053456555,123.261743082962)) ;
#83770=CARTESIAN_POINT('Ctrl Pts',(-20.6137506150888,37.5601484270623,123.47272578721)) ;
#83771=CARTESIAN_POINT('Ctrl Pts',(-20.5852316440179,37.5700558209699,123.679059674677)) ;
#83772=CARTESIAN_POINT('Ctrl Pts',(-20.5210197943171,37.5800675519591,123.879505655746)) ;
#83773=CARTESIAN_POINT('Ctrl Pts',(-20.4224065041356,37.5900997696738,124.065948303167)) ;
#83774=CARTESIAN_POINT('Ctrl Pts',(-20.2954706315988,37.59995227892,124.229610493564)) ;
#83775=CARTESIAN_POINT('Ctrl Pts',(-20.1408283212273,37.609910215463,124.370729363786)) ;
#83776=CARTESIAN_POINT('Ctrl Pts',(-19.9624090573161,37.6199490854713,124.48343363066)) ;
#83777=CARTESIAN_POINT('Ctrl Pts',(-19.7704588435921,37.6298222406296,124.562502743437)) ;
#83778=CARTESIAN_POINT('Ctrl Pts',(-19.5636464572191,37.6398955154793,124.607865012722)) ;
#83779=CARTESIAN_POINT('Ctrl Pts',(-19.3573352443777,37.6497158326567,124.616683318652)) ;
#83780=CARTESIAN_POINT('Ctrl Pts',(-19.1473126609859,37.6597945184502,124.589037290867)) ;
#83781=CARTESIAN_POINT('Ctrl Pts',(-18.9497170068523,37.6696460298333,124.526820882821)) ;
#83782=CARTESIAN_POINT('Ctrl Pts',(-18.7617822134983,37.6797194761399,124.429288117211)) ;
#83783=CARTESIAN_POINT('Ctrl Pts',(-18.5974727396535,37.6895607512646,124.303521835439)) ;
#83784=CARTESIAN_POINT('Ctrl Pts',(-18.4549977309688,37.6995458509214,124.149384967092)) ;
#83785=CARTESIAN_POINT('Ctrl Pts',(-18.3414230044762,37.7095533270557,123.972266854178)) ;
#83786=CARTESIAN_POINT('Ctrl Pts',(-18.2608486938713,37.7194759147646,123.779863616156)) ;
#83787=CARTESIAN_POINT('Ctrl Pts',(-18.2142702298317,37.729462519038,123.575125889961)) ;
#83788=CARTESIAN_POINT('Ctrl Pts',(-18.2042901761544,37.7395026473721,123.364303674408)) ;
#83789=CARTESIAN_POINT('Ctrl Pts',(-18.2300893061444,37.7493420819055,123.159042211176)) ;
#83790=CARTESIAN_POINT('Ctrl Pts',(-18.2923486019064,37.7594061363965,122.956858603344)) ;
#83791=CARTESIAN_POINT('Ctrl Pts',(-18.3872136998659,37.7692970556336,122.77179660064)) ;
#83792=CARTESIAN_POINT('Ctrl Pts',(-18.5136767992949,37.7792890489397,122.60407891323)) ;
#83793=CARTESIAN_POINT('Ctrl Pts',(-18.6670286119021,37.789251912899,122.461423763276)) ;
#83794=CARTESIAN_POINT('Ctrl Pts',(-18.8415186737119,37.7991561727167,122.347777335576)) ;
#83795=CARTESIAN_POINT('Ctrl Pts',(-19.0361446776308,37.8092166632881,122.265052855607)) ;
#83796=CARTESIAN_POINT('Ctrl Pts',(-19.2376613638147,37.8190570129192,122.218146463825)) ;
#83797=CARTESIAN_POINT('Ctrl Pts',(-19.4488650436602,37.8291199884092,122.206437418726)) ;
#83798=CARTESIAN_POINT('Ctrl Pts',(-19.6554019408263,37.8390143085526,122.231332716202)) ;
#83799=CARTESIAN_POINT('Ctrl Pts',(-19.8555475570371,37.8489560216842,122.291445922081)) ;
#83800=CARTESIAN_POINT('Ctrl Pts',(-20.0434591182195,37.8589589114783,122.385921690692)) ;
#83801=CARTESIAN_POINT('Ctrl Pts',(-20.2124620853633,37.8689987686388,122.512333026513)) ;
#83802=CARTESIAN_POINT('Ctrl Pts',(-20.3542123367619,37.8788229494764,122.662567208184)) ;
#83803=CARTESIAN_POINT('Ctrl Pts',(-20.4706389075393,37.8888799229796,122.839032447305)) ;
#83804=CARTESIAN_POINT('Ctrl Pts',(-20.5533481466804,37.8988080471667,123.030678526418)) ;
#83805=CARTESIAN_POINT('Ctrl Pts',(-20.6021910285097,37.9087617422401,123.234157913246)) ;
#83806=CARTESIAN_POINT('Ctrl Pts',(-20.6147789282106,37.9188079358154,123.4449832549)) ;
#83807=CARTESIAN_POINT('Ctrl Pts',(-20.5912446252773,37.9286560381753,123.650677870567)) ;
#83808=CARTESIAN_POINT('Ctrl Pts',(-20.5322977195808,37.9386176264029,123.851625135048)) ;
#83809=CARTESIAN_POINT('Ctrl Pts',(-20.4384823086868,37.9486462965591,124.040450654678)) ;
#83810=CARTESIAN_POINT('Ctrl Pts',(-20.3148504533172,37.9585565994409,124.20813777863)) ;
#83811=CARTESIAN_POINT('Ctrl Pts',(-20.1639729427983,37.9684914832488,124.352574766539)) ;
#83812=CARTESIAN_POINT('Ctrl Pts',(-19.9883521310107,37.9785326249394,124.469690942097)) ;
#83813=CARTESIAN_POINT('Ctrl Pts',(-19.7980710765372,37.9884197461034,124.553374463438)) ;
#83814=CARTESIAN_POINT('Ctrl Pts',(-19.5941095918449,37.9984120889519,124.603607303031)) ;
#83815=CARTESIAN_POINT('Ctrl Pts',(-19.3854195842662,38.0083603901759,124.617543166151)) ;
#83816=CARTESIAN_POINT('Ctrl Pts',(-19.177694220947,38.018297967858,124.595361007265)) ;
#83817=CARTESIAN_POINT('Ctrl Pts',(-18.9759006217927,38.0282845423085,124.53736043578)) ;
#83818=CARTESIAN_POINT('Ctrl Pts',(-18.7865662327341,38.038313352217,124.444601890689)) ;
#83819=CARTESIAN_POINT('Ctrl Pts',(-18.6186516542393,38.0481916735238,124.322405716065)) ;
#83820=CARTESIAN_POINT('Ctrl Pts',(-18.472489585433,38.0581833208712,124.171531238114)) ;
#83821=CARTESIAN_POINT('Ctrl Pts',(-18.3546061530968,38.068217844309,123.996595612871)) ;
#83822=CARTESIAN_POINT('Ctrl Pts',(-18.2699432567758,38.0780812011876,123.807284310517)) ;
#83823=CARTESIAN_POINT('Ctrl Pts',(-18.2183482654027,38.0881514278679,123.601982881661)) ;
#83824=CARTESIAN_POINT('Ctrl Pts',(-18.2035357134123,38.0979937360026,123.395589024256)) ;
#83825=CARTESIAN_POINT('Ctrl Pts',(-18.2242703551438,38.107954468026,123.187217212771)) ;
#83826=CARTESIAN_POINT('Ctrl Pts',(-18.2817100388421,38.1179923572241,122.984164140469)) ;
#83827=CARTESIAN_POINT('Ctrl Pts',(-18.3717050512653,38.1278666401429,122.797069690323)) ;
#83828=CARTESIAN_POINT('Ctrl Pts',(-18.4951947344798,38.1379363847604,122.62515584992)) ;
#83829=CARTESIAN_POINT('Ctrl Pts',(-18.6430558971096,38.147769695106,122.480657473056)) ;
#83830=CARTESIAN_POINT('Ctrl Pts',(-18.816822434158,38.1577999384587,122.361207113094)) ;
#83831=CARTESIAN_POINT('Ctrl Pts',(-19.0089987785869,38.1678322264371,122.274295739322)) ;
#83832=CARTESIAN_POINT('Ctrl Pts',(-19.2090434292556,38.1776594029052,122.222666245532)) ;
#83833=CARTESIAN_POINT('Ctrl Pts',(-19.4186876276623,38.187664785772,122.205831123598)) ;
#83834=CARTESIAN_POINT('Ctrl Pts',(-19.627653582682,38.1976474247647,122.225683031831)) ;
#83835=CARTESIAN_POINT('Ctrl Pts',(-19.8311151594825,38.2076914919014,122.282093509122)) ;
#83836=CARTESIAN_POINT('Ctrl Pts',(-20.0176420041598,38.2175127107054,122.37064600163)) ;
#83837=CARTESIAN_POINT('Ctrl Pts',(-20.1899591987326,38.2275495496434,122.492420098757)) ;
#83838=CARTESIAN_POINT('Ctrl Pts',(-20.3379110188023,38.2375739617412,122.64250885033)) ;
#83839=CARTESIAN_POINT('Ctrl Pts',(-20.4558734175795,38.2474260461465,122.81276043771)) ;
#83840=CARTESIAN_POINT('Ctrl Pts',(-20.5439817152443,38.2574169428896,123.00339930315)) ;
#83841=CARTESIAN_POINT('Ctrl Pts',(-20.5974030969993,38.2673349347906,123.204972777987)) ;
#83842=CARTESIAN_POINT('Ctrl Pts',(-20.6152555329228,38.2773630502476,123.415021619111)) ;
#83843=CARTESIAN_POINT('Ctrl Pts',(-20.5967206678449,38.2872482261897,123.622015760556)) ;
#83844=CARTESIAN_POINT('Ctrl Pts',(-20.5424483507648,38.2972375845966,123.824894040502)) ;
#83845=CARTESIAN_POINT('Ctrl Pts',(-20.4529119922513,38.3072787321768,124.016061119421)) ;
#83846=CARTESIAN_POINT('Ctrl Pts',(-20.3343454404401,38.3171113551833,124.18538604575)) ;
#83847=CARTESIAN_POINT('Ctrl Pts',(-20.1862012398777,38.3271054262941,124.334369805916)) ;
#83848=CARTESIAN_POINT('Ctrl Pts',(-20.0135915942845,38.3371340839349,124.455455362226)) ;
#83849=CARTESIAN_POINT('Ctrl Pts',(-19.8254446593735,38.3470184101277,124.54364378584)) ;
#83850=CARTESIAN_POINT('Ctrl Pts',(-19.6233091252654,38.3569841536184,124.598773682484)) ;
#83851=CARTESIAN_POINT('Ctrl Pts',(-19.4133488542568,38.3670125327496,124.617784427648)) ;
#83852=CARTESIAN_POINT('Ctrl Pts',(-19.2058864394032,38.3769133789565,124.600587770816)) ;
#83853=CARTESIAN_POINT('Ctrl Pts',(-19.0014247677989,38.3869720363736,124.546746007214)) ;
#83854=CARTESIAN_POINT('Ctrl Pts',(-18.8131022759335,38.3968295991555,124.460160335888)) ;
#83855=CARTESIAN_POINT('Ctrl Pts',(-18.6390069736978,38.4068980017087,124.339821060971)) ;
#83856=CARTESIAN_POINT('Ctrl Pts',(-18.4916162320444,38.4167534004483,124.194179107453)) ;
#83857=CARTESIAN_POINT('Ctrl Pts',(-18.3695561134866,38.4267482675222,124.023151845071)) ;
#83858=CARTESIAN_POINT('Ctrl Pts',(-18.2791222095453,38.4367795625056,123.832631966761)) ;
#83859=CARTESIAN_POINT('Ctrl Pts',(-18.2237417212463,38.4466460872322,123.632728866384)) ;
#83860=CARTESIAN_POINT('Ctrl Pts',(-18.2033366605409,38.4566335579279,123.423780131102)) ;
#83861=CARTESIAN_POINT('Ctrl Pts',(-18.2193409223718,38.4665783174918,123.215291231871)) ;
#83862=CARTESIAN_POINT('Ctrl Pts',(-18.2719426702172,38.4766238734406,123.010781908858)) ;
#83863=CARTESIAN_POINT('Ctrl Pts',(-18.3574578438676,38.4864834618157,122.821937909227)) ;
#83864=CARTESIAN_POINT('Ctrl Pts',(-18.4758459844247,38.4964844169518,122.648227494575)) ;
#83865=CARTESIAN_POINT('Ctrl Pts',(-18.6211083978513,38.5063886442293,122.499006540837)) ;
#83866=CARTESIAN_POINT('Ctrl Pts',(-18.7923421242233,38.5164307211245,122.375568110277)) ;
#83867=CARTESIAN_POINT('Ctrl Pts',(-18.9798774217074,38.5263383338106,122.284845068347)) ;
#83868=CARTESIAN_POINT('Ctrl Pts',(-19.1832184871999,38.5363928644264,122.227224428102)) ;
#83869=CARTESIAN_POINT('Ctrl Pts',(-19.3894682309684,38.5462536509752,122.206072298328)) ;
#83870=CARTESIAN_POINT('Ctrl Pts',(-19.5990133797797,38.5562474060463,122.220862897589)) ;
#83871=CARTESIAN_POINT('Ctrl Pts',(-19.8015015919299,38.5661727662863,122.271381257439)) ;
#83872=CARTESIAN_POINT('Ctrl Pts',(-19.9940600695036,38.5762006956816,122.357136872003)) ;
#83873=CARTESIAN_POINT('Ctrl Pts',(-20.1665038714254,38.5860869624809,122.473213604027)) ;
#83874=CARTESIAN_POINT('Ctrl Pts',(-20.3184039133706,38.5961187313791,122.619467213453)) ;
#83875=CARTESIAN_POINT('Ctrl Pts',(-20.4409492915006,38.6060003272227,122.787261733951)) ;
#83876=CARTESIAN_POINT('Ctrl Pts',(-20.5341860438392,38.6160622126907,122.977102521833)) ;
#83877=CARTESIAN_POINT('Ctrl Pts',(-20.5919300802782,38.6259196467096,123.176157000518)) ;
#83878=CARTESIAN_POINT('Ctrl Pts',(-20.6149768427881,38.6359128897515,123.384951999739)) ;
#83879=CARTESIAN_POINT('Ctrl Pts',(-20.6015180584844,38.6458436506379,123.593303638436)) ;
#83880=CARTESIAN_POINT('Ctrl Pts',(-20.5353364781107,38.6591926428351,123.866067846683)) ;
#83881=CARTESIAN_POINT('Ctrl Pts',(-20.3999665698266,38.6724610156515,124.113595090077)) ;
#83882=CARTESIAN_POINT('Ctrl Pts',(-20.2075244528949,38.6857439570358,124.315918873025)) ;
#83883=CARTESIAN_POINT('Ctrl Pts',(-20.0375784179767,38.6957867428781,124.441187515618)) ;
#83884=CARTESIAN_POINT('Ctrl Pts',(-19.8521844358346,38.7056366854302,124.53344877468)) ;
#83885=CARTESIAN_POINT('Ctrl Pts',(-19.6507787501863,38.7156339183491,124.593496881762)) ;
#83886=CARTESIAN_POINT('Ctrl Pts',(-19.4415865793863,38.7256488136837,124.617384098665)) ;
#83887=CARTESIAN_POINT('Ctrl Pts',(-19.1637205474223,38.7388884903219,124.600727732205)) ;
#83888=CARTESIAN_POINT('Ctrl Pts',(-18.8297226674719,38.7554357147272,124.490328749291)) ;
#83889=CARTESIAN_POINT('Ctrl Pts',(-18.5515626228593,38.7720831518583,124.271315968218)) ;
#83890=CARTESIAN_POINT('Ctrl Pts',(-18.3844931738527,38.7853726493365,124.047426592264)) ;
#83891=CARTESIAN_POINT('Ctrl Pts',(-18.2905580424256,38.7952460571589,123.862315169489)) ;
#83892=CARTESIAN_POINT('Ctrl Pts',(-18.2290723693852,38.8052984347516,123.660137301504)) ;
#83893=CARTESIAN_POINT('Ctrl Pts',(-18.2040857533093,38.8152020882925,123.453418521977)) ;
#83894=CARTESIAN_POINT('Ctrl Pts',(-18.2149101918065,38.8251463572878,123.244669041056)) ;
#83895=CARTESIAN_POINT('Ctrl Pts',(-18.2776890698287,38.8384773656205,122.971450399707)) ;
#83896=CARTESIAN_POINT('Ctrl Pts',(-18.4435331913446,38.8550989461448,122.659461152855)) ;
#83897=CARTESIAN_POINT('Ctrl Pts',(-18.7042960227545,38.8716416168431,122.423288632422)) ;
#83898=CARTESIAN_POINT('Ctrl Pts',(-18.9539076969586,38.8849907764061,122.295137393368)) ;
#83899=CARTESIAN_POINT('Ctrl Pts',(-19.2195502286589,38.8982189265656,122.21266634664)) ;
#83900=CARTESIAN_POINT('Ctrl Pts',(-19.5728078616279,38.9148496037031,122.198403767171)) ;
#83901=CARTESIAN_POINT('Ctrl Pts',(-19.9761466167671,38.9347525429912,122.326687068324)) ;
#83902=CARTESIAN_POINT('Ctrl Pts',(-20.3116532401564,38.9546554095944,122.584476648909)) ;
#83903=CARTESIAN_POINT('Ctrl Pts',(-20.5398098713944,38.9745685746993,122.941266374104)) ;
#83904=CARTESIAN_POINT('Ctrl Pts',(-20.6324050392952,38.9946044038406,123.357036057847)) ;
#83905=CARTESIAN_POINT('Ctrl Pts',(-20.5783888068868,39.0144229787187,123.775059915529)) ;
#83906=CARTESIAN_POINT('Ctrl Pts',(-20.3841956945606,39.0343932797607,124.152516109212)) ;
#83907=CARTESIAN_POINT('Ctrl Pts',(-20.0739570774436,39.0542848121252,124.440209333799)) ;
#83908=CARTESIAN_POINT('Ctrl Pts',(-19.6816966830104,39.0743079099418,124.605463079056)) ;
#83909=CARTESIAN_POINT('Ctrl Pts',(-19.2612631464682,39.0941046628617,124.62700383692)) ;
#83910=CARTESIAN_POINT('Ctrl Pts',(-18.8551291542701,39.1140657513505,124.503871232136)) ;
#83911=CARTESIAN_POINT('Ctrl Pts',(-18.5155747700048,39.1340440202826,124.248566128734)) ;
#83912=CARTESIAN_POINT('Ctrl Pts',(-18.2848897271834,39.1538640350736,123.895929288)) ;
#83913=CARTESIAN_POINT('Ctrl Pts',(-18.1867323135785,39.1738024443255,123.48348235109)) ;
#83914=CARTESIAN_POINT('Ctrl Pts',(-18.2364347214362,39.1938495617179,123.06008016948)) ;
#83915=CARTESIAN_POINT('Ctrl Pts',(-18.4258541864355,39.2136958075517,122.683047672444)) ;
#83916=CARTESIAN_POINT('Ctrl Pts',(-18.7315120380653,39.2335447760638,122.391994355)) ;
#83917=CARTESIAN_POINT('Ctrl Pts',(-19.1222232914194,39.2535950783751,122.2215247231)) ;
#83918=CARTESIAN_POINT('Ctrl Pts',(-19.5432352942313,39.2734300008063,122.194986111622)) ;
#83919=CARTESIAN_POINT('Ctrl Pts',(-19.9499550927427,39.2933604020322,122.313413163743)) ;
#83920=CARTESIAN_POINT('Ctrl Pts',(-20.2916490239367,39.313245347391,122.562710718802)) ;
#83921=CARTESIAN_POINT('Ctrl Pts',(-20.5292736425933,39.3333179555424,122.917142170104)) ;
#83922=CARTESIAN_POINT('Ctrl Pts',(-20.6303535167698,39.3531092718706,123.32570516107)) ;
#83923=CARTESIAN_POINT('Ctrl Pts',(-20.5868689588886,39.3730740616378,123.747941864772)) ;
#83924=CARTESIAN_POINT('Ctrl Pts',(-20.4007639600174,39.3930570173881,124.129914819336)) ;
#83925=CARTESIAN_POINT('Ctrl Pts',(-20.0987295327906,39.4128655393642,124.42351592743)) ;
#83926=CARTESIAN_POINT('Ctrl Pts',(-19.7115171487444,39.4328511141001,124.598356581541)) ;
#83927=CARTESIAN_POINT('Ctrl Pts',(-19.2898686561888,39.4527337541685,124.630327663352)) ;
#83928=CARTESIAN_POINT('Ctrl Pts',(-18.8812200067832,39.4726890663004,124.516450733859)) ;
#83929=CARTESIAN_POINT('Ctrl Pts',(-18.5370775098728,39.4925634229082,124.271087917632)) ;
#83930=CARTESIAN_POINT('Ctrl Pts',(-18.2958623876815,39.5125456297692,123.921382096351)) ;
#83931=CARTESIAN_POINT('Ctrl Pts',(-18.1889226838399,39.5324767077192,123.511215629101)) ;
#83932=CARTESIAN_POINT('Ctrl Pts',(-18.2282858913957,39.5524036825742,123.089434397404)) ;
#83933=CARTESIAN_POINT('Ctrl Pts',(-18.4076742807777,39.5722361415231,122.707733435929)) ;
#83934=CARTESIAN_POINT('Ctrl Pts',(-18.6583860005917,39.5888938256983,122.45771230889)) ;
#83935=CARTESIAN_POINT('Ctrl Pts',(-18.899856660283,39.6021430496054,122.318686767975)) ;
#83936=CARTESIAN_POINT('Ctrl Pts',(-19.0984023707433,39.6121920710566,122.246593172769)) ;
#83937=CARTESIAN_POINT('Ctrl Pts',(-19.3025721748883,39.6220520792871,122.210698625699)) ;
#83938=CARTESIAN_POINT('Ctrl Pts',(-19.5818091090242,39.6353355925117,122.209905164428)) ;
#83939=CARTESIAN_POINT('Ctrl Pts',(-19.9238636732146,39.6519815115125,122.300943991679)) ;
#83940=CARTESIAN_POINT('Ctrl Pts',(-20.2129499026306,39.6685354893286,122.501708337776)) ;
#83941=CARTESIAN_POINT('Ctrl Pts',(-20.3943693157841,39.6818952183002,122.716154682349)) ;
#83942=CARTESIAN_POINT('Ctrl Pts',(-20.4992257257281,39.6917882700969,122.895780883899)) ;
#83943=CARTESIAN_POINT('Ctrl Pts',(-20.5722643729361,39.7017782353779,123.092667938302)) ;
#83944=CARTESIAN_POINT('Ctrl Pts',(-20.6099946155583,39.7117301162387,123.298490471332)) ;
#83945=CARTESIAN_POINT('Ctrl Pts',(-20.6112491614818,39.7217784679306,123.5097123281)) ;
#83946=CARTESIAN_POINT('Ctrl Pts',(-20.5767745820442,39.7316197520368,123.713735911497)) ;
#83947=CARTESIAN_POINT('Ctrl Pts',(-20.5068084652051,39.7416064551624,123.911647798122)) ;
#83948=CARTESIAN_POINT('Ctrl Pts',(-20.404149955336,39.7515414839799,124.093590220558)) ;
#83949=CARTESIAN_POINT('Ctrl Pts',(-20.2697572467411,39.7615972788868,124.256736870422)) ;
#83950=CARTESIAN_POINT('Ctrl Pts',(-20.1128745784745,39.771425642176,124.391246879686)) ;
#83951=CARTESIAN_POINT('Ctrl Pts',(-19.9310134309257,39.781486612074,124.499192637866)) ;
#83952=CARTESIAN_POINT('Ctrl Pts',(-19.7359479982454,39.7914008909638,124.572688744676)) ;
#83953=CARTESIAN_POINT('Ctrl Pts',(-19.5292237033137,39.801409885432,124.611969713177)) ;
#83954=CARTESIAN_POINT('Ctrl Pts',(-19.3183814454034,39.8114397199958,124.614334357562)) ;
#83955=CARTESIAN_POINT('Ctrl Pts',(-19.1138104499501,39.821297950068,124.581026337363)) ;
#83956=CARTESIAN_POINT('Ctrl Pts',(-18.9153042209363,39.8312966558104,124.511985709217)) ;
#83957=CARTESIAN_POINT('Ctrl Pts',(-18.7335269819325,39.8411913117292,124.410773872078)) ;
#83958=CARTESIAN_POINT('Ctrl Pts',(-18.5694363601387,39.8512543761131,124.277299024287)) ;
#83959=CARTESIAN_POINT('Ctrl Pts',(-18.4338684191718,39.861094034393,124.121008559524)) ;
#83960=CARTESIAN_POINT('Ctrl Pts',(-18.3248828525009,39.8711572014749,123.939715182308)) ;
#83961=CARTESIAN_POINT('Ctrl Pts',(-18.2504503795783,39.881051446602,123.745455644195)) ;
#83962=CARTESIAN_POINT('Ctrl Pts',(-18.2101397445367,39.8909932682066,123.540397862087)) ;
#83963=CARTESIAN_POINT('Ctrl Pts',(-18.2059424849837,39.9009957991247,123.330126961265)) ;
#83964=CARTESIAN_POINT('Ctrl Pts',(-18.2387400782455,39.9110304255822,123.121743701287)) ;
#83965=CARTESIAN_POINT('Ctrl Pts',(-18.3056247063555,39.9208759605686,122.925856511835)) ;
#83966=CARTESIAN_POINT('Ctrl Pts',(-18.4064938974703,39.9308593854076,122.741821100437)) ;
#83967=CARTESIAN_POINT('Ctrl Pts',(-18.5373982393695,39.9408097757727,122.578645629989)) ;
#83968=CARTESIAN_POINT('Ctrl Pts',(-18.6952153467067,39.9508074160698,122.439801679769)) ;
#83969=CARTESIAN_POINT('Ctrl Pts',(-18.8756822321668,39.960846496633,122.330394247099)) ;
#83970=CARTESIAN_POINT('Ctrl Pts',(-19.0680855968778,39.9706726474021,122.255165125593)) ;
#83971=CARTESIAN_POINT('Ctrl Pts',(-19.2752888310551,39.9807292223312,122.213206637334)) ;
#83972=CARTESIAN_POINT('Ctrl Pts',(-19.4842192729442,39.9906697617115,122.20828893783)) ;
#83973=CARTESIAN_POINT('Ctrl Pts',(-19.6901728378794,40.0005741546879,122.238964162981)) ;
#83974=CARTESIAN_POINT('Ctrl Pts',(-19.8904453981696,40.0106208088928,122.306001788064)) ;
#83975=CARTESIAN_POINT('Ctrl Pts',(-20.0733802135455,40.0205163708312,122.405136531576)) ;
#83976=CARTESIAN_POINT('Ctrl Pts',(-20.2390148331265,40.0305784486768,122.536666604298)) ;
#83977=CARTESIAN_POINT('Ctrl Pts',(-20.3763608552124,40.0404211470905,122.691467800279)) ;
#83978=CARTESIAN_POINT('Ctrl Pts',(-20.4867687239541,40.050411922052,122.870114190149)) ;
#83979=CARTESIAN_POINT('Ctrl Pts',(-20.5639763620447,40.0603397870711,123.064036076896)) ;
#83980=CARTESIAN_POINT('Ctrl Pts',(-20.6069421627515,40.0703285318373,123.269592676975)) ;
#83981=CARTESIAN_POINT('Ctrl Pts',(-20.6132830460432,40.0803613174242,123.480421510486)) ;
#83982=CARTESIAN_POINT('Ctrl Pts',(-20.5836334756742,40.0902280020449,123.685712616004)) ;
#83983=CARTESIAN_POINT('Ctrl Pts',(-20.5187331389451,40.100189894208,123.884836795131)) ;
#83984=CARTESIAN_POINT('Ctrl Pts',(-20.4192475497836,40.1102233711206,124.070827756619)) ;
#83985=CARTESIAN_POINT('Ctrl Pts',(-20.2911532710343,40.1201077123689,124.234483925835)) ;
#83986=CARTESIAN_POINT('Ctrl Pts',(-20.1338366504222,40.13017065449,124.375890206505)) ;
#83987=CARTESIAN_POINT('Ctrl Pts',(-19.9581654257089,40.1400210561096,124.485576275425)) ;
#83988=CARTESIAN_POINT('Ctrl Pts',(-19.7628967023069,40.1500479448992,124.564969159993)) ;
#83989=CARTESIAN_POINT('Ctrl Pts',(-19.5566424479521,40.1600765598555,124.60872174278)) ;
#83990=CARTESIAN_POINT('Ctrl Pts',(-19.3498138019929,40.1699217829755,124.61625506074)) ;
#83991=CARTESIAN_POINT('Ctrl Pts',(-19.1416957832697,40.1799124667815,124.587896764921)) ;
#83992=CARTESIAN_POINT('Ctrl Pts',(-18.9408691373841,40.1899503488539,124.523084939537)) ;
#83993=CARTESIAN_POINT('Ctrl Pts',(-18.7577650040935,40.1997947084927,124.426605483624)) ;
#83994=CARTESIAN_POINT('Ctrl Pts',(-18.5916351108559,40.2097795791075,124.298338376431)) ;
#83995=CARTESIAN_POINT('Ctrl Pts',(-18.4508347705853,40.2197188624361,124.143903010517)) ;
#83996=CARTESIAN_POINT('Ctrl Pts',(-18.3379319966298,40.2297594718093,123.96557517779)) ;
#83997=CARTESIAN_POINT('Ctrl Pts',(-18.2587923174509,40.2396443227225,123.773397813617)) ;
#83998=CARTESIAN_POINT('Ctrl Pts',(-18.213460031334,40.2496462788913,123.568102243328)) ;
#83999=CARTESIAN_POINT('Ctrl Pts',(-18.204367545909,40.2595648756118,123.359747486292)) ;
#84000=CARTESIAN_POINT('Ctrl Pts',(-18.2319750563764,40.2696116976876,123.150373468902)) ;
#84001=CARTESIAN_POINT('Ctrl Pts',(-18.2942593625659,40.2794859788003,122.952312214751)) ;
#84002=CARTESIAN_POINT('Ctrl Pts',(-18.3915852031377,40.2895401788449,122.764722269776)) ;
#84003=CARTESIAN_POINT('Ctrl Pts',(-18.5179539789495,40.2994356084801,122.599419714225)) ;
#84004=CARTESIAN_POINT('Ctrl Pts',(-18.6735953670539,40.3094972367975,122.456211498221)) ;
#84005=CARTESIAN_POINT('Ctrl Pts',(-18.8479090387008,40.3193418656274,122.34462186564)) ;
#84006=CARTESIAN_POINT('Ctrl Pts',(-19.0408896885059,40.329301913233,122.263369317502)) ;
#84007=CARTESIAN_POINT('Ctrl Pts',(-19.246736340465,40.339340219407,122.216899416783)) ;
#84008=CARTESIAN_POINT('Ctrl Pts',(-19.454082103357,40.3492135188397,122.20664050289)) ;
#84009=CARTESIAN_POINT('Ctrl Pts',(-19.6641481133357,40.359286780426,122.233123002106)) ;
#84010=CARTESIAN_POINT('Ctrl Pts',(-19.861509253522,40.3691070063827,122.293870082184)) ;
#84011=CARTESIAN_POINT('Ctrl Pts',(-20.050164432258,40.3791860703222,122.390230258189)) ;
#84012=CARTESIAN_POINT('Ctrl Pts',(-20.2155277669988,40.389036160342,122.514970602576)) ;
#84013=CARTESIAN_POINT('Ctrl Pts',(-20.3600033921578,40.3991149139558,122.669891379684)) ;
#84014=CARTESIAN_POINT('Ctrl Pts',(-20.4726264427281,40.4089363812152,122.843004495884)) ;
#84015=CARTESIAN_POINT('Ctrl Pts',(-20.5557528282333,40.4190019795729,123.037552166323)) ;
#84016=CARTESIAN_POINT('Ctrl Pts',(-20.6030259622588,40.4289046353476,123.24035156858)) ;
#84017=CARTESIAN_POINT('Ctrl Pts',(-20.6145983075349,40.4389554611772,123.451291704677)) ;
#84018=CARTESIAN_POINT('Ctrl Pts',(-20.5900018171462,40.4488296655161,123.657461665772)) ;
#84019=CARTESIAN_POINT('Ctrl Pts',(-20.5288150242809,40.4589021155552,123.860137172536)) ;
#84020=CARTESIAN_POINT('Ctrl Pts',(-20.4358132666408,40.4687311323287,124.044705992598)) ;
#84021=CARTESIAN_POINT('Ctrl Pts',(-20.3094637393586,40.4787979782435,124.214444033496)) ;
#84022=CARTESIAN_POINT('Ctrl Pts',(-20.1581261325448,40.4886881495453,124.357060562804)) ;
#84023=CARTESIAN_POINT('Ctrl Pts',(-19.9828174861627,40.4986803431691,124.472776119996)) ;
#84024=CARTESIAN_POINT('Ctrl Pts',(-19.7905608688836,40.5086431537925,124.555869129345)) ;
#84025=CARTESIAN_POINT('Ctrl Pts',(-19.5880954730282,40.518547426636,124.604552612878)) ;
#84026=CARTESIAN_POINT('Ctrl Pts',(-19.3770061385178,40.5286079184406,124.617357350951)) ;
#84027=CARTESIAN_POINT('Ctrl Pts',(-19.1714136665381,40.5384482501129,124.594104016423)) ;
#84028=CARTESIAN_POINT('Ctrl Pts',(-18.9684724548646,40.5485112962047,124.534440348117)) ;
#84029=CARTESIAN_POINT('Ctrl Pts',(-18.7821897791034,40.5584053518998,124.441849138628)) ;
#84030=CARTESIAN_POINT('Ctrl Pts',(-18.6136871793535,40.5683480522227,124.318199437492)) ;
#84031=CARTESIAN_POINT('Ctrl Pts',(-18.4682360875354,40.5783537931503,124.166208379419)) ;
#84032=CARTESIAN_POINT('Ctrl Pts',(-18.3514206949662,40.5883747036659,123.990896048269)) ;
#84033=CARTESIAN_POINT('Ctrl Pts',(-18.2676944058122,40.5982654391158,123.80055651548)) ;
#84034=CARTESIAN_POINT('Ctrl Pts',(-18.2174871451412,40.6082569798447,123.596600026153)) ;
#84035=CARTESIAN_POINT('Ctrl Pts',(-18.2035765211451,40.6182048402663,123.387929661451)) ;
#84036=CARTESIAN_POINT('Ctrl Pts',(-18.2256975259737,40.6281515094527,123.179981133137)) ;
#84037=CARTESIAN_POINT('Ctrl Pts',(-18.2843962838863,40.6381995855883,122.977065937708)) ;
#84038=CARTESIAN_POINT('Ctrl Pts',(-18.3754280473038,40.6480471835939,122.791125024287)) ;
#84039=CARTESIAN_POINT('Ctrl Pts',(-18.4982372741933,40.6580089066784,122.621498389461)) ;
#84040=CARTESIAN_POINT('Ctrl Pts',(-18.6498469120804,40.6680375417614,122.474969319783)) ;
#84041=CARTESIAN_POINT('Ctrl Pts',(-18.8224769707275,40.6779478500794,122.358338766406)) ;
#84042=CARTESIAN_POINT('Ctrl Pts',(-19.0129988131327,40.6878827472153,122.272737599559)) ;
#84043=CARTESIAN_POINT('Ctrl Pts',(-19.2176901817854,40.6979238301579,122.221162632871)) ;
#84044=CARTESIAN_POINT('Ctrl Pts',(-19.4250098113896,40.7078111729861,122.206002229052)) ;
#84045=CARTESIAN_POINT('Ctrl Pts',(-19.6340061907446,40.7178026879254,122.226929971137)) ;
#84046=CARTESIAN_POINT('Ctrl Pts',(-19.835373853098,40.7277540791219,122.283688979789)) ;
#84047=CARTESIAN_POINT('Ctrl Pts',(-20.0236219719852,40.7376866124545,122.374049360346)) ;
#84048=CARTESIAN_POINT('Ctrl Pts',(-20.1944682418108,40.747683770354,122.496443508176)) ;
#84049=CARTESIAN_POINT('Ctrl Pts',(-20.3413742173031,40.7576687805175,122.646434347578)) ;
#84050=CARTESIAN_POINT('Ctrl Pts',(-20.4604016388904,40.7677116070873,122.82078190189)) ;
#84051=CARTESIAN_POINT('Ctrl Pts',(-20.545965381587,40.7775418413922,123.008934982547)) ;
#84052=CARTESIAN_POINT('Ctrl Pts',(-20.5989226624239,40.7876178666269,123.213993657036)) ;
#84053=CARTESIAN_POINT('Ctrl Pts',(-20.6152177266927,40.7974701031178,123.420521265477)) ;
#84054=CARTESIAN_POINT('Ctrl Pts',(-20.595146371147,40.8075433095519,123.631304261666)) ;
#84055=CARTESIAN_POINT('Ctrl Pts',(-20.5400095589462,40.8173848190591,123.830735669813)) ;
#84056=CARTESIAN_POINT('Ctrl Pts',(-20.4507245478584,40.8273457658389,124.020150570781)) ;
#84057=CARTESIAN_POINT('Ctrl Pts',(-20.3286295016058,40.8373835946389,124.192262277119)) ;
#84058=CARTESIAN_POINT('Ctrl Pts',(-20.1811994395748,40.8472579043934,124.338439950334)) ;
#84059=CARTESIAN_POINT('Ctrl Pts',(-20.0072892729552,40.8573276020665,124.459100741627)) ;
#84060=CARTESIAN_POINT('Ctrl Pts',(-19.8195861561062,40.8671610733539,124.545769392456)) ;
#84061=CARTESIAN_POINT('Ctrl Pts',(-19.615872314466,40.8771907198839,124.600164946026)) ;
#84062=CARTESIAN_POINT('Ctrl Pts',(-19.4056431537582,40.8872252342113,124.617731140901)) ;
#84063=CARTESIAN_POINT('Ctrl Pts',(-19.1998966584607,40.8970505196821,124.599424022294)) ;
#84064=CARTESIAN_POINT('Ctrl Pts',(-18.9967300700441,40.9070547612307,124.545129020329)) ;
#84065=CARTESIAN_POINT('Ctrl Pts',(-18.8064674138369,40.9170374063098,124.456466503023)) ;
#84066=CARTESIAN_POINT('Ctrl Pts',(-18.6336010926336,40.9270826034013,124.335200573966)) ;
#84067=CARTESIAN_POINT('Ctrl Pts',(-18.4874473673318,40.9369057191614,124.189290879588)) ;
#84068=CARTESIAN_POINT('Ctrl Pts',(-18.3658653930389,40.9469403309617,124.016894765703)) ;
#84069=CARTESIAN_POINT('Ctrl Pts',(-18.2766790054836,40.9569653397348,123.825931009398)) ;
#84070=CARTESIAN_POINT('Ctrl Pts',(-18.2225124709899,40.9668172645764,123.626017271798)) ;
#84071=CARTESIAN_POINT('Ctrl Pts',(-18.203299075712,40.9768082028991,123.416882417543)) ;
#84072=CARTESIAN_POINT('Ctrl Pts',(-18.220432722887,40.9867261880456,123.209055352599)) ;
#84073=CARTESIAN_POINT('Ctrl Pts',(-18.2739197568231,40.9967542889411,123.005147713301)) ;
#84074=CARTESIAN_POINT('Ctrl Pts',(-18.3606743272535,41.0066395298837,122.816298472625)) ;
#84075=CARTESIAN_POINT('Ctrl Pts',(-18.4797205533408,41.0166286428503,122.643290607372)) ;
#84076=CARTESIAN_POINT('Ctrl Pts',(-18.6281007078246,41.0266707071911,122.493120515096)) ;
#84077=CARTESIAN_POINT('Ctrl Pts',(-18.7964346106993,41.0364999085956,122.373256813908)) ;
#84078=CARTESIAN_POINT('Ctrl Pts',(-18.9861689447885,41.0465067493538,122.282435666155)) ;
#84079=CARTESIAN_POINT('Ctrl Pts',(-19.1884902487412,41.0564942735457,122.226152190945)) ;
#84080=CARTESIAN_POINT('Ctrl Pts',(-19.3983530804929,41.0665239193543,122.205918577425)) ;
#84081=CARTESIAN_POINT('Ctrl Pts',(-19.605339265154,41.076397950093,122.221929297578)) ;
#84082=CARTESIAN_POINT('Ctrl Pts',(-19.8089638120336,41.0863972729571,122.274027018011)) ;
#84083=CARTESIAN_POINT('Ctrl Pts',(-19.9989028196144,41.0963081085327,122.359763952569)) ;
#84084=CARTESIAN_POINT('Ctrl Pts',(-20.1734602703495,41.1063623565068,122.478901029742)) ;
#84085=CARTESIAN_POINT('Ctrl Pts',(-20.3219594050165,41.1162211007695,122.62353974216)) ;
#84086=CARTESIAN_POINT('Ctrl Pts',(-20.4457241103997,41.1262891868425,122.795209530907)) ;
#84087=CARTESIAN_POINT('Ctrl Pts',(-20.535863063905,41.136144670022,122.981787012691)) ;
#84088=CARTESIAN_POINT('Ctrl Pts',(-20.5936332050625,41.1461395158162,123.183805523602)) ;
#84089=CARTESIAN_POINT('Ctrl Pts',(-20.6150774326418,41.1561708114787,123.393606067351)) ;
#84090=CARTESIAN_POINT('Ctrl Pts',(-20.6003488779222,41.1660373547686,123.600515251708)) ;
#84091=CARTESIAN_POINT('Ctrl Pts',(-20.5496364134409,41.176024750532,123.804239891869)) ;
#84092=CARTESIAN_POINT('Ctrl Pts',(-20.4647624232787,41.185969791262,123.995347573894)) ;
#84093=CARTESIAN_POINT('Ctrl Pts',(-20.3467582709289,41.1960142974787,124.170441035072)) ;
#84094=CARTESIAN_POINT('Ctrl Pts',(-20.2028932956802,41.205877803616,124.319807442047)) ;
#84095=CARTESIAN_POINT('Ctrl Pts',(-20.0333415512162,41.2158706644521,124.443797445221)) ;
#84096=CARTESIAN_POINT('Ctrl Pts',(-19.8460833020742,41.225796858171,124.535960566689)) ;
#84097=CARTESIAN_POINT('Ctrl Pts',(-19.6438582487859,41.2358157842036,124.594776911831)) ;
#84098=CARTESIAN_POINT('Ctrl Pts',(-19.4366299850422,41.2457307835712,124.617551938462)) ;
#84099=CARTESIAN_POINT('Ctrl Pts',(-19.2257234112187,41.2557855551285,124.603768112369)) ;
#84100=CARTESIAN_POINT('Ctrl Pts',(-19.0243302973375,41.265644517426,124.55466833159)) ;
#84101=CARTESIAN_POINT('Ctrl Pts',(-18.8318135036879,41.2756387612639,124.470587736357)) ;
#84102=CARTESIAN_POINT('Ctrl Pts',(-18.6579190557029,41.2855639906881,124.35520482749)) ;
#84103=CARTESIAN_POINT('Ctrl Pts',(-18.5051729929965,41.2955919545796,124.209940587375)) ;
#84104=CARTESIAN_POINT('Ctrl Pts',(-18.3815316967757,41.30547821421,124.042837487095)) ;
#84105=CARTESIAN_POINT('Ctrl Pts',(-18.2873498166845,41.3155099772878,123.854175099983)) ;
#84106=CARTESIAN_POINT('Ctrl Pts',(-18.2280402925463,41.3253916035819,123.655039695236)) ;
#84107=CARTESIAN_POINT('Ctrl Pts',(-18.2037261419787,41.3354533730681,123.444942864468)) ;
#84108=CARTESIAN_POINT('Ctrl Pts',(-18.2159492400391,41.3453112405636,123.238034912573)) ;
#84109=CARTESIAN_POINT('Ctrl Pts',(-18.2640991524596,41.3553028656809,123.033597999841)) ;
#84110=CARTESIAN_POINT('Ctrl Pts',(-18.3466098748585,41.3652396647892,122.841666401691)) ;
#84111=CARTESIAN_POINT('Ctrl Pts',(-18.4615560357131,41.3752304943465,122.665869308741)) ;
#84112=CARTESIAN_POINT('Ctrl Pts',(-18.6059270402561,41.3852537300597,122.512369557892)) ;
#84113=CARTESIAN_POINT('Ctrl Pts',(-18.7725080465758,41.3951500780889,122.387730247027)) ;
#84114=CARTESIAN_POINT('Ctrl Pts',(-18.9597602693054,41.4051396405914,122.292617765238)) ;
#84115=CARTESIAN_POINT('Ctrl Pts',(-19.1618068495338,41.4151799482759,122.231566049931)) ;
#84116=CARTESIAN_POINT('Ctrl Pts',(-19.3672327140925,41.4250222516231,122.206620712325)) ;
#84117=CARTESIAN_POINT('Ctrl Pts',(-19.5776398977284,41.4350459599022,122.21764350523)) ;
#84118=CARTESIAN_POINT('Ctrl Pts',(-19.8485692369757,41.4482681373699,122.280066833461)) ;
#84119=CARTESIAN_POINT('Ctrl Pts',(-20.0983813608666,41.4615607224292,122.412161972798)) ;
#84120=CARTESIAN_POINT('Ctrl Pts',(-20.303073356928,41.4748455783508,122.602192135613)) ;
#84121=CARTESIAN_POINT('Ctrl Pts',(-20.4297314686523,41.4848178055236,122.769227486127)) ;
#84122=CARTESIAN_POINT('Ctrl Pts',(-20.5251912543411,41.4947264219626,122.954404447147)) ;
#84123=CARTESIAN_POINT('Ctrl Pts',(-20.5878572647725,41.5047796273463,123.156230096444)) ;
#84124=CARTESIAN_POINT('Ctrl Pts',(-20.6141674277665,41.5146447611066,123.361965495425)) ;
#84125=CARTESIAN_POINT('Ctrl Pts',(-20.6014118208167,41.5279838187329,123.642111014814)) ;
#84126=CARTESIAN_POINT('Ctrl Pts',(-20.494885952926,41.544553006066,123.977938704161)) ;
#84127=CARTESIAN_POINT('Ctrl Pts',(-20.2793745820825,41.5611981459171,124.258685789852)) ;
#84128=CARTESIAN_POINT('Ctrl Pts',(-20.0579576947335,41.5744704483905,124.428476506012)) ;
#84129=CARTESIAN_POINT('Ctrl Pts',(-19.8719402894778,41.5844514118381,124.52554227184)) ;
#84130=CARTESIAN_POINT('Ctrl Pts',(-19.6726896538698,41.5943932439074,124.588712900572)) ;
#84131=CARTESIAN_POINT('Ctrl Pts',(-19.39515947758,41.6077128131228,124.625810170929)) ;
#84132=CARTESIAN_POINT('Ctrl Pts',(-19.0464439657701,41.6242429680556,124.581269960781)) ;
#84133=CARTESIAN_POINT('Ctrl Pts',(-18.6680926078095,41.6442646935477,124.386344269769)) ;
#84134=CARTESIAN_POINT('Ctrl Pts',(-18.3816919436633,41.6640760901545,124.077301459505)) ;
#84135=CARTESIAN_POINT('Ctrl Pts',(-18.2159314047826,41.6840613388633,123.686131291422)) ;
#84136=CARTESIAN_POINT('Ctrl Pts',(-18.1939891745708,41.7039554014993,123.263631019772)) ;
#84137=CARTESIAN_POINT('Ctrl Pts',(-18.3171493950975,41.7238870806729,122.858127957561)) ;
#84138=CARTESIAN_POINT('Ctrl Pts',(-18.5719340628339,41.7438511351449,122.51860266307)) ;
#84139=CARTESIAN_POINT('Ctrl Pts',(-18.9256476276961,41.7637320369078,122.287092846652)) ;
#84140=CARTESIAN_POINT('Ctrl Pts',(-19.3381948683728,41.7836706985162,122.189526548591)) ;
#84141=CARTESIAN_POINT('Ctrl Pts',(-19.7584053445719,41.8035672237715,122.238430566627)) ;
#84142=CARTESIAN_POINT('Ctrl Pts',(-20.1370057693331,41.8234622622258,122.427169239193)) ;
#84143=CARTESIAN_POINT('Ctrl Pts',(-20.4294053281451,41.8434260855319,122.734843250388)) ;
#84144=CARTESIAN_POINT('Ctrl Pts',(-20.5988096520374,41.8633002096609,123.122013415926)) ;
#84145=CARTESIAN_POINT('Ctrl Pts',(-20.6264542889846,41.8832752853882,123.545855735373)) ;
#84146=CARTESIAN_POINT('Ctrl Pts',(-20.5073566083067,41.9032288547448,123.953056646348)) ;
#84147=CARTESIAN_POINT('Ctrl Pts',(-20.2585450342421,41.9230667649326,124.29366905313)) ;
#84148=CARTESIAN_POINT('Ctrl Pts',(-19.9062556139249,41.9430425935036,124.530937461275)) ;
#84149=CARTESIAN_POINT('Ctrl Pts',(-19.4952528460471,41.9629606382138,124.632990013257)) ;
#84150=CARTESIAN_POINT('Ctrl Pts',(-19.0748806212009,41.9828308840015,124.589826715437)) ;
#84151=CARTESIAN_POINT('Ctrl Pts',(-18.6915025085209,42.0028798871011,124.403663986878)) ;
#84152=CARTESIAN_POINT('Ctrl Pts',(-18.3981608610353,42.0226591283419,124.102123408947)) ;
#84153=CARTESIAN_POINT('Ctrl Pts',(-18.2226406675483,42.0426891920508,123.714185684315)) ;
#84154=CARTESIAN_POINT('Ctrl Pts',(-18.1909502299276,42.0625714769527,123.292557552484)) ;
#84155=CARTESIAN_POINT('Ctrl Pts',(-18.3038833814422,42.0824537778457,122.885208178774)) ;
#84156=CARTESIAN_POINT('Ctrl Pts',(-18.5504266417596,42.1024368874641,122.539145783805)) ;
#84157=CARTESIAN_POINT('Ctrl Pts',(-18.8986862807476,42.122327282842,122.299139021908)) ;
#84158=CARTESIAN_POINT('Ctrl Pts',(-19.3078323184584,42.1422240728762,122.191754248238)) ;
#84159=CARTESIAN_POINT('Ctrl Pts',(-19.7296141903488,42.1621411268179,122.230019843799)) ;
#84160=CARTESIAN_POINT('Ctrl Pts',(-20.1146546190343,42.1821446750214,122.410843614084)) ;
#84161=CARTESIAN_POINT('Ctrl Pts',(-20.4133983649852,42.202082968674,122.711612553304)) ;
#84162=CARTESIAN_POINT('Ctrl Pts',(-20.5914741681142,42.2219044561069,123.093609268308)) ;
#84163=CARTESIAN_POINT('Ctrl Pts',(-20.6292246758247,42.2418828490978,123.516673289908)) ;
#84164=CARTESIAN_POINT('Ctrl Pts',(-20.5204944696321,42.2617812307115,123.925630779362)) ;
#84165=CARTESIAN_POINT('Ctrl Pts',(-20.3195273000853,42.2783641614414,124.215224407757)) ;
#84166=CARTESIAN_POINT('Ctrl Pts',(-20.106668699646,42.2916383970302,124.395804380293)) ;
#84167=CARTESIAN_POINT('Ctrl Pts',(-19.9243029543144,42.3016848144864,124.502286299798)) ;
#84168=CARTESIAN_POINT('Ctrl Pts',(-19.7302093566461,42.3115300397057,124.574250347447)) ;
#84169=CARTESIAN_POINT('Ctrl Pts',(-19.454606237044,42.3248650107451,124.625183227152)) ;
#84170=CARTESIAN_POINT('Ctrl Pts',(-19.1029744052115,42.3414478675377,124.597295491216)) ;
#84171=CARTESIAN_POINT('Ctrl Pts',(-18.7810077769034,42.3580908698871,124.450748766499)) ;
#84172=CARTESIAN_POINT('Ctrl Pts',(-18.5658476550181,42.3713346009188,124.273892948555)) ;
#84173=CARTESIAN_POINT('Ctrl Pts',(-18.4283770364785,42.3813889955934,124.113388633526)) ;
#84174=CARTESIAN_POINT('Ctrl Pts',(-18.3228682596185,42.3912300569819,123.935378247258)) ;
#84175=CARTESIAN_POINT('Ctrl Pts',(-18.2480350846399,42.4012962813384,123.737465749298)) ;
#84176=CARTESIAN_POINT('Ctrl Pts',(-18.2094758316958,42.4111768942581,123.53331998125)) ;
#84177=CARTESIAN_POINT('Ctrl Pts',(-18.2065221797275,42.4211701874177,123.323284136936)) ;
#84178=CARTESIAN_POINT('Ctrl Pts',(-18.2398729765059,42.4311211956413,123.116720768107)) ;
#84179=CARTESIAN_POINT('Ctrl Pts',(-18.3093895953043,42.4411697100033,122.917259886208)) ;
#84180=CARTESIAN_POINT('Ctrl Pts',(-18.4101750501696,42.451011216066,122.736545002513)) ;
#84181=CARTESIAN_POINT('Ctrl Pts',(-18.5423307476065,42.4609968686957,122.573475467159)) ;
#84182=CARTESIAN_POINT('Ctrl Pts',(-18.7000496641721,42.4709358775406,122.436369799845)) ;
#84183=CARTESIAN_POINT('Ctrl Pts',(-18.8809998215444,42.4809768028336,122.327702252941)) ;
#84184=CARTESIAN_POINT('Ctrl Pts',(-19.075104637649,42.4908671245885,122.253109681038)) ;
#84185=CARTESIAN_POINT('Ctrl Pts',(-19.2812985955346,42.5008630979219,122.212630849789)) ;
#84186=CARTESIAN_POINT('Ctrl Pts',(-19.4900575848041,42.510794497504,122.208578593669)) ;
#84187=CARTESIAN_POINT('Ctrl Pts',(-19.6979366117902,42.520800037981,122.24078115684)) ;
#84188=CARTESIAN_POINT('Ctrl Pts',(-19.8974710231854,42.5308330219123,122.309135094637)) ;
#84189=CARTESIAN_POINT('Ctrl Pts',(-20.0790398642152,42.5406886527391,122.408984399467)) ;
#84190=CARTESIAN_POINT('Ctrl Pts',(-20.2429987573532,42.5506880549323,122.540492343443)) ;
#84191=CARTESIAN_POINT('Ctrl Pts',(-20.3804073367586,42.5605825242934,122.696711264063)) ;
#84192=CARTESIAN_POINT('Ctrl Pts',(-20.4903548510497,42.5706456384576,122.877413023356)) ;
#84193=CARTESIAN_POINT('Ctrl Pts',(-20.5657866640294,42.580485284174,123.070066475262)) ;
#84194=CARTESIAN_POINT('Ctrl Pts',(-20.6078006789638,42.5905484517297,123.277382573781)) ;
#84195=CARTESIAN_POINT('Ctrl Pts',(-20.6129143402783,42.6004427075246,123.48535102237)) ;
#84196=CARTESIAN_POINT('Ctrl Pts',(-20.5822609083431,42.6103844859843,123.692072366378)) ;
#84197=CARTESIAN_POINT('Ctrl Pts',(-20.5158291283224,42.6203871788145,123.891620696624)) ;
#84198=CARTESIAN_POINT('Ctrl Pts',(-20.4151804975653,42.6304212007683,124.076996124411)) ;
#84199=CARTESIAN_POINT('Ctrl Pts',(-20.2865490933976,42.6402689918573,124.239226619396)) ;
#84200=CARTESIAN_POINT('Ctrl Pts',(-20.1299261467673,42.6502505164063,124.378854112824)) ;
#84201=CARTESIAN_POINT('Ctrl Pts',(-19.9519781253064,42.6601997398973,124.488795047195)) ;
#84202=CARTESIAN_POINT('Ctrl Pts',(-19.7567858477738,42.6701973961138,124.566794955655)) ;
#84203=CARTESIAN_POINT('Ctrl Pts',(-19.5500874626473,42.6802376091689,124.609497549118)) ;
#84204=CARTESIAN_POINT('Ctrl Pts',(-19.3435610750483,42.6900656564452,124.615984151148)) ;
#84205=CARTESIAN_POINT('Ctrl Pts',(-19.1343128423954,42.7001200034775,124.586163345661)) ;
#84206=CARTESIAN_POINT('Ctrl Pts',(-18.9357761785149,42.7100611398061,124.520862042553)) ;
#84207=CARTESIAN_POINT('Ctrl Pts',(-18.7519747196911,42.7199653728858,124.423017051191)) ;
#84208=CARTESIAN_POINT('Ctrl Pts',(-18.5856939200554,42.7300120697294,124.29280902179)) ;
#84209=CARTESIAN_POINT('Ctrl Pts',(-18.4464957947498,42.7399076210097,124.138158890315)) ;
#84210=CARTESIAN_POINT('Ctrl Pts',(-18.3344432793517,42.7499696988492,123.958773213698)) ;
#84211=CARTESIAN_POINT('Ctrl Pts',(-18.2568373001376,42.7598124079452,123.766927664689)) ;
#84212=CARTESIAN_POINT('Ctrl Pts',(-18.2125966963191,42.7698031401837,123.561630546517)) ;
#84213=CARTESIAN_POINT('Ctrl Pts',(-18.2047563020714,42.7797311654124,123.35304849605)) ;
#84214=CARTESIAN_POINT('Ctrl Pts',(-18.2330695491077,42.789719312063,123.144978918657)) ;
#84215=CARTESIAN_POINT('Ctrl Pts',(-18.2976873840925,42.799754329903,122.944147828888)) ;
#84216=CARTESIAN_POINT('Ctrl Pts',(-18.3943257759869,42.8096191270081,122.760659901221)) ;
#84217=CARTESIAN_POINT('Ctrl Pts',(-18.5221133593397,42.8195798593643,122.594758697312)) ;
#84218=CARTESIAN_POINT('Ctrl Pts',(-18.6781228108456,42.8296133217613,122.452804639824)) ;
#84219=CARTESIAN_POINT('Ctrl Pts',(-18.8536233433113,42.8394988559727,122.341445375326)) ;
#84220=CARTESIAN_POINT('Ctrl Pts',(-19.0492358229451,42.8495636966527,122.26084028791)) ;
#84221=CARTESIAN_POINT('Ctrl Pts',(-19.2514442585677,42.8594118283815,122.216302493889)) ;
#84222=CARTESIAN_POINT('Ctrl Pts',(-19.4620358055281,42.8694393253717,122.206847322742)) ;
#84223=CARTESIAN_POINT('Ctrl Pts',(-19.6710341574969,42.8794677774167,122.234659846651)) ;
#84224=CARTESIAN_POINT('Ctrl Pts',(-19.8684540618217,42.8893130439808,122.296792882877)) ;
#84225=CARTESIAN_POINT('Ctrl Pts',(-20.0550738088005,42.8993037169218,122.393179126527)) ;
#84226=CARTESIAN_POINT('Ctrl Pts',(-20.2226209396394,42.9093415990102,122.521475164468)) ;
#84227=CARTESIAN_POINT('Ctrl Pts',(-20.3628676291703,42.9191859694499,122.673680087124)) ;
#84228=CARTESIAN_POINT('Ctrl Pts',(-20.4764790858517,42.9291707968453,122.850155959111)) ;
#84229=CARTESIAN_POINT('Ctrl Pts',(-20.5574622870053,42.9391102422506,123.042816232772)) ;
#84230=CARTESIAN_POINT('Ctrl Pts',(-20.6041616186596,42.9491502465365,123.248636423166)) ;
#84231=CARTESIAN_POINT('Ctrl Pts',(-20.6144023760936,42.9590373557221,123.456265606785)) ;
#84232=CARTESIAN_POINT('Ctrl Pts',(-20.5884050697669,42.9690374156246,123.664852246182)) ;
#84233=CARTESIAN_POINT('Ctrl Pts',(-20.5272465507079,42.9789548315393,123.864211860364)) ;
#84234=CARTESIAN_POINT('Ctrl Pts',(-20.4311397225098,42.9890016462801,124.052262571585)) ;
#84235=CARTESIAN_POINT('Ctrl Pts',(-20.3061446771948,42.9988771234767,124.218074771365)) ;
#84236=CARTESIAN_POINT('Ctrl Pts',(-20.1516108795258,43.008933219198,124.362292449822)) ;
#84237=CARTESIAN_POINT('Ctrl Pts',(-19.9772349402535,43.018826381213,124.475727085091)) ;
#84238=CARTESIAN_POINT('Ctrl Pts',(-19.7826262183255,43.0288886172357,124.558584692657)) ;
#84239=CARTESIAN_POINT('Ctrl Pts',(-19.5810180214014,43.0387330828646,124.605386435808)) ;
#84240=CARTESIAN_POINT('Ctrl Pts',(-19.3719712696387,43.0486931755687,124.617355627248)) ;
#84241=CARTESIAN_POINT('Ctrl Pts',(-19.162444446929,43.0587314645498,124.592241353779)) ;
#84242=CARTESIAN_POINT('Ctrl Pts',(-18.9636256595679,43.068604787656,124.53250285335)) ;
#84243=CARTESIAN_POINT('Ctrl Pts',(-18.774542404624,43.0786779717411,124.437233832824)) ;
#84244=CARTESIAN_POINT('Ctrl Pts',(-18.6088995227669,43.088498484029,124.313922050298)) ;
#84245=CARTESIAN_POINT('Ctrl Pts',(-18.4633850579159,43.0985764801448,124.159993820606)) ;
#84246=CARTESIAN_POINT('Ctrl Pts',(-18.3493042591805,43.1084305551281,123.987014257358)) ;
#84247=CARTESIAN_POINT('Ctrl Pts',(-18.2650619365002,43.1184944367118,123.792978328618)) ;
#84248=CARTESIAN_POINT('Ctrl Pts',(-18.2166935633452,43.1283778626855,123.590869297813)) ;
#84249=CARTESIAN_POINT('Ctrl Pts',(-18.2036737600321,43.1383784666066,123.381065490452)) ;
#84250=CARTESIAN_POINT('Ctrl Pts',(-18.226966748946,43.1482982509444,123.173787194636)) ;
#84251=CARTESIAN_POINT('Ctrl Pts',(-18.286681255959,43.1583456013013,122.97121296391)) ;
#84252=CARTESIAN_POINT('Ctrl Pts',(-18.3788852089591,43.1682229435356,122.785107675015)) ;
#84253=CARTESIAN_POINT('Ctrl Pts',(-18.5043642202227,43.1782928246102,122.614654111536)) ;
#84254=CARTESIAN_POINT('Ctrl Pts',(-18.6537874671552,43.1881225298119,122.471849925775)) ;
#84255=CARTESIAN_POINT('Ctrl Pts',(-18.8296636074183,43.1981891909783,122.354200223767)) ;
#84256=CARTESIAN_POINT('Ctrl Pts',(-19.0200097582387,43.2080794128456,122.270467347616)) ;
#84257=CARTESIAN_POINT('Ctrl Pts',(-19.2239389860699,43.2180715889558,122.220108587182)) ;
#84258=CARTESIAN_POINT('Ctrl Pts',(-19.4329190392225,43.2280344190684,122.206163569416)) ;
#84259=CARTESIAN_POINT('Ctrl Pts',(-19.6400002172605,43.2379386314687,122.228059005943)) ;
#84260=CARTESIAN_POINT('Ctrl Pts',(-19.8432008782305,43.2479993455566,122.286655349108)) ;
#84261=CARTESIAN_POINT('Ctrl Pts',(-20.0291416113698,43.2578388485394,122.377370325286)) ;
#84262=CARTESIAN_POINT('Ctrl Pts',(-20.2004350392593,43.2679049871058,122.501580201474)) ;
#84263=CARTESIAN_POINT('Ctrl Pts',(-20.3448645376767,43.2777875015918,122.65097173677)) ;
#84264=CARTESIAN_POINT('Ctrl Pts',(-20.4627595418713,43.2877798009473,122.824800722048)) ;
#84265=CARTESIAN_POINT('Ctrl Pts',(-20.5484179727521,43.2977328679007,123.015743378607)) ;
#84266=CARTESIAN_POINT('Ctrl Pts',(-20.5999443496352,43.307767576106,123.220298980291)) ;
#84267=CARTESIAN_POINT('Ctrl Pts',(-20.6151020046759,43.3176557970101,123.427639351467)) ;
#84268=CARTESIAN_POINT('Ctrl Pts',(-20.5941477370278,43.3276502200406,123.636694552893)) ;
#84269=CARTESIAN_POINT('Ctrl Pts',(-20.5374094838607,43.3375955594868,123.837931569304)) ;
#84270=CARTESIAN_POINT('Ctrl Pts',(-20.4469569802207,43.3475429040981,124.02649364133)) ;
#84271=CARTESIAN_POINT('Ctrl Pts',(-20.3237223272501,43.3575907995091,124.198051257851)) ;
#84272=CARTESIAN_POINT('Ctrl Pts',(-20.1757015005492,43.3674384449884,124.342795665365)) ;
#84273=CARTESIAN_POINT('Ctrl Pts',(-20.0031972366942,43.3774001589024,124.46152863281)) ;
#84274=CARTESIAN_POINT('Ctrl Pts',(-19.8112856932042,43.3874287831934,124.548856656598)) ;
#84275=CARTESIAN_POINT('Ctrl Pts',(-19.6095733525184,43.3973391438501,124.600973582111)) ;
#84276=CARTESIAN_POINT('Ctrl Pts',(-19.4013914577083,43.4072738424234,124.617866015945)) ;
#84277=CARTESIAN_POINT('Ctrl Pts',(-19.1912336801749,43.4173156672776,124.597937770818)) ;
#84278=CARTESIAN_POINT('Ctrl Pts',(-18.9908383852225,43.427200241022,124.542869334189)) ;
#84279=CARTESIAN_POINT('Ctrl Pts',(-18.8007562631651,43.4372020903851,124.453033623645)) ;
#84280=CARTESIAN_POINT('Ctrl Pts',(-18.6304420125934,43.4471213919592,124.332653745502)) ;
#84281=CARTESIAN_POINT('Ctrl Pts',(-18.4817975922359,43.4571655003045,124.182701661743)) ;
#84282=CARTESIAN_POINT('Ctrl Pts',(-18.3632946073683,43.4670499237467,124.011990264435)) ;
#84283=CARTESIAN_POINT('Ctrl Pts',(-18.2746464011047,43.4770662856562,123.82097505322)) ;
#84284=CARTESIAN_POINT('Ctrl Pts',(-18.2209433721218,43.4871029411616,123.616933241554)) ;
#84285=CARTESIAN_POINT('Ctrl Pts',(-18.2032793807859,43.4969330713509,123.411004635612)) ;
#84286=CARTESIAN_POINT('Ctrl Pts',(-18.2220212371663,43.5070091244408,123.20004552969)) ;
#84287=CARTESIAN_POINT('Ctrl Pts',(-18.2757963342158,43.5168613536266,122.999978140461)) ;
#84288=CARTESIAN_POINT('Ctrl Pts',(-18.3652659387053,43.5269345614259,122.808072789942)) ;
#84289=CARTESIAN_POINT('Ctrl Pts',(-18.4839781003294,43.5367760727773,122.638602022809)) ;
#84290=CARTESIAN_POINT('Ctrl Pts',(-18.6315156170314,43.5467370108148,122.49000026879)) ;
#84291=CARTESIAN_POINT('Ctrl Pts',(-18.8041793234811,43.5567748727398,122.368686470592)) ;
#84292=CARTESIAN_POINT('Ctrl Pts',(-18.9920325810589,43.5666490587369,122.280289825011)) ;
#84293=CARTESIAN_POINT('Ctrl Pts',(-19.1963084092414,43.5767192183147,122.22480654154)) ;
#84294=CARTESIAN_POINT('Ctrl Pts',(-19.402160991638,43.5865509657406,122.205953810568)) ;
#84295=CARTESIAN_POINT('Ctrl Pts',(-19.6124556385658,43.5965870458119,122.222937574671)) ;
#84296=CARTESIAN_POINT('Ctrl Pts',(-19.8161059834079,43.6066040926644,122.276596417447)) ;
#84297=CARTESIAN_POINT('Ctrl Pts',(-20.0049292669574,43.616486350831,122.363254720361)) ;
#84298=CARTESIAN_POINT('Ctrl Pts',(-20.1777775708207,43.6264740336273,122.482430150644)) ;
#84299=CARTESIAN_POINT('Ctrl Pts',(-20.3268505663484,43.6364206903441,122.629119310291)) ;
#84300=CARTESIAN_POINT('Ctrl Pts',(-20.4493262904899,43.6464777484242,122.801435835122)) ;
#84301=CARTESIAN_POINT('Ctrl Pts',(-20.5381405147354,43.6562959279737,122.987771873157)) ;
#84302=CARTESIAN_POINT('Ctrl Pts',(-20.5950205298352,43.6663318624127,123.190941554761)) ;
#84303=CARTESIAN_POINT('Ctrl Pts',(-20.6151355410255,43.6763565168417,123.400737123359)) ;
#84304=CARTESIAN_POINT('Ctrl Pts',(-20.5992612062192,43.6862085364212,123.607251304135)) ;
#84305=CARTESIAN_POINT('Ctrl Pts',(-20.5473617823272,43.6961994501361,123.810752814889)) ;
#84306=CARTESIAN_POINT('Ctrl Pts',(-20.4616503372551,43.7061174389757,124.000855972249)) ;
#84307=CARTESIAN_POINT('Ctrl Pts',(-20.3429941356077,43.7161455497065,124.17509706111)) ;
#84308=CARTESIAN_POINT('Ctrl Pts',(-20.1980312028953,43.7260307476149,124.324012626185)) ;
#84309=CARTESIAN_POINT('Ctrl Pts',(-20.0279376936583,43.7360200228829,124.447192063469)) ;
#84310=CARTESIAN_POINT('Ctrl Pts',(-19.8378630861795,43.7460614810524,124.539030414508)) ;
#84311=CARTESIAN_POINT('Ctrl Pts',(-19.6390701324391,43.7558929448407,124.595638016703)) ;
#84312=CARTESIAN_POINT('Ctrl Pts',(-19.4299206998209,43.7658978771446,124.617705082745)) ;
#84313=CARTESIAN_POINT('Ctrl Pts',(-19.2204529465553,43.7758842410393,124.603030014934)) ;
#84314=CARTESIAN_POINT('Ctrl Pts',(-19.0159260256037,43.7859138699252,124.551840171341)) ;
#84315=CARTESIAN_POINT('Ctrl Pts',(-18.8262138026566,43.7957890920336,124.467467725213)) ;
#84316=CARTESIAN_POINT('Ctrl Pts',(-18.6517412402782,43.8057903044307,124.350192701147)) ;
#84317=CARTESIAN_POINT('Ctrl Pts',(-18.5014974685159,43.8156988836662,124.205849690348)) ;
#84318=CARTESIAN_POINT('Ctrl Pts',(-18.3768780512125,43.8257537362222,124.035148133203)) ;
#84319=CARTESIAN_POINT('Ctrl Pts',(-18.2853633379775,43.835612318497,123.849147658235)) ;
#84320=CARTESIAN_POINT('Ctrl Pts',(-18.2262007825756,43.8456804479396,123.645952411411)) ;
#84321=CARTESIAN_POINT('Ctrl Pts',(-18.203715267376,43.8555359196287,123.439965697177)) ;
#84322=CARTESIAN_POINT('Ctrl Pts',(-18.2168996593856,43.865530768015,123.230263427159)) ;
#84323=CARTESIAN_POINT('Ctrl Pts',(-18.2669194322133,43.8755620647995,123.025387399113)) ;
#84324=CARTESIAN_POINT('Ctrl Pts',(-18.3500573743321,43.8854286010096,122.835344597124)) ;
#84325=CARTESIAN_POINT('Ctrl Pts',(-18.4660377743392,43.8954160239704,122.660345771646)) ;
#84326=CARTESIAN_POINT('Ctrl Pts',(-18.6099846193016,43.9053609629902,122.508677841172)) ;
#84327=CARTESIAN_POINT('Ctrl Pts',(-18.7797941717303,43.9154058488502,122.383164608696)) ;
#84328=CARTESIAN_POINT('Ctrl Pts',(-18.9654667340032,43.9252743839364,122.290585232131)) ;
#84329=CARTESIAN_POINT('Ctrl Pts',(-19.1661752384791,43.9352402519431,122.230514467672)) ;
#84330=CARTESIAN_POINT('Ctrl Pts',(-19.3755016092463,43.9452628993956,122.206300298723)) ;
#84331=CARTESIAN_POINT('Ctrl Pts',(-19.583752931223,43.9551865384032,122.218617120769)) ;
#84332=CARTESIAN_POINT('Ctrl Pts',(-19.7872305258696,43.9651292634089,122.266516179803)) ;
#84333=CARTESIAN_POINT('Ctrl Pts',(-19.9811657967004,43.9751748694608,122.350095113591)) ;
#84334=CARTESIAN_POINT('Ctrl Pts',(-20.1545571070679,43.9850362919819,122.463777119903)) ;
#84335=CARTESIAN_POINT('Ctrl Pts',(-20.3078102053902,43.9950298604311,122.607448060503)) ;
#84336=CARTESIAN_POINT('Ctrl Pts',(-20.4330542345469,44.0049553311864,122.774384345054)) ;
#84337=CARTESIAN_POINT('Ctrl Pts',(-20.5283647722935,44.0149830051423,122.962392956857)) ;
#84338=CARTESIAN_POINT('Ctrl Pts',(-20.588933840108,44.0248701831839,123.161260937744)) ;
#84339=CARTESIAN_POINT('Ctrl Pts',(-20.6145511580893,44.0348985625521,123.37049929144)) ;
#84340=CARTESIAN_POINT('Ctrl Pts',(-20.6037082962981,44.0447928052736,123.578247921938)) ;
#84341=CARTESIAN_POINT('Ctrl Pts',(-20.5408575074722,44.0581457219245,123.851835509504)) ;
#84342=CARTESIAN_POINT('Ctrl Pts',(-20.4095228682182,44.0713482396712,124.100006403082)) ;
#84343=CARTESIAN_POINT('Ctrl Pts',(-20.2186591011258,44.0847041449522,124.305849465822)) ;
#84344=CARTESIAN_POINT('Ctrl Pts',(-20.0529407671226,44.09460079359,124.431709382734)) ;
#84345=CARTESIAN_POINT('Ctrl Pts',(-19.865133373299,44.1046489316425,124.528373373342)) ;
#84346=CARTESIAN_POINT('Ctrl Pts',(-19.6665214872006,44.1145398918202,124.589983507587)) ;
#84347=CARTESIAN_POINT('Ctrl Pts',(-19.4581739575967,44.124532727697,124.616965016942)) ;
#84348=CARTESIAN_POINT('Ctrl Pts',(-19.2473737978853,44.1345718226986,124.606831455382)) ;
#84349=CARTESIAN_POINT('Ctrl Pts',(-19.0455363706327,44.1444091785497,124.561650521355)) ;
#84350=CARTESIAN_POINT('Ctrl Pts',(-18.7855906137243,44.1578021264805,124.453535581331)) ;
#84351=CARTESIAN_POINT('Ctrl Pts',(-18.5635140073878,44.1709688029074,124.282902241153)) ;
#84352=CARTESIAN_POINT('Ctrl Pts',(-18.3921555813385,44.1843535843142,124.059820793974)) ;
#84353=CARTESIAN_POINT('Ctrl Pts',(-18.2962312056799,44.194215366958,123.875972393078)) ;
#84354=CARTESIAN_POINT('Ctrl Pts',(-18.2325177147997,44.2042145149111,123.67569306529)) ;
#84355=CARTESIAN_POINT('Ctrl Pts',(-18.2046131479773,44.2141173075282,123.469337303131)) ;
#84356=CARTESIAN_POINT('Ctrl Pts',(-18.213138129981,44.2241668874191,123.258291526556)) ;
#84357=CARTESIAN_POINT('Ctrl Pts',(-18.2717479171345,44.2373539612286,122.987197784556)) ;
#84358=CARTESIAN_POINT('Ctrl Pts',(-18.4346577722479,44.2541067511998,122.670626830962)) ;
#84359=CARTESIAN_POINT('Ctrl Pts',(-18.6920466309599,44.2705954032945,122.432275015599)) ;
#84360=CARTESIAN_POINT('Ctrl Pts',(-18.9400674710734,44.2839522294779,122.300862352034)) ;
#84361=CARTESIAN_POINT('Ctrl Pts',(-19.138050968932,44.2938486143558,122.236740395541)) ;
#84362=CARTESIAN_POINT('Ctrl Pts',(-19.3463245926845,44.3038551288763,122.207560046898)) ;
#84363=CARTESIAN_POINT('Ctrl Pts',(-19.6235857637495,44.3170452523927,122.216668886464)) ;
#84364=CARTESIAN_POINT('Ctrl Pts',(-19.9644817452573,44.3338118135422,122.320510300557)) ;
#84365=CARTESIAN_POINT('Ctrl Pts',(-20.3009628630552,44.3535963022503,122.573194318011)) ;
#84366=CARTESIAN_POINT('Ctrl Pts',(-20.5338593298856,44.3735417498468,122.927488552972)) ;
#84367=CARTESIAN_POINT('Ctrl Pts',(-20.6313432869638,44.3934534120027,123.339498229976)) ;
#84368=CARTESIAN_POINT('Ctrl Pts',(-20.5833486351149,44.4133456040216,123.759794081848)) ;
#84369=CARTESIAN_POINT('Ctrl Pts',(-20.3928831894929,44.4333867345762,124.140920711645)) ;
#84370=CARTESIAN_POINT('Ctrl Pts',(-20.0872651790941,44.4532050691918,124.43118843213)) ;
#84371=CARTESIAN_POINT('Ctrl Pts',(-19.6984334120506,44.4731776344114,124.601580084721)) ;
#84372=CARTESIAN_POINT('Ctrl Pts',(-19.2762688089198,44.493066850583,124.629069320153)) ;
#84373=CARTESIAN_POINT('Ctrl Pts',(-18.8676588274966,44.5130904249057,124.509843418797)) ;
#84374=CARTESIAN_POINT('Ctrl Pts',(-18.5278180218302,44.5328875879939,124.261320788567)) ;
#84375=CARTESIAN_POINT('Ctrl Pts',(-18.2904318127847,44.5528530818177,123.909483353914)) ;
#84376=CARTESIAN_POINT('Ctrl Pts',(-18.1878781245095,44.5728067895591,123.497677772688)) ;
#84377=CARTESIAN_POINT('Ctrl Pts',(-18.2318637933429,44.5927141662857,123.076780022158)) ;
#84378=CARTESIAN_POINT('Ctrl Pts',(-18.4153836924114,44.6125663778343,122.696570163402)) ;
#84379=CARTESIAN_POINT('Ctrl Pts',(-18.721213427716,44.63263876478,122.398901462891)) ;
#84380=CARTESIAN_POINT('Ctrl Pts',(-19.1059665362462,44.6524766344203,122.226015016883)) ;
#84381=CARTESIAN_POINT('Ctrl Pts',(-19.5267471287715,44.6723272889734,122.192956241741)) ;
#84382=CARTESIAN_POINT('Ctrl Pts',(-19.9374777977326,44.6923792233138,122.307204924401)) ;
#84383=CARTESIAN_POINT('Ctrl Pts',(-20.2808528712217,44.7122124108799,122.552178876658)) ;
#84384=CARTESIAN_POINT('Ctrl Pts',(-20.5217265853229,44.7321416231106,122.900618651357)) ;
#84385=CARTESIAN_POINT('Ctrl Pts',(-20.6295648496897,44.752026588325,123.309611273299)) ;
#84386=CARTESIAN_POINT('Ctrl Pts',(-20.5903665879315,44.7721003294696,123.734542133322)) ;
#84387=CARTESIAN_POINT('Ctrl Pts',(-20.4110379245902,44.79189351125,124.115354659194)) ;
#84388=CARTESIAN_POINT('Ctrl Pts',(-20.1109493954123,44.8118562192527,124.41549537119)) ;
#84389=CARTESIAN_POINT('Ctrl Pts',(-19.7255903117033,44.8318391709951,124.594483377586)) ;
#84390=CARTESIAN_POINT('Ctrl Pts',(-19.3059767207478,44.8516497907673,124.631738883303)) ;
#84391=CARTESIAN_POINT('Ctrl Pts',(-18.8952790350949,44.8716335068002,124.523139946406)) ;
#84392=CARTESIAN_POINT('Ctrl Pts',(-18.5479537981365,44.8915149706975,124.28197876055)) ;
#84393=CARTESIAN_POINT('Ctrl Pts',(-18.302732820425,44.9114703005419,123.935816472258)) ;
#84394=CARTESIAN_POINT('Ctrl Pts',(-18.1904707648224,44.9313457613473,123.528324077861)) ;
#84395=CARTESIAN_POINT('Ctrl Pts',(-18.2239253980212,44.9513300813989,123.104770271589)) ;
#84396=CARTESIAN_POINT('Ctrl Pts',(-18.3996904016786,44.9712581141885,122.719111274452)) ;
#84397=CARTESIAN_POINT('Ctrl Pts',(-18.6468965811825,44.9878668761283,122.467052957218)) ;
#84398=CARTESIAN_POINT('Ctrl Pts',(-18.885415024673,45.0010545148184,122.325643231264)) ;
#84399=CARTESIAN_POINT('Ctrl Pts',(-19.0816687636844,45.0110409491785,122.251110513577)) ;
#84400=CARTESIAN_POINT('Ctrl Pts',(-19.2884343852017,45.0210503231378,122.211902199266)) ;
#84401=CARTESIAN_POINT('Ctrl Pts',(-19.5677616357913,45.0343403567031,122.208107593301)) ;
#84402=CARTESIAN_POINT('Ctrl Pts',(-19.9099464874213,45.0509343443656,122.29446682086)) ;
#84403=CARTESIAN_POINT('Ctrl Pts',(-20.2026694566148,45.0675665996411,122.492797279563)) ;
#84404=CARTESIAN_POINT('Ctrl Pts',(-20.384991023903,45.080808983309,122.703234497855)) ;
#84405=CARTESIAN_POINT('Ctrl Pts',(-20.4925937355116,45.0907231915364,122.881741621572)) ;
#84406=CARTESIAN_POINT('Ctrl Pts',(-20.568416740875,45.1007798308081,123.07908485721)) ;
#84407=CARTESIAN_POINT('Ctrl Pts',(-20.6082256043889,45.1106256372282,123.282226390095)) ;
#84408=CARTESIAN_POINT('Ctrl Pts',(-20.612596696362,45.1206706368614,123.493357737852)) ;
#84409=CARTESIAN_POINT('Ctrl Pts',(-20.5694219253255,45.1339516592341,123.769153352634)) ;
#84410=CARTESIAN_POINT('Ctrl Pts',(-20.4566672380709,45.1471491057588,124.026150825483)) ;
#84411=CARTESIAN_POINT('Ctrl Pts',(-20.280126516246,45.1605634035657,124.246100642346)) ;
#84412=CARTESIAN_POINT('Ctrl Pts',(-20.1246823586444,45.1704024689685,124.382580114351)) ;
#84413=CARTESIAN_POINT('Ctrl Pts',(-19.9456254623816,45.1803856752462,124.49202682819)) ;
#84414=CARTESIAN_POINT('Ctrl Pts',(-19.7508537829088,45.190336910159,124.568420987033)) ;
#84415=CARTESIAN_POINT('Ctrl Pts',(-19.5448027598535,45.2003379098606,124.610291845591)) ;
#84416=CARTESIAN_POINT('Ctrl Pts',(-19.3339774210853,45.2103692556479,124.615434704807)) ;
#84417=CARTESIAN_POINT('Ctrl Pts',(-19.1291027096562,45.220223020353,124.58473277515)) ;
#84418=CARTESIAN_POINT('Ctrl Pts',(-18.9302085771127,45.2301936740213,124.518626237724)) ;
#84419=CARTESIAN_POINT('Ctrl Pts',(-18.7452783058747,45.2401909176785,124.418690904311)) ;
#84420=CARTESIAN_POINT('Ctrl Pts',(-18.5801193737719,45.2502243736227,124.287508830628)) ;
#84421=CARTESIAN_POINT('Ctrl Pts',(-18.4424514372433,45.2600798779231,124.13263744952)) ;
#84422=CARTESIAN_POINT('Ctrl Pts',(-18.3319695805143,45.2700793142092,123.953834867365)) ;
#84423=CARTESIAN_POINT('Ctrl Pts',(-18.2547793585316,45.2799737737251,123.760632288585)) ;
#84424=CARTESIAN_POINT('Ctrl Pts',(-18.2116609512092,45.2900368931767,123.553551735828)) ;
#84425=CARTESIAN_POINT('Ctrl Pts',(-18.2050676042058,45.2998765275887,123.346762433404)) ;
#84426=CARTESIAN_POINT('Ctrl Pts',(-18.2348732954205,45.3099397350745,123.13734193917)) ;
#84427=CARTESIAN_POINT('Ctrl Pts',(-18.299665433266,45.3198338424537,122.93966000259)) ;
#84428=CARTESIAN_POINT('Ctrl Pts',(-18.3977574508029,45.3297761746461,122.75511979076)) ;
#84429=CARTESIAN_POINT('Ctrl Pts',(-18.5271124110106,45.3397768009611,122.589336702802)) ;
#84430=CARTESIAN_POINT('Ctrl Pts',(-18.6841544889452,45.349818535243,122.448281249036)) ;
#84431=CARTESIAN_POINT('Ctrl Pts',(-18.8592295883591,45.3596439611921,122.338633546838)) ;
#84432=CARTESIAN_POINT('Ctrl Pts',(-19.0550454530649,45.3697007877197,122.258943893974)) ;
#84433=CARTESIAN_POINT('Ctrl Pts',(-19.2591518279753,45.3796282208413,122.215318487918)) ;
#84434=CARTESIAN_POINT('Ctrl Pts',(-19.468181276108,45.3895782132475,122.20718013329)) ;
#84435=CARTESIAN_POINT('Ctrl Pts',(-19.6775673120917,45.3996334143215,122.236125936073)) ;
#84436=CARTESIAN_POINT('Ctrl Pts',(-19.8742295194565,45.4094556883738,122.299140356534)) ;
#84437=CARTESIAN_POINT('Ctrl Pts',(-20.061457560878,45.4195115823331,122.397284056323)) ;
#84438=CARTESIAN_POINT('Ctrl Pts',(-20.2266741638109,45.4294523041782,122.52527460033)) ;
#84439=CARTESIAN_POINT('Ctrl Pts',(-20.3671232504393,45.4393566482648,122.678999529168)) ;
#84440=CARTESIAN_POINT('Ctrl Pts',(-20.4802264787038,45.4494033155643,122.857355769901)) ;
#84441=CARTESIAN_POINT('Ctrl Pts',(-20.5596285804351,45.4592988740142,123.04967868684)) ;
#84442=CARTESIAN_POINT('Ctrl Pts',(-20.6051710365697,45.4693609527189,123.256223873825)) ;
#84443=CARTESIAN_POINT('Ctrl Pts',(-20.6140833446175,45.4792036511847,123.462979287271)) ;
#84444=CARTESIAN_POINT('Ctrl Pts',(-20.5870525350675,45.4891944250792,123.671243809474)) ;
#84445=CARTESIAN_POINT('Ctrl Pts',(-20.5246209778266,45.4991222943141,123.870412109524)) ;
#84446=CARTESIAN_POINT('Ctrl Pts',(-20.4282957886132,45.5091110232839,124.057023148898)) ;
#84447=CARTESIAN_POINT('Ctrl Pts',(-20.3000887267814,45.5191504252677,124.224668111442)) ;
#84448=CARTESIAN_POINT('Ctrl Pts',(-20.1480643821402,45.5289905930044,124.364985804919)) ;
#84449=CARTESIAN_POINT('Ctrl Pts',(-19.9704897783103,45.5390388033789,124.479388559856)) ;
#84450=CARTESIAN_POINT('Ctrl Pts',(-19.7775671836577,45.5489859736667,124.560097142958)) ;
#84451=CARTESIAN_POINT('Ctrl Pts',(-19.5744414701754,45.5588968219218,124.606523876973)) ;
#84452=CARTESIAN_POINT('Ctrl Pts',(-19.3632945131307,45.5689531495995,124.616929810979)) ;
#84453=CARTESIAN_POINT('Ctrl Pts',(-19.1577990571512,45.5788035623681,124.591231951628)) ;
#84454=CARTESIAN_POINT('Ctrl Pts',(-18.9562025286816,45.5888304482018,124.529644846341)) ;
#84455=CARTESIAN_POINT('Ctrl Pts',(-18.7685671889028,45.5988590638326,124.433479707402)) ;
#84456=CARTESIAN_POINT('Ctrl Pts',(-18.6033345097439,45.6087042872101,124.308847799277)) ;
#84457=CARTESIAN_POINT('Ctrl Pts',(-18.4597435271059,45.6186949693117,124.155554328125)) ;
#84458=CARTESIAN_POINT('Ctrl Pts',(-18.3448064911182,45.6287328579441,123.978575656932)) ;
#84459=CARTESIAN_POINT('Ctrl Pts',(-18.2635978094481,45.6385771930473,123.788206651437)) ;
#84460=CARTESIAN_POINT('Ctrl Pts',(-18.215612918174,45.6485621552448,123.583878844602)) ;
#84461=CARTESIAN_POINT('Ctrl Pts',(-18.2037886155601,45.6585010967782,123.37523545725)) ;
#84462=CARTESIAN_POINT('Ctrl Pts',(-18.2286862705219,45.6685429817496,123.16561689975)) ;
#84463=CARTESIAN_POINT('Ctrl Pts',(-18.2885437879519,45.6784295296579,122.966555275257)) ;
#84464=CARTESIAN_POINT('Ctrl Pts',(-18.3827734140441,45.6884234551579,122.778797314709)) ;
#84465=CARTESIAN_POINT('Ctrl Pts',(-18.5074028980685,45.6983595462843,122.6111225881)) ;
#84466=CARTESIAN_POINT('Ctrl Pts',(-18.6606617579988,45.7083888152643,122.466359772254)) ;
#84467=CARTESIAN_POINT('Ctrl Pts',(-18.834052688656,45.7182711978236,122.351852188486)) ;
#84468=CARTESIAN_POINT('Ctrl Pts',(-19.0278880707733,45.7283237149114,122.267728229744)) ;
#84469=CARTESIAN_POINT('Ctrl Pts',(-19.2301906235251,45.7382178357354,122.219193860073)) ;
#84470=CARTESIAN_POINT('Ctrl Pts',(-19.4413039395695,45.7482798151558,122.206261137265)) ;
#84471=CARTESIAN_POINT('Ctrl Pts',(-19.6469492061947,45.7581243483847,122.229642983626)) ;
#84472=CARTESIAN_POINT('Ctrl Pts',(-19.847942922004,45.768084427291,122.288339198138)) ;
#84473=CARTESIAN_POINT('Ctrl Pts',(-20.0369764458074,45.7781227038636,122.382139593977)) ;
#84474=CARTESIAN_POINT('Ctrl Pts',(-20.2043294583818,45.7879960904014,122.504984319071)) ;
#84475=CARTESIAN_POINT('Ctrl Pts',(-20.3506163202273,45.7980690331685,122.658044794021)) ;
#84476=CARTESIAN_POINT('Ctrl Pts',(-20.4654246764655,45.8078904472968,122.829707697927)) ;
#84477=CARTESIAN_POINT('Ctrl Pts',(-20.5510305730476,45.8179650773691,123.023395222281)) ;
#84478=CARTESIAN_POINT('Ctrl Pts',(-20.6005900658558,45.827831714686,123.224841812656)) ;
#84479=CARTESIAN_POINT('Ctrl Pts',(-20.6151763356349,45.8378552600578,123.435053208665)) ;
#84480=CARTESIAN_POINT('Ctrl Pts',(-20.592528635638,45.847881011575,123.644618732393)) ;
#84481=CARTESIAN_POINT('Ctrl Pts',(-20.5351846913682,45.8577345985843,123.843665085029)) ;
#84482=CARTESIAN_POINT('Ctrl Pts',(-20.4435052217378,45.8677115588123,124.032319507282)) ;
#84483=CARTESIAN_POINT('Ctrl Pts',(-20.3196371636077,45.8777327018408,124.202720700626)) ;
#84484=CARTESIAN_POINT('Ctrl Pts',(-20.1704222805544,45.8876153078607,124.347330375355)) ;
#84485=CARTESIAN_POINT('Ctrl Pts',(-19.9951347291686,45.8976837784934,124.465921431324)) ;
#84486=CARTESIAN_POINT('Ctrl Pts',(-19.8065276112628,45.9075138616771,124.550478460805)) ;
#84487=CARTESIAN_POINT('Ctrl Pts',(-19.6014167263255,45.9175804213574,124.602468015969)) ;
#84488=CARTESIAN_POINT('Ctrl Pts',(-19.3940227475724,45.9274706711867,124.61765622834)) ;
#84489=CARTESIAN_POINT('Ctrl Pts',(-19.1850008925533,45.9374628369355,124.596848271941)) ;
#84490=CARTESIAN_POINT('Ctrl Pts',(-18.9834082274553,45.9474256805316,124.540036386113)) ;
#84491=CARTESIAN_POINT('Ctrl Pts',(-18.7956023361387,45.9573298493593,124.450088171428)) ;
#84492=CARTESIAN_POINT('Ctrl Pts',(-18.6237362733502,45.9673907242537,124.326851238018)) ;
#84493=CARTESIAN_POINT('Ctrl Pts',(-18.4788922942551,45.977229627583,124.179140512665)) ;
#84494=CARTESIAN_POINT('Ctrl Pts',(-18.359037504779,45.9872980039569,124.004715589726)) ;
#84495=CARTESIAN_POINT('Ctrl Pts',(-18.2729630369527,45.9971786205896,123.815633475423)) ;
#84496=CARTESIAN_POINT('Ctrl Pts',(-18.22005104732,46.0071697808186,123.612393236317)) ;
#84497=CARTESIAN_POINT('Ctrl Pts',(-18.2032574682917,46.0171228542507,123.403791948476)) ;
#84498=CARTESIAN_POINT('Ctrl Pts',(-18.2231668439234,46.0271586898633,123.193765792517)) ;
#84499=CARTESIAN_POINT('Ctrl Pts',(-18.278298274426,46.0370488165935,122.993273294469)) ;
#84500=CARTESIAN_POINT('Ctrl Pts',(-18.3680085315035,46.0470409983628,122.803337401315)) ;
#84501=CARTESIAN_POINT('Ctrl Pts',(-18.48883758189,46.0569869383372,122.632688949944)) ;
#84502=CARTESIAN_POINT('Ctrl Pts',(-18.6371890134999,46.0669341220967,122.485284985213)) ;
#84503=CARTESIAN_POINT('Ctrl Pts',(-18.8107407202325,46.076982060387,122.364873623863)) ;
#84504=CARTESIAN_POINT('Ctrl Pts',(-18.9986732432391,46.0868296952006,122.278026559726)) ;
#84505=CARTESIAN_POINT('Ctrl Pts',(-19.2009700027035,46.0967914088986,122.223885449461)) ;
#84506=CARTESIAN_POINT('Ctrl Pts',(-19.411042470006,46.1068200447197,122.205834191344)) ;
#84507=CARTESIAN_POINT('Ctrl Pts',(-19.6185632505069,46.1167303594715,122.224242554186)) ;
#84508=CARTESIAN_POINT('Ctrl Pts',(-19.8203927501633,46.1266652301342,122.278012310979)) ;
#84509=CARTESIAN_POINT('Ctrl Pts',(-20.0117474066158,46.1367064125359,122.367127720079)) ;
#84510=CARTESIAN_POINT('Ctrl Pts',(-20.1821838321545,46.1465933840007,122.486134507027)) ;
#84511=CARTESIAN_POINT('Ctrl Pts',(-20.3311988089654,46.1565928162633,122.634375530162)) ;
#84512=CARTESIAN_POINT('Ctrl Pts',(-20.4513952266997,46.1665128815199,122.804835876269)) ;
#84513=CARTESIAN_POINT('Ctrl Pts',(-20.5412360542906,46.1765497341041,122.995747933808)) ;
#84514=CARTESIAN_POINT('Ctrl Pts',(-20.59587728788,46.186462393444,123.196855992653)) ;
#84515=CARTESIAN_POINT('Ctrl Pts',(-20.6153750507368,46.1964536053589,123.406008416068)) ;
#84516=CARTESIAN_POINT('Ctrl Pts',(-20.5977036062115,46.2064952467621,123.616357743328)) ;
#84517=CARTESIAN_POINT('Ctrl Pts',(-20.5454116592005,46.2163240409691,123.816292436209)) ;
#84518=CARTESIAN_POINT('Ctrl Pts',(-20.4571378572033,46.2264004520904,124.008815850834)) ;
#84519=CARTESIAN_POINT('Ctrl Pts',(-20.339495499964,46.2362525851328,124.179339841369)) ;
#84520=CARTESIAN_POINT('Ctrl Pts',(-20.1909503583246,46.2463258194742,124.330227020492)) ;
#84521=CARTESIAN_POINT('Ctrl Pts',(-20.022359060117,46.2561673208008,124.450184743589)) ;
#84522=CARTESIAN_POINT('Ctrl Pts',(-19.8335905201032,46.2661282723956,124.540828601706)) ;
#84523=CARTESIAN_POINT('Ctrl Pts',(-19.6302804392769,46.2761660901162,124.597348545521)) ;
#84524=CARTESIAN_POINT('Ctrl Pts',(-19.4236714780948,46.2860404393733,124.617764022101)) ;
#84525=CARTESIAN_POINT('Ctrl Pts',(-19.2126193295471,46.2961099901155,124.601674273063)) ;
#84526=CARTESIAN_POINT('Ctrl Pts',(-19.0122872962936,46.3059440096241,124.550514499661)) ;
#84527=CARTESIAN_POINT('Ctrl Pts',(-18.8198464982895,46.3159781642036,124.46413465279)) ;
#84528=CARTESIAN_POINT('Ctrl Pts',(-18.6459181761566,46.3259940900261,124.345423519706)) ;
#84529=CARTESIAN_POINT('Ctrl Pts',(-18.4970009615531,46.3358763452203,124.200552798175)) ;
#84530=CARTESIAN_POINT('Ctrl Pts',(-18.3739944708057,46.3458651517313,124.030382105074)) ;
#84531=CARTESIAN_POINT('Ctrl Pts',(-18.2826050981716,46.355813718994,123.842218558594)) ;
#84532=CARTESIAN_POINT('Ctrl Pts',(-18.2248950683396,46.365868524296,123.638888671338)) ;
#84533=CARTESIAN_POINT('Ctrl Pts',(-18.2035713060587,46.3756873075596,123.433561300174)) ;
#84534=CARTESIAN_POINT('Ctrl Pts',(-18.2179813445457,46.3857230799201,123.223075302304)) ;
#84535=CARTESIAN_POINT('Ctrl Pts',(-18.2692515878222,46.3957477789488,123.018648166375)) ;
#84536=CARTESIAN_POINT('Ctrl Pts',(-18.3533370689887,46.4055997822079,122.829360936852)) ;
#84537=CARTESIAN_POINT('Ctrl Pts',(-18.4703613694233,46.4155907166051,122.654971104637)) ;
#84538=CARTESIAN_POINT('Ctrl Pts',(-18.6147606329656,46.4255086390362,122.504524558652)) ;
#84539=CARTESIAN_POINT('Ctrl Pts',(-18.7849011229507,46.4355369947185,122.380053429102)) ;
#84540=CARTESIAN_POINT('Ctrl Pts',(-18.9713293231097,46.4454212792291,122.28824983603)) ;
#84541=CARTESIAN_POINT('Ctrl Pts',(-19.1729140858886,46.455413963137,122.229120010516)) ;
#84542=CARTESIAN_POINT('Ctrl Pts',(-19.3824991228755,46.4654427001447,122.206173308855)) ;
#84543=CARTESIAN_POINT('Ctrl Pts',(-19.5899010964574,46.4753280967736,122.219495009534)) ;
#84544=CARTESIAN_POINT('Ctrl Pts',(-19.7939762357025,46.4853159821875,122.268837874836)) ;
#84545=CARTESIAN_POINT('Ctrl Pts',(-19.9857528123901,46.4952666848481,122.352485219102)) ;
#84546=CARTESIAN_POINT('Ctrl Pts',(-20.1615560713129,46.5053070029455,122.469269470923)) ;
#84547=CARTESIAN_POINT('Ctrl Pts',(-20.312061766034,46.5151815682787,122.612283972297)) ;
#84548=CARTESIAN_POINT('Ctrl Pts',(-20.4371930749062,46.5251812283398,122.781168558307)) ;
#84549=CARTESIAN_POINT('Ctrl Pts',(-20.5304591793014,46.5350902235075,122.967483463169)) ;
#84550=CARTESIAN_POINT('Ctrl Pts',(-20.5907489828305,46.5451449646707,123.170049998762)) ;
#84551=CARTESIAN_POINT('Ctrl Pts',(-20.6147246473763,46.5550035765845,123.37595414604)) ;
#84552=CARTESIAN_POINT('Ctrl Pts',(-20.6024582716505,46.5650716988639,123.587231213569)) ;
#84553=CARTESIAN_POINT('Ctrl Pts',(-20.5546964518429,46.5749271695671,123.788861895035)) ;
#84554=CARTESIAN_POINT('Ctrl Pts',(-20.4720783495954,46.5849220290604,123.982053985397)) ;
#84555=CARTESIAN_POINT('Ctrl Pts',(-20.3563663950888,46.5949532824024,124.15836793779)) ;
#84556=CARTESIAN_POINT('Ctrl Pts',(-20.2144077351763,46.6048199812755,124.309619911489)) ;
#84557=CARTESIAN_POINT('Ctrl Pts',(-20.0465524126368,46.6148067970267,124.435697555555)) ;
#84558=CARTESIAN_POINT('Ctrl Pts',(-19.8600955779439,46.6247540022221,124.530446736084)) ;
#84559=CARTESIAN_POINT('Ctrl Pts',(-19.658107114407,46.6347969903484,124.591866563251)) ;
#84560=CARTESIAN_POINT('Ctrl Pts',(-19.4521805478414,46.6446643449699,124.616961781733)) ;
#84561=CARTESIAN_POINT('Ctrl Pts',(-19.2429425710295,46.654630238268,124.606374914884)) ;
#84562=CARTESIAN_POINT('Ctrl Pts',(-19.0375622495762,46.6646540156441,124.559128817244)) ;
#84563=CARTESIAN_POINT('Ctrl Pts',(-18.8454096947828,46.6745795635758,124.477797817512)) ;
#84564=CARTESIAN_POINT('Ctrl Pts',(-18.669747000263,46.6845200399968,124.364570074209)) ;
#84565=CARTESIAN_POINT('Ctrl Pts',(-18.5149640442547,46.6945662496597,124.220891203878)) ;
#84566=CARTESIAN_POINT('Ctrl Pts',(-18.3896311544296,46.7044275063215,124.055728940118)) ;
#84567=CARTESIAN_POINT('Ctrl Pts',(-18.2933092985916,46.7144211345968,123.869046552226)) ;
#84568=CARTESIAN_POINT('Ctrl Pts',(-18.2311685573197,46.724346531907,123.669818227534)) ;
#84569=CARTESIAN_POINT('Ctrl Pts',(-18.2042912868287,46.7343744398172,123.460747783017)) ;
#84570=CARTESIAN_POINT('Ctrl Pts',(-18.2137735619061,46.7442607554864,123.253092008572)) ;
#84571=CARTESIAN_POINT('Ctrl Pts',(-18.2597106116491,46.7542923503902,123.047294541768)) ;
#84572=CARTESIAN_POINT('Ctrl Pts',(-18.3393267948155,46.7641745933419,122.855362781302)) ;
#84573=CARTESIAN_POINT('Ctrl Pts',(-18.4529567609936,46.7742340643717,122.677029439703)) ;
#84574=CARTESIAN_POINT('Ctrl Pts',(-18.5931277415802,46.7841005090349,122.524119542989)) ;
#84575=CARTESIAN_POINT('Ctrl Pts',(-18.7589660899219,46.7940666334836,122.396081360997)) ;
#84576=CARTESIAN_POINT('Ctrl Pts',(-18.9458707343078,46.8040968768747,122.298455537853)) ;
#84577=CARTESIAN_POINT('Ctrl Pts',(-19.1440685456171,46.8139899118278,122.235347192875)) ;
#84578=CARTESIAN_POINT('Ctrl Pts',(-19.353458752379,46.8240408260646,122.207116932518)) ;
#84579=CARTESIAN_POINT('Ctrl Pts',(-19.5612106214837,46.8339306522892,122.215512469215)) ;
#84580=CARTESIAN_POINT('Ctrl Pts',(-19.8352624788568,46.8472654673361,122.274762009686)) ;
#84581=CARTESIAN_POINT('Ctrl Pts',(-20.0862026626761,46.8605425585076,122.404067043679)) ;
#84582=CARTESIAN_POINT('Ctrl Pts',(-20.2927726621347,46.8737908471059,122.590867832793)) ;
#84583=CARTESIAN_POINT('Ctrl Pts',(-20.4224375530319,46.8838456885999,122.757782588646)) ;
#84584=CARTESIAN_POINT('Ctrl Pts',(-20.5192876968314,46.8936766779075,122.940402665893)) ;
#84585=CARTESIAN_POINT('Ctrl Pts',(-20.5846756847044,46.9037532422307,123.141863683039)) ;
#84586=CARTESIAN_POINT('Ctrl Pts',(-20.6134306387111,46.9136025673647,123.346938432967)) ;
#84587=CARTESIAN_POINT('Ctrl Pts',(-20.6042235799873,46.9269505670019,123.627443340569)) ;
#84588=CARTESIAN_POINT('Ctrl Pts',(-20.5014828829124,46.9435353265385,123.964713423941)) ;
#84589=CARTESIAN_POINT('Ctrl Pts',(-20.2906566355743,46.9601038778866,124.2470189635)) ;
#84590=CARTESIAN_POINT('Ctrl Pts',(-20.0699818080453,46.9734637027056,124.420721815992)) ;
#84591=CARTESIAN_POINT('Ctrl Pts',(-19.8865380012834,46.9833691115362,124.51931119778)) ;
#84592=CARTESIAN_POINT('Ctrl Pts',(-19.6878068412282,46.9933291381203,124.585185778078)) ;
#84593=CARTESIAN_POINT('Ctrl Pts',(-19.4120461780084,47.0065867223056,124.62597415739)) ;
#84594=CARTESIAN_POINT('Ctrl Pts',(-19.0603318090092,47.0232379338003,124.585529981602)) ;
#84595=CARTESIAN_POINT('Ctrl Pts',(-18.6814960970596,47.0431561479106,124.396231532548)) ;
#84596=CARTESIAN_POINT('Ctrl Pts',(-18.3898810922891,47.0630339111314,124.090210992981)) ;
#84597=CARTESIAN_POINT('Ctrl Pts',(-18.2194529069462,47.0830465789186,123.700392596067)) ;
#84598=CARTESIAN_POINT('Ctrl Pts',(-18.1921466433378,47.1028591015852,123.279930301551)) ;
#84599=CARTESIAN_POINT('Ctrl Pts',(-18.3102874267524,47.1228424015851,122.871872118256)) ;
#84600=CARTESIAN_POINT('Ctrl Pts',(-18.5598052667018,47.1427366786864,122.530215788296)) ;
#84601=CARTESIAN_POINT('Ctrl Pts',(-18.9111816446954,47.1626694404441,122.293251063936)) ;
#84602=CARTESIAN_POINT('Ctrl Pts',(-19.3230996718903,47.1826354462089,122.190530008854)) ;
#84603=CARTESIAN_POINT('Ctrl Pts',(-19.7435526621383,47.2025139783737,122.234047576491)) ;
#84604=CARTESIAN_POINT('Ctrl Pts',(-20.1251992562022,47.2224536450341,122.418602153129)) ;
#84605=CARTESIAN_POINT('Ctrl Pts',(-20.4204439982056,47.2423485196794,122.721609107295)) ;
#84606=CARTESIAN_POINT('Ctrl Pts',(-20.5949958913168,47.2622556589728,123.107115801826)) ;
#84607=CARTESIAN_POINT('Ctrl Pts',(-20.6282641793116,47.2821662070513,123.52929662423)) ;
#84608=CARTESIAN_POINT('Ctrl Pts',(-20.5136941343494,47.3022347924084,123.940242952693)) ;
#84609=CARTESIAN_POINT('Ctrl Pts',(-20.2695209604141,47.3220165897232,124.28289844978)) ;
#84610=CARTESIAN_POINT('Ctrl Pts',(-19.9197275897854,47.3420241366677,124.524725500337)) ;
#84611=CARTESIAN_POINT('Ctrl Pts',(-19.5119619969569,47.3618458749706,124.631757155408)) ;
#84612=CARTESIAN_POINT('Ctrl Pts',(-19.0889034892236,47.3818258948748,124.593693820885)) ;
#84613=CARTESIAN_POINT('Ctrl Pts',(-18.7055979157497,47.401743346137,124.41357834132)) ;
#84614=CARTESIAN_POINT('Ctrl Pts',(-18.4066951513726,47.4216182673097,124.114802948108)) ;
#84615=CARTESIAN_POINT('Ctrl Pts',(-18.2266177235489,47.4416426358605,123.72901779228)) ;
#84616=CARTESIAN_POINT('Ctrl Pts',(-18.1894085958522,47.461509320234,123.308171325423)) ;
#84617=CARTESIAN_POINT('Ctrl Pts',(-18.2977813339801,47.4814531420802,122.898242749511)) ;
#84618=CARTESIAN_POINT('Ctrl Pts',(-18.5392371408358,47.5013605113317,122.550578280407)) ;
#84619=CARTESIAN_POINT('Ctrl Pts',(-18.8838107916012,47.5212352090784,122.305940570887)) ;
#84620=CARTESIAN_POINT('Ctrl Pts',(-19.2933813903598,47.5412171516001,122.192858540616)) ;
#84621=CARTESIAN_POINT('Ctrl Pts',(-19.7151773385406,47.561119818511,122.226545830922)) ;
#84622=CARTESIAN_POINT('Ctrl Pts',(-20.099857981226,47.5809751760497,122.400636940011)) ;
#84623=CARTESIAN_POINT('Ctrl Pts',(-20.4047900928406,47.6010392147657,122.698899589428)) ;
#84624=CARTESIAN_POINT('Ctrl Pts',(-20.5876551935011,47.6208943944907,123.079589159602)) ;
#84625=CARTESIAN_POINT('Ctrl Pts',(-20.630201683294,47.6408744991552,123.502119743328)) ;
#84626=CARTESIAN_POINT('Ctrl Pts',(-20.5273230946429,47.660683604325,123.910681522273)) ;
#84627=CARTESIAN_POINT('Ctrl Pts',(-20.2895043292247,47.6806762246657,124.262875655293)) ;
#84628=CARTESIAN_POINT('Ctrl Pts',(-20.005035238579,47.6972157071698,124.469774758122)) ;
#84629=CARTESIAN_POINT('Ctrl Pts',(-19.7428589411892,47.710580025234,124.570749541603)) ;
#84630=CARTESIAN_POINT('Ctrl Pts',(-19.4702099350432,47.7237976277355,124.624411960442)) ;
#84631=CARTESIAN_POINT('Ctrl Pts',(-19.1168449928776,47.7404552220133,124.600779206886)) ;
#84632=CARTESIAN_POINT('Ctrl Pts',(-18.7302031446882,47.760320924055,124.43052412299)) ;
#84633=CARTESIAN_POINT('Ctrl Pts',(-18.4743682268421,47.776950650745,124.186579044811)) ;
#84634=CARTESIAN_POINT('Ctrl Pts',(-18.3289986202607,47.7902397658829,123.947912625341)) ;
#84635=CARTESIAN_POINT('Ctrl Pts',(-18.2525289132203,47.80020411286,123.752907855463)) ;
#84636=CARTESIAN_POINT('Ctrl Pts',(-18.2110894697858,47.8101324808615,123.548334684544)) ;
#84637=CARTESIAN_POINT('Ctrl Pts',(-18.2034573469909,47.8234159139502,123.26919781636)) ;
#84638=CARTESIAN_POINT('Ctrl Pts',(-18.2859430189476,47.8400679916905,122.924823299534)) ;
#84639=CARTESIAN_POINT('Ctrl Pts',(-18.4796140200425,47.8566193609914,122.631051222548)) ;
#84640=CARTESIAN_POINT('Ctrl Pts',(-18.6881382843732,47.8699067891403,122.445096809951)) ;
#84641=CARTESIAN_POINT('Ctrl Pts',(-18.8678491409432,47.8799513288404,122.334247522911)) ;
#84642=CARTESIAN_POINT('Ctrl Pts',(-19.0600721113435,47.8897941706643,122.257599498801)) ;
#84643=CARTESIAN_POINT('Ctrl Pts',(-19.2654626383406,47.8997784549112,122.214420614964)) ;
#84644=CARTESIAN_POINT('Ctrl Pts',(-19.4745348605085,47.9097281003104,122.207626209341)) ;
#84645=CARTESIAN_POINT('Ctrl Pts',(-19.682692403788,47.9197278619988,122.237130756495)) ;
#84646=CARTESIAN_POINT('Ctrl Pts',(-19.8830746242283,47.9297592079577,122.302862418087)) ;
#84647=CARTESIAN_POINT('Ctrl Pts',(-20.0658794612454,47.9396141624348,122.40037377344)) ;
#84648=CARTESIAN_POINT('Ctrl Pts',(-20.2312034863803,47.9495867004353,122.529268259751)) ;
#84649=CARTESIAN_POINT('Ctrl Pts',(-20.3719768873054,47.9595816941703,122.685311409787)) ;
#84650=CARTESIAN_POINT('Ctrl Pts',(-20.4837075519426,47.9696157529644,122.864217847032)) ;
#84651=CARTESIAN_POINT('Ctrl Pts',(-20.561590830256,47.9794710957874,123.056234967956)) ;
#84652=CARTESIAN_POINT('Ctrl Pts',(-20.6058491698567,47.989470575133,123.261705399765)) ;
#84653=CARTESIAN_POINT('Ctrl Pts',(-20.6139152861985,47.9993650238883,123.469600664788)) ;
#84654=CARTESIAN_POINT('Ctrl Pts',(-20.5852299955288,48.0094281433228,123.679168568782)) ;
#84655=CARTESIAN_POINT('Ctrl Pts',(-20.522223787543,48.019267788564,123.876235991037)) ;
#84656=CARTESIAN_POINT('Ctrl Pts',(-20.4240386262326,48.0293309527501,124.063598469787)) ;
#84657=CARTESIAN_POINT('Ctrl Pts',(-20.2968105185812,48.0392252224989,124.228190134964)) ;
#84658=CARTESIAN_POINT('Ctrl Pts',(-20.1426174173993,48.0491669485127,124.369245419551)) ;
#84659=CARTESIAN_POINT('Ctrl Pts',(-19.9651875449329,48.0591698371721,124.482184152979)) ;
#84660=CARTESIAN_POINT('Ctrl Pts',(-19.7700259574284,48.0692096859661,124.562519679078)) ;
#84661=CARTESIAN_POINT('Ctrl Pts',(-19.5683733991087,48.0790339014269,124.607243543306)) ;
#84662=CARTESIAN_POINT('Ctrl Pts',(-19.3571780841245,48.0890907449205,124.616781601427)) ;
#84663=CARTESIAN_POINT('Ctrl Pts',(-19.1502186646684,48.0990193543165,124.589576537769)) ;
#84664=CARTESIAN_POINT('Ctrl Pts',(-18.9504848243982,48.1089712383544,124.527263966995)) ;
#84665=CARTESIAN_POINT('Ctrl Pts',(-18.7629118785965,48.119024191162,124.429914062262)) ;
#84666=CARTESIAN_POINT('Ctrl Pts',(-18.5986752513259,48.1288470676282,124.304701794279)) ;
#84667=CARTESIAN_POINT('Ctrl Pts',(-18.4551028259504,48.1389028001983,124.149549504682)) ;
#84668=CARTESIAN_POINT('Ctrl Pts',(-18.3422586437204,48.148843565186,123.973638765055)) ;
#84669=CARTESIAN_POINT('Ctrl Pts',(-18.2613684519812,48.1587478980916,123.781768982557)) ;
#84670=CARTESIAN_POINT('Ctrl Pts',(-18.2144911981124,48.1687945669723,123.575842264722)) ;
#84671=CARTESIAN_POINT('Ctrl Pts',(-18.2040462151921,48.1786901302781,123.368035261619)) ;
#84672=CARTESIAN_POINT('Ctrl Pts',(-18.2302679712022,48.1887521879784,123.158160931143)) ;
#84673=CARTESIAN_POINT('Ctrl Pts',(-18.2910782469109,48.1985949656059,122.960347491377)) ;
#84674=CARTESIAN_POINT('Ctrl Pts',(-18.3862593780217,48.2085854438577,122.773151847488)) ;
#84675=CARTESIAN_POINT('Ctrl Pts',(-18.5117691377216,48.2185144165013,122.606345569241)) ;
#84676=CARTESIAN_POINT('Ctrl Pts',(-18.6650588076118,48.2285055533808,122.462742642378)) ;
#84677=CARTESIAN_POINT('Ctrl Pts',(-18.8416404902588,48.2385276708698,122.347792998566)) ;
#84678=CARTESIAN_POINT('Ctrl Pts',(-19.0330683521124,48.248428181272,122.266070937534)) ;
#84679=CARTESIAN_POINT('Ctrl Pts',(-19.2375119544187,48.2584171740181,122.218087239322)) ;
#84680=CARTESIAN_POINT('Ctrl Pts',(-19.4466837042948,48.2683824180687,122.206504347386)) ;
#84681=CARTESIAN_POINT('Ctrl Pts',(-19.653498629586,48.2782866825819,122.230779258632)) ;
#84682=CARTESIAN_POINT('Ctrl Pts',(-19.8559842562716,48.2883447742801,122.291642965385)) ;
#84683=CARTESIAN_POINT('Ctrl Pts',(-20.0410138891386,48.2981947147085,122.384646494879)) ;
#84684=CARTESIAN_POINT('Ctrl Pts',(-20.2103684268925,48.308221725882,122.510161016601)) ;
#84685=CARTESIAN_POINT('Ctrl Pts',(-20.3549894371285,48.3182503124941,122.663586480818)) ;
#84686=CARTESIAN_POINT('Ctrl Pts',(-20.4689725657444,48.3280955266068,122.836337103123)) ;
#84687=CARTESIAN_POINT('Ctrl Pts',(-20.552967115562,48.3380862747864,123.028853190084)) ;
#84688=CARTESIAN_POINT('Ctrl Pts',(-20.6020368136756,48.3481239083719,123.234091529741)) ;
#84689=CARTESIAN_POINT('Ctrl Pts',(-20.6148256880223,48.3579691975847,123.440677314626)) ;
#84690=CARTESIAN_POINT('Ctrl Pts',(-20.591694430975,48.3679505983906,123.649222812979)) ;
#84691=CARTESIAN_POINT('Ctrl Pts',(-20.5328217842057,48.3779028313805,123.850002497856)) ;
#84692=CARTESIAN_POINT('Ctrl Pts',(-20.4397876862182,48.3879016428371,124.038518382421)) ;
#84693=CARTESIAN_POINT('Ctrl Pts',(-20.314622824821,48.3979407467678,124.208436648988)) ;
#84694=CARTESIAN_POINT('Ctrl Pts',(-20.1654041702261,48.4077656891871,124.351272582354)) ;
#84695=CARTESIAN_POINT('Ctrl Pts',(-19.9898488299125,48.4178203766631,124.468988144029)) ;
#84696=CARTESIAN_POINT('Ctrl Pts',(-19.7985107535511,48.4277631790199,124.55316317497)) ;
#84697=CARTESIAN_POINT('Ctrl Pts',(-19.5964148607437,48.4376669749596,124.603261723256)) ;
#84698=CARTESIAN_POINT('Ctrl Pts',(-19.3857034827114,48.4477137543347,124.617586751126)) ;
#84699=CARTESIAN_POINT('Ctrl Pts',(-19.1787979364258,48.4576094126293,124.595621172365)) ;
#84700=CARTESIAN_POINT('Ctrl Pts',(-18.975541301345,48.4676709798799,124.537136964074)) ;
#84701=CARTESIAN_POINT('Ctrl Pts',(-18.7895837084427,48.4775156243172,124.446269114341)) ;
#84702=CARTESIAN_POINT('Ctrl Pts',(-18.6198326405228,48.4874756705599,124.323679623546)) ;
#84703=CARTESIAN_POINT('Ctrl Pts',(-18.4731016776164,48.4975139665783,124.172014555145)) ;
#84704=CARTESIAN_POINT('Ctrl Pts',(-18.3565226797059,48.5073873079966,124.000238817597)) ;
#84705=CARTESIAN_POINT('Ctrl Pts',(-18.2699091400072,48.5174604117959,123.807037640738)) ;
#84706=CARTESIAN_POINT('Ctrl Pts',(-18.2191835073536,48.5272812269148,123.606859946643)) ;
#84707=CARTESIAN_POINT('Ctrl Pts',(-18.2033538660541,48.5373580919928,123.395643623774)) ;
#84708=CARTESIAN_POINT('Ctrl Pts',(-18.2240803976646,48.547222831648,123.189269074831)) ;
#84709=CARTESIAN_POINT('Ctrl Pts',(-18.2806840950281,48.5572452348894,122.986320575425)) ;
#84710=CARTESIAN_POINT('Ctrl Pts',(-18.372181360659,48.5672709591779,122.796429427149)) ;
#84711=CARTESIAN_POINT('Ctrl Pts',(-18.4928501657698,48.5771257421992,122.628035078555)) ;
#84712=CARTESIAN_POINT('Ctrl Pts',(-18.6424187453956,48.5871045859224,122.480923741899)) ;
#84713=CARTESIAN_POINT('Ctrl Pts',(-18.8161460063999,48.5971234781591,122.361848181127)) ;
#84714=CARTESIAN_POINT('Ctrl Pts',(-19.005167762733,48.6070066872001,122.275518623979)) ;
#84715=CARTESIAN_POINT('Ctrl Pts',(-19.2100373399335,48.6170749965403,122.222445396054)) ;
#84716=CARTESIAN_POINT('Ctrl Pts',(-19.4160689419314,48.626905121873,122.205898319748)) ;
#84717=CARTESIAN_POINT('Ctrl Pts',(-19.6267500732107,48.63697167425,122.225565271417)) ;
#84718=CARTESIAN_POINT('Ctrl Pts',(-19.827264205147,48.6468619111437,122.280674205092)) ;
#84719=CARTESIAN_POINT('Ctrl Pts',(-20.0172632939002,48.6568541359377,122.370249356566)) ;
#84720=CARTESIAN_POINT('Ctrl Pts',(-20.1882096971853,48.6668167562886,122.491258777972)) ;
#84721=CARTESIAN_POINT('Ctrl Pts',(-20.3350743946117,48.6767217590518,122.638900209885)) ;
#84722=CARTESIAN_POINT('Ctrl Pts',(-20.4557702176987,48.6867795214499,122.812492107969)) ;
#84723=CARTESIAN_POINT('Ctrl Pts',(-20.5428321318592,48.6966300408287,123.000408249078)) ;
#84724=CARTESIAN_POINT('Ctrl Pts',(-20.5973596016546,48.7066616178269,123.204118638861)) ;
#84725=CARTESIAN_POINT('Ctrl Pts',(-20.6152472704221,48.7166713529318,123.413816470762)) ;
#84726=CARTESIAN_POINT('Ctrl Pts',(-20.596827642037,48.7265809295581,123.621312650826)) ;
#84727=CARTESIAN_POINT('Ctrl Pts',(-20.5430718776097,48.7365083154147,123.822985220348)) ;
#84728=CARTESIAN_POINT('Ctrl Pts',(-20.4539262829434,48.746553249905,124.014413117639)) ;
#84729=CARTESIAN_POINT('Ctrl Pts',(-20.3349016053117,48.756439182093,124.184803478514)) ;
#84730=CARTESIAN_POINT('Ctrl Pts',(-20.1867787456366,48.766432488046,124.333775750932)) ;
#84731=CARTESIAN_POINT('Ctrl Pts',(-20.0158011499558,48.7763781258279,124.454128865026)) ;
#84732=CARTESIAN_POINT('Ctrl Pts',(-19.8266660386154,48.7863253941738,124.543373159768)) ;
#84733=CARTESIAN_POINT('Ctrl Pts',(-19.6228207603563,48.7963732963109,124.598744958645)) ;
#84734=CARTESIAN_POINT('Ctrl Pts',(-19.4166583359961,48.8062209911511,124.617674236778)) ;
#84735=CARTESIAN_POINT('Ctrl Pts',(-19.2079107140701,48.8161825008955,124.600980619408)) ;
#84736=CARTESIAN_POINT('Ctrl Pts',(-19.0039065477696,48.8262118925043,124.547658863247)) ;
#84737=CARTESIAN_POINT('Ctrl Pts',(-18.8145476302912,48.8361193880591,124.460899954782)) ;
#84738=CARTESIAN_POINT('Ctrl Pts',(-18.6422518271585,48.8460647797221,124.342481564474)) ;
#84739=CARTESIAN_POINT('Ctrl Pts',(-18.4921671250518,48.8560666973195,124.195169722798)) ;
#84740=CARTESIAN_POINT('Ctrl Pts',(-18.3698192760209,48.8661067648717,124.023195652858)) ;
#84741=CARTESIAN_POINT('Ctrl Pts',(-18.2806985265947,48.8759310763115,123.836856177689)) ;
#84742=CARTESIAN_POINT('Ctrl Pts',(-18.2237077358343,48.8859873174676,123.633290201079)) ;
#84743=CARTESIAN_POINT('Ctrl Pts',(-18.2034272663934,48.8959182392032,123.425474801886)) ;
#84744=CARTESIAN_POINT('Ctrl Pts',(-18.2191289139483,48.9058614752794,123.217054132415)) ;
#84745=CARTESIAN_POINT('Ctrl Pts',(-18.2707970023579,48.9158427592919,123.013643957691)) ;
#84746=CARTESIAN_POINT('Ctrl Pts',(-18.3578513256861,48.9258870609176,122.821289635891)) ;
#84747=CARTESIAN_POINT('Ctrl Pts',(-18.4740534699962,48.935715142137,122.650406878368)) ;
#84748=CARTESIAN_POINT('Ctrl Pts',(-18.621678191689,48.9457917449862,122.498533628722)) ;
#84749=CARTESIAN_POINT('Ctrl Pts',(-18.7896140891355,48.9556438241047,122.377226241393)) ;
#84750=CARTESIAN_POINT('Ctrl Pts',(-18.9800970457834,48.9657170824136,122.284765868234)) ;
#84751=CARTESIAN_POINT('Ctrl Pts',(-19.1791159230783,48.9755585417939,122.228160557319)) ;
#84752=CARTESIAN_POINT('Ctrl Pts',(-19.3873388554528,48.9855196372063,122.205934289294)) ;
#84753=CARTESIAN_POINT('Ctrl Pts',(-19.5978306689872,48.995556921603,122.220722311465)) ;
#84754=CARTESIAN_POINT('Ctrl Pts',(-19.7993884804198,49.0054332603383,122.270668665904)) ;
#84755=CARTESIAN_POINT('Ctrl Pts',(-19.992754216528,49.0154953864916,122.356380838616)) ;
#84756=CARTESIAN_POINT('Ctrl Pts',(-20.1649869075803,49.0253635604681,122.472078092719)) ;
#84757=CARTESIAN_POINT('Ctrl Pts',(-20.3168522787746,49.0353691089719,122.617582456607)) ;
#84758=CARTESIAN_POINT('Ctrl Pts',(-20.4408428299329,49.0453517408675,122.786952869297)) ;
#84759=CARTESIAN_POINT('Ctrl Pts',(-20.5338891114472,49.0553956832892,122.976482688953)) ;
#84760=CARTESIAN_POINT('Ctrl Pts',(-20.5916223966733,49.0652238313164,123.174870972758)) ;
#84761=CARTESIAN_POINT('Ctrl Pts',(-20.6150709603759,49.0752136986908,123.38357704141)) ;
#84762=CARTESIAN_POINT('Ctrl Pts',(-20.6013063782785,49.0852574376463,123.594278915098)) ;
#84763=CARTESIAN_POINT('Ctrl Pts',(-20.5526930823634,49.0950791861842,123.79495727049)) ;
#84764=CARTESIAN_POINT('Ctrl Pts',(-20.4686518773646,49.105114163794,123.988462046128)) ;
#84765=CARTESIAN_POINT('Ctrl Pts',(-20.3519125739174,49.1151390765517,124.163938848035)) ;
#84766=CARTESIAN_POINT('Ctrl Pts',(-20.2093168597284,49.1249910196455,124.314159557755)) ;
#84767=CARTESIAN_POINT('Ctrl Pts',(-20.0406693363286,49.1349819809746,124.439317919305)) ;
#84768=CARTESIAN_POINT('Ctrl Pts',(-19.854241583189,49.1448998558431,124.532750813393)) ;
#84769=CARTESIAN_POINT('Ctrl Pts',(-19.6522481376843,49.1549283748443,124.593089435573)) ;
#84770=CARTESIAN_POINT('Ctrl Pts',(-19.4458571981503,49.1648120536421,124.617196619252)) ;
#84771=CARTESIAN_POINT('Ctrl Pts',(-19.2360620898884,49.1748069970819,124.605427828753)) ;
#84772=CARTESIAN_POINT('Ctrl Pts',(-19.0309256506428,49.1848338509043,124.556904560052)) ;
#84773=CARTESIAN_POINT('Ctrl Pts',(-18.8399656511367,49.1947180152432,124.474946591072)) ;
#84774=CARTESIAN_POINT('Ctrl Pts',(-18.664180747488,49.2047061132856,124.360128702838)) ;
#84775=CARTESIAN_POINT('Ctrl Pts',(-18.5114556865831,49.2146572197427,124.217117734899)) ;
#84776=CARTESIAN_POINT('Ctrl Pts',(-18.3848137951546,49.2247022709108,124.048141099064)) ;
#84777=CARTESIAN_POINT('Ctrl Pts',(-18.291067478107,49.2345640312691,123.863220173348)) ;
#84778=CARTESIAN_POINT('Ctrl Pts',(-18.2296182846069,49.2445268480995,123.662986260319)) ;
#84779=CARTESIAN_POINT('Ctrl Pts',(-18.2040446119018,49.2545615293803,123.453590802208)) ;
#84780=CARTESIAN_POINT('Ctrl Pts',(-18.2146977103563,49.2644465591611,123.246021049742)) ;
#84781=CARTESIAN_POINT('Ctrl Pts',(-18.2621126124949,49.274512152559,123.039825967864)) ;
#84782=CARTESIAN_POINT('Ctrl Pts',(-18.3425873172727,49.2843513209205,122.849236798402)) ;
#84783=CARTESIAN_POINT('Ctrl Pts',(-18.4572075820245,49.294413918662,122.67146142508)) ;
#84784=CARTESIAN_POINT('Ctrl Pts',(-18.5987775243,49.304310931069,122.518966636729)) ;
#84785=CARTESIAN_POINT('Ctrl Pts',(-18.7648162010161,49.3142422528946,122.392390628733)) ;
#84786=CARTESIAN_POINT('Ctrl Pts',(-18.952480025907,49.3242840156491,122.295703968439)) ;
#84787=CARTESIAN_POINT('Ctrl Pts',(-19.1509683025373,49.3341722145398,122.233882221204)) ;
#84788=CARTESIAN_POINT('Ctrl Pts',(-19.3593098400291,49.3441661531396,122.206854423686)) ;
#84789=CARTESIAN_POINT('Ctrl Pts',(-19.5680935725974,49.3541069741765,122.216376406783)) ;
#84790=CARTESIAN_POINT('Ctrl Pts',(-19.77246713365,49.3640663564647,122.261825261247)) ;
#84791=CARTESIAN_POINT('Ctrl Pts',(-19.9666684170184,49.3740641161171,122.342274287404)) ;
#84792=CARTESIAN_POINT('Ctrl Pts',(-20.1444533728029,49.3841002523194,122.455885738796)) ;
#84793=CARTESIAN_POINT('Ctrl Pts',(-20.2971096658251,49.3939510498103,122.595827064741)) ;
#84794=CARTESIAN_POINT('Ctrl Pts',(-20.4250477465985,49.4039119148866,122.761600407615)) ;
#84795=CARTESIAN_POINT('Ctrl Pts',(-20.5227053010492,49.413940782517,122.948471659109)) ;
#84796=CARTESIAN_POINT('Ctrl Pts',(-20.5857337882693,49.4238510186534,123.147044510219)) ;
#84797=CARTESIAN_POINT('Ctrl Pts',(-20.6139392662548,49.4337859719679,123.354001283637)) ;
#84798=CARTESIAN_POINT('Ctrl Pts',(-20.6055025813455,49.4438269023775,123.56491960417)) ;
#84799=CARTESIAN_POINT('Ctrl Pts',(-20.5613836249676,49.4537147991591,123.768066893831)) ;
#84800=CARTESIAN_POINT('Ctrl Pts',(-20.4822199801657,49.4637042508178,123.962579565154)) ;
#84801=CARTESIAN_POINT('Ctrl Pts',(-20.3706836503675,49.4736633411831,124.139761384585)) ;
#84802=CARTESIAN_POINT('Ctrl Pts',(-20.2313302611011,49.4835606534894,124.29429460168)) ;
#84803=CARTESIAN_POINT('Ctrl Pts',(-20.0645865632603,49.4936170793897,124.42424335629)) ;
#84804=CARTESIAN_POINT('Ctrl Pts',(-19.8812921299888,49.5034870819794,124.521540983639)) ;
#84805=CARTESIAN_POINT('Ctrl Pts',(-19.681378547272,49.5134910151567,124.586788973033)) ;
#84806=CARTESIAN_POINT('Ctrl Pts',(-19.4734493643751,49.5234782756206,124.616182758674)) ;
#84807=CARTESIAN_POINT('Ctrl Pts',(-19.2627909875329,49.5335053272063,124.608876433656)) ;
#84808=CARTESIAN_POINT('Ctrl Pts',(-19.0593249390386,49.5433964170324,124.565892080854)) ;
#84809=CARTESIAN_POINT('Ctrl Pts',(-18.799884789262,49.5566941718134,124.461822818187)) ;
#84810=CARTESIAN_POINT('Ctrl Pts',(-18.5749111535208,49.5698922314216,124.293969511799)) ;
#84811=CARTESIAN_POINT('Ctrl Pts',(-18.4005901141605,49.5832889719908,124.072839422484)) ;
#84812=CARTESIAN_POINT('Ctrl Pts',(-18.3021399347806,49.5931598840642,123.890105721718)) ;
#84813=CARTESIAN_POINT('Ctrl Pts',(-18.2356163079452,49.6032334458323,123.689098930403)) ;
#84814=CARTESIAN_POINT('Ctrl Pts',(-18.2055086116115,49.6130548584207,123.484778378006)) ;
#84815=CARTESIAN_POINT('Ctrl Pts',(-18.2112827916809,49.6231288756517,123.273123424791)) ;
#84816=CARTESIAN_POINT('Ctrl Pts',(-18.2665397113971,49.6362876626163,123.001992298951)) ;
#84817=CARTESIAN_POINT('Ctrl Pts',(-18.392790369239,49.6496537657104,122.747437472296)) ;
#84818=CARTESIAN_POINT('Ctrl Pts',(-18.5783672784974,49.6629677005995,122.537851142176)) ;
#84819=CARTESIAN_POINT('Ctrl Pts',(-18.7409926332398,49.672867740047,122.407995171193)) ;
#84820=CARTESIAN_POINT('Ctrl Pts',(-18.9247419738745,49.6828321431815,122.307378326656)) ;
#84821=CARTESIAN_POINT('Ctrl Pts',(-19.1245307678255,49.6928621103026,122.239933892101)) ;
#84822=CARTESIAN_POINT('Ctrl Pts',(-19.3303117175903,49.7027643869117,122.208520852537)) ;
#84823=CARTESIAN_POINT('Ctrl Pts',(-19.6091931851167,49.7160303160808,122.21423648019)) ;
#84824=CARTESIAN_POINT('Ctrl Pts',(-19.9485295576993,49.7326518471873,122.312721939524)) ;
#84825=CARTESIAN_POINT('Ctrl Pts',(-20.2902094160068,49.7525266758319,122.561479387571)) ;
#84826=CARTESIAN_POINT('Ctrl Pts',(-20.4884697069658,49.7691998839338,122.855392710273)) ;
#84827=CARTESIAN_POINT('Ctrl Pts',(-20.5789967303349,49.7824510089151,123.118823468172)) ;
#84828=CARTESIAN_POINT('Ctrl Pts',(-20.6234021150388,49.7956933277359,123.393723395703)) ;
#84829=CARTESIAN_POINT('Ctrl Pts',(-20.5867774609634,49.8124265680754,123.747547976554)) ;
#84830=CARTESIAN_POINT('Ctrl Pts',(-20.4028093076993,49.8322557162633,124.127010811538)) ;
#84831=CARTESIAN_POINT('Ctrl Pts',(-20.0997798926132,49.852180411364,124.42294390878)) ;
#84832=CARTESIAN_POINT('Ctrl Pts',(-19.7138203126562,49.8721036399474,124.597719619346)) ;
#84833=CARTESIAN_POINT('Ctrl Pts',(-19.2914296712832,49.8920307790735,124.630422663148)) ;
#84834=CARTESIAN_POINT('Ctrl Pts',(-18.8840520052967,49.9119072416892,124.517817536054)) ;
#84835=CARTESIAN_POINT('Ctrl Pts',(-18.5377036256357,49.9318844702945,124.27191551634)) ;
#84836=CARTESIAN_POINT('Ctrl Pts',(-18.2968245024389,49.9518193282682,123.923098282419)) ;
#84837=CARTESIAN_POINT('Ctrl Pts',(-18.189244149917,49.971715777199,123.513986183938)) ;
#84838=CARTESIAN_POINT('Ctrl Pts',(-18.2273108184386,49.9916370612656,123.092101326508)) ;
#84839=CARTESIAN_POINT('Ctrl Pts',(-18.4075015764664,50.0115937109365,122.707903617813)) ;
#84840=CARTESIAN_POINT('Ctrl Pts',(-18.7066393081926,50.0314710040481,122.409408094434)) ;
#84841=CARTESIAN_POINT('Ctrl Pts',(-19.0894747132605,50.0513574762766,122.229768593168)) ;
#84842=CARTESIAN_POINT('Ctrl Pts',(-19.5143647079176,50.0714190422006,122.191861118502)) ;
#84843=CARTESIAN_POINT('Ctrl Pts',(-19.9220057248458,50.0912594497413,122.300397245321)) ;
#84844=CARTESIAN_POINT('Ctrl Pts',(-20.269364749244,50.1111107737143,122.540224979063)) ;
#84845=CARTESIAN_POINT('Ctrl Pts',(-20.5159525618895,50.1311640436657,122.888006920519)) ;
#84846=CARTESIAN_POINT('Ctrl Pts',(-20.6278796826559,50.150984701049,123.294433905217)) ;
#84847=CARTESIAN_POINT('Ctrl Pts',(-20.5948465512445,50.1709561223796,123.71765363184)) ;
#84848=CARTESIAN_POINT('Ctrl Pts',(-20.4200332314794,50.1908496147432,124.10299591866)) ;
#84849=CARTESIAN_POINT('Ctrl Pts',(-20.1222394668476,50.2108737009843,124.407164798566)) ;
#84850=CARTESIAN_POINT('Ctrl Pts',(-19.7427028446322,50.2306785800972,124.589700978199)) ;
#84851=CARTESIAN_POINT('Ctrl Pts',(-19.3205721862812,50.2506375957951,124.633229805539)) ;
#84852=CARTESIAN_POINT('Ctrl Pts',(-18.9086034727282,50.2706236194241,124.528993219994)) ;
#84853=CARTESIAN_POINT('Ctrl Pts',(-18.5595577971267,50.2904321151846,124.293209206143)) ;
#84854=CARTESIAN_POINT('Ctrl Pts',(-18.3093968949596,50.3104147542902,123.949887481206)) ;
#84855=CARTESIAN_POINT('Ctrl Pts',(-18.1920567395981,50.3302962020842,123.543654845403)) ;
#84856=CARTESIAN_POINT('Ctrl Pts',(-18.2201436547661,50.3502526688217,123.120348131323)) ;
#84857=CARTESIAN_POINT('Ctrl Pts',(-18.3901205711742,50.3701300657773,122.733311899486)) ;
#84858=CARTESIAN_POINT('Ctrl Pts',(-18.6832550770662,50.3901120119526,122.425821701632)) ;
#84859=CARTESIAN_POINT('Ctrl Pts',(-19.0629300478071,50.4100411109893,122.237453775053)) ;
#84860=CARTESIAN_POINT('Ctrl Pts',(-19.4839074313654,50.429969734202,122.18990649363)) ;
#84861=CARTESIAN_POINT('Ctrl Pts',(-19.8941981218103,50.4498040583084,122.287670822097)) ;
#84862=CARTESIAN_POINT('Ctrl Pts',(-20.1900713511371,50.4664563456918,122.481987303005)) ;
#84863=CARTESIAN_POINT('Ctrl Pts',(-20.3755130654345,50.479716846714,122.690239021733)) ;
#84864=CARTESIAN_POINT('Ctrl Pts',(-20.4862810393611,50.4897183239153,122.8689492502)) ;
#84865=CARTESIAN_POINT('Ctrl Pts',(-20.5642531757108,50.4997503447748,123.064919125253)) ;
#84866=CARTESIAN_POINT('Ctrl Pts',(-20.6065416927143,50.5096138885003,123.267915656053)) ;
#84867=CARTESIAN_POINT('Ctrl Pts',(-20.6135616619196,50.5195826021705,123.47738461801)) ;
#84868=CARTESIAN_POINT('Ctrl Pts',(-20.5737480165566,50.5329283495742,123.755049799615)) ;
#84869=CARTESIAN_POINT('Ctrl Pts',(-20.4644112173549,50.5460789046468,124.01246056538)) ;
#84870=CARTESIAN_POINT('Ctrl Pts',(-20.2913080349741,50.5594642851967,124.234313475355)) ;
#84871=CARTESIAN_POINT('Ctrl Pts',(-20.136897698789,50.5693522211896,124.373521055531)) ;
#84872=CARTESIAN_POINT('Ctrl Pts',(-19.9590515618089,50.5793434110022,124.485228977949)) ;
#84873=CARTESIAN_POINT('Ctrl Pts',(-19.7652513978111,50.5892955095405,124.564155971045)) ;
#84874=CARTESIAN_POINT('Ctrl Pts',(-19.5587718390512,50.599341765991,124.608506610613)) ;
#84875=CARTESIAN_POINT('Ctrl Pts',(-19.3518494007043,50.6091912133851,124.616330381746)) ;
#84876=CARTESIAN_POINT('Ctrl Pts',(-19.144275513289,50.6191538658803,124.588436795362)) ;
#84877=CARTESIAN_POINT('Ctrl Pts',(-18.9435668721036,50.6291769515224,124.524268876107)) ;
#84878=CARTESIAN_POINT('Ctrl Pts',(-18.758740003588,50.6391020672793,124.427384612171)) ;
#84879=CARTESIAN_POINT('Ctrl Pts',(-18.5915092232509,50.6491545456791,124.298203194396)) ;
#84880=CARTESIAN_POINT('Ctrl Pts',(-18.4519664488922,50.6590060443818,124.145139257447)) ;
#84881=CARTESIAN_POINT('Ctrl Pts',(-18.3393284230792,50.6689777835844,123.968364363511)) ;
#84882=CARTESIAN_POINT('Ctrl Pts',(-18.2589073168524,50.6789729913501,123.774195216805)) ;
#84883=CARTESIAN_POINT('Ctrl Pts',(-18.2135079778918,50.6890069928191,123.568211141614)) ;
#84884=CARTESIAN_POINT('Ctrl Pts',(-18.2043916883253,50.6988623509115,123.361200369958)) ;
#84885=CARTESIAN_POINT('Ctrl Pts',(-18.2314639870011,50.7088618265048,123.152768262259)) ;
#84886=CARTESIAN_POINT('Ctrl Pts',(-18.2934523109721,50.7187562749999,122.954165767823)) ;
#84887=CARTESIAN_POINT('Ctrl Pts',(-18.3906320047257,50.7288193992276,122.766288923649)) ;
#84888=CARTESIAN_POINT('Ctrl Pts',(-18.515967951093,50.7386590255562,122.601680143843)) ;
#84889=CARTESIAN_POINT('Ctrl Pts',(-18.671206799712,50.7487222605992,122.457990491376)) ;
#84890=CARTESIAN_POINT('Ctrl Pts',(-18.8461841647024,50.7586162658332,122.345485242714)) ;
#84891=CARTESIAN_POINT('Ctrl Pts',(-19.0387184734415,50.768558979049,122.264163925914)) ;
#84892=CARTESIAN_POINT('Ctrl Pts',(-19.2437750813141,50.7785647188472,122.217162069722)) ;
#84893=CARTESIAN_POINT('Ctrl Pts',(-19.454181494152,50.7885856209936,122.206701103383)) ;
#84894=CARTESIAN_POINT('Ctrl Pts',(-19.66053430919,50.7984763910424,122.232355977739)) ;
#84895=CARTESIAN_POINT('Ctrl Pts',(-19.8613997985619,50.8084678018222,122.293768556927)) ;
#84896=CARTESIAN_POINT('Ctrl Pts',(-20.0477153832223,50.8184161474867,122.388776879898)) ;
#84897=CARTESIAN_POINT('Ctrl Pts',(-20.2149291809395,50.8283610055478,122.514309604095)) ;
#84898=CARTESIAN_POINT('Ctrl Pts',(-20.3591331058569,50.8384158409408,122.668841760372)) ;
#84899=CARTESIAN_POINT('Ctrl Pts',(-20.4719728911623,50.8482382130423,122.841803139184)) ;
#84900=CARTESIAN_POINT('Ctrl Pts',(-20.555331401532,50.858294080486,123.036064303744)) ;
#84901=CARTESIAN_POINT('Ctrl Pts',(-20.6027823192798,50.8682348103439,123.23959968748)) ;
#84902=CARTESIAN_POINT('Ctrl Pts',(-20.6147815729296,50.878139148895,123.44747770564)) ;
#84903=CARTESIAN_POINT('Ctrl Pts',(-20.5900240767088,50.8881858303235,123.657216643882)) ;
#84904=CARTESIAN_POINT('Ctrl Pts',(-20.5303079529691,50.8980813377928,123.856531746283)) ;
#84905=CARTESIAN_POINT('Ctrl Pts',(-20.4353433394466,50.9081436062914,124.045523747935)) ;
#84906=CARTESIAN_POINT('Ctrl Pts',(-20.3118409988346,50.917985596562,124.21156392592)) ;
#84907=CARTESIAN_POINT('Ctrl Pts',(-20.1594362435033,50.9279790134429,124.356126658546)) ;
#84908=CARTESIAN_POINT('Ctrl Pts',(-19.9854190300829,50.9379035012951,124.471276812575)) ;
#84909=CARTESIAN_POINT('Ctrl Pts',(-19.7927265192482,50.9479031352036,124.55527997658)) ;
#84910=CARTESIAN_POINT('Ctrl Pts',(-19.5886058865393,50.9578892454603,124.60450108156)) ;
#84911=CARTESIAN_POINT('Ctrl Pts',(-19.3780314592793,50.9679251966475,124.61737349996)) ;
#84912=CARTESIAN_POINT('Ctrl Pts',(-19.1720910866892,50.9777818349823,124.594220179101)) ;
#84913=CARTESIAN_POINT('Ctrl Pts',(-18.9704025499293,50.9877807950603,124.535105151428)) ;
#84914=CARTESIAN_POINT('Ctrl Pts',(-18.7838328347708,50.9976760253741,124.4430065962)) ;
#84915=CARTESIAN_POINT('Ctrl Pts',(-18.6133502426643,51.0077365378427,124.317874563771)) ;
#84916=CARTESIAN_POINT('Ctrl Pts',(-18.4701391587835,51.0175858293889,124.168301037552)) ;
#84917=CARTESIAN_POINT('Ctrl Pts',(-18.3525641864338,51.0276130153211,123.993338577093)) ;
#84918=CARTESIAN_POINT('Ctrl Pts',(-18.267643184674,51.0376415517804,123.80035451897)) ;
#84919=CARTESIAN_POINT('Ctrl Pts',(-18.218060405156,51.0474867917454,123.599415288978)) ;
#84920=CARTESIAN_POINT('Ctrl Pts',(-18.2033518857591,51.0574774866686,123.389889933825)) ;
#84921=CARTESIAN_POINT('Ctrl Pts',(-18.2258151202182,51.0675153074272,123.18006296061)) ;
#84922=CARTESIAN_POINT('Ctrl Pts',(-18.2829055891925,51.0773599012041,122.981124529681)) ;
#84923=CARTESIAN_POINT('Ctrl Pts',(-18.374543826743,51.0873438965802,122.792311132886)) ;
#84924=CARTESIAN_POINT('Ctrl Pts',(-18.497178925122,51.0972929451416,122.622862413352)) ;
#84925=CARTESIAN_POINT('Ctrl Pts',(-18.6480196169421,51.1072953841161,122.476338494011)) ;
#84926=CARTESIAN_POINT('Ctrl Pts',(-18.8224928721173,51.1173166254125,122.358249517239)) ;
#84927=CARTESIAN_POINT('Ctrl Pts',(-19.0122492011059,51.127209303852,122.273123769501)) ;
#84928=CARTESIAN_POINT('Ctrl Pts',(-19.2158038373338,51.1371993577996,122.221412219631)) ;
#84929=CARTESIAN_POINT('Ctrl Pts',(-19.4245865714748,51.1471577189481,122.206028609409)) ;
#84930=CARTESIAN_POINT('Ctrl Pts',(-19.6317117699765,51.1570573458329,122.226497827974)) ;
#84931=CARTESIAN_POINT('Ctrl Pts',(-19.8350849559763,51.1671052426363,122.283522987711)) ;
#84932=CARTESIAN_POINT('Ctrl Pts',(-20.022696372349,51.1770006002723,122.373481440644)) ;
#84933=CARTESIAN_POINT('Ctrl Pts',(-20.1946528304489,51.1870622527289,122.496627883948)) ;
#84934=CARTESIAN_POINT('Ctrl Pts',(-20.3394665608581,51.1969068570009,122.644499616688)) ;
#84935=CARTESIAN_POINT('Ctrl Pts',(-20.4583901002709,51.2068669786989,122.816839675595)) ;
#84936=CARTESIAN_POINT('Ctrl Pts',(-20.5458920206449,51.2169050130614,123.008866436735)) ;
#84937=CARTESIAN_POINT('Ctrl Pts',(-20.5982377519266,51.2267793256479,123.209773659771)) ;
#84938=CARTESIAN_POINT('Ctrl Pts',(-20.615219420683,51.2368488064306,123.420755084816)) ;
#84939=CARTESIAN_POINT('Ctrl Pts',(-20.5958818047259,51.2466831424477,123.626614553327)) ;
#84940=CARTESIAN_POINT('Ctrl Pts',(-20.5405510012675,51.2567161001759,123.830145681177)) ;
#84941=CARTESIAN_POINT('Ctrl Pts',(-20.4503035157272,51.2667364987511,124.020498806758)) ;
#84942=CARTESIAN_POINT('Ctrl Pts',(-20.3306797939829,51.2766020725223,124.189949471815)) ;
#84943=CARTESIAN_POINT('Ctrl Pts',(-20.1804458345177,51.2866709471784,124.339042785219)) ;
#84944=CARTESIAN_POINT('Ctrl Pts',(-20.0104561735626,51.2965163780839,124.457150465107)) ;
#84945=CARTESIAN_POINT('Ctrl Pts',(-19.8202797994579,51.3064960029546,124.545737849271)) ;
#84946=CARTESIAN_POINT('Ctrl Pts',(-19.616714022503,51.3165146858687,124.599784861309)) ;
#84947=CARTESIAN_POINT('Ctrl Pts',(-19.4096995310272,51.3263979510525,124.617864751251)) ;
#84948=CARTESIAN_POINT('Ctrl Pts',(-19.1988827452184,51.3364662451439,124.599299463664)) ;
#84949=CARTESIAN_POINT('Ctrl Pts',(-18.9991976018258,51.3462963753292,124.545926781667)) ;
#84950=CARTESIAN_POINT('Ctrl Pts',(-18.8072530956794,51.3563629235443,124.456872690114)) ;
#84951=CARTESIAN_POINT('Ctrl Pts',(-18.6367526325519,51.366253172233,124.337824103863)) ;
#84952=CARTESIAN_POINT('Ctrl Pts',(-18.4876976832283,51.376245354009,124.1898183886)) ;
#84953=CARTESIAN_POINT('Ctrl Pts',(-18.3671179776991,51.3862081346368,124.018565014349)) ;
#84954=CARTESIAN_POINT('Ctrl Pts',(-18.2781468980494,51.3961125393105,123.830292783191)) ;
#84955=CARTESIAN_POINT('Ctrl Pts',(-18.2225158405115,51.4061725337896,123.626267180242)) ;
#84956=CARTESIAN_POINT('Ctrl Pts',(-18.2033820488565,51.4160211557594,123.420089212083)) ;
#84957=CARTESIAN_POINT('Ctrl Pts',(-18.220176478215,51.4260515951712,123.209899707613)) ;
#84958=CARTESIAN_POINT('Ctrl Pts',(-18.2735217851603,51.436061310806,123.006313697817)) ;
#84959=CARTESIAN_POINT('Ctrl Pts',(-18.3603349962703,51.4459720634986,122.816927498495)) ;
#84960=CARTESIAN_POINT('Ctrl Pts',(-18.4785193359598,51.455901336445,122.644849590924)) ;
#84961=CARTESIAN_POINT('Ctrl Pts',(-18.6265725102153,51.4659440278377,122.494343311464)) ;
#84962=CARTESIAN_POINT('Ctrl Pts',(-18.7957733587672,51.4758305610552,122.373613107459)) ;
#84963=CARTESIAN_POINT('Ctrl Pts',(-18.9852153494115,51.4858237059872,122.282818770106)) ;
#84964=CARTESIAN_POINT('Ctrl Pts',(-19.1866163697418,51.4957693868237,122.226639312132)) ;
#84965=CARTESIAN_POINT('Ctrl Pts',(-19.3947137007887,51.5057166439722,122.205852968183)) ;
#84966=CARTESIAN_POINT('Ctrl Pts',(-19.6053345562994,51.5157645478442,122.221908810466)) ;
#84967=CARTESIAN_POINT('Ctrl Pts',(-19.8059405043631,51.5256122469422,122.273080725535)) ;
#84968=CARTESIAN_POINT('Ctrl Pts',(-19.9970579122772,51.5355737379209,122.358685508991)) ;
#84969=CARTESIAN_POINT('Ctrl Pts',(-20.1714467611568,51.5456032003348,122.477219168564)) ;
#84970=CARTESIAN_POINT('Ctrl Pts',(-20.3208357337139,51.5555104314347,122.62235338658)) ;
#84971=CARTESIAN_POINT('Ctrl Pts',(-20.4435745272734,51.5654568101121,122.791629667315)) ;
#84972=CARTESIAN_POINT('Ctrl Pts',(-20.5356748438808,51.575461578921,122.980744980658)) ;
#84973=CARTESIAN_POINT('Ctrl Pts',(-20.5933963675229,51.5854826999412,123.183354761338)) ;
#84974=CARTESIAN_POINT('Ctrl Pts',(-20.6150184502875,51.5953735657938,123.390171536173)) ;
#84975=CARTESIAN_POINT('Ctrl Pts',(-20.6005649524091,51.6053643745531,123.599699839258)) ;
#84976=CARTESIAN_POINT('Ctrl Pts',(-20.5501094987751,51.6153150327334,123.802728492899)) ;
#84977=CARTESIAN_POINT('Ctrl Pts',(-20.4655583773895,51.6252512423755,123.993724149889)) ;
#84978=CARTESIAN_POINT('Ctrl Pts',(-20.3487803568357,51.6352344091004,124.168144479374)) ;
#84979=CARTESIAN_POINT('Ctrl Pts',(-20.2023614827982,51.6452782063107,124.32025219371)) ;
#84980=CARTESIAN_POINT('Ctrl Pts',(-20.0356625555616,51.655106422479,124.442383564606)) ;
#84981=CARTESIAN_POINT('Ctrl Pts',(-19.8457170220924,51.6651829899482,124.536080304452)) ;
#84982=CARTESIAN_POINT('Ctrl Pts',(-19.6468633598627,51.6750350756376,124.594176636831)) ;
#84983=CARTESIAN_POINT('Ctrl Pts',(-19.4364191049559,51.685108343043,124.617542351253)) ;
#84984=CARTESIAN_POINT('Ctrl Pts',(-19.2299340144037,51.6949497594666,124.604264983939)) ;
#84985=CARTESIAN_POINT('Ctrl Pts',(-19.0262804084281,51.7049110176093,124.555507886137)) ;
#84986=CARTESIAN_POINT('Ctrl Pts',(-18.8328905076921,51.7149476940412,124.471123415834)) ;
#84987=CARTESIAN_POINT('Ctrl Pts',(-18.6596436603667,51.7248263019051,124.356557651577)) ;
#84988=CARTESIAN_POINT('Ctrl Pts',(-18.506152939823,51.7348865305439,124.211091737001)) ;
#84989=CARTESIAN_POINT('Ctrl Pts',(-18.3825894189891,51.7447535147047,124.044441759415)) ;
#84990=CARTESIAN_POINT('Ctrl Pts',(-18.288197260969,51.7547590809574,123.856492609393)) ;
#84991=CARTESIAN_POINT('Ctrl Pts',(-18.2280368454756,51.764742869372,123.655369944984)) ;
#84992=CARTESIAN_POINT('Ctrl Pts',(-18.2037955443594,51.7747887261746,123.44558720362)) ;
#84993=CARTESIAN_POINT('Ctrl Pts',(-18.2158049422002,51.7846146033906,123.239365703502)) ;
#84994=CARTESIAN_POINT('Ctrl Pts',(-18.2635681761334,51.7946050792319,123.034837434973)) ;
#84995=CARTESIAN_POINT('Ctrl Pts',(-18.3470677407397,51.8046486551307,122.840901092914)) ;
#84996=CARTESIAN_POINT('Ctrl Pts',(-18.460050036264,51.8144704474287,122.668070690443)) ;
#84997=CARTESIAN_POINT('Ctrl Pts',(-18.6040154321595,51.8245054130546,122.513860046172)) ;
#84998=CARTESIAN_POINT('Ctrl Pts',(-18.7727581101242,51.8345303299877,122.387582237159)) ;
#84999=CARTESIAN_POINT('Ctrl Pts',(-18.9574116325095,51.8443822683638,122.293758444843)) ;
#85000=CARTESIAN_POINT('Ctrl Pts',(-19.1582249159221,51.8543732443885,122.232272280437)) ;
#85001=CARTESIAN_POINT('Ctrl Pts',(-19.3651733728884,51.8642910651922,122.206630479533)) ;
#85002=CARTESIAN_POINT('Ctrl Pts',(-19.5757113303297,51.8743197857568,122.217393836154)) ;
#85003=CARTESIAN_POINT('Ctrl Pts',(-19.7782673536523,51.8842027123659,122.263734533123)) ;
#85004=CARTESIAN_POINT('Ctrl Pts',(-19.9721412663142,51.8942069974854,122.345208741606)) ;
#85005=CARTESIAN_POINT('Ctrl Pts',(-20.1485965825961,51.9041906786933,122.458925895138)) ;
#85006=CARTESIAN_POINT('Ctrl Pts',(-20.3033084600691,51.9142316774232,122.602515954827)) ;
#85007=CARTESIAN_POINT('Ctrl Pts',(-20.4283341936151,51.9240641222903,122.767130738101)) ;
#85008=CARTESIAN_POINT('Ctrl Pts',(-20.5249880230487,51.9340591207207,122.953701580357)) ;
#85009=CARTESIAN_POINT('Ctrl Pts',(-20.5875824491008,51.9440906694703,123.155104794156)) ;
#85010=CARTESIAN_POINT('Ctrl Pts',(-20.6140701866757,51.9539560477758,123.360796237962)) ;
#85011=CARTESIAN_POINT('Ctrl Pts',(-20.6049369884442,51.9639178952361,123.570032777721)) ;
#85012=CARTESIAN_POINT('Ctrl Pts',(-20.5589475425777,51.9739528360503,123.775913422753)) ;
#85013=CARTESIAN_POINT('Ctrl Pts',(-20.4794278314996,51.9838377970674,123.967942136483)) ;
#85014=CARTESIAN_POINT('Ctrl Pts',(-20.3657283845521,51.9939034059863,124.14637155563)) ;
#85015=CARTESIAN_POINT('Ctrl Pts',(-20.2260994155027,52.003742581028,124.299028744683)) ;
#85016=CARTESIAN_POINT('Ctrl Pts',(-20.0585850427289,52.0138051365279,124.428181893886)) ;
#85017=CARTESIAN_POINT('Ctrl Pts',(-19.874133546261,52.0237023112208,124.524491578189)) ;
#85018=CARTESIAN_POINT('Ctrl Pts',(-19.6753166357075,52.0336330261442,124.588188263668)) ;
#85019=CARTESIAN_POINT('Ctrl Pts',(-19.4660674265901,52.0436770542218,124.616477182065)) ;
#85020=CARTESIAN_POINT('Ctrl Pts',(-19.2583751604447,52.0535632560751,124.608298744114)) ;
#85021=CARTESIAN_POINT('Ctrl Pts',(-19.0530285450914,52.0635564225419,124.564023365578)) ;
#85022=CARTESIAN_POINT('Ctrl Pts',(-18.8594658865747,52.0734958935291,124.485230512348)) ;
#85023=CARTESIAN_POINT('Ctrl Pts',(-18.681171591748,52.0835124078833,124.373224330543)) ;
#85024=CARTESIAN_POINT('Ctrl Pts',(-18.5262256114229,52.0934424343601,124.233278642585)) ;
#85025=CARTESIAN_POINT('Ctrl Pts',(-18.3964520684742,52.1034949698696,124.066502860236)) ;
#85026=CARTESIAN_POINT('Ctrl Pts',(-18.2995181668881,52.1133413730892,123.883591053163)) ;
#85027=CARTESIAN_POINT('Ctrl Pts',(-18.2344303663657,52.1233034159433,123.684540728996)) ;
#85028=CARTESIAN_POINT('Ctrl Pts',(-18.2049633408895,52.133331966734,123.475764348543)) ;
#85029=CARTESIAN_POINT('Ctrl Pts',(-18.2120381030114,52.1432422924516,123.267547761259)) ;
#85030=CARTESIAN_POINT('Ctrl Pts',(-18.2547347149684,52.1531772042812,123.063088669452)) ;
#85031=CARTESIAN_POINT('Ctrl Pts',(-18.3332871503977,52.1632182110493,122.867161311579)) ;
#85032=CARTESIAN_POINT('Ctrl Pts',(-18.4428555005339,52.1731058438815,122.690501470127)) ;
#85033=CARTESIAN_POINT('Ctrl Pts',(-18.582582312004,52.1830962749795,122.533706157524)) ;
#85034=CARTESIAN_POINT('Ctrl Pts',(-18.7469172566811,52.1930517115367,122.404087576833)) ;
#85035=CARTESIAN_POINT('Ctrl Pts',(-18.9302412953445,52.2029626596361,122.305087020515)) ;
#85036=CARTESIAN_POINT('Ctrl Pts',(-19.1299410619868,52.2129747357338,122.238509440795)) ;
#85037=CARTESIAN_POINT('Ctrl Pts',(-19.3385091445612,52.2230020578087,122.207996703187)) ;
#85038=CARTESIAN_POINT('Ctrl Pts',(-19.5457346255432,52.2328608327629,122.213537169316)) ;
#85039=CARTESIAN_POINT('Ctrl Pts',(-19.8221907945134,52.2462870255753,122.270185645489)) ;
#85040=CARTESIAN_POINT('Ctrl Pts',(-20.0713994992223,52.2593710413567,122.394141575625)) ;
#85041=CARTESIAN_POINT('Ctrl Pts',(-20.2838395622631,52.272844490112,122.581345054792)) ;
#85042=CARTESIAN_POINT('Ctrl Pts',(-20.412650215348,52.2826774479178,122.743072361352)) ;
#85043=CARTESIAN_POINT('Ctrl Pts',(-20.5134840114003,52.2926407213685,122.926645543791)) ;
#85044=CARTESIAN_POINT('Ctrl Pts',(-20.5809847415257,52.3026777951864,123.126566369539)) ;
#85045=CARTESIAN_POINT('Ctrl Pts',(-20.6126263091998,52.3125527981981,123.331769600244)) ;
#85046=CARTESIAN_POINT('Ctrl Pts',(-20.6080629083535,52.3226204778243,123.543345637874)) ;
#85047=CARTESIAN_POINT('Ctrl Pts',(-20.567868291895,52.332461328042,123.746312988223)) ;
#85048=CARTESIAN_POINT('Ctrl Pts',(-20.4670269754835,52.345797526518,124.007905058879)) ;
#85049=CARTESIAN_POINT('Ctrl Pts',(-20.3015604237131,52.3590150503324,124.235140155152)) ;
#85050=CARTESIAN_POINT('Ctrl Pts',(-20.0837896410243,52.3723499768236,124.411582706571)) ;
#85051=CARTESIAN_POINT('Ctrl Pts',(-19.900255890719,52.3823330774182,124.513471532459)) ;
#85052=CARTESIAN_POINT('Ctrl Pts',(-19.7005525301672,52.3923778533179,124.582048554509)) ;
#85053=CARTESIAN_POINT('Ctrl Pts',(-19.496714380431,52.4021957765038,124.614579095384)) ;
#85054=CARTESIAN_POINT('Ctrl Pts',(-19.2854774970839,52.4122450904591,124.611577339329)) ;
#85055=CARTESIAN_POINT('Ctrl Pts',(-19.0108629775907,52.4255488310817,124.558542159798)) ;
#85056=CARTESIAN_POINT('Ctrl Pts',(-18.6949729851528,52.4420390265583,124.406311397953)) ;
#85057=CARTESIAN_POINT('Ctrl Pts',(-18.446743481216,52.458758191483,124.151888766635)) ;
#85058=CARTESIAN_POINT('Ctrl Pts',(-18.3113738894575,52.4719191851531,123.910570921189)) ;
#85059=CARTESIAN_POINT('Ctrl Pts',(-18.2412220343529,52.4819154072584,123.712480369397)) ;
#85060=CARTESIAN_POINT('Ctrl Pts',(-18.2069072499247,52.4919392467921,123.504562221584)) ;
#85061=CARTESIAN_POINT('Ctrl Pts',(-18.2093339290395,52.5051325687854,123.227174035408)) ;
#85062=CARTESIAN_POINT('Ctrl Pts',(-18.3035482233452,52.5217917405627,122.885761998308)) ;
#85063=CARTESIAN_POINT('Ctrl Pts',(-18.5490022666075,52.5417019160484,122.540816632851)) ;
#85064=CARTESIAN_POINT('Ctrl Pts',(-18.896602436041,52.5615919038928,122.299840270026)) ;
#85065=CARTESIAN_POINT('Ctrl Pts',(-19.3079252000315,52.5815973519076,122.191722541258)) ;
#85066=CARTESIAN_POINT('Ctrl Pts',(-19.7281008050595,52.6014337459349,122.229713440232)) ;
#85067=CARTESIAN_POINT('Ctrl Pts',(-20.1132537389157,52.6214415398316,122.410106061638)) ;
#85068=CARTESIAN_POINT('Ctrl Pts',(-20.4112472617472,52.6412681761255,122.708408581873)) ;
#85069=CARTESIAN_POINT('Ctrl Pts',(-20.591586675119,52.6612471190794,123.093018079891)) ;
#85070=CARTESIAN_POINT('Ctrl Pts',(-20.6290084966282,52.6811789209484,123.515109816037)) ;
#85071=CARTESIAN_POINT('Ctrl Pts',(-20.5220590950608,52.701003221446,123.922971129483)) ;
#85072=CARTESIAN_POINT('Ctrl Pts',(-20.2786176824893,52.7210992227858,124.273924750652)) ;
#85073=CARTESIAN_POINT('Ctrl Pts',(-19.9358039298988,52.7408576388898,124.51720323267)) ;
#85074=CARTESIAN_POINT('Ctrl Pts',(-19.5241772464082,52.7609513317739,124.630789979139)) ;
#85075=CARTESIAN_POINT('Ctrl Pts',(-19.2461498794551,52.7740622976805,124.608685688099)) ;
#85076=CARTESIAN_POINT('Ctrl Pts',(-19.1099523892177,52.7807756724684,124.573829556462)) ;
#85077=CARTESIAN_POINT('Ctrl Pts',(-20.8283360085486,11.7999200508426,122.926058340311)) ;
#85078=CARTESIAN_POINT('Ctrl Pts',(-20.8845464538574,11.8065469016607,123.090182099353)) ;
#85079=CARTESIAN_POINT('Ctrl Pts',(-20.9394674069342,11.8197775281417,123.437524293028)) ;
#85080=CARTESIAN_POINT('Ctrl Pts',(-20.8387914871724,11.8397531494004,123.958813977782)) ;
#85081=CARTESIAN_POINT('Ctrl Pts',(-20.5666784354472,11.8596704843023,124.412866308854)) ;
#85082=CARTESIAN_POINT('Ctrl Pts',(-20.1575619136445,11.8795437610183,124.747046208683)) ;
#85083=CARTESIAN_POINT('Ctrl Pts',(-19.6551371496748,11.8995682511823,124.92249916066)) ;
#85084=CARTESIAN_POINT('Ctrl Pts',(-19.1270451744641,11.919436092333,124.915907267661)) ;
#85085=CARTESIAN_POINT('Ctrl Pts',(-18.6308008607008,11.9393817432125,124.729592278927)) ;
#85086=CARTESIAN_POINT('Ctrl Pts',(-18.2288280457431,11.9592871438295,124.385624086374)) ;
#85087=CARTESIAN_POINT('Ctrl Pts',(-17.9678591535732,11.9791613716459,123.926365470291)) ;
#85088=CARTESIAN_POINT('Ctrl Pts',(-17.8787398474485,11.9991471625235,123.402691583813)) ;
#85089=CARTESIAN_POINT('Ctrl Pts',(-17.9735233382965,12.0190414051832,122.882536434516)) ;
#85090=CARTESIAN_POINT('Ctrl Pts',(-18.2387585289407,12.0389201212553,122.425519450945)) ;
#85091=CARTESIAN_POINT('Ctrl Pts',(-18.6476197278655,12.0589595710999,122.084275218605)) ;
#85092=CARTESIAN_POINT('Ctrl Pts',(-19.1441777499651,12.0788227326378,121.904537351317)) ;
#85093=CARTESIAN_POINT('Ctrl Pts',(-19.6750288445506,12.098802100652,121.904738156225)) ;
#85094=CARTESIAN_POINT('Ctrl Pts',(-20.1701856143784,12.1186126811748,122.084100255283)) ;
#85095=CARTESIAN_POINT('Ctrl Pts',(-20.5782317220315,12.1385936094604,122.423828694064)) ;
#85096=CARTESIAN_POINT('Ctrl Pts',(-20.8444525967082,12.1584862813298,122.880697423595)) ;
#85097=CARTESIAN_POINT('Ctrl Pts',(-20.9398398136422,12.1784126116169,123.401645628938)) ;
#85098=CARTESIAN_POINT('Ctrl Pts',(-20.851062860932,12.1983831657092,123.924943760388)) ;
#85099=CARTESIAN_POINT('Ctrl Pts',(-20.6345502730467,12.2149150047968,124.307289073383)) ;
#85100=CARTESIAN_POINT('Ctrl Pts',(-20.3891153931417,12.2282547436244,124.557618291671)) ;
#85101=CARTESIAN_POINT('Ctrl Pts',(-20.1744356948872,12.238286985843,124.71063155409)) ;
#85102=CARTESIAN_POINT('Ctrl Pts',(-19.9407461181023,12.2481446864865,124.82243808738)) ;
#85103=CARTESIAN_POINT('Ctrl Pts',(-19.6879479903912,12.2581365511257,124.893369098924)) ;
#85104=CARTESIAN_POINT('Ctrl Pts',(-19.4284766803744,12.2680591008858,124.919096784819)) ;
#85105=CARTESIAN_POINT('Ctrl Pts',(-19.0804161519456,12.2813368743793,124.893600455121)) ;
#85106=CARTESIAN_POINT('Ctrl Pts',(-18.7455915471493,12.2946842133199,124.776633305253)) ;
#85107=CARTESIAN_POINT('Ctrl Pts',(-18.4584578761078,12.3078914451131,124.581565716411)) ;
#85108=CARTESIAN_POINT('Ctrl Pts',(-18.2699644759195,12.3178785612028,124.39900581103)) ;
#85109=CARTESIAN_POINT('Ctrl Pts',(-18.1163990348321,12.3278294667826,124.187285865335)) ;
#85110=CARTESIAN_POINT('Ctrl Pts',(-18.0010402192528,12.33788456879,123.949600254045)) ;
#85111=CARTESIAN_POINT('Ctrl Pts',(-17.9299289800127,12.3477062421111,123.701455973458)) ;
#85112=CARTESIAN_POINT('Ctrl Pts',(-17.9019096964941,12.357764713186,123.438645136577)) ;
#85113=CARTESIAN_POINT('Ctrl Pts',(-17.9200603909808,12.3676893243625,123.178453886709)) ;
#85114=CARTESIAN_POINT('Ctrl Pts',(-18.0035385415921,12.3809666632629,122.839641054544)) ;
#85115=CARTESIAN_POINT('Ctrl Pts',(-18.1740845283454,12.3942655425005,122.530112925337)) ;
#85116=CARTESIAN_POINT('Ctrl Pts',(-18.4148347268114,12.4075044146712,122.278925757333)) ;
#85117=CARTESIAN_POINT('Ctrl Pts',(-18.626729428275,12.4175110328078,122.123187062121)) ;
#85118=CARTESIAN_POINT('Ctrl Pts',(-18.8632335737039,12.4275419778693,122.006787551109)) ;
#85119=CARTESIAN_POINT('Ctrl Pts',(-19.1118364896857,12.4373981512211,121.934037501767)) ;
#85120=CARTESIAN_POINT('Ctrl Pts',(-19.3729328187221,12.447397422184,121.904821743981)) ;
#85121=CARTESIAN_POINT('Ctrl Pts',(-19.6324990778504,12.4572918739413,121.920913539679)) ;
#85122=CARTESIAN_POINT('Ctrl Pts',(-19.8895297331301,12.4673551897507,121.982929816623)) ;
#85123=CARTESIAN_POINT('Ctrl Pts',(-20.1266869407979,12.4771940464903,122.086036295395)) ;
#85124=CARTESIAN_POINT('Ctrl Pts',(-20.3474074551281,12.4872601683079,122.231757371538)) ;
#85125=CARTESIAN_POINT('Ctrl Pts',(-20.5359559653956,12.4971433960322,122.410425895404)) ;
#85126=CARTESIAN_POINT('Ctrl Pts',(-20.6927050538892,12.5071328573109,122.620969850052)) ;
#85127=CARTESIAN_POINT('Ctrl Pts',(-20.810144830431,12.5170965677374,122.855005173606)) ;
#85128=CARTESIAN_POINT('Ctrl Pts',(-20.8856671720647,12.5270915704683,123.106592117066)) ;
#85129=CARTESIAN_POINT('Ctrl Pts',(-20.916070552576,12.5371279014786,123.36856478643)) ;
#85130=CARTESIAN_POINT('Ctrl Pts',(-20.9012433064245,12.5469741308209,123.62690469604)) ;
#85131=CARTESIAN_POINT('Ctrl Pts',(-20.8414337010136,12.5569596290961,123.882363589347)) ;
#85132=CARTESIAN_POINT('Ctrl Pts',(-20.7388385515527,12.5668945320791,124.122491967746)) ;
#85133=CARTESIAN_POINT('Ctrl Pts',(-20.5941950356551,12.5769520351743,124.343654958997)) ;
#85134=CARTESIAN_POINT('Ctrl Pts',(-20.4178326753157,12.5867736915449,124.532143914003)) ;
#85135=CARTESIAN_POINT('Ctrl Pts',(-20.2068320884318,12.59682975421,124.691210472913)) ;
#85136=CARTESIAN_POINT('Ctrl Pts',(-19.9738765529842,12.6067704189132,124.809442393321)) ;
#85137=CARTESIAN_POINT('Ctrl Pts',(-19.7250875546676,12.6166748228617,124.885930317569)) ;
#85138=CARTESIAN_POINT('Ctrl Pts',(-19.4630957051046,12.6267213078553,124.918354057249)) ;
#85139=CARTESIAN_POINT('Ctrl Pts',(-19.2033273420661,12.636617535667,124.905216890975)) ;
#85140=CARTESIAN_POINT('Ctrl Pts',(-18.9456557927353,12.6466771192305,124.846275394572)) ;
#85141=CARTESIAN_POINT('Ctrl Pts',(-18.7071089141504,12.6565291288993,124.74562108305)) ;
#85142=CARTESIAN_POINT('Ctrl Pts',(-18.4867674844916,12.6664916603389,124.604252671323)) ;
#85143=CARTESIAN_POINT('Ctrl Pts',(-18.2932471898541,12.6765232085783,124.425230066221)) ;
#85144=CARTESIAN_POINT('Ctrl Pts',(-18.1357855764971,12.6864146197913,124.218414587344)) ;
#85145=CARTESIAN_POINT('Ctrl Pts',(-18.0146947587827,12.6964308734993,123.984694568915)) ;
#85146=CARTESIAN_POINT('Ctrl Pts',(-17.9364655443542,12.706460976344,123.732995067848)) ;
#85147=CARTESIAN_POINT('Ctrl Pts',(-17.9032103304628,12.7163174252977,123.476104767026)) ;
#85148=CARTESIAN_POINT('Ctrl Pts',(-17.9149031126223,12.72631643607,123.213643474476)) ;
#85149=CARTESIAN_POINT('Ctrl Pts',(-17.9711347927928,12.736211652988,122.959716591098)) ;
#85150=CARTESIAN_POINT('Ctrl Pts',(-18.0722621730133,12.7462721683453,122.715478970838)) ;
#85151=CARTESIAN_POINT('Ctrl Pts',(-18.2111849666589,12.7561214617324,122.497067612659)) ;
#85152=CARTESIAN_POINT('Ctrl Pts',(-18.3885653163835,12.7661486374124,122.30221638746)) ;
#85153=CARTESIAN_POINT('Ctrl Pts',(-18.5975514154094,12.7761772130396,122.141639073802)) ;
#85154=CARTESIAN_POINT('Ctrl Pts',(-18.8267178958733,12.7860223065854,122.021590045095)) ;
#85155=CARTESIAN_POINT('Ctrl Pts',(-19.0767118104658,12.7960135480172,121.94132806078)) ;
#85156=CARTESIAN_POINT('Ctrl Pts',(-19.3380817266942,12.8060493291605,121.906076455516)) ;
#85157=CARTESIAN_POINT('Ctrl Pts',(-19.596780887396,12.8159015348902,121.916202048577)) ;
#85158=CARTESIAN_POINT('Ctrl Pts',(-19.8527792150898,12.8258636290072,121.970959750396)) ;
#85159=CARTESIAN_POINT('Ctrl Pts',(-20.0967365608284,12.8358861898343,122.070232238452)) ;
#85160=CARTESIAN_POINT('Ctrl Pts',(-20.3178000252107,12.8458139614859,122.208825541157)) ;
#85161=CARTESIAN_POINT('Ctrl Pts',(-20.5136248486434,12.8558563456107,122.38570732732)) ;
#85162=CARTESIAN_POINT('Ctrl Pts',(-20.67339581321,12.8657455696813,122.590690688902)) ;
#85163=CARTESIAN_POINT('Ctrl Pts',(-20.7968031363708,12.8757348178486,122.822371490678)) ;
#85164=CARTESIAN_POINT('Ctrl Pts',(-20.8776695418149,12.8856933948906,123.071257865387)) ;
#85165=CARTESIAN_POINT('Ctrl Pts',(-20.9145160925794,12.8955929639819,123.328801889037)) ;
#85166=CARTESIAN_POINT('Ctrl Pts',(-20.9058665992661,12.9056408760659,123.592681474373)) ;
#85167=CARTESIAN_POINT('Ctrl Pts',(-20.8525411197741,12.9155362303731,123.847236588034)) ;
#85168=CARTESIAN_POINT('Ctrl Pts',(-20.7542629977425,12.9255978808643,124.092671346512)) ;
#85169=CARTESIAN_POINT('Ctrl Pts',(-20.6178824497922,12.9354424963268,124.312521389387)) ;
#85170=CARTESIAN_POINT('Ctrl Pts',(-20.4440872979319,12.9454025752282,124.508228135365)) ;
#85171=CARTESIAN_POINT('Ctrl Pts',(-20.2370284211193,12.9554407695865,124.671653791003)) ;
#85172=CARTESIAN_POINT('Ctrl Pts',(-20.008735431722,12.9653144849861,124.795042874335)) ;
#85173=CARTESIAN_POINT('Ctrl Pts',(-19.7576063109488,12.9753861945204,124.878511544747)) ;
#85174=CARTESIAN_POINT('Ctrl Pts',(-19.5019831838198,12.9852186349729,124.916346652394)) ;
#85175=CARTESIAN_POINT('Ctrl Pts',(-19.2384448043294,12.9952504558983,124.909813965164)) ;
#85176=CARTESIAN_POINT('Ctrl Pts',(-18.9804789488314,13.0052708257839,124.856943439991)) ;
#85177=CARTESIAN_POINT('Ctrl Pts',(-18.7391020985709,13.0151375969176,124.762195065093)) ;
#85178=CARTESIAN_POINT('Ctrl Pts',(-18.5133119731303,13.025208368107,124.624195283185)) ;
#85179=CARTESIAN_POINT('Ctrl Pts',(-18.3193460395093,13.0350515286286,124.453039947988)) ;
#85180=CARTESIAN_POINT('Ctrl Pts',(-18.1551409871327,13.045031761815,124.248545739038)) ;
#85181=CARTESIAN_POINT('Ctrl Pts',(-18.0288968334375,13.0550502818502,124.01751953666)) ;
#85182=CARTESIAN_POINT('Ctrl Pts',(-17.9452843626105,13.0649335902339,123.771589310434)) ;
#85183=CARTESIAN_POINT('Ctrl Pts',(-17.9050279627347,13.0750018744047,123.510130021932)) ;
#85184=CARTESIAN_POINT('Ctrl Pts',(-17.9103427016909,13.0848320010723,123.251814495464)) ;
#85185=CARTESIAN_POINT('Ctrl Pts',(-17.9612809092981,13.0948985732789,122.992269532793)) ;
#85186=CARTESIAN_POINT('Ctrl Pts',(-18.0550171292814,13.1047887295196,122.749822905915)) ;
#85187=CARTESIAN_POINT('Ctrl Pts',(-18.1903054658587,13.114781257096,122.524782428398)) ;
#85188=CARTESIAN_POINT('Ctrl Pts',(-18.3622584156365,13.1247427469703,122.327401305476)) ;
#85189=CARTESIAN_POINT('Ctrl Pts',(-18.5644359884156,13.1346519688575,122.163265725879)) ;
#85190=CARTESIAN_POINT('Ctrl Pts',(-18.7952652342093,13.1447005486678,122.035044644749)) ;
#85191=CARTESIAN_POINT('Ctrl Pts',(-19.0407361930169,13.1545835231379,121.950173803814)) ;
#85192=CARTESIAN_POINT('Ctrl Pts',(-19.3000068336127,13.1645784342806,121.908192940554)) ;
#85193=CARTESIAN_POINT('Ctrl Pts',(-19.5633186687248,13.1745988208542,121.912239958628)) ;
#85194=CARTESIAN_POINT('Ctrl Pts',(-19.8190763964686,13.1845089247113,121.961246286646)) ;
#85195=CARTESIAN_POINT('Ctrl Pts',(-20.0631402215822,13.1944366369212,122.053450497386)) ;
#85196=CARTESIAN_POINT('Ctrl Pts',(-20.2899638294564,13.2044797466884,122.188360062557)) ;
#85197=CARTESIAN_POINT('Ctrl Pts',(-20.4869257177344,13.214366167144,122.35780741445)) ;
#85198=CARTESIAN_POINT('Ctrl Pts',(-20.6535775719235,13.2243593447496,122.560745126669)) ;
#85199=CARTESIAN_POINT('Ctrl Pts',(-20.781768758078,13.2343050076535,122.788511159415)) ;
#85200=CARTESIAN_POINT('Ctrl Pts',(-20.8689866491185,13.2442523038587,123.034949721076)) ;
#85201=CARTESIAN_POINT('Ctrl Pts',(-20.9122331010744,13.2543000694366,123.295421612396)) ;
#85202=CARTESIAN_POINT('Ctrl Pts',(-20.9098535935215,13.2641482826542,123.554208720169)) ;
#85203=CARTESIAN_POINT('Ctrl Pts',(-20.862891829645,13.2741078554483,123.811687555265)) ;
#85204=CARTESIAN_POINT('Ctrl Pts',(-20.7708019573289,13.2841444764808,124.058831482253)) ;
#85205=CARTESIAN_POINT('Ctrl Pts',(-20.6396072016662,13.2940249912912,124.282931024446)) ;
#85206=CARTESIAN_POINT('Ctrl Pts',(-20.4686846093292,13.3040776425982,124.484308739774)) ;
#85207=CARTESIAN_POINT('Ctrl Pts',(-20.2685764087636,13.3139730408782,124.650446241866)) ;
#85208=CARTESIAN_POINT('Ctrl Pts',(-20.0392572485433,13.3240231625843,124.781393384691)) ;
#85209=CARTESIAN_POINT('Ctrl Pts',(-19.7947435724965,13.3339074421262,124.869123479395)) ;
#85210=CARTESIAN_POINT('Ctrl Pts',(-19.5359835923959,13.3439022234181,124.914032922456)) ;
#85211=CARTESIAN_POINT('Ctrl Pts',(-19.2745480154649,13.3538500686049,124.913233748315)) ;
#85212=CARTESIAN_POINT('Ctrl Pts',(-19.0174771736584,13.3637870319923,124.867483970433)) ;
#85213=CARTESIAN_POINT('Ctrl Pts',(-18.770953528208,13.3737699967295,124.777666914607)) ;
#85214=CARTESIAN_POINT('Ctrl Pts',(-18.5426825818329,13.3838138481452,124.645222231553)) ;
#85215=CARTESIAN_POINT('Ctrl Pts',(-18.3447626868737,13.3936420494799,124.479227338155)) ;
#85216=CARTESIAN_POINT('Ctrl Pts',(-18.174439114941,13.403718622078,124.276543144147)) ;
#85217=CARTESIAN_POINT('Ctrl Pts',(-18.0446799079283,13.4135707020855,124.052439270463)) ;
#85218=CARTESIAN_POINT('Ctrl Pts',(-17.9536328215657,13.4236439870896,123.803921128187)) ;
#85219=CARTESIAN_POINT('Ctrl Pts',(-17.908245672822,13.4334853388001,123.549293611183)) ;
#85220=CARTESIAN_POINT('Ctrl Pts',(-17.9067874767793,13.4434468381966,123.287535568875)) ;
#85221=CARTESIAN_POINT('Ctrl Pts',(-17.9515894545495,13.4534826143266,123.027629899913)) ;
#85222=CARTESIAN_POINT('Ctrl Pts',(-18.0392686443259,13.4633710409642,122.783013986504)) ;
#85223=CARTESIAN_POINT('Ctrl Pts',(-18.1693153244225,13.4733863630391,122.554183172307)) ;
#85224=CARTESIAN_POINT('Ctrl Pts',(-18.3378376719635,13.4834167119393,122.35150318048)) ;
#85225=CARTESIAN_POINT('Ctrl Pts',(-18.5349010784944,13.493260087546,122.183945153477)) ;
#85226=CARTESIAN_POINT('Ctrl Pts',(-18.761992836842,13.5032895244431,122.050165209368)) ;
#85227=CARTESIAN_POINT('Ctrl Pts',(-19.0091803607605,13.513321402376,121.958500067657)) ;
#85228=CARTESIAN_POINT('Ctrl Pts',(-19.2631820189547,13.5231510254815,121.911588708017)) ;
#85229=CARTESIAN_POINT('Ctrl Pts',(-19.5256857167379,13.5331404966346,121.908671418978)) ;
#85230=CARTESIAN_POINT('Ctrl Pts',(-19.7859990638554,13.543184345397,121.952270006427)) ;
#85231=CARTESIAN_POINT('Ctrl Pts',(-20.0294662569613,13.5530060509287,122.037953136693)) ;
#85232=CARTESIAN_POINT('Ctrl Pts',(-20.2595578583272,13.5630410907565,122.166795368885)) ;
#85233=CARTESIAN_POINT('Ctrl Pts',(-20.4631193550347,13.573065797648,122.334030527681)) ;
#85234=CARTESIAN_POINT('Ctrl Pts',(-20.6320196881759,13.5829185019887,122.530273988873)) ;
#85235=CARTESIAN_POINT('Ctrl Pts',(-20.7664821078402,13.5929066241964,122.755672189208)) ;
#85236=CARTESIAN_POINT('Ctrl Pts',(-20.8592301070909,13.6028350943037,122.999547591303)) ;
#85237=CARTESIAN_POINT('Ctrl Pts',(-20.9089521249442,13.6128240714709,123.257308236829)) ;
#85238=CARTESIAN_POINT('Ctrl Pts',(-20.9127323662985,13.6228618787506,123.521057016566)) ;
#85239=CARTESIAN_POINT('Ctrl Pts',(-20.8718783998989,13.6327081796139,123.776564736996)) ;
#85240=CARTESIAN_POINT('Ctrl Pts',(-20.7862945910431,13.6427339229932,124.025746367502)) ;
#85241=CARTESIAN_POINT('Ctrl Pts',(-20.6580767870656,13.6527647894322,124.256070820692)) ;
#85242=CARTESIAN_POINT('Ctrl Pts',(-20.4954356848382,13.662602148231,124.457000727745)) ;
#85243=CARTESIAN_POINT('Ctrl Pts',(-20.2977665459096,13.6725941091647,124.629841734287)) ;
#85244=CARTESIAN_POINT('Ctrl Pts',(-20.0718975262772,13.6826264717213,124.765837185899)) ;
#85245=CARTESIAN_POINT('Ctrl Pts',(-19.8300805604924,13.6924916322957,124.859254064222)) ;
#85246=CARTESIAN_POINT('Ctrl Pts',(-19.5733470333744,13.7024535368734,124.910489003739)) ;
#85247=CARTESIAN_POINT('Ctrl Pts',(-19.3097110945833,13.7124884669491,124.915979322584)) ;
#85248=CARTESIAN_POINT('Ctrl Pts',(-19.052903569064,13.7223734138028,124.876639088694)) ;
#85249=CARTESIAN_POINT('Ctrl Pts',(-18.802425491904,13.7324390901142,124.791752081939)) ;
#85250=CARTESIAN_POINT('Ctrl Pts',(-18.5755121673576,13.7422780097491,124.667718382011)) ;
#85251=CARTESIAN_POINT('Ctrl Pts',(-18.3688230223248,13.7523415194835,124.502800514481)) ;
#85252=CARTESIAN_POINT('Ctrl Pts',(-18.1969779972077,13.7622351326453,124.307654410282)) ;
#85253=CARTESIAN_POINT('Ctrl Pts',(-18.0603814063974,13.7721791394587,124.084921230377)) ;
#85254=CARTESIAN_POINT('Ctrl Pts',(-17.9638424346081,13.782180093813,123.840436569305)) ;
#85255=CARTESIAN_POINT('Ctrl Pts',(-17.9114952956979,13.7922188515053,123.581898288947)) ;
#85256=CARTESIAN_POINT('Ctrl Pts',(-17.9044097597817,13.8020430356753,123.323804444879)) ;
#85257=CARTESIAN_POINT('Ctrl Pts',(-17.942755586416,13.8121011012747,123.062308840123)) ;
#85258=CARTESIAN_POINT('Ctrl Pts',(-18.0252033616295,13.8220311480494,122.814707785698)) ;
#85259=CARTESIAN_POINT('Ctrl Pts',(-18.1490450109907,13.8319825903865,122.58437299172)) ;
#85260=CARTESIAN_POINT('Ctrl Pts',(-18.312830616674,13.8420293875658,122.377301209051)) ;
#85261=CARTESIAN_POINT('Ctrl Pts',(-18.5060204476613,13.8518773282459,122.20510405819)) ;
#85262=CARTESIAN_POINT('Ctrl Pts',(-18.7282785603277,13.8618389595885,122.066811224224)) ;
#85263=CARTESIAN_POINT('Ctrl Pts',(-18.9729559764164,13.8718676189644,121.968851551182)) ;
#85264=CARTESIAN_POINT('Ctrl Pts',(-19.2278374256175,13.8817779218526,121.915423966121)) ;
#85265=CARTESIAN_POINT('Ctrl Pts',(-19.4887668418426,13.8917128164148,121.906358743324)) ;
#85266=CARTESIAN_POINT('Ctrl Pts',(-19.7500201068666,13.9017539150817,121.943366287556)) ;
#85267=CARTESIAN_POINT('Ctrl Pts',(-19.997114009859,13.9116411975861,122.023756349265)) ;
#85268=CARTESIAN_POINT('Ctrl Pts',(-20.229100640813,13.9216329380966,122.146710775795)) ;
#85269=CARTESIAN_POINT('Ctrl Pts',(-20.435328819661,13.931583487332,122.307501482509)) ;
#85270=CARTESIAN_POINT('Ctrl Pts',(-20.610513668173,13.9415191649668,122.501085313789)) ;
#85271=CARTESIAN_POINT('Ctrl Pts',(-20.7503773911135,13.9515045827596,122.723134407814)) ;
#85272=CARTESIAN_POINT('Ctrl Pts',(-20.8496809192691,13.9615333756301,122.967254089343)) ;
#85273=CARTESIAN_POINT('Ctrl Pts',(-20.9045337829199,13.9714128868581,123.221012810142)) ;
#85274=CARTESIAN_POINT('Ctrl Pts',(-20.9152110491903,13.981406423531,123.483425425094)) ;
#85275=CARTESIAN_POINT('Ctrl Pts',(-20.8794859206276,13.9914386917948,123.744619970286)) ;
#85276=CARTESIAN_POINT('Ctrl Pts',(-20.8008196116492,14.0013026538007,123.991638075795)) ;
#85277=CARTESIAN_POINT('Ctrl Pts',(-20.6780078275285,14.0113727151456,124.226013909898)) ;
#85278=CARTESIAN_POINT('Ctrl Pts',(-20.5199890005443,14.0212150794943,124.43079250126)) ;
#85279=CARTESIAN_POINT('Ctrl Pts',(-20.3271803845075,14.0311757519968,124.607819487763)) ;
#85280=CARTESIAN_POINT('Ctrl Pts',(-20.1045706887236,14.0412138230646,124.749326629548)) ;
#85281=CARTESIAN_POINT('Ctrl Pts',(-19.8649107838462,14.051087438025,124.848860391817)) ;
#85282=CARTESIAN_POINT('Ctrl Pts',(-19.6065853682649,14.0611596726063,124.906317466992)) ;
#85283=CARTESIAN_POINT('Ctrl Pts',(-19.3486353561911,14.0709836910551,124.91805722916)) ;
#85284=CARTESIAN_POINT('Ctrl Pts',(-19.0863513066081,14.0810486120311,124.884370279709)) ;
#85285=CARTESIAN_POINT('Ctrl Pts',(-18.7548552994364,14.0942589103259,124.781024489845)) ;
#85286=CARTESIAN_POINT('Ctrl Pts',(-18.4555139703643,14.1075743570578,124.592476583949)) ;
#85287=CARTESIAN_POINT('Ctrl Pts',(-18.2182215362896,14.1208646023251,124.336059674344)) ;
#85288=CARTESIAN_POINT('Ctrl Pts',(-18.0753754053462,14.1309153519322,124.113963002068)) ;
#85289=CARTESIAN_POINT('Ctrl Pts',(-17.9751742641188,14.1407279589144,123.876319735043)) ;
#85290=CARTESIAN_POINT('Ctrl Pts',(-17.9159189092107,14.1507990569087,123.618416063707)) ;
#85291=CARTESIAN_POINT('Ctrl Pts',(-17.9028526558769,14.1606886296836,123.35883798821)) ;
#85292=CARTESIAN_POINT('Ctrl Pts',(-17.9449956703198,14.1739587364869,123.012660958945)) ;
#85293=CARTESIAN_POINT('Ctrl Pts',(-18.110043879932,14.1905754234094,122.603035428979)) ;
#85294=CARTESIAN_POINT('Ctrl Pts',(-18.4039594470265,14.2071494667256,122.274938448092)) ;
#85295=CARTESIAN_POINT('Ctrl Pts',(-18.6963137378166,14.2204460341574,122.08351795448)) ;
#85296=CARTESIAN_POINT('Ctrl Pts',(-18.9385848307681,14.2304760977348,121.979689993019)) ;
#85297=CARTESIAN_POINT('Ctrl Pts',(-19.1916875088085,14.240369989584,121.920298097705)) ;
#85298=CARTESIAN_POINT('Ctrl Pts',(-19.5394066171243,14.2536227453696,121.899565963118)) ;
#85299=CARTESIAN_POINT('Ctrl Pts',(-19.9747350131759,14.270350850362,121.989580778364)) ;
#85300=CARTESIAN_POINT('Ctrl Pts',(-20.4235622970495,14.2901816868405,122.266085506153)) ;
#85301=CARTESIAN_POINT('Ctrl Pts',(-20.7535383605483,14.3101070787307,122.680152104981)) ;
#85302=CARTESIAN_POINT('Ctrl Pts',(-20.9224097639681,14.3300322920827,123.182173590077)) ;
#85303=CARTESIAN_POINT('Ctrl Pts',(-20.909967365172,14.3499573055678,123.711540173755)) ;
#85304=CARTESIAN_POINT('Ctrl Pts',(-20.7187416801209,14.3698337772678,124.204034514213)) ;
#85305=CARTESIAN_POINT('Ctrl Pts',(-20.3693357021894,14.3898130951767,124.603894071184)) ;
#85306=CARTESIAN_POINT('Ctrl Pts',(-19.9052962266747,14.4097460987527,124.85959923876)) ;
#85307=CARTESIAN_POINT('Ctrl Pts',(-19.3830046122281,14.4296413687804,124.941993474064)) ;
#85308=CARTESIAN_POINT('Ctrl Pts',(-18.863111653506,14.4495627066862,124.841603993362)) ;
#85309=CARTESIAN_POINT('Ctrl Pts',(-18.4079099213766,14.4695203299524,124.569231338478)) ;
#85310=CARTESIAN_POINT('Ctrl Pts',(-18.0742589102781,14.4894001619096,124.159636622647)) ;
#85311=CARTESIAN_POINT('Ctrl Pts',(-17.8989537036202,14.5092820132065,123.661028976949)) ;
#85312=CARTESIAN_POINT('Ctrl Pts',(-17.9053799742444,14.5293530303103,123.127680005003)) ;
#85313=CARTESIAN_POINT('Ctrl Pts',(-18.090928041147,14.5491602540634,122.634917461125)) ;
#85314=CARTESIAN_POINT('Ctrl Pts',(-18.4354593545979,14.5691413896322,122.230840604619)) ;
#85315=CARTESIAN_POINT('Ctrl Pts',(-18.8964698224689,14.5890688829714,121.970192630458)) ;
#85316=CARTESIAN_POINT('Ctrl Pts',(-19.4158400705055,14.6088895443292,121.881168125595)) ;
#85317=CARTESIAN_POINT('Ctrl Pts',(-19.9411622969537,14.628986733551,121.976797339529)) ;
#85318=CARTESIAN_POINT('Ctrl Pts',(-20.3952297063123,14.6487504125593,122.241401014461)) ;
#85319=CARTESIAN_POINT('Ctrl Pts',(-20.7369043382646,14.6688076912324,122.650295252524)) ;
#85320=CARTESIAN_POINT('Ctrl Pts',(-20.9160056364455,14.6886031149798,123.145152863214)) ;
#85321=CARTESIAN_POINT('Ctrl Pts',(-20.9171281004685,14.7085667597074,123.675691935841)) ;
#85322=CARTESIAN_POINT('Ctrl Pts',(-20.7357205067967,14.7285502509815,124.174887049982)) ;
#85323=CARTESIAN_POINT('Ctrl Pts',(-20.398657784175,14.7483577461308,124.579349028364)) ;
#85324=CARTESIAN_POINT('Ctrl Pts',(-19.9402292141674,14.7683403368509,124.847300212365)) ;
#85325=CARTESIAN_POINT('Ctrl Pts',(-19.4202472432439,14.7882229908422,124.942207693304)) ;
#85326=CARTESIAN_POINT('Ctrl Pts',(-18.8972710117422,14.8081812357052,124.854072619313)) ;
#85327=CARTESIAN_POINT('Ctrl Pts',(-18.4373523571738,14.8280568227468,124.59403836842)) ;
#85328=CARTESIAN_POINT('Ctrl Pts',(-18.0917464518894,14.8480377108821,124.190871761856)) ;
#85329=CARTESIAN_POINT('Ctrl Pts',(-17.9052470733622,14.8679728519931,123.694860655022)) ;
#85330=CARTESIAN_POINT('Ctrl Pts',(-17.8988327545552,14.8878848700041,123.165719308424)) ;
#85331=CARTESIAN_POINT('Ctrl Pts',(-18.0726432682034,14.9077730882477,122.666502021473)) ;
#85332=CARTESIAN_POINT('Ctrl Pts',(-18.3508412756587,14.9243713920946,122.324182529583)) ;
#85333=CARTESIAN_POINT('Ctrl Pts',(-18.6332517724376,14.9376439819974,122.119434069299)) ;
#85334=CARTESIAN_POINT('Ctrl Pts',(-18.8696162522265,14.9476513969483,122.004144120758)) ;
#85335=CARTESIAN_POINT('Ctrl Pts',(-19.122481344444,14.9576587436809,121.931865885675)) ;
#85336=CARTESIAN_POINT('Ctrl Pts',(-19.4692168268051,14.9709251034825,121.895493051636)) ;
#85337=CARTESIAN_POINT('Ctrl Pts',(-19.9027943031777,14.9874397611055,121.963407923393)) ;
#85338=CARTESIAN_POINT('Ctrl Pts',(-20.289623579524,15.0040371943481,122.175392008362)) ;
#85339=CARTESIAN_POINT('Ctrl Pts',(-20.5428597744861,15.0173851914931,122.41816948796)) ;
#85340=CARTESIAN_POINT('Ctrl Pts',(-20.6967684183011,15.0272809458447,122.627784026657)) ;
#85341=CARTESIAN_POINT('Ctrl Pts',(-20.81329530157,15.0372688997761,122.862950598469)) ;
#85342=CARTESIAN_POINT('Ctrl Pts',(-20.8871174069244,15.0472261234808,123.114018836122)) ;
#85343=CARTESIAN_POINT('Ctrl Pts',(-20.9163251075997,15.0572616700375,123.376101669285)) ;
#85344=CARTESIAN_POINT('Ctrl Pts',(-20.9000253490332,15.0671487813136,123.635429990405)) ;
#85345=CARTESIAN_POINT('Ctrl Pts',(-20.8387149445651,15.0771401864144,123.890722088326)) ;
#85346=CARTESIAN_POINT('Ctrl Pts',(-20.7344102203298,15.0870858076292,124.130366678656)) ;
#85347=CARTESIAN_POINT('Ctrl Pts',(-20.5904612859192,15.0970350558975,124.348645357239)) ;
#85348=CARTESIAN_POINT('Ctrl Pts',(-20.4088366867784,15.1070815510661,124.540239084563)) ;
#85349=CARTESIAN_POINT('Ctrl Pts',(-20.2009583169496,15.1169328938577,124.694555578007)) ;
#85350=CARTESIAN_POINT('Ctrl Pts',(-19.966949092894,15.126904673985,124.812422819299)) ;
#85351=CARTESIAN_POINT('Ctrl Pts',(-19.7153621269984,15.1368998739627,124.888039277954)) ;
#85352=CARTESIAN_POINT('Ctrl Pts',(-19.4534809990243,15.1469338656587,124.918615290549)) ;
#85353=CARTESIAN_POINT('Ctrl Pts',(-19.1948823108826,15.1567892706313,124.903936975073)) ;
#85354=CARTESIAN_POINT('Ctrl Pts',(-18.9390660225398,15.166788568477,124.844078851224)) ;
#85355=CARTESIAN_POINT('Ctrl Pts',(-18.6998538262199,15.1766836810822,124.742011656425)) ;
#85356=CARTESIAN_POINT('Ctrl Pts',(-18.4784349324494,15.1867443266172,124.59760214482)) ;
#85357=CARTESIAN_POINT('Ctrl Pts',(-18.289374519982,15.1965932036064,124.420815614991)) ;
#85358=CARTESIAN_POINT('Ctrl Pts',(-18.1305264432099,15.2066219147,124.210528253693)) ;
#85359=CARTESIAN_POINT('Ctrl Pts',(-18.0112304288892,15.2166513159561,123.975504636893)) ;
#85360=CARTESIAN_POINT('Ctrl Pts',(-17.9354501387818,15.2264915077521,123.728262940677)) ;
#85361=CARTESIAN_POINT('Ctrl Pts',(-17.9027451697684,15.2364949369451,123.467452153963)) ;
#85362=CARTESIAN_POINT('Ctrl Pts',(-17.9158870952322,15.2464804494113,123.205327859872)) ;
#85363=CARTESIAN_POINT('Ctrl Pts',(-17.9749122216437,15.2565215457953,122.94817162508)) ;
#85364=CARTESIAN_POINT('Ctrl Pts',(-18.075352673942,15.2663647417463,122.709774454952)) ;
#85365=CARTESIAN_POINT('Ctrl Pts',(-18.2172239193815,15.2763510528007,122.489051700623)) ;
#85366=CARTESIAN_POINT('Ctrl Pts',(-18.3942788891156,15.2862857380584,122.297122889139)) ;
#85367=CARTESIAN_POINT('Ctrl Pts',(-18.6046088256348,15.2963432992754,122.137133343391)) ;
#85368=CARTESIAN_POINT('Ctrl Pts',(-18.8338906873732,15.306164940884,122.018552182692)) ;
#85369=CARTESIAN_POINT('Ctrl Pts',(-19.0859639637451,15.316221004475,121.939290081059)) ;
#85370=CARTESIAN_POINT('Ctrl Pts',(-19.3450573076827,15.3261616802368,121.905856443279)) ;
#85371=CARTESIAN_POINT('Ctrl Pts',(-19.6050966128801,15.3360660390251,121.917057614141)) ;
#85372=CARTESIAN_POINT('Ctrl Pts',(-19.8628314894455,15.3461126936009,121.974204391667)) ;
#85373=CARTESIAN_POINT('Ctrl Pts',(-20.1032054022461,15.3560082882438,122.073524957395)) ;
#85374=CARTESIAN_POINT('Ctrl Pts',(-20.3263274818967,15.3660702349007,122.215360141734)) ;
#85375=CARTESIAN_POINT('Ctrl Pts',(-20.5173806023937,15.3759198588328,122.390011089637)) ;
#85376=CARTESIAN_POINT('Ctrl Pts',(-20.6776940933443,15.3858830978627,122.596996909064)) ;
#85377=CARTESIAN_POINT('Ctrl Pts',(-20.8000760560513,15.3959076726385,122.830296872806)) ;
#85378=CARTESIAN_POINT('Ctrl Pts',(-20.8793976462342,15.4058262353262,123.078576451367)) ;
#85379=CARTESIAN_POINT('Ctrl Pts',(-20.9151255754094,15.4158184220502,123.338734291713)) ;
#85380=CARTESIAN_POINT('Ctrl Pts',(-20.9046224904582,15.4258532206344,123.602218432797)) ;
#85381=CARTESIAN_POINT('Ctrl Pts',(-20.8499613006373,15.4357084113081,123.855389436239)) ;
#85382=CARTESIAN_POINT('Ctrl Pts',(-20.7510911952532,15.4457077594611,124.098804793932)) ;
#85383=CARTESIAN_POINT('Ctrl Pts',(-20.6131053102038,15.4556028851362,124.319258702986)) ;
#85384=CARTESIAN_POINT('Ctrl Pts',(-20.4360576038621,15.4656634280843,124.51555709839)) ;
#85385=CARTESIAN_POINT('Ctrl Pts',(-20.2320397835465,15.4755127023512,124.674867184459)) ;
#85386=CARTESIAN_POINT('Ctrl Pts',(-19.9996679689736,15.4855399269211,124.799102630686)) ;
#85387=CARTESIAN_POINT('Ctrl Pts',(-19.7489910633449,15.4955683261089,124.880464971312)) ;
#85388=CARTESIAN_POINT('Ctrl Pts',(-19.4928458279102,15.5054140765224,124.916870140584)) ;
#85389=CARTESIAN_POINT('Ctrl Pts',(-19.2304605256444,15.5154028669231,124.908855957832)) ;
#85390=CARTESIAN_POINT('Ctrl Pts',(-18.9721684140402,15.5254477953228,124.854455310312)) ;
#85391=CARTESIAN_POINT('Ctrl Pts',(-18.7323714755152,15.5352722801118,124.7587411508)) ;
#85392=CARTESIAN_POINT('Ctrl Pts',(-18.5074627778425,15.545329677653,124.619968276734)) ;
#85393=CARTESIAN_POINT('Ctrl Pts',(-18.3128405903418,15.5552557692392,124.446263039187)) ;
#85394=CARTESIAN_POINT('Ctrl Pts',(-18.150350868832,15.5652105543838,124.241248427742)) ;
#85395=CARTESIAN_POINT('Ctrl Pts',(-18.0251521487945,15.5752479240414,124.009084692641)) ;
#85396=CARTESIAN_POINT('Ctrl Pts',(-17.9432016162711,15.585136734163,123.762469410516)) ;
#85397=CARTESIAN_POINT('Ctrl Pts',(-17.9044670409744,15.5951260932141,123.502838762861)) ;
#85398=CARTESIAN_POINT('Ctrl Pts',(-17.9115749765126,15.6050846406702,123.24124293323)) ;
#85399=CARTESIAN_POINT('Ctrl Pts',(-17.9630623576573,15.6149842172212,122.986221570105)) ;
#85400=CARTESIAN_POINT('Ctrl Pts',(-18.0595417871603,15.6250321290519,122.740459685975)) ;
#85401=CARTESIAN_POINT('Ctrl Pts',(-18.1949986414737,15.6349274769125,122.518438659765)) ;
#85402=CARTESIAN_POINT('Ctrl Pts',(-18.3697629356532,15.6449891534437,122.320059129432)) ;
#85403=CARTESIAN_POINT('Ctrl Pts',(-18.5718644577124,15.6548336711928,122.158541982419)) ;
#85404=CARTESIAN_POINT('Ctrl Pts',(-18.8011526189207,15.6647941149076,122.032301199326)) ;
#85405=CARTESIAN_POINT('Ctrl Pts',(-19.0509357609831,15.6748309477258,121.947606476504)) ;
#85406=CARTESIAN_POINT('Ctrl Pts',(-19.3074921480599,15.6847097444726,121.907773626489)) ;
#85407=CARTESIAN_POINT('Ctrl Pts',(-19.5717593834283,15.694769060601,121.913104494787)) ;
#85408=CARTESIAN_POINT('Ctrl Pts',(-19.8262605890557,15.7046395073542,121.963283380412)) ;
#85409=CARTESIAN_POINT('Ctrl Pts',(-20.0714198955884,15.7146321456122,122.057380334014)) ;
#85410=CARTESIAN_POINT('Ctrl Pts',(-20.2971021415107,15.7246641611601,122.193630102715)) ;
#85411=CARTESIAN_POINT('Ctrl Pts',(-20.4928065396954,15.7345300174667,122.363722707075)) ;
#85412=CARTESIAN_POINT('Ctrl Pts',(-20.659353254304,15.7445993069358,122.569307538849)) ;
#85413=CARTESIAN_POINT('Ctrl Pts',(-20.7848456281026,15.7544428644871,122.795525024093)) ;
#85414=CARTESIAN_POINT('Ctrl Pts',(-20.8711257023825,15.764422991275,123.043184928911)) ;
#85415=CARTESIAN_POINT('Ctrl Pts',(-20.9127559215498,15.7744415398749,123.303142599032)) ;
#85416=CARTESIAN_POINT('Ctrl Pts',(-20.9092242705699,15.7843248403981,123.562873547571)) ;
#85417=CARTESIAN_POINT('Ctrl Pts',(-20.8596396741269,15.7943931274462,123.822725252708)) ;
#85418=CARTESIAN_POINT('Ctrl Pts',(-20.7681651750302,15.8042232504649,124.064360555124)) ;
#85419=CARTESIAN_POINT('Ctrl Pts',(-20.6332871001612,15.8142898343902,124.291882100143)) ;
#85420=CARTESIAN_POINT('Ctrl Pts',(-20.4638049151612,15.8241799474047,124.48896825144)) ;
#85421=CARTESIAN_POINT('Ctrl Pts',(-20.2609877478758,15.8341726361673,124.655734358688)) ;
#85422=CARTESIAN_POINT('Ctrl Pts',(-20.0329028474693,15.8441335245231,124.784198130911)) ;
#85423=CARTESIAN_POINT('Ctrl Pts',(-19.7872175767508,15.8540514694031,124.871145968037)) ;
#85424=CARTESIAN_POINT('Ctrl Pts',(-19.5278485703835,15.8640592224993,124.914811107078)) ;
#85425=CARTESIAN_POINT('Ctrl Pts',(-19.2642689030462,15.8740903164583,124.91223920911)) ;
#85426=CARTESIAN_POINT('Ctrl Pts',(-19.0097316360131,15.8839382844863,124.865387875955)) ;
#85427=CARTESIAN_POINT('Ctrl Pts',(-18.761882854262,15.8940002406122,124.773318370912)) ;
#85428=CARTESIAN_POINT('Ctrl Pts',(-18.5376157807696,15.9038974522133,124.641576258663)) ;
#85429=CARTESIAN_POINT('Ctrl Pts',(-18.3384056514573,15.9138286188779,124.472982338498)) ;
#85430=CARTESIAN_POINT('Ctrl Pts',(-18.1698491513015,15.9238708030821,124.269933564785)) ;
#85431=CARTESIAN_POINT('Ctrl Pts',(-18.0409623377378,15.9337574713353,124.044330723478)) ;
#85432=CARTESIAN_POINT('Ctrl Pts',(-17.9518555076836,15.9437505833135,123.79731633989)) ;
#85433=CARTESIAN_POINT('Ctrl Pts',(-17.9072992563308,15.9536962609293,123.539779663906)) ;
#85434=CARTESIAN_POINT('Ctrl Pts',(-17.9076038590327,15.9636435639143,123.278362513842)) ;
#85435=CARTESIAN_POINT('Ctrl Pts',(-17.954039484633,15.9736912876611,123.018441119269)) ;
#85436=CARTESIAN_POINT('Ctrl Pts',(-18.0429092629221,15.9835396614236,122.77537631077)) ;
#85437=CARTESIAN_POINT('Ctrl Pts',(-18.1733362386872,15.9934986338693,122.548480377477)) ;
#85438=CARTESIAN_POINT('Ctrl Pts',(-18.3428858266523,16.0035374957505,122.346380568049)) ;
#85439=CARTESIAN_POINT('Ctrl Pts',(-18.5414869910732,16.0134160999223,122.179156901752)) ;
#85440=CARTESIAN_POINT('Ctrl Pts',(-18.7699271953843,16.0234676411256,122.046612208989)) ;
#85441=CARTESIAN_POINT('Ctrl Pts',(-19.0141072069317,16.0333630391059,121.957051725276)) ;
#85442=CARTESIAN_POINT('Ctrl Pts',(-19.2740547380586,16.0434142716512,121.910401805192)) ;
#85443=CARTESIAN_POINT('Ctrl Pts',(-19.5338803406111,16.0533004622755,121.909579455401)) ;
#85444=CARTESIAN_POINT('Ctrl Pts',(-19.7926868268136,16.0632930015913,121.953875934243)) ;
#85445=CARTESIAN_POINT('Ctrl Pts',(-20.0387894173471,16.073241447486,122.04213980991)) ;
#85446=CARTESIAN_POINT('Ctrl Pts',(-20.265712566684,16.0831782500179,122.171300244256)) ;
#85447=CARTESIAN_POINT('Ctrl Pts',(-20.4679516213838,16.0931612574692,122.338455368566)) ;
#85448=CARTESIAN_POINT('Ctrl Pts',(-20.6387206153012,16.103205098884,122.539669360996)) ;
#85449=CARTESIAN_POINT('Ctrl Pts',(-20.7696595815421,16.1130332975079,122.762338547933)) ;
#85450=CARTESIAN_POINT('Ctrl Pts',(-20.8623125592493,16.1231098909501,123.010343765831)) ;
#85451=CARTESIAN_POINT('Ctrl Pts',(-20.9095729442255,16.1329618902917,123.264952690282)) ;
#85452=CARTESIAN_POINT('Ctrl Pts',(-20.9121762627497,16.1430354771156,123.529617389355)) ;
#85453=CARTESIAN_POINT('Ctrl Pts',(-20.869730533684,16.152875702213,123.784725112839)) ;
#85454=CARTESIAN_POINT('Ctrl Pts',(-20.7834213237411,16.1628414062417,124.031959888329)) ;
#85455=CARTESIAN_POINT('Ctrl Pts',(-20.6543616553613,16.1728680395483,124.261695407877)) ;
#85456=CARTESIAN_POINT('Ctrl Pts',(-20.4893937694131,16.1827823352601,124.463343826805)) ;
#85457=CARTESIAN_POINT('Ctrl Pts',(-20.2907385375805,16.1927706239526,124.634927879414)) ;
#85458=CARTESIAN_POINT('Ctrl Pts',(-20.063944204818,16.2028093571109,124.769667401044)) ;
#85459=CARTESIAN_POINT('Ctrl Pts',(-19.8221495313365,16.2126526889385,124.861577146822)) ;
#85460=CARTESIAN_POINT('Ctrl Pts',(-19.5634230879079,16.2226804148181,124.911613949581)) ;
#85461=CARTESIAN_POINT('Ctrl Pts',(-19.2997995110888,16.2327127512066,124.915252649983)) ;
#85462=CARTESIAN_POINT('Ctrl Pts',(-19.0447508850932,16.2425422515072,124.87443461805)) ;
#85463=CARTESIAN_POINT('Ctrl Pts',(-18.7964127409365,16.252531755424,124.789315485236)) ;
#85464=CARTESIAN_POINT('Ctrl Pts',(-18.5657100501157,16.2625755959364,124.661096709419)) ;
#85465=CARTESIAN_POINT('Ctrl Pts',(-18.3649684583117,16.2723973017045,124.498860195946)) ;
#85466=CARTESIAN_POINT('Ctrl Pts',(-18.1912776614032,16.2824323488368,124.30043121603)) ;
#85467=CARTESIAN_POINT('Ctrl Pts',(-18.0554378922695,16.2924570262737,124.074705597496)) ;
#85468=CARTESIAN_POINT('Ctrl Pts',(-17.9619696621494,16.3023098411282,123.833243322249)) ;
#85469=CARTESIAN_POINT('Ctrl Pts',(-17.9107123152974,16.3122975507357,123.575850309162)) ;
#85470=CARTESIAN_POINT('Ctrl Pts',(-17.9049458569947,16.3222275607298,123.314954275145)) ;
#85471=CARTESIAN_POINT('Ctrl Pts',(-17.9444047205986,16.332217315949,123.055411337041)) ;
#85472=CARTESIAN_POINT('Ctrl Pts',(-18.0289611024086,16.3422439246319,122.805854001657)) ;
#85473=CARTESIAN_POINT('Ctrl Pts',(-18.1535398915879,16.3521278646537,122.577945287591)) ;
#85474=CARTESIAN_POINT('Ctrl Pts',(-18.3170581793031,16.3621170921922,122.372577155451)) ;
#85475=CARTESIAN_POINT('Ctrl Pts',(-18.5151613636324,16.3721599627159,122.198204531201)) ;
#85476=CARTESIAN_POINT('Ctrl Pts',(-18.7355937159182,16.3819923494713,122.06340510794)) ;
#85477=CARTESIAN_POINT('Ctrl Pts',(-18.9797379454661,16.3919856426429,121.966674506609)) ;
#85478=CARTESIAN_POINT('Ctrl Pts',(-19.2380933202206,16.4020176482913,121.914136786792)) ;
#85479=CARTESIAN_POINT('Ctrl Pts',(-19.4972319162803,16.4118829042603,121.907050750478)) ;
#85480=CARTESIAN_POINT('Ctrl Pts',(-19.7563049005742,16.4218447841678,121.944708800064)) ;
#85481=CARTESIAN_POINT('Ctrl Pts',(-20.0065704728934,16.4318797175297,122.027782317763)) ;
#85482=CARTESIAN_POINT('Ctrl Pts',(-20.235395236987,16.441764675909,122.150815185132)) ;
#85483=CARTESIAN_POINT('Ctrl Pts',(-20.4430095418267,16.4518303028317,122.314647056948)) ;
#85484=CARTESIAN_POINT('Ctrl Pts',(-20.6153156253427,16.461669408496,122.507485556433)) ;
#85485=CARTESIAN_POINT('Ctrl Pts',(-20.7548759132793,16.4717322235013,122.732057555602)) ;
#85486=CARTESIAN_POINT('Ctrl Pts',(-20.8514951454901,16.48162842955,122.973534637153)) ;
#85487=CARTESIAN_POINT('Ctrl Pts',(-20.9056579365925,16.4915692525753,123.229061857975)) ;
#85488=CARTESIAN_POINT('Ctrl Pts',(-20.9147539350784,16.501573835554,123.491844043348)) ;
#85489=CARTESIAN_POINT('Ctrl Pts',(-20.8777116944424,16.5115947299987,123.752558207369)) ;
#85490=CARTESIAN_POINT('Ctrl Pts',(-20.7973193962089,16.5214866505881,123.9997713371)) ;
#85491=CARTESIAN_POINT('Ctrl Pts',(-20.6743097948123,16.5314800829335,124.231787262463)) ;
#85492=CARTESIAN_POINT('Ctrl Pts',(-20.5135843010475,16.5414256878334,124.437884102592)) ;
#85493=CARTESIAN_POINT('Ctrl Pts',(-20.3198274952116,16.5513729613149,124.613376926942)) ;
#85494=CARTESIAN_POINT('Ctrl Pts',(-20.0961655477988,16.5614208757913,124.753706244345)) ;
#85495=CARTESIAN_POINT('Ctrl Pts',(-19.8564832755268,16.5712685161386,124.851295914385)) ;
#85496=CARTESIAN_POINT('Ctrl Pts',(-19.6007546274818,16.5812302315152,124.907216087891)) ;
#85497=CARTESIAN_POINT('Ctrl Pts',(-19.3374019357033,16.591258855088,124.917623305779)) ;
#85498=CARTESIAN_POINT('Ctrl Pts',(-19.0793392609636,16.6011692171544,124.882650735253)) ;
#85499=CARTESIAN_POINT('Ctrl Pts',(-18.8304294039593,16.6111039108068,124.803856446845)) ;
#85500=CARTESIAN_POINT('Ctrl Pts',(-18.596627686363,16.6211457539347,124.681515843378)) ;
#85501=CARTESIAN_POINT('Ctrl Pts',(-18.3907224983714,16.6310302595051,124.523120625139)) ;
#85502=CARTESIAN_POINT('Ctrl Pts',(-18.213179611499,16.6410323632903,124.329353348425)) ;
#85503=CARTESIAN_POINT('Ctrl Pts',(-18.0729347335421,16.6509507147053,124.109605240172)) ;
#85504=CARTESIAN_POINT('Ctrl Pts',(-17.9717684511152,16.6609983707262,123.865757550208)) ;
#85505=CARTESIAN_POINT('Ctrl Pts',(-17.9151801485084,16.6708695637544,123.612544609832)) ;
#85506=CARTESIAN_POINT('Ctrl Pts',(-17.9031486210089,16.6809352768979,123.348363900477)) ;
#85507=CARTESIAN_POINT('Ctrl Pts',(-17.9361680628292,16.6907877374706,123.091490849331)) ;
#85508=CARTESIAN_POINT('Ctrl Pts',(-18.041350571431,16.7042162001931,122.754758769299)) ;
#85509=CARTESIAN_POINT('Ctrl Pts',(-18.2267930848674,16.7172971477102,122.460500377085)) ;
#85510=CARTESIAN_POINT('Ctrl Pts',(-18.4863600281543,16.7307716459448,122.219764136354)) ;
#85511=CARTESIAN_POINT('Ctrl Pts',(-18.7036600720593,16.7406037495542,122.079903461464)) ;
#85512=CARTESIAN_POINT('Ctrl Pts',(-18.9447043729808,16.7505696526809,121.977589420528)) ;
#85513=CARTESIAN_POINT('Ctrl Pts',(-19.2015822289623,16.7605970619911,121.918702174221)) ;
#85514=CARTESIAN_POINT('Ctrl Pts',(-19.4616612966653,16.7705080933577,121.90540119112)) ;
#85515=CARTESIAN_POINT('Ctrl Pts',(-19.8072674417979,16.7837524009787,121.947145247852)) ;
#85516=CARTESIAN_POINT('Ctrl Pts',(-20.2188607320283,16.8004528836499,122.113061781685)) ;
#85517=CARTESIAN_POINT('Ctrl Pts',(-20.5455735820307,16.8169597128057,122.405977428994)) ;
#85518=CARTESIAN_POINT('Ctrl Pts',(-20.7373318770542,16.8302703410433,122.698474315006)) ;
#85519=CARTESIAN_POINT('Ctrl Pts',(-20.8410538416381,16.8402629045834,122.939759731386)) ;
#85520=CARTESIAN_POINT('Ctrl Pts',(-20.9012068159582,16.8502929875849,123.196350988495)) ;
#85521=CARTESIAN_POINT('Ctrl Pts',(-20.9212193192341,16.8634665915827,123.542025913649)) ;
#85522=CARTESIAN_POINT('Ctrl Pts',(-20.832303368653,16.8801042968141,123.975028581527)) ;
#85523=CARTESIAN_POINT('Ctrl Pts',(-20.5559527242748,16.8999860593815,124.425665773585)) ;
#85524=CARTESIAN_POINT('Ctrl Pts',(-20.2087278908941,16.916682411598,124.701769095248)) ;
#85525=CARTESIAN_POINT('Ctrl Pts',(-19.8917137009118,16.9298394393871,124.83996615317)) ;
#85526=CARTESIAN_POINT('Ctrl Pts',(-19.5501593226237,16.9432167940307,124.923024211938)) ;
#85527=CARTESIAN_POINT('Ctrl Pts',(-19.1108610444918,16.9597476282895,124.912764903616)) ;
#85528=CARTESIAN_POINT('Ctrl Pts',(-18.6161741406845,16.9797123180326,124.720936570403)) ;
#85529=CARTESIAN_POINT('Ctrl Pts',(-18.2178875673859,16.9996288114562,124.372240740112)) ;
#85530=CARTESIAN_POINT('Ctrl Pts',(-17.9619000053034,17.0195185308058,123.909658769635)) ;
#85531=CARTESIAN_POINT('Ctrl Pts',(-17.8790923718899,17.0395252604536,123.384478022634)) ;
#85532=CARTESIAN_POINT('Ctrl Pts',(-17.9792607793457,17.0593633141005,122.866706624068)) ;
#85533=CARTESIAN_POINT('Ctrl Pts',(-18.251654980879,17.0793566523141,122.410555995914)) ;
#85534=CARTESIAN_POINT('Ctrl Pts',(-18.6614413308425,17.0992394517207,122.076728435462)) ;
#85535=CARTESIAN_POINT('Ctrl Pts',(-19.1602498824996,17.1191316326394,121.901928665033)) ;
#85536=CARTESIAN_POINT('Ctrl Pts',(-19.6893506726758,17.1390338111345,121.906954280708)) ;
#85537=CARTESIAN_POINT('Ctrl Pts',(-20.1877372859541,17.1590711223382,122.094250728715)) ;
#85538=CARTESIAN_POINT('Ctrl Pts',(-20.5885147516778,17.1788835638791,122.436171529998)) ;
#85539=CARTESIAN_POINT('Ctrl Pts',(-20.8514859106502,17.198948804614,122.899836288904)) ;
#85540=CARTESIAN_POINT('Ctrl Pts',(-20.9395751047835,17.2187060094698,123.417764524091)) ;
#85541=CARTESIAN_POINT('Ctrl Pts',(-20.8451902721094,17.2387392821155,123.941511312625)) ;
#85542=CARTESIAN_POINT('Ctrl Pts',(-20.5803738327966,17.2585521905694,124.396949460866)) ;
#85543=CARTESIAN_POINT('Ctrl Pts',(-20.1731152784338,17.2785483366968,124.738041234505)) ;
#85544=CARTESIAN_POINT('Ctrl Pts',(-19.6769118272769,17.2984100899193,124.918872799759)) ;
#85545=CARTESIAN_POINT('Ctrl Pts',(-19.1436416860639,17.3184786070474,124.919193987262)) ;
#85546=CARTESIAN_POINT('Ctrl Pts',(-18.648109623505,17.3383094800442,124.739265310968)) ;
#85547=CARTESIAN_POINT('Ctrl Pts',(-18.2411319113203,17.3582313908609,124.40073894506)) ;
#85548=CARTESIAN_POINT('Ctrl Pts',(-17.9740323769222,17.3781608342962,123.94322080473)) ;
#85549=CARTESIAN_POINT('Ctrl Pts',(-17.8790250602224,17.3980705044126,123.422734778079)) ;
#85550=CARTESIAN_POINT('Ctrl Pts',(-17.9662662127267,17.4179438616755,122.901724773555)) ;
#85551=CARTESIAN_POINT('Ctrl Pts',(-18.2276294818176,17.4379353962934,122.439190238654)) ;
#85552=CARTESIAN_POINT('Ctrl Pts',(-18.6285734387837,17.4578010137041,122.095521594485)) ;
#85553=CARTESIAN_POINT('Ctrl Pts',(-19.1253152085356,17.4777819435324,121.907762643509)) ;
#85554=CARTESIAN_POINT('Ctrl Pts',(-19.6552200286643,17.4977204056155,121.901390129916)) ;
#85555=CARTESIAN_POINT('Ctrl Pts',(-20.1546489410619,17.5176125988372,122.075060293898)) ;
#85556=CARTESIAN_POINT('Ctrl Pts',(-20.5661552710587,17.5375833138726,122.410136115304)) ;
#85557=CARTESIAN_POINT('Ctrl Pts',(-20.837318013256,17.5573929855387,122.861593772204)) ;
#85558=CARTESIAN_POINT('Ctrl Pts',(-20.9394053743083,17.5773862022299,123.382882566089)) ;
#85559=CARTESIAN_POINT('Ctrl Pts',(-20.8584272459729,17.5972371144262,123.904456907226)) ;
#85560=CARTESIAN_POINT('Ctrl Pts',(-20.6013722647494,17.6173117207453,124.371835879059)) ;
#85561=CARTESIAN_POINT('Ctrl Pts',(-20.2709413387604,17.6338283526286,124.661087804809)) ;
#85562=CARTESIAN_POINT('Ctrl Pts',(-19.9567456572262,17.6471670603227,124.816311506479)) ;
#85563=CARTESIAN_POINT('Ctrl Pts',(-19.7085634180374,17.657009434631,124.889285728244)) ;
#85564=CARTESIAN_POINT('Ctrl Pts',(-19.4460346302332,17.6670644546137,124.918920394545)) ;
#85565=CARTESIAN_POINT('Ctrl Pts',(-19.0989340056819,17.6802966112713,124.897325675655)) ;
#85566=CARTESIAN_POINT('Ctrl Pts',(-18.6800921880835,17.6969115786164,124.757498322391)) ;
#85567=CARTESIAN_POINT('Ctrl Pts',(-18.3346383771164,17.7135061656276,124.483309875907)) ;
#85568=CARTESIAN_POINT('Ctrl Pts',(-18.1268953740658,17.726739733983,124.204383339548)) ;
#85569=CARTESIAN_POINT('Ctrl Pts',(-18.0083495823601,17.7367833517917,123.968592623646)) ;
#85570=CARTESIAN_POINT('Ctrl Pts',(-17.9336310060421,17.7466702760265,123.71972753629)) ;
#85571=CARTESIAN_POINT('Ctrl Pts',(-17.9024800444537,17.7566609304733,123.459055825321)) ;
#85572=CARTESIAN_POINT('Ctrl Pts',(-17.91707504202,17.7666226889273,123.197677226246)) ;
#85573=CARTESIAN_POINT('Ctrl Pts',(-17.9967448142101,17.7799625539945,122.856223951778)) ;
#85574=CARTESIAN_POINT('Ctrl Pts',(-18.1639793074523,17.7932713369078,122.544584740488)) ;
#85575=CARTESIAN_POINT('Ctrl Pts',(-18.4009261605596,17.8064670943519,122.291390427509)) ;
#85576=CARTESIAN_POINT('Ctrl Pts',(-18.6098409160699,17.8164289780284,122.133625520298)) ;
#85577=CARTESIAN_POINT('Ctrl Pts',(-18.8450658298774,17.826472087543,122.013949993326)) ;
#85578=CARTESIAN_POINT('Ctrl Pts',(-19.092621766734,17.8363243375422,121.938100172443)) ;
#85579=CARTESIAN_POINT('Ctrl Pts',(-19.3525817752957,17.8462958744927,121.905367673207)) ;
#85580=CARTESIAN_POINT('Ctrl Pts',(-19.6149678521797,17.8562911399702,121.918326097359)) ;
#85581=CARTESIAN_POINT('Ctrl Pts',(-19.8719764054818,17.8663251128439,121.977174194731)) ;
#85582=CARTESIAN_POINT('Ctrl Pts',(-20.1107443124788,17.8761805276062,122.07756701248)) ;
#85583=CARTESIAN_POINT('Ctrl Pts',(-20.3317665609879,17.886179805115,122.219601552815)) ;
#85584=CARTESIAN_POINT('Ctrl Pts',(-20.5230159036683,17.896074989278,122.39585448978)) ;
#85585=CARTESIAN_POINT('Ctrl Pts',(-20.6833174072794,17.9061353689188,122.60604307054)) ;
#85586=CARTESIAN_POINT('Ctrl Pts',(-20.8023179831757,17.9159852379269,122.835939812967)) ;
#85587=CARTESIAN_POINT('Ctrl Pts',(-20.8815806037002,17.9260167991348,123.08734301173)) ;
#85588=CARTESIAN_POINT('Ctrl Pts',(-20.9153942834191,17.9360272480171,123.348249186297)) ;
#85589=CARTESIAN_POINT('Ctrl Pts',(-20.9038056440646,17.9459339874341,123.608321329956)) ;
#85590=CARTESIAN_POINT('Ctrl Pts',(-20.8475549821368,17.9558720035025,123.863336913945)) ;
#85591=CARTESIAN_POINT('Ctrl Pts',(-20.7473491124227,17.9658772499537,124.106450718163)) ;
#85592=CARTESIAN_POINT('Ctrl Pts',(-20.6056897092289,17.97591131101,124.328835897672)) ;
#85593=CARTESIAN_POINT('Ctrl Pts',(-20.4312337067048,17.9857563920681,124.519908095883)) ;
#85594=CARTESIAN_POINT('Ctrl Pts',(-20.2236664013566,17.9957421980216,124.680396433313)) ;
#85595=CARTESIAN_POINT('Ctrl Pts',(-19.992579689612,18.0056770185758,124.801991034309)) ;
#85596=CARTESIAN_POINT('Ctrl Pts',(-19.7408295621782,18.015734543708,124.882346278087)) ;
#85597=CARTESIAN_POINT('Ctrl Pts',(-19.4850812770158,18.0255561943594,124.917339204616)) ;
#85598=CARTESIAN_POINT('Ctrl Pts',(-19.2210175734843,18.0356122578641,124.907651917327)) ;
#85599=CARTESIAN_POINT('Ctrl Pts',(-18.9656796380445,18.045552924928,124.85243013731)) ;
#85600=CARTESIAN_POINT('Ctrl Pts',(-18.7243886052584,18.055457318594,124.754831562349)) ;
#85601=CARTESIAN_POINT('Ctrl Pts',(-18.5006574893832,18.065503842357,124.61470975614)) ;
#85602=CARTESIAN_POINT('Ctrl Pts',(-18.307369291185,18.0753999253734,124.440656203214)) ;
#85603=CARTESIAN_POINT('Ctrl Pts',(-18.1445872821212,18.0854666246034,124.232186912263)) ;
#85604=CARTESIAN_POINT('Ctrl Pts',(-18.0231672453592,18.0952902350045,124.004324151478)) ;
#85605=CARTESIAN_POINT('Ctrl Pts',(-17.9408459619243,18.105346095182,123.753251808151)) ;
#85606=CARTESIAN_POINT('Ctrl Pts',(-17.9041508391774,18.1152792414869,123.494778928388)) ;
#85607=CARTESIAN_POINT('Ctrl Pts',(-17.9123669611964,18.1252244972575,123.233587463902)) ;
#85608=CARTESIAN_POINT('Ctrl Pts',(-17.965820602866,18.135207795696,122.976706518041)) ;
#85609=CARTESIAN_POINT('Ctrl Pts',(-18.063904304486,18.1452449758426,122.731876350353)) ;
#85610=CARTESIAN_POINT('Ctrl Pts',(-18.2001593676184,18.1550995285521,122.511623169625)) ;
#85611=CARTESIAN_POINT('Ctrl Pts',(-18.3748041349657,18.1650990469994,122.315340175389)) ;
#85612=CARTESIAN_POINT('Ctrl Pts',(-18.5786232758408,18.1749941294615,122.153792991792)) ;
#85613=CARTESIAN_POINT('Ctrl Pts',(-18.8111647901301,18.1850546749676,122.028081402506)) ;
#85614=CARTESIAN_POINT('Ctrl Pts',(-19.0567404030301,18.1949039822156,121.94625334283)) ;
#85615=CARTESIAN_POINT('Ctrl Pts',(-19.3172903973273,18.204931072303,121.906964506293)) ;
#85616=CARTESIAN_POINT('Ctrl Pts',(-19.5807510422382,18.2149599764399,121.914213939927)) ;
#85617=CARTESIAN_POINT('Ctrl Pts',(-19.8342692925352,18.2248038415392,121.965616328592)) ;
#85618=CARTESIAN_POINT('Ctrl Pts',(-20.0789732695833,18.2347996682476,122.061118208397)) ;
#85619=CARTESIAN_POINT('Ctrl Pts',(-20.3037898720174,18.2448248848966,122.198476327115)) ;
#85620=CARTESIAN_POINT('Ctrl Pts',(-20.4989049499709,18.2547147170542,122.37016702887)) ;
#85621=CARTESIAN_POINT('Ctrl Pts',(-20.6631753421901,18.2647055731389,122.574966335763)) ;
#85622=CARTESIAN_POINT('Ctrl Pts',(-20.788773377905,18.2746506677318,122.804154170433)) ;
#85623=CARTESIAN_POINT('Ctrl Pts',(-20.8731939482788,18.2846025714999,123.051690442556)) ;
#85624=CARTESIAN_POINT('Ctrl Pts',(-20.9134619567521,18.2946389709693,123.312337432225)) ;
#85625=CARTESIAN_POINT('Ctrl Pts',(-20.9081339354844,18.304528041058,123.572166354225)) ;
#85626=CARTESIAN_POINT('Ctrl Pts',(-20.8577276976876,18.3145173304289,123.829783197126)) ;
#85627=CARTESIAN_POINT('Ctrl Pts',(-20.7634652567705,18.3244758966386,124.073909818492)) ;
#85628=CARTESIAN_POINT('Ctrl Pts',(-20.6295842577516,18.3343754678554,124.296985254271)) ;
#85629=CARTESIAN_POINT('Ctrl Pts',(-20.4564060477001,18.3444233822697,124.496275231277)) ;
#85630=CARTESIAN_POINT('Ctrl Pts',(-20.2544457726215,18.3543187251302,124.660147079943)) ;
#85631=CARTESIAN_POINT('Ctrl Pts',(-20.0233589167788,18.3643804190777,124.788582887775)) ;
#85632=CARTESIAN_POINT('Ctrl Pts',(-19.7788516309637,18.3742248721618,124.873135508736)) ;
#85633=CARTESIAN_POINT('Ctrl Pts',(-19.5205311753707,18.3841855571203,124.915333903471)) ;
#85634=CARTESIAN_POINT('Ctrl Pts',(-19.2568158507944,18.3942214896288,124.91156959599)) ;
#85635=CARTESIAN_POINT('Ctrl Pts',(-19.0015267672572,18.4041101053169,124.863056912793)) ;
#85636=CARTESIAN_POINT('Ctrl Pts',(-18.7552413200576,18.4141245144593,124.770264913515)) ;
#85637=CARTESIAN_POINT('Ctrl Pts',(-18.5287491933341,18.4241583234171,124.635287434208)) ;
#85638=CARTESIAN_POINT('Ctrl Pts',(-18.3326736838035,18.4339887776733,124.467040337069)) ;
#85639=CARTESIAN_POINT('Ctrl Pts',(-18.1646552309895,18.4440664452515,124.262399712302)) ;
#85640=CARTESIAN_POINT('Ctrl Pts',(-18.0374628156085,18.4539183133737,124.036835965427)) ;
#85641=CARTESIAN_POINT('Ctrl Pts',(-17.9492624861745,18.4639913509391,123.787301761498)) ;
#85642=CARTESIAN_POINT('Ctrl Pts',(-17.9067521481246,18.47383390429,123.532143869047)) ;
#85643=CARTESIAN_POINT('Ctrl Pts',(-17.9083434021815,18.4838142997834,123.269885593791)) ;
#85644=CARTESIAN_POINT('Ctrl Pts',(-17.9561323187471,18.4938327777612,123.010990190508)) ;
#85645=CARTESIAN_POINT('Ctrl Pts',(-18.0463999219275,18.5037160920673,122.767424084949)) ;
#85646=CARTESIAN_POINT('Ctrl Pts',(-18.1801054394556,18.513784394606,122.53915993018)) ;
#85647=CARTESIAN_POINT('Ctrl Pts',(-18.3471840847822,18.5236144418794,122.342083268111)) ;
#85648=CARTESIAN_POINT('Ctrl Pts',(-18.5504477114517,18.5336813132949,122.172834206145)) ;
#85649=CARTESIAN_POINT('Ctrl Pts',(-18.7760961055222,18.543570352094,122.043850044035)) ;
#85650=CARTESIAN_POINT('Ctrl Pts',(-19.0231397001699,18.5535670502281,121.954587201367)) ;
#85651=CARTESIAN_POINT('Ctrl Pts',(-19.2808470530102,18.5635194759401,121.909875533707)) ;
#85652=CARTESIAN_POINT('Ctrl Pts',(-19.5420744376569,18.573460778173,121.910226123319)) ;
#85653=CARTESIAN_POINT('Ctrl Pts',(-19.8004561957054,18.5834440172569,121.955853427861)) ;
#85654=CARTESIAN_POINT('Ctrl Pts',(-20.048172080969,18.5934828188255,122.046518326737)) ;
#85655=CARTESIAN_POINT('Ctrl Pts',(-20.2723410125305,18.6033309249472,122.17589057555)) ;
#85656=CARTESIAN_POINT('Ctrl Pts',(-20.4750350377161,18.6133911205225,122.345583287443)) ;
#85657=CARTESIAN_POINT('Ctrl Pts',(-20.6422769769176,18.6232888038339,122.544802617581)) ;
#85658=CARTESIAN_POINT('Ctrl Pts',(-20.7735588255307,18.6332198442079,122.770350862156)) ;
#85659=CARTESIAN_POINT('Ctrl Pts',(-20.8644257386545,18.6432620618645,123.018108220622)) ;
#85660=CARTESIAN_POINT('Ctrl Pts',(-20.9103608198524,18.6531487225985,123.2738391975)) ;
#85661=CARTESIAN_POINT('Ctrl Pts',(-20.9116439914806,18.663141831201,123.536431039595)) ;
#85662=CARTESIAN_POINT('Ctrl Pts',(-20.8674236850463,18.6730875298392,123.794025919388)) ;
#85663=CARTESIAN_POINT('Ctrl Pts',(-20.7796339406571,18.6830347521103,124.040260003737)) ;
#85664=CARTESIAN_POINT('Ctrl Pts',(-20.648865853499,18.6930827776904,124.269647102596)) ;
#85665=CARTESIAN_POINT('Ctrl Pts',(-20.4837880164837,18.7029300248333,124.468930982032)) ;
#85666=CARTESIAN_POINT('Ctrl Pts',(-20.2848353076597,18.712893201924,124.639124066068)) ;
#85667=CARTESIAN_POINT('Ctrl Pts',(-20.057643225627,18.7229229229575,124.772734603442)) ;
#85668=CARTESIAN_POINT('Ctrl Pts',(-19.8138733025437,18.7328273904903,124.864024891333)) ;
#85669=CARTESIAN_POINT('Ctrl Pts',(-19.5549244555012,18.7428518763201,124.91225661059)) ;
#85670=CARTESIAN_POINT('Ctrl Pts',(-19.2946394655604,18.752755711444,124.914979535986)) ;
#85671=CARTESIAN_POINT('Ctrl Pts',(-19.0340712151648,18.762806902154,124.871903053952)) ;
#85672=CARTESIAN_POINT('Ctrl Pts',(-18.7890046631621,18.7726913448123,124.785719653912)) ;
#85673=CARTESIAN_POINT('Ctrl Pts',(-18.5599429927726,18.7826843526642,124.657344067074)) ;
#85674=CARTESIAN_POINT('Ctrl Pts',(-18.3575852293697,18.7926326723805,124.491794444498)) ;
#85675=CARTESIAN_POINT('Ctrl Pts',(-18.1869857767214,18.8025695110899,124.294126119609)) ;
#85676=CARTESIAN_POINT('Ctrl Pts',(-18.0523654033191,18.8125525000095,124.068917991237)) ;
#85677=CARTESIAN_POINT('Ctrl Pts',(-17.9588008233373,18.8225963793736,123.822148861517)) ;
#85678=CARTESIAN_POINT('Ctrl Pts',(-17.9099472787027,18.832424444732,123.568497660891)) ;
#85679=CARTESIAN_POINT('Ctrl Pts',(-17.9056636523394,18.8425015332869,123.303776150982)) ;
#85680=CARTESIAN_POINT('Ctrl Pts',(-17.9463206545568,18.8523516854432,123.048068626949)) ;
#85681=CARTESIAN_POINT('Ctrl Pts',(-18.0325884242925,18.8624321658956,122.797675319086)) ;
#85682=CARTESIAN_POINT('Ctrl Pts',(-18.1574960786457,18.8722466636644,122.571957568326)) ;
#85683=CARTESIAN_POINT('Ctrl Pts',(-18.3234918042426,18.8823149596845,122.366002659658)) ;
#85684=CARTESIAN_POINT('Ctrl Pts',(-18.5195168321674,18.8922137921673,122.194898302409)) ;
#85685=CARTESIAN_POINT('Ctrl Pts',(-18.7455899254507,18.9022666721818,122.058322027411)) ;
#85686=CARTESIAN_POINT('Ctrl Pts',(-18.9874685791596,18.912136487678,121.96454261231)) ;
#85687=CARTESIAN_POINT('Ctrl Pts',(-19.247074514884,18.9222091687608,121.913098195303)) ;
#85688=CARTESIAN_POINT('Ctrl Pts',(-19.5054282253465,18.9320416473318,121.907540984529)) ;
#85689=CARTESIAN_POINT('Ctrl Pts',(-19.7660476083419,18.9420722813179,121.946964015993)) ;
#85690=CARTESIAN_POINT('Ctrl Pts',(-20.015663124333,18.952103838537,122.031786628564)) ;
#85691=CARTESIAN_POINT('Ctrl Pts',(-20.242340733487,18.9619335474087,122.155620704585)) ;
#85692=CARTESIAN_POINT('Ctrl Pts',(-20.4478596794803,18.9719229962108,122.318956902595)) ;
#85693=CARTESIAN_POINT('Ctrl Pts',(-20.6223353947974,18.9819668486108,122.517002479713)) ;
#85694=CARTESIAN_POINT('Ctrl Pts',(-20.7571909721581,18.9917885619429,122.737075061606)) ;
#85695=CARTESIAN_POINT('Ctrl Pts',(-20.8544420213186,19.0018235669316,122.982196100149)) ;
#85696=CARTESIAN_POINT('Ctrl Pts',(-20.9068867752531,19.0118484053792,123.24037432519)) ;
#85697=CARTESIAN_POINT('Ctrl Pts',(-20.9141429657687,19.0217006183344,123.499179168148)) ;
#85698=CARTESIAN_POINT('Ctrl Pts',(-20.8762673910892,19.0316905745282,123.758937854536)) ;
#85699=CARTESIAN_POINT('Ctrl Pts',(-20.7943862514496,19.0416186848114,124.00666549439)) ;
#85700=CARTESIAN_POINT('Ctrl Pts',(-20.6703510230735,19.051607284891,124.238008956621)) ;
#85701=CARTESIAN_POINT('Ctrl Pts',(-20.5071291776537,19.0616338768185,124.444859269663)) ;
#85702=CARTESIAN_POINT('Ctrl Pts',(-20.3134350002054,19.0715190048827,124.617949216475)) ;
#85703=CARTESIAN_POINT('Ctrl Pts',(-20.0905630047009,19.0815101223562,124.756761630848)) ;
#85704=CARTESIAN_POINT('Ctrl Pts',(-19.8455702342905,19.091550738208,124.854732580101)) ;
#85705=CARTESIAN_POINT('Ctrl Pts',(-19.5927186533089,19.1013837290617,124.907978535889)) ;
#85706=CARTESIAN_POINT('Ctrl Pts',(-19.3302830880624,19.111376860512,124.917403980521)) ;
#85707=CARTESIAN_POINT('Ctrl Pts',(-19.0692443271857,19.1214089089474,124.880431822587)) ;
#85708=CARTESIAN_POINT('Ctrl Pts',(-18.8226828953735,19.1312741554898,124.800366929372)) ;
#85709=CARTESIAN_POINT('Ctrl Pts',(-18.5911601979227,19.1412360303166,124.678161518773)) ;
#85710=CARTESIAN_POINT('Ctrl Pts',(-18.3831390570505,19.1512709934279,124.516107567008)) ;
#85711=CARTESIAN_POINT('Ctrl Pts',(-18.2086970669107,19.1611558378903,124.323580061315)) ;
#85712=CARTESIAN_POINT('Ctrl Pts',(-18.0679004045374,19.171221890731,124.099692955036)) ;
#85713=CARTESIAN_POINT('Ctrl Pts',(-17.9700782692514,19.18105940664,123.860343413881)) ;
#85714=CARTESIAN_POINT('Ctrl Pts',(-17.9137587529611,19.1911281547489,123.601857544703)) ;
#85715=CARTESIAN_POINT('Ctrl Pts',(-17.9034670306657,19.2010086717799,123.342371871998)) ;
#85716=CARTESIAN_POINT('Ctrl Pts',(-17.9382401306853,19.2109998587144,123.08216562488)) ;
#85717=CARTESIAN_POINT('Ctrl Pts',(-18.017346517817,19.2209529249893,122.83281725219)) ;
#85718=CARTESIAN_POINT('Ctrl Pts',(-18.1396020443988,19.2309887625219,122.599158531839)) ;
#85719=CARTESIAN_POINT('Ctrl Pts',(-18.2981172600277,19.2408788887333,122.393170709056)) ;
#85720=CARTESIAN_POINT('Ctrl Pts',(-18.4916634610177,19.2508710706413,122.215735660309)) ;
#85721=CARTESIAN_POINT('Ctrl Pts',(-18.7121126054784,19.2608170105799,122.075322038536)) ;
#85722=CARTESIAN_POINT('Ctrl Pts',(-18.9534330921312,19.270764194344,121.974810909958)) ;
#85723=CARTESIAN_POINT('Ctrl Pts',(-19.2111660245585,19.2808121326514,121.917443070718)) ;
#85724=CARTESIAN_POINT('Ctrl Pts',(-19.46968806927,19.2906597673917,121.905712436638)) ;
#85725=CARTESIAN_POINT('Ctrl Pts',(-19.7293828802566,19.3006214813655,121.938618525281)) ;
#85726=CARTESIAN_POINT('Ctrl Pts',(-19.9810273924312,19.3106501161564,122.01696448955)) ;
#85727=CARTESIAN_POINT('Ctrl Pts',(-20.2124964374937,19.3205604347535,122.136300351223)) ;
#85728=CARTESIAN_POINT('Ctrl Pts',(-20.4206742458988,19.330495291065,122.293871266416)) ;
#85729=CARTESIAN_POINT('Ctrl Pts',(-20.6000312207341,19.3405365270257,122.487400631673)) ;
#85730=CARTESIAN_POINT('Ctrl Pts',(-20.7410617512557,19.3504232986057,122.705636493677)) ;
#85731=CARTESIAN_POINT('Ctrl Pts',(-20.8434829085783,19.3604234773119,122.947608430064)) ;
#85732=CARTESIAN_POINT('Ctrl Pts',(-20.9020842657226,19.3703407555215,123.201594819178)) ;
#85733=CARTESIAN_POINT('Ctrl Pts',(-20.9157885273105,19.3803880019352,123.465233400112)) ;
#85734=CARTESIAN_POINT('Ctrl Pts',(-20.8843312394049,19.3902618909165,123.722835831488)) ;
#85735=CARTESIAN_POINT('Ctrl Pts',(-20.8073413256974,19.400323908497,123.975764420132)) ;
#85736=CARTESIAN_POINT('Ctrl Pts',(-20.6898211294301,19.4101949702313,124.207038033062)) ;
#85737=CARTESIAN_POINT('Ctrl Pts',(-20.5325845494946,19.4201890335916,124.417401603479)) ;
#85738=CARTESIAN_POINT('Ctrl Pts',(-20.3400856995338,19.430221191625,124.59752229965)) ;
#85739=CARTESIAN_POINT('Ctrl Pts',(-20.1232221891283,19.4400850678652,124.739562342653)) ;
#85740=CARTESIAN_POINT('Ctrl Pts',(-19.8800650899672,19.4501555825034,124.843936496975)) ;
#85741=CARTESIAN_POINT('Ctrl Pts',(-19.6283151955898,19.4599962194444,124.903158307787)) ;
#85742=CARTESIAN_POINT('Ctrl Pts',(-19.3668809125715,19.4699633482846,124.91881772904)) ;
#85743=CARTESIAN_POINT('Ctrl Pts',(-19.1054682843621,19.4799773214091,124.888425374719)) ;
#85744=CARTESIAN_POINT('Ctrl Pts',(-18.7709161948087,19.4932620552724,124.788603773578)) ;
#85745=CARTESIAN_POINT('Ctrl Pts',(-18.4713172138264,19.5064873199872,124.604876555852)) ;
#85746=CARTESIAN_POINT('Ctrl Pts',(-18.2302531727005,19.519797842542,124.351369013514)) ;
#85747=CARTESIAN_POINT('Ctrl Pts',(-18.0847512811712,19.5298264874442,124.131644354945)) ;
#85748=CARTESIAN_POINT('Ctrl Pts',(-17.9809400631191,19.5397075197981,123.89362910154)) ;
#85749=CARTESIAN_POINT('Ctrl Pts',(-17.9188886192552,19.5496884924782,123.638788056693)) ;
#85750=CARTESIAN_POINT('Ctrl Pts',(-17.902254691945,19.5596696200642,123.377037428699)) ;
#85751=CARTESIAN_POINT('Ctrl Pts',(-17.9400916999754,19.5729128103256,123.031015386685)) ;
#85752=CARTESIAN_POINT('Ctrl Pts',(-18.1006952198866,19.5895808056864,122.618253916938)) ;
#85753=CARTESIAN_POINT('Ctrl Pts',(-18.3897868588537,19.6061013056984,122.287674714517)) ;
#85754=CARTESIAN_POINT('Ctrl Pts',(-18.6800761568763,19.6194143220144,122.092482801336)) ;
#85755=CARTESIAN_POINT('Ctrl Pts',(-18.9182029603172,19.6293308802474,121.986519910248)) ;
#85756=CARTESIAN_POINT('Ctrl Pts',(-19.1738678812539,19.6393585485503,121.922922940547)) ;
#85757=CARTESIAN_POINT('Ctrl Pts',(-19.5194780323658,19.652539138295,121.898097021449)) ;
#85758=CARTESIAN_POINT('Ctrl Pts',(-19.9563288314783,19.6692872774143,121.982471851941)) ;
#85759=CARTESIAN_POINT('Ctrl Pts',(-20.4082007931077,19.6890820199249,122.252403503244)) ;
#85760=CARTESIAN_POINT('Ctrl Pts',(-20.7451774511471,19.7091264127337,122.664799510157)) ;
#85761=CARTESIAN_POINT('Ctrl Pts',(-20.9190665009058,19.7289655950324,123.162745067453)) ;
#85762=CARTESIAN_POINT('Ctrl Pts',(-20.9138754834601,19.7488909187253,123.692173591397)) ;
#85763=CARTESIAN_POINT('Ctrl Pts',(-20.7282061366091,19.7688145567768,124.188186165143)) ;
#85764=CARTESIAN_POINT('Ctrl Pts',(-20.384618994923,19.7887394302423,124.591086031158)) ;
#85765=CARTESIAN_POINT('Ctrl Pts',(-19.9254980781481,19.8086180373213,124.852590538209)) ;
#85766=CARTESIAN_POINT('Ctrl Pts',(-19.4021944235472,19.8285954801532,124.942415684017)) ;
#85767=CARTESIAN_POINT('Ctrl Pts',(-18.8808504945977,19.8485273282379,124.848110950266)) ;
#85768=CARTESIAN_POINT('Ctrl Pts',(-18.4236327836799,19.8684225965805,124.582537401173)) ;
#85769=CARTESIAN_POINT('Ctrl Pts',(-18.0835396042065,19.8883450949926,124.176670177314)) ;
#85770=CARTESIAN_POINT('Ctrl Pts',(-17.9021501379471,19.9083045768686,123.678122009356)) ;
#85771=CARTESIAN_POINT('Ctrl Pts',(-17.9016826808945,19.928182329328,123.14988706624)) ;
#85772=CARTESIAN_POINT('Ctrl Pts',(-18.0801848929392,19.9480641200625,122.652414260717)) ;
#85773=CARTESIAN_POINT('Ctrl Pts',(-18.4216899540666,19.9681374589135,122.242615414334)) ;
#85774=CARTESIAN_POINT('Ctrl Pts',(-18.8764503196767,19.9879419261493,121.977339845321)) ;
#85775=CARTESIAN_POINT('Ctrl Pts',(-19.398725666126,20.0079252665571,121.881194515216)) ;
#85776=CARTESIAN_POINT('Ctrl Pts',(-19.9205991086772,20.0278402311551,121.96959503457)) ;
#85777=CARTESIAN_POINT('Ctrl Pts',(-20.3807214883969,20.0477087658715,122.228929102253)) ;
#85778=CARTESIAN_POINT('Ctrl Pts',(-20.7270865861408,20.0677611500832,122.633789392997)) ;
#85779=CARTESIAN_POINT('Ctrl Pts',(-20.9126916804623,20.0875351138724,123.125708607321)) ;
#85780=CARTESIAN_POINT('Ctrl Pts',(-20.9197926939565,20.1075894928938,123.658461280195)) ;
#85781=CARTESIAN_POINT('Ctrl Pts',(-20.7466018541178,20.127386230467,124.1554690317)) ;
#85782=CARTESIAN_POINT('Ctrl Pts',(-20.4126503321151,20.1473540428185,124.567785296605)) ;
#85783=CARTESIAN_POINT('Ctrl Pts',(-19.9576268829892,20.1673130188835,124.840673205932)) ;
#85784=CARTESIAN_POINT('Ctrl Pts',(-19.4386508322908,20.1872079371609,124.94188751217)) ;
#85785=CARTESIAN_POINT('Ctrl Pts',(-18.9161782831837,20.2071042496112,124.860571732585)) ;
#85786=CARTESIAN_POINT('Ctrl Pts',(-18.4521872012561,20.2270121829853,124.606170401089)) ;
#85787=CARTESIAN_POINT('Ctrl Pts',(-18.1022237455605,20.2469620732738,124.207890683089)) ;
#85788=CARTESIAN_POINT('Ctrl Pts',(-17.9093454009066,20.2668393037751,123.715999312751)) ;
#85789=CARTESIAN_POINT('Ctrl Pts',(-17.8955608540406,20.2868219726461,123.185097942073)) ;
#85790=CARTESIAN_POINT('Ctrl Pts',(-18.0637245954641,20.3067548592265,122.682641570739)) ;
#85791=CARTESIAN_POINT('Ctrl Pts',(-18.3925761888793,20.3266676052444,122.268015072213)) ;
#85792=CARTESIAN_POINT('Ctrl Pts',(-18.7672875195584,20.3432373265862,122.036639218976)) ;
#85793=CARTESIAN_POINT('Ctrl Pts',(-19.1020112523894,20.3565373378912,121.93602784581)) ;
#85794=CARTESIAN_POINT('Ctrl Pts',(-19.4482933884682,20.3698075256411,121.894667854607)) ;
#85795=CARTESIAN_POINT('Ctrl Pts',(-19.8857616860693,20.3864349080065,121.957330261882)) ;
#85796=CARTESIAN_POINT('Ctrl Pts',(-20.2753843629908,20.4030571977517,122.165611719854)) ;
#85797=CARTESIAN_POINT('Ctrl Pts',(-20.5295904307739,20.4163024121462,122.403368996714)) ;
#85798=CARTESIAN_POINT('Ctrl Pts',(-20.6866680641732,20.4262143771069,122.61117509767)) ;
#85799=CARTESIAN_POINT('Ctrl Pts',(-20.806737474672,20.4362730002714,122.846628519742)) ;
#85800=CARTESIAN_POINT('Ctrl Pts',(-20.8828053848385,20.4461131143872,123.093815056759)) ;
#85801=CARTESIAN_POINT('Ctrl Pts',(-20.9157850235484,20.4561788993448,123.356230024175)) ;
#85802=CARTESIAN_POINT('Ctrl Pts',(-20.9028213821857,20.4660622171327,123.615663268066)) ;
#85803=CARTESIAN_POINT('Ctrl Pts',(-20.8449589694743,20.4760516549913,123.871692434311)) ;
#85804=CARTESIAN_POINT('Ctrl Pts',(-20.74368006627,20.486015369044,124.113161475895)) ;
#85805=CARTESIAN_POINT('Ctrl Pts',(-20.6017961937113,20.4960103807032,124.334224144279)) ;
#85806=CARTESIAN_POINT('Ctrl Pts',(-20.4226668968658,20.5060466723975,124.527786878245)) ;
#85807=CARTESIAN_POINT('Ctrl Pts',(-20.2168574908497,20.5158930500909,124.684641027028)) ;
#85808=CARTESIAN_POINT('Ctrl Pts',(-19.9839816914647,20.5258779942416,124.805469402538)) ;
#85809=CARTESIAN_POINT('Ctrl Pts',(-19.7348364121739,20.5358149653716,124.883819573151)) ;
#85810=CARTESIAN_POINT('Ctrl Pts',(-19.4729804417369,20.5458647500033,124.917956892684)) ;
#85811=CARTESIAN_POINT('Ctrl Pts',(-19.2143536333705,20.5557152120808,124.906538794214)) ;
#85812=CARTESIAN_POINT('Ctrl Pts',(-18.9584230841274,20.5656872256012,124.850373618486)) ;
#85813=CARTESIAN_POINT('Ctrl Pts',(-18.7155134690777,20.5756823727206,124.75033150436)) ;
#85814=CARTESIAN_POINT('Ctrl Pts',(-18.4930284866175,20.5857163424567,124.608850714625)) ;
#85815=CARTESIAN_POINT('Ctrl Pts',(-18.301639069362,20.5955718881273,124.43432218421)) ;
#85816=CARTESIAN_POINT('Ctrl Pts',(-18.1409105781554,20.6055706451405,124.22651165924)) ;
#85817=CARTESIAN_POINT('Ctrl Pts',(-18.0196900933075,20.6154677803777,123.996357848347)) ;
#85818=CARTESIAN_POINT('Ctrl Pts',(-17.9389969296105,20.6255208762173,123.744826815494)) ;
#85819=CARTESIAN_POINT('Ctrl Pts',(-17.9037758541384,20.6354043849479,123.487479681158)) ;
#85820=CARTESIAN_POINT('Ctrl Pts',(-17.9132711224096,20.645399257594,123.225004546721)) ;
#85821=CARTESIAN_POINT('Ctrl Pts',(-17.9687399657228,20.6554192192297,122.96758422729)) ;
#85822=CARTESIAN_POINT('Ctrl Pts',(-18.0667172219578,20.6653245830296,122.726428828135)) ;
#85823=CARTESIAN_POINT('Ctrl Pts',(-18.2051112656729,20.6752651706371,122.504892851635)) ;
#85824=CARTESIAN_POINT('Ctrl Pts',(-18.3808832318701,20.6852679887378,122.309400454705)) ;
#85825=CARTESIAN_POINT('Ctrl Pts',(-18.5888185798447,20.6953027004619,122.147247116949)) ;
#85826=CARTESIAN_POINT('Ctrl Pts',(-18.8171665168026,20.7051476071992,122.025597143536)) ;
#85827=CARTESIAN_POINT('Ctrl Pts',(-19.0664811329135,20.7151334597682,121.943845159401)) ;
#85828=CARTESIAN_POINT('Ctrl Pts',(-19.3249386776779,20.7250682681813,121.906617308344)) ;
#85829=CARTESIAN_POINT('Ctrl Pts',(-19.5890636684313,20.7351257952623,121.915166166779)) ;
#85830=CARTESIAN_POINT('Ctrl Pts',(-19.8417720817048,20.7449474502594,121.967799082809)) ;
#85831=CARTESIAN_POINT('Ctrl Pts',(-20.0873597067846,20.7550034944324,122.065317687553)) ;
#85832=CARTESIAN_POINT('Ctrl Pts',(-20.3094854721539,20.7649442344776,122.202825084637)) ;
#85833=CARTESIAN_POINT('Ctrl Pts',(-20.5041808420828,20.7748483555505,122.375555985901)) ;
#85834=CARTESIAN_POINT('Ctrl Pts',(-20.6681287825517,20.7848958967047,122.582504505087)) ;
#85835=CARTESIAN_POINT('Ctrl Pts',(-20.7919881814226,20.7947946483051,122.811292280779)) ;
#85836=CARTESIAN_POINT('Ctrl Pts',(-20.8755740195429,20.8048431272709,123.061746962003)) ;
#85837=CARTESIAN_POINT('Ctrl Pts',(-20.9138090117843,20.8147306243546,123.318779270284)) ;
#85838=CARTESIAN_POINT('Ctrl Pts',(-20.9072479453517,20.8247237146527,123.581282226704)) ;
#85839=CARTESIAN_POINT('Ctrl Pts',(-20.8553241322653,20.834675884713,123.837624769112)) ;
#85840=CARTESIAN_POINT('Ctrl Pts',(-20.7601574063262,20.8446143046275,124.080820832448)) ;
#85841=CARTESIAN_POINT('Ctrl Pts',(-20.6237998714096,20.8545994347131,124.305038244249)) ;
#85842=CARTESIAN_POINT('Ctrl Pts',(-20.4494221518513,20.8646361241272,124.502900480269)) ;
#85843=CARTESIAN_POINT('Ctrl Pts',(-20.2473013388322,20.8744908081197,124.664842526609)) ;
#85844=CARTESIAN_POINT('Ctrl Pts',(-20.0170290666669,20.8844902921675,124.7913425284)) ;
#85845=CARTESIAN_POINT('Ctrl Pts',(-19.7708926225284,20.8943853809444,124.875346148885)) ;
#85846=CARTESIAN_POINT('Ctrl Pts',(-19.5096857275806,20.9044459355906,124.915966548158)) ;
#85847=CARTESIAN_POINT('Ctrl Pts',(-19.2508869429393,20.9142951999635,124.910873014686)) ;
#85848=CARTESIAN_POINT('Ctrl Pts',(-18.9922127135504,20.9243224524113,124.860678227348)) ;
#85849=CARTESIAN_POINT('Ctrl Pts',(-18.7463889477668,20.9343507499815,124.765668763576)) ;
#85850=CARTESIAN_POINT('Ctrl Pts',(-18.5246560820803,20.9441968789875,124.632331993503)) ;
#85851=CARTESIAN_POINT('Ctrl Pts',(-18.3260748632208,20.9541907843496,124.460462272426)) ;
#85852=CARTESIAN_POINT('Ctrl Pts',(-18.1602131738219,20.9642148820326,124.255803821438)) ;
#85853=CARTESIAN_POINT('Ctrl Pts',(-18.0338336778558,20.9741047098866,124.028700863845)) ;
#85854=CARTESIAN_POINT('Ctrl Pts',(-17.9475715523185,20.9840966913171,123.780706945075)) ;
#85855=CARTESIAN_POINT('Ctrl Pts',(-17.9059277190108,20.9940436960829,123.522648076826)) ;
#85856=CARTESIAN_POINT('Ctrl Pts',(-17.9092446774268,21.0039933474727,123.26119173999)) ;
#85857=CARTESIAN_POINT('Ctrl Pts',(-17.9585439446535,21.0140303504501,123.002085877506)) ;
#85858=CARTESIAN_POINT('Ctrl Pts',(-18.0505382977171,21.0239192588851,122.759033267901)) ;
#85859=CARTESIAN_POINT('Ctrl Pts',(-18.1842691504711,21.0339085913626,122.533148901569)) ;
#85860=CARTESIAN_POINT('Ctrl Pts',(-18.3548109388882,21.0438671467997,122.334658060956)) ;
#85861=CARTESIAN_POINT('Ctrl Pts',(-18.5556391649582,21.0537667180002,122.16926520889)) ;
#85862=CARTESIAN_POINT('Ctrl Pts',(-18.7855363124599,21.0638146432522,122.039439979611)) ;
#85863=CARTESIAN_POINT('Ctrl Pts',(-19.030698238794,21.0737099427782,121.952623471748)) ;
#85864=CARTESIAN_POINT('Ctrl Pts',(-19.291450065471,21.0837717992262,121.908950298832)) ;
#85865=CARTESIAN_POINT('Ctrl Pts',(-19.5501399989178,21.0936156456428,121.91111408291)) ;
#85866=CARTESIAN_POINT('Ctrl Pts',(-19.807740031436,21.1035785947709,121.957838664783)) ;
#85867=CARTESIAN_POINT('Ctrl Pts',(-20.0549347555783,21.1136126311989,122.049642784503)) ;
#85868=CARTESIAN_POINT('Ctrl Pts',(-20.2792391844421,21.1235000581569,122.180784673848)) ;
#85869=CARTESIAN_POINT('Ctrl Pts',(-20.4802501125778,21.1335144924933,122.350672310585)) ;
#85870=CARTESIAN_POINT('Ctrl Pts',(-20.6485231786559,21.1435494371282,122.553690979311)) ;
#85871=CARTESIAN_POINT('Ctrl Pts',(-20.776994667693,21.1533817871592,122.777909498819)) ;
#85872=CARTESIAN_POINT('Ctrl Pts',(-20.8667919124949,21.1634572262764,123.026935129347)) ;
#85873=CARTESIAN_POINT('Ctrl Pts',(-20.911151449371,21.173309691511,123.282075921991)) ;
#85874=CARTESIAN_POINT('Ctrl Pts',(-20.9107346702923,21.1833825690879,123.546735142883)) ;
#85875=CARTESIAN_POINT('Ctrl Pts',(-20.8653838187256,21.1932251652804,123.801404395061)) ;
#85876=CARTESIAN_POINT('Ctrl Pts',(-20.776098005712,21.2032055493957,124.048000989328)) ;
#85877=CARTESIAN_POINT('Ctrl Pts',(-20.6444053880161,21.2132240300445,124.275965170634)) ;
#85878=CARTESIAN_POINT('Ctrl Pts',(-20.4778156031857,21.2231073450449,124.47526543333)) ;
#85879=CARTESIAN_POINT('Ctrl Pts',(-20.2754160656576,21.2331756421353,124.645605897759)) ;
#85880=CARTESIAN_POINT('Ctrl Pts',(-20.0520068570127,21.2430057105076,124.775388910782)) ;
#85881=CARTESIAN_POINT('Ctrl Pts',(-19.8038192003743,21.253072502976,124.866829885988)) ;
#85882=CARTESIAN_POINT('Ctrl Pts',(-19.5479997475856,21.2629618364645,124.912863623908)) ;
#85883=CARTESIAN_POINT('Ctrl Pts',(-19.2852043849924,21.2729639678806,124.914202847899)) ;
#85884=CARTESIAN_POINT('Ctrl Pts',(-19.0280750006297,21.2828878375016,124.870388521691)) ;
#85885=CARTESIAN_POINT('Ctrl Pts',(-18.77960570535,21.2929313530188,124.781491000549)) ;
#85886=CARTESIAN_POINT('Ctrl Pts',(-18.5538025555048,21.3028135659071,124.653119146439)) ;
#85887=CARTESIAN_POINT('Ctrl Pts',(-18.3500349006823,21.3128816431265,124.484434278303)) ;
#85888=CARTESIAN_POINT('Ctrl Pts',(-18.1823229673718,21.3227201478607,124.28760693878)) ;
#85889=CARTESIAN_POINT('Ctrl Pts',(-18.0480641582105,21.3327829162901,124.059823359472)) ;
#85890=CARTESIAN_POINT('Ctrl Pts',(-17.9571706997418,21.3426799095728,123.816123607726)) ;
#85891=CARTESIAN_POINT('Ctrl Pts',(-17.9089560570351,21.3526111372076,123.559639960323)) ;
#85892=CARTESIAN_POINT('Ctrl Pts',(-17.9062641201702,21.3626532958498,123.295759494904)) ;
#85893=CARTESIAN_POINT('Ctrl Pts',(-17.9485807750656,21.3725400053808,123.039404443611)) ;
#85894=CARTESIAN_POINT('Ctrl Pts',(-18.0352662045675,21.3825329778094,122.791531975748)) ;
#85895=CARTESIAN_POINT('Ctrl Pts',(-18.1631733074527,21.392479172346,122.56359572005)) ;
#85896=CARTESIAN_POINT('Ctrl Pts',(-18.3282744150043,21.4024245471975,122.360963544721)) ;
#85897=CARTESIAN_POINT('Ctrl Pts',(-18.5284565572223,21.4124794665574,122.188538399723)) ;
#85898=CARTESIAN_POINT('Ctrl Pts',(-18.7500672200615,21.4223009860009,122.056167239099)) ;
#85899=CARTESIAN_POINT('Ctrl Pts',(-18.9971032250605,21.4323667547678,121.961729368594)) ;
#85900=CARTESIAN_POINT('Ctrl Pts',(-19.252665844166,21.4422686764229,121.912504687733)) ;
#85901=CARTESIAN_POINT('Ctrl Pts',(-19.516526510854,21.4523117352439,121.908111222315)) ;
#85902=CARTESIAN_POINT('Ctrl Pts',(-19.7735943063744,21.4622177292866,121.949174521215)) ;
#85903=CARTESIAN_POINT('Ctrl Pts',(-20.0206585177756,21.4721555023684,122.033793699405)) ;
#85904=CARTESIAN_POINT('Ctrl Pts',(-20.2514967965682,21.4821958661007,122.161575037695)) ;
#85905=CARTESIAN_POINT('Ctrl Pts',(-20.4536528904977,21.4920832098242,122.324826619752)) ;
#85906=CARTESIAN_POINT('Ctrl Pts',(-20.6265093028174,21.5020754403929,122.522468692439)) ;
#85907=CARTESIAN_POINT('Ctrl Pts',(-20.7617843910413,21.5120239681765,122.746204499775)) ;
#85908=CARTESIAN_POINT('Ctrl Pts',(-20.8563752029685,21.5219607518998,122.989574942634)) ;
#85909=CARTESIAN_POINT('Ctrl Pts',(-20.9078459005937,21.5319437526968,123.246853300404)) ;
#85910=CARTESIAN_POINT('Ctrl Pts',(-20.9134112422956,21.5419876395375,123.510706398789)) ;
#85911=CARTESIAN_POINT('Ctrl Pts',(-20.8745423295287,21.5518156631121,123.766077419227)) ;
#85912=CARTESIAN_POINT('Ctrl Pts',(-20.7899649656379,21.5618929113257,124.016964720075)) ;
#85913=CARTESIAN_POINT('Ctrl Pts',(-20.6660716447633,21.571742466631,124.244301696396)) ;
#85914=CARTESIAN_POINT('Ctrl Pts',(-20.5009218271621,21.5818251748287,124.451413147156)) ;
#85915=CARTESIAN_POINT('Ctrl Pts',(-20.3077024679785,21.5916377677552,124.622265315751)) ;
#85916=CARTESIAN_POINT('Ctrl Pts',(-20.082372609264,21.6017049600131,124.76077174282)) ;
#85917=CARTESIAN_POINT('Ctrl Pts',(-19.8403774418101,21.6116037894757,124.856379349723)) ;
#85918=CARTESIAN_POINT('Ctrl Pts',(-19.5816048957035,21.6216577806659,124.909420890267)) ;
#85919=CARTESIAN_POINT('Ctrl Pts',(-19.3222374612088,21.6315295054491,124.916826891635)) ;
#85920=CARTESIAN_POINT('Ctrl Pts',(-19.0604462619463,21.6415999475793,124.878403745685)) ;
#85921=CARTESIAN_POINT('Ctrl Pts',(-18.8151200955136,21.6514330260096,124.797161576374)) ;
#85922=CARTESIAN_POINT('Ctrl Pts',(-18.5827353405762,21.661463499511,124.672775000186)) ;
#85923=CARTESIAN_POINT('Ctrl Pts',(-18.3759109672851,21.6714950988097,124.509291299171)) ;
#85924=CARTESIAN_POINT('Ctrl Pts',(-18.2037611889679,21.6813247998478,124.316724488468)) ;
#85925=CARTESIAN_POINT('Ctrl Pts',(-18.0647714451557,21.6913142379043,124.094017139833)) ;
#85926=CARTESIAN_POINT('Ctrl Pts',(-17.9666536761754,21.7013581411204,123.848992514289)) ;
#85927=CARTESIAN_POINT('Ctrl Pts',(-17.9132395630017,21.7111796619339,123.596478590155)) ;
#85928=CARTESIAN_POINT('Ctrl Pts',(-17.9036603191974,21.721215386181,123.332930237762)) ;
#85929=CARTESIAN_POINT('Ctrl Pts',(-17.9406169716176,21.7312375401135,123.072144554952)) ;
#85930=CARTESIAN_POINT('Ctrl Pts',(-18.0205753951748,21.7410997718708,122.825638668101)) ;
#85931=CARTESIAN_POINT('Ctrl Pts',(-18.1426765255731,21.7510588423287,122.5941443993)) ;
#85932=CARTESIAN_POINT('Ctrl Pts',(-18.3046553200881,21.7610940147049,122.386052860544)) ;
#85933=CARTESIAN_POINT('Ctrl Pts',(-18.4970548092859,21.7709743998631,122.211659235178)) ;
#85934=CARTESIAN_POINT('Ctrl Pts',(-18.7206332905695,21.7810311144571,122.070794791818)) ;
#85935=CARTESIAN_POINT('Ctrl Pts',(-18.9610017685015,21.7909103830291,121.972655816629)) ;
#85936=CARTESIAN_POINT('Ctrl Pts',(-19.2174642405481,21.8009013405148,121.916435631599)) ;
#85937=CARTESIAN_POINT('Ctrl Pts',(-19.4811229674523,21.81094199915,121.906127926293)) ;
#85938=CARTESIAN_POINT('Ctrl Pts',(-19.7372102471354,21.820774978858,121.940589760359)) ;
#85939=CARTESIAN_POINT('Ctrl Pts',(-19.987662151828,21.8307681121077,122.019553890229)) ;
#85940=CARTESIAN_POINT('Ctrl Pts',(-20.221266587985,21.8408001644911,122.141771264833)) ;
#85941=CARTESIAN_POINT('Ctrl Pts',(-20.4268046448549,21.8506653934424,122.299749040127)) ;
#85942=CARTESIAN_POINT('Ctrl Pts',(-20.6040649592092,21.8606273346856,122.492404487236)) ;
#85943=CARTESIAN_POINT('Ctrl Pts',(-20.7458436231991,21.8706620497224,122.714735308757)) ;
#85944=CARTESIAN_POINT('Ctrl Pts',(-20.8457694698757,21.8805478200664,122.954570602703)) ;
#85945=CARTESIAN_POINT('Ctrl Pts',(-20.903532112246,21.8906104174552,123.212586648096)) ;
#85946=CARTESIAN_POINT('Ctrl Pts',(-20.9154805876386,21.9004608292904,123.471189998348)) ;
#85947=CARTESIAN_POINT('Ctrl Pts',(-20.882426858183,21.9104879985763,123.73260477288)) ;
#85948=CARTESIAN_POINT('Ctrl Pts',(-20.8038186859197,21.9205154792905,123.984131914222)) ;
#85949=CARTESIAN_POINT('Ctrl Pts',(-20.6854109255077,21.9303585318698,124.214093694813)) ;
#85950=CARTESIAN_POINT('Ctrl Pts',(-20.5270023291853,21.9403524353084,124.423570385325)) ;
#85951=CARTESIAN_POINT('Ctrl Pts',(-20.3336537691034,21.9503795580848,124.602604087814)) ;
#85952=CARTESIAN_POINT('Ctrl Pts',(-20.1153478377517,21.9602702629769,124.743677527019)) ;
#85953=CARTESIAN_POINT('Ctrl Pts',(-19.8735692667385,21.9702622898272,124.846083256019)) ;
#85954=CARTESIAN_POINT('Ctrl Pts',(-19.6188372985755,21.9802082713157,124.904607587831)) ;
#85955=CARTESIAN_POINT('Ctrl Pts',(-19.3577931878943,21.9901554439376,124.918542373026)) ;
#85956=CARTESIAN_POINT('Ctrl Pts',(-19.0957252140819,22.0002033852638,124.886329581241)) ;
#85957=CARTESIAN_POINT('Ctrl Pts',(-18.8481898209292,22.0100510190716,124.810847917876)) ;
#85958=CARTESIAN_POINT('Ctrl Pts',(-18.6144904935636,22.0200127337566,124.692911935522)) ;
#85959=CARTESIAN_POINT('Ctrl Pts',(-18.4035879139127,22.0300413666351,124.534852114603)) ;
#85960=CARTESIAN_POINT('Ctrl Pts',(-18.2254150484394,22.0399516921703,124.344920009527)) ;
#85961=CARTESIAN_POINT('Ctrl Pts',(-18.0819977432726,22.049886522642,124.126756044865)) ;
#85962=CARTESIAN_POINT('Ctrl Pts',(-17.9777399583878,22.059927855024,123.884350623129)) ;
#85963=CARTESIAN_POINT('Ctrl Pts',(-17.9179599830939,22.0698207284628,123.631344850412)) ;
#85964=CARTESIAN_POINT('Ctrl Pts',(-17.9022371535386,22.0797898942807,123.369827155738)) ;
#85965=CARTESIAN_POINT('Ctrl Pts',(-17.9327716986324,22.0898186279972,123.108078060828)) ;
#85966=CARTESIAN_POINT('Ctrl Pts',(-18.0314269334723,22.1030111467684,122.775654275456)) ;
#85967=CARTESIAN_POINT('Ctrl Pts',(-18.2167874151558,22.1163710148111,122.472935258562)) ;
#85968=CARTESIAN_POINT('Ctrl Pts',(-18.4689775945887,22.1295963519599,122.233681798304)) ;
#85969=CARTESIAN_POINT('Ctrl Pts',(-18.6872947818254,22.1395775778005,122.088312201797)) ;
#85970=CARTESIAN_POINT('Ctrl Pts',(-18.9290513962181,22.1496131447834,121.982956255966)) ;
#85971=CARTESIAN_POINT('Ctrl Pts',(-19.1809335406282,22.1594762227455,121.921719585)) ;
#85972=CARTESIAN_POINT('Ctrl Pts',(-19.4449971797,22.1695465215466,121.904746363636)) ;
#85973=CARTESIAN_POINT('Ctrl Pts',(-19.7020801434068,22.1793888201144,121.933241045844)) ;
#85974=CARTESIAN_POINT('Ctrl Pts',(-19.9535498675344,22.1893495182842,122.005881902579)) ;
#85975=CARTESIAN_POINT('Ctrl Pts',(-20.1901770423832,22.1993875524637,122.122446448014)) ;
#85976=CARTESIAN_POINT('Ctrl Pts',(-20.3998103087612,22.2092612893102,122.275407092462)) ;
#85977=CARTESIAN_POINT('Ctrl Pts',(-20.5832357329711,22.2193330732354,122.466165386452)) ;
#85978=CARTESIAN_POINT('Ctrl Pts',(-20.7274078859713,22.2291651944366,122.680609736101)) ;
#85979=CARTESIAN_POINT('Ctrl Pts',(-20.8349279101504,22.239198218462,122.921333612289)) ;
#85980=CARTESIAN_POINT('Ctrl Pts',(-20.8982607406429,22.2492140986587,123.176824810715)) ;
#85981=CARTESIAN_POINT('Ctrl Pts',(-20.9165125593692,22.2590976177529,123.43591069118)) ;
#85982=CARTESIAN_POINT('Ctrl Pts',(-20.8895476418826,22.2690880301166,123.697042256073)) ;
#85983=CARTESIAN_POINT('Ctrl Pts',(-20.794199097017,22.28235119332,124.032313731486)) ;
#85984=CARTESIAN_POINT('Ctrl Pts',(-20.6136506128505,22.2956287635712,124.335485744995)) ;
#85985=CARTESIAN_POINT('Ctrl Pts',(-20.3624307998912,22.3089590660778,124.579675665852)) ;
#85986=CARTESIAN_POINT('Ctrl Pts',(-20.1474734503822,22.3188577478942,124.726159691664)) ;
#85987=CARTESIAN_POINT('Ctrl Pts',(-19.9083044716856,22.3288472629417,124.8343602261)) ;
#85988=CARTESIAN_POINT('Ctrl Pts',(-19.6550143972876,22.3387953147168,124.89911320866)) ;
#85989=CARTESIAN_POINT('Ctrl Pts',(-19.3945571768419,22.3487367179953,124.919216158149)) ;
#85990=CARTESIAN_POINT('Ctrl Pts',(-19.0469801715719,22.3620233827762,124.885646801854)) ;
#85991=CARTESIAN_POINT('Ctrl Pts',(-18.6334919756593,22.378633804431,124.731055814575)) ;
#85992=CARTESIAN_POINT('Ctrl Pts',(-18.2305162797271,22.3985450666818,124.387992218144)) ;
#85993=CARTESIAN_POINT('Ctrl Pts',(-17.9681847100688,22.4184891958467,123.927340765981)) ;
#85994=CARTESIAN_POINT('Ctrl Pts',(-17.8789700282879,22.4384123584518,123.405435456902)) ;
#85995=CARTESIAN_POINT('Ctrl Pts',(-17.9722068017202,22.4583024808584,122.88499296031)) ;
#85996=CARTESIAN_POINT('Ctrl Pts',(-18.2392469664603,22.4783074344585,122.425313505132)) ;
#85997=CARTESIAN_POINT('Ctrl Pts',(-18.6435932599694,22.4981456914741,122.086755742294)) ;
#85998=CARTESIAN_POINT('Ctrl Pts',(-19.1427570950757,22.5181399922607,121.904630400796)) ;
#85999=CARTESIAN_POINT('Ctrl Pts',(-19.6712866823868,22.5380252343051,121.904256042346)) ;
#86000=CARTESIAN_POINT('Ctrl Pts',(-20.1684531083155,22.557900180781,122.082765057008)) ;
#86001=CARTESIAN_POINT('Ctrl Pts',(-20.5778666143493,22.5779332507221,122.423256582873)) ;
#86002=CARTESIAN_POINT('Ctrl Pts',(-20.8439539041053,22.5978217576225,122.879952432642)) ;
#86003=CARTESIAN_POINT('Ctrl Pts',(-20.9398901568453,22.6176766174038,123.398949134001)) ;
#86004=CARTESIAN_POINT('Ctrl Pts',(-20.8512776370932,22.6377274511915,123.92432167666)) ;
#86005=CARTESIAN_POINT('Ctrl Pts',(-20.5928105483306,22.6574933930808,124.381851942389)) ;
#86006=CARTESIAN_POINT('Ctrl Pts',(-20.1896636816174,22.6775061245401,124.728595251841)) ;
#86007=CARTESIAN_POINT('Ctrl Pts',(-19.6948416932879,22.6973989594837,124.915260290639)) ;
#86008=CARTESIAN_POINT('Ctrl Pts',(-19.1659292643134,22.7173059828232,124.922744509421)) ;
#86009=CARTESIAN_POINT('Ctrl Pts',(-18.6655675605648,22.7372212477239,124.749699013636)) ;
#86010=CARTESIAN_POINT('Ctrl Pts',(-18.2524453398778,22.7572529398836,124.413924653691)) ;
#86011=CARTESIAN_POINT('Ctrl Pts',(-17.9812029359813,22.7770959864566,123.961563010291)) ;
#86012=CARTESIAN_POINT('Ctrl Pts',(-17.8790677895418,22.7970125343564,123.442240253503)) ;
#86013=CARTESIAN_POINT('Ctrl Pts',(-17.9604555657489,22.8169447773477,122.918716094646)) ;
#86014=CARTESIAN_POINT('Ctrl Pts',(-18.2149597212616,22.836848612157,122.454982006216)) ;
#86015=CARTESIAN_POINT('Ctrl Pts',(-18.6119455544731,22.8567490123445,122.105477724641)) ;
#86016=CARTESIAN_POINT('Ctrl Pts',(-19.1055301645696,22.8766986887238,121.911730698857)) ;
#86017=CARTESIAN_POINT('Ctrl Pts',(-19.6351375624815,22.8966312129442,121.898173547559)) ;
#86018=CARTESIAN_POINT('Ctrl Pts',(-20.1374387737837,22.9165512219304,122.065632357375)) ;
#86019=CARTESIAN_POINT('Ctrl Pts',(-20.5530897144561,22.9365081281066,122.395063821693)) ;
#86020=CARTESIAN_POINT('Ctrl Pts',(-20.8308724977881,22.9563939676081,122.844830062582)) ;
#86021=CARTESIAN_POINT('Ctrl Pts',(-20.9388539512202,22.9763651397439,123.364411422884)) ;
#86022=CARTESIAN_POINT('Ctrl Pts',(-20.8643389626638,22.9961793367283,123.885825621413)) ;
#86023=CARTESIAN_POINT('Ctrl Pts',(-20.6149971103256,23.0161605226965,124.354606393768)) ;
#86024=CARTESIAN_POINT('Ctrl Pts',(-20.2875827610197,23.0327360280858,124.64946647421)) ;
#86025=CARTESIAN_POINT('Ctrl Pts',(-19.9761963329815,23.0460454759494,124.808750590775)) ;
#86026=CARTESIAN_POINT('Ctrl Pts',(-19.6403478940357,23.059413173726,124.911784399414)) ;
#86027=CARTESIAN_POINT('Ctrl Pts',(-19.2023596389031,23.0759037453919,124.927929061235)) ;
#86028=CARTESIAN_POINT('Ctrl Pts',(-18.6980186540393,23.0958240177247,124.767071885537)) ;
#86029=CARTESIAN_POINT('Ctrl Pts',(-18.3484072158521,23.1124410534457,124.497150544743)) ;
#86030=CARTESIAN_POINT('Ctrl Pts',(-18.1364154882604,23.1257319037268,124.219541419118)) ;
#86031=CARTESIAN_POINT('Ctrl Pts',(-18.0158927766921,23.1357009488813,123.986966551078)) ;
#86032=CARTESIAN_POINT('Ctrl Pts',(-17.937590459842,23.1456043395148,123.738742873997)) ;
#86033=CARTESIAN_POINT('Ctrl Pts',(-17.9031973751966,23.1556621256276,123.476711455943)) ;
#86034=CARTESIAN_POINT('Ctrl Pts',(-17.9143593563858,23.1655141622773,123.218025990263)) ;
#86035=CARTESIAN_POINT('Ctrl Pts',(-17.9896268659552,23.1788792864205,122.874973437508)) ;
#86036=CARTESIAN_POINT('Ctrl Pts',(-18.151401302181,23.1921053493835,122.562854577334)) ;
#86037=CARTESIAN_POINT('Ctrl Pts',(-18.3866165742264,23.2054089976658,122.304238650459)) ;
#86038=CARTESIAN_POINT('Ctrl Pts',(-18.5942744744476,23.2154005288288,122.143499851417)) ;
#86039=CARTESIAN_POINT('Ctrl Pts',(-18.8279217544426,23.2254399766281,122.02101181735)) ;
#86040=CARTESIAN_POINT('Ctrl Pts',(-19.0743059149406,23.235283752142,121.942132253362)) ;
#86041=CARTESIAN_POINT('Ctrl Pts',(-19.3342082548891,23.2452693935296,121.906215557607)) ;
#86042=CARTESIAN_POINT('Ctrl Pts',(-19.595203409344,23.2552061778914,121.915784532965)) ;
#86043=CARTESIAN_POINT('Ctrl Pts',(-19.8533817478491,23.2652560123588,121.971267328799)) ;
#86044=CARTESIAN_POINT('Ctrl Pts',(-20.0932669657549,23.2751064618619,122.068597590794)) ;
#86045=CARTESIAN_POINT('Ctrl Pts',(-20.3156335651349,23.285078475844,122.207190765456)) ;
#86046=CARTESIAN_POINT('Ctrl Pts',(-20.5110432440586,23.2950736336911,122.382771699199)) ;
#86047=CARTESIAN_POINT('Ctrl Pts',(-20.6733357401702,23.3051075600548,122.590562603099)) ;
#86048=CARTESIAN_POINT('Ctrl Pts',(-20.7952641776477,23.3149632684872,122.81909160789)) ;
#86049=CARTESIAN_POINT('Ctrl Pts',(-20.8771604366914,23.3249614178259,123.068699179642)) ;
#86050=CARTESIAN_POINT('Ctrl Pts',(-20.9143466504709,23.3348608209994,123.326212352676)) ;
#86051=CARTESIAN_POINT('Ctrl Pts',(-20.9061903378289,23.3449120178879,123.590193277281)) ;
#86052=CARTESIAN_POINT('Ctrl Pts',(-20.8532554613795,23.3547943417008,123.844458307403)) ;
#86053=CARTESIAN_POINT('Ctrl Pts',(-20.7564386685029,23.3647892373574,124.088610236154)) ;
#86054=CARTESIAN_POINT('Ctrl Pts',(-20.6179988147476,23.3748103367399,124.312644230857)) ;
#86055=CARTESIAN_POINT('Ctrl Pts',(-20.4449168413211,23.384717604602,124.507129660358)) ;
#86056=CARTESIAN_POINT('Ctrl Pts',(-20.240390604112,23.3946559484272,124.669516991948)) ;
#86057=CARTESIAN_POINT('Ctrl Pts',(-20.0093102113973,23.4046593677277,124.794907442227)) ;
#86058=CARTESIAN_POINT('Ctrl Pts',(-19.7590948886003,23.4146939184348,124.878100956568)) ;
#86059=CARTESIAN_POINT('Ctrl Pts',(-19.5031986835257,23.4245388680404,124.916298887153)) ;
#86060=CARTESIAN_POINT('Ctrl Pts',(-19.240901379397,23.4345247101533,124.909881080696)) ;
#86061=CARTESIAN_POINT('Ctrl Pts',(-18.9848919832439,23.4444595175224,124.858447576063)) ;
#86062=CARTESIAN_POINT('Ctrl Pts',(-18.7388649759424,23.4545170592357,124.761980421742)) ;
#86063=CARTESIAN_POINT('Ctrl Pts',(-18.5183526283299,23.4643386567478,124.627795609594)) ;
#86064=CARTESIAN_POINT('Ctrl Pts',(-18.3195736794291,23.4743949162283,124.453691135326)) ;
#86065=CARTESIAN_POINT('Ctrl Pts',(-18.1562934925279,23.4843348525287,124.249783586925)) ;
#86066=CARTESIAN_POINT('Ctrl Pts',(-18.0306337931109,23.4942419732731,124.021771235105)) ;
#86067=CARTESIAN_POINT('Ctrl Pts',(-17.9454129427096,23.5042848791984,123.771998892176)) ;
#86068=CARTESIAN_POINT('Ctrl Pts',(-17.9053473190908,23.5141926602976,123.514723390938)) ;
#86069=CARTESIAN_POINT('Ctrl Pts',(-17.9101532963783,23.5242030293,123.251696708579)) ;
#86070=CARTESIAN_POINT('Ctrl Pts',(-17.961184062847,23.5342338678688,122.993085702516)) ;
#86071=CARTESIAN_POINT('Ctrl Pts',(-18.0542237398046,23.5440867075085,122.751450868495)) ;
#86072=CARTESIAN_POINT('Ctrl Pts',(-18.1892126976711,23.5540747086735,122.526373711805)) ;
#86073=CARTESIAN_POINT('Ctrl Pts',(-18.3602268731788,23.5640035276526,122.329304006708)) ;
#86074=CARTESIAN_POINT('Ctrl Pts',(-18.5637893871461,23.5739912303749,122.163599331592)) ;
#86075=CARTESIAN_POINT('Ctrl Pts',(-18.7943337470643,23.5840272301776,122.035538227318)) ;
#86076=CARTESIAN_POINT('Ctrl Pts',(-19.0390033894445,23.593882099979,121.95058970854)) ;
#86077=CARTESIAN_POINT('Ctrl Pts',(-19.2983352169612,23.6038815304026,121.908467679911)) ;
#86078=CARTESIAN_POINT('Ctrl Pts',(-19.5583918752554,23.6137766478679,121.911699650908)) ;
#86079=CARTESIAN_POINT('Ctrl Pts',(-19.8181268029097,23.6238371413848,121.960855606037)) ;
#86080=CARTESIAN_POINT('Ctrl Pts',(-20.0602942162802,23.633686621586,122.052288166794)) ;
#86081=CARTESIAN_POINT('Ctrl Pts',(-20.2872341468449,23.6437130718498,122.186156421621)) ;
#86082=CARTESIAN_POINT('Ctrl Pts',(-20.4871135693957,23.6537443623279,122.358035384557)) ;
#86083=CARTESIAN_POINT('Ctrl Pts',(-20.6513848025357,23.6635857499797,122.55778850806)) ;
#86084=CARTESIAN_POINT('Ctrl Pts',(-20.7809994490433,23.6735891508709,122.786461903559)) ;
#86085=CARTESIAN_POINT('Ctrl Pts',(-20.8686943861811,23.6835735336621,123.033800795154)) ;
#86086=CARTESIAN_POINT('Ctrl Pts',(-20.9120896033788,23.6936126236755,123.2939975435)) ;
#86087=CARTESIAN_POINT('Ctrl Pts',(-20.9100555677439,23.7034584325847,123.552746650312)) ;
#86088=CARTESIAN_POINT('Ctrl Pts',(-20.8629995601481,23.7134428554037,123.810834394173)) ;
#86089=CARTESIAN_POINT('Ctrl Pts',(-20.7723339495502,23.7233824806449,124.055836429127)) ;
#86090=CARTESIAN_POINT('Ctrl Pts',(-20.6391535588763,23.7334221701635,124.283563391533)) ;
#86091=CARTESIAN_POINT('Ctrl Pts',(-20.4711070029557,23.7433103585821,124.481782915492)) ;
#86092=CARTESIAN_POINT('Ctrl Pts',(-20.2694803443746,23.7532998845842,124.649877833456)) ;
#86093=CARTESIAN_POINT('Ctrl Pts',(-20.042335267145,23.7632583859393,124.7798313255)) ;
#86094=CARTESIAN_POINT('Ctrl Pts',(-19.7977296828341,23.773157979943,124.868459892283)) ;
#86095=CARTESIAN_POINT('Ctrl Pts',(-19.5376387109747,23.7832058680643,124.913842306988)) ;
#86096=CARTESIAN_POINT('Ctrl Pts',(-19.2775559394141,23.7931012933098,124.913585868621)) ;
#86097=CARTESIAN_POINT('Ctrl Pts',(-19.0172389437925,23.8031626840104,124.867462659727)) ;
#86098=CARTESIAN_POINT('Ctrl Pts',(-18.774152370709,23.8130082676971,124.778813564933)) ;
#86099=CARTESIAN_POINT('Ctrl Pts',(-18.5470679864683,23.8229712410063,124.648540906934)) ;
#86100=CARTESIAN_POINT('Ctrl Pts',(-18.3449854684297,23.8329969078321,124.479471088792)) ;
#86101=CARTESIAN_POINT('Ctrl Pts',(-18.1771183031737,23.8429113856984,124.280226434427)) ;
#86102=CARTESIAN_POINT('Ctrl Pts',(-18.0449530498413,23.8528999003734,124.053415180834)) ;
#86103=CARTESIAN_POINT('Ctrl Pts',(-17.9542174865925,23.8629440112888,123.805578221622)) ;
#86104=CARTESIAN_POINT('Ctrl Pts',(-17.9082598864059,23.8727721488834,123.551388438519)) ;
#86105=CARTESIAN_POINT('Ctrl Pts',(-17.9069862290974,23.8828487169423,123.286644032258)) ;
#86106=CARTESIAN_POINT('Ctrl Pts',(-17.9505929400621,23.8927008788465,123.031379907163)) ;
#86107=CARTESIAN_POINT('Ctrl Pts',(-18.0395746759122,23.9027738408033,122.782125620061)) ;
#86108=CARTESIAN_POINT('Ctrl Pts',(-18.1675552431538,23.9126164028062,122.557328161597)) ;
#86109=CARTESIAN_POINT('Ctrl Pts',(-18.3342353084014,23.9225968393,122.35484385985)) ;
#86110=CARTESIAN_POINT('Ctrl Pts',(-18.5346335209383,23.9326151446244,122.184110750498)) ;
#86111=CARTESIAN_POINT('Ctrl Pts',(-18.7583418735152,23.9424991085438,122.052074633009)) ;
#86112=CARTESIAN_POINT('Ctrl Pts',(-19.0060227711856,23.9525649852824,121.959294062984)) ;
#86113=CARTESIAN_POINT('Ctrl Pts',(-19.2602154899171,23.9624040861433,121.911839822886)) ;
#86114=CARTESIAN_POINT('Ctrl Pts',(-19.5238406827779,23.972437169009,121.90852668778)) ;
#86115=CARTESIAN_POINT('Ctrl Pts',(-19.7836670395102,23.9824588542845,121.951641266166)) ;
#86116=CARTESIAN_POINT('Ctrl Pts',(-20.0283217952903,23.992325549383,122.037454405699)) ;
#86117=CARTESIAN_POINT('Ctrl Pts',(-20.256860421925,24.0022854391175,122.165053725248)) ;
#86118=CARTESIAN_POINT('Ctrl Pts',(-20.4610242017121,24.012320426943,122.331938946934)) ;
#86119=CARTESIAN_POINT('Ctrl Pts',(-20.6309297767146,24.0222071310173,122.528544653014)) ;
#86120=CARTESIAN_POINT('Ctrl Pts',(-20.7664224941324,24.0322722752502,122.755656874661)) ;
#86121=CARTESIAN_POINT('Ctrl Pts',(-20.858590344017,24.0421115659788,122.997281659938)) ;
#86122=CARTESIAN_POINT('Ctrl Pts',(-20.9088537868088,24.0521741234172,123.256862342196)) ;
#86123=CARTESIAN_POINT('Ctrl Pts',(-20.9129308819633,24.0620711746693,123.516929777868)) ;
#86124=CARTESIAN_POINT('Ctrl Pts',(-20.8725108015801,24.0720023814176,123.77475646931)) ;
#86125=CARTESIAN_POINT('Ctrl Pts',(-20.7867177695425,24.0820445656364,124.024315773816)) ;
#86126=CARTESIAN_POINT('Ctrl Pts',(-20.661034087862,24.0919311937473,124.251717624557)) ;
#86127=CARTESIAN_POINT('Ctrl Pts',(-20.4963706306924,24.1019244662797,124.456275571947)) ;
#86128=CARTESIAN_POINT('Ctrl Pts',(-20.2995736659004,24.1118695418212,124.628245533589)) ;
#86129=CARTESIAN_POINT('Ctrl Pts',(-20.0760604743478,24.1218190925494,124.763934584824)) ;
#86130=CARTESIAN_POINT('Ctrl Pts',(-19.8301158593886,24.1318584273974,124.859366095419)) ;
#86131=CARTESIAN_POINT('Ctrl Pts',(-19.5752990612999,24.1417445663413,124.910102290642)) ;
#86132=CARTESIAN_POINT('Ctrl Pts',(-19.3126616551709,24.151742679315,124.916221608112)) ;
#86133=CARTESIAN_POINT('Ctrl Pts',(-19.0549019437606,24.1616624416675,124.877102085613)) ;
#86134=CARTESIAN_POINT('Ctrl Pts',(-18.8048861129423,24.1717018372801,124.792908728752)) ;
#86135=CARTESIAN_POINT('Ctrl Pts',(-18.5763150218767,24.1816110230684,124.668144211837)) ;
#86136=CARTESIAN_POINT('Ctrl Pts',(-18.3718886839389,24.1915462072259,124.50573368631)) ;
#86137=CARTESIAN_POINT('Ctrl Pts',(-18.1971228535137,24.2015872646118,124.308047316945)) ;
#86138=CARTESIAN_POINT('Ctrl Pts',(-18.0612783306157,24.2114744226451,124.086547050275)) ;
#86139=CARTESIAN_POINT('Ctrl Pts',(-17.9645493227509,24.221466702321,123.842445202394)) ;
#86140=CARTESIAN_POINT('Ctrl Pts',(-17.9119696693637,24.2314152193661,123.586335183678)) ;
#86141=CARTESIAN_POINT('Ctrl Pts',(-17.9042989976674,24.2413519969365,123.325341447214)) ;
#86142=CARTESIAN_POINT('Ctrl Pts',(-17.9419176299516,24.2513350330834,123.06567537359)) ;
#86143=CARTESIAN_POINT('Ctrl Pts',(-18.0249900888699,24.2613787846771,122.815181470846)) ;
#86144=CARTESIAN_POINT('Ctrl Pts',(-18.1471098273281,24.2712073138897,122.587547692865)) ;
#86145=CARTESIAN_POINT('Ctrl Pts',(-18.3107425634225,24.2812826747984,122.379462252064)) ;
#86146=CARTESIAN_POINT('Ctrl Pts',(-18.5037560854593,24.2911392736856,122.206642338797)) ;
#86147=CARTESIAN_POINT('Ctrl Pts',(-18.7282169843324,24.3012022677035,122.066922869341)) ;
#86148=CARTESIAN_POINT('Ctrl Pts',(-18.9691137819942,24.311080201993,121.970094344382)) ;
#86149=CARTESIAN_POINT('Ctrl Pts',(-19.2261436370484,24.321080849551,121.915522158594)) ;
#86150=CARTESIAN_POINT('Ctrl Pts',(-19.4866572465794,24.3309986959891,121.906283510334)) ;
#86151=CARTESIAN_POINT('Ctrl Pts',(-19.7481874126353,24.3410498129947,121.942965407598)) ;
#86152=CARTESIAN_POINT('Ctrl Pts',(-19.995044655726,24.3509205483053,122.022786909086)) ;
#86153=CARTESIAN_POINT('Ctrl Pts',(-20.2288798534327,24.3609912555483,122.146628302463)) ;
#86154=CARTESIAN_POINT('Ctrl Pts',(-20.4328576975085,24.3708242630002,122.305301061164)) ;
#86155=CARTESIAN_POINT('Ctrl Pts',(-20.6102013492879,24.3808547553025,122.500299127757)) ;
#86156=CARTESIAN_POINT('Ctrl Pts',(-20.7503713756113,24.3908863503759,122.723582642861)) ;
#86157=CARTESIAN_POINT('Ctrl Pts',(-20.8481322685785,24.4007160495141,122.962664906748)) ;
#86158=CARTESIAN_POINT('Ctrl Pts',(-20.9045567151015,24.4107054993957,123.219049565126)) ;
#86159=CARTESIAN_POINT('Ctrl Pts',(-20.9149976124652,24.4207493572114,123.482781782384)) ;
#86160=CARTESIAN_POINT('Ctrl Pts',(-20.8808031916903,24.4305710478016,123.738611883266)) ;
#86161=CARTESIAN_POINT('Ctrl Pts',(-20.8016222714478,24.440606138342,123.990150687533)) ;
#86162=CARTESIAN_POINT('Ctrl Pts',(-20.6794652177334,24.4506306573247,124.223569827565)) ;
#86163=CARTESIAN_POINT('Ctrl Pts',(-20.5216485278088,24.4604905027349,124.429046599541)) ;
#86164=CARTESIAN_POINT('Ctrl Pts',(-20.3290856748974,24.4704502790506,124.60632034406)) ;
#86165=CARTESIAN_POINT('Ctrl Pts',(-20.1069640189552,24.4804784763652,124.748123595379)) ;
#86166=CARTESIAN_POINT('Ctrl Pts',(-19.8666180274097,24.4903860186555,124.848283735091)) ;
#86167=CARTESIAN_POINT('Ctrl Pts',(-19.6093832914182,24.5004186692194,124.905987754454)) ;
#86168=CARTESIAN_POINT('Ctrl Pts',(-19.3499154760575,24.510302625646,124.918048718704)) ;
#86169=CARTESIAN_POINT('Ctrl Pts',(-19.0894596086663,24.5202923270079,124.885168267668)) ;
#86170=CARTESIAN_POINT('Ctrl Pts',(-18.8375518685682,24.5303333222839,124.806629416254)) ;
#86171=CARTESIAN_POINT('Ctrl Pts',(-18.607775073596,24.5401662115523,124.688434190657)) ;
#86172=CARTESIAN_POINT('Ctrl Pts',(-18.3982021069512,24.5501593699197,124.530191196066)) ;
#86173=CARTESIAN_POINT('Ctrl Pts',(-18.2189836852721,24.5601914122718,124.336829304906)) ;
#86174=CARTESIAN_POINT('Ctrl Pts',(-18.0781826899015,24.5700566562302,124.119164288488)) ;
#86175=CARTESIAN_POINT('Ctrl Pts',(-17.9756353809418,24.5800185474762,123.878288988731)) ;
#86176=CARTESIAN_POINT('Ctrl Pts',(-17.9164583703033,24.5900534474947,123.621321390185)) ;
#86177=CARTESIAN_POINT('Ctrl Pts',(-17.9025709875067,24.5999385279093,123.361889607157)) ;
#86178=CARTESIAN_POINT('Ctrl Pts',(-17.9345306575501,24.6100037000341,123.0993606842)) ;
#86179=CARTESIAN_POINT('Ctrl Pts',(-18.009793838017,24.6198509347576,122.851745183802)) ;
#86180=CARTESIAN_POINT('Ctrl Pts',(-18.1285188816227,24.6298817460754,122.616416570995)) ;
#86181=CARTESIAN_POINT('Ctrl Pts',(-18.2864282941797,24.6398913619889,122.406008126817)) ;
#86182=CARTESIAN_POINT('Ctrl Pts',(-18.4763620674248,24.6498021413926,122.227839272266)) ;
#86183=CARTESIAN_POINT('Ctrl Pts',(-18.6944258490363,24.6597314071816,122.084521998851)) ;
#86184=CARTESIAN_POINT('Ctrl Pts',(-18.9368657879906,24.6697741004942,121.980279706775)) ;
#86185=CARTESIAN_POINT('Ctrl Pts',(-19.1897153085028,24.679660633189,121.92048694765)) ;
#86186=CARTESIAN_POINT('Ctrl Pts',(-19.4518476983688,24.6896537782922,121.904901247144)) ;
#86187=CARTESIAN_POINT('Ctrl Pts',(-19.7114689211226,24.6995994589663,121.935024786244)) ;
#86188=CARTESIAN_POINT('Ctrl Pts',(-19.9621203216531,24.709546716593,122.009272431099)) ;
#86189=CARTESIAN_POINT('Ctrl Pts',(-20.1982874731001,24.7195946187145,122.127349372162)) ;
#86190=CARTESIAN_POINT('Ctrl Pts',(-20.4062771468984,24.7294423243362,122.281336350192)) ;
#86191=CARTESIAN_POINT('Ctrl Pts',(-20.5870191315301,24.7394037909703,122.470689270979)) ;
#86192=CARTESIAN_POINT('Ctrl Pts',(-20.7328443334499,24.7494333442385,122.690250749449)) ;
#86193=CARTESIAN_POINT('Ctrl Pts',(-20.8371756815299,24.7593402362659,122.928777696645)) ;
#86194=CARTESIAN_POINT('Ctrl Pts',(-20.8992448149416,24.7692878803789,123.182694125672)) ;
#86195=CARTESIAN_POINT('Ctrl Pts',(-20.9165397755815,24.7792879234078,123.444949438803)) ;
#86196=CARTESIAN_POINT('Ctrl Pts',(-20.8874649816599,24.7893266894018,123.707130191398)) ;
#86197=CARTESIAN_POINT('Ctrl Pts',(-20.8154023193973,24.7991517514241,123.955080646736)) ;
#86198=CARTESIAN_POINT('Ctrl Pts',(-20.6991263352566,24.8092062987504,124.192325406435)) ;
#86199=CARTESIAN_POINT('Ctrl Pts',(-20.5447671392046,24.8191495421996,124.403167472963)) ;
#86200=CARTESIAN_POINT('Ctrl Pts',(-20.3574869860895,24.8290517138075,124.58383784483)) ;
#86201=CARTESIAN_POINT('Ctrl Pts',(-20.1383185841272,24.8391045494177,124.731315017245)) ;
#86202=CARTESIAN_POINT('Ctrl Pts',(-19.901213310372,24.8489776071032,124.836683877999)) ;
#86203=CARTESIAN_POINT('Ctrl Pts',(-19.646468082972,24.8589728686289,124.900684701347)) ;
#86204=CARTESIAN_POINT('Ctrl Pts',(-19.3836496123046,24.8689982380494,124.919067997293)) ;
#86205=CARTESIAN_POINT('Ctrl Pts',(-19.1251299071319,24.878888070576,124.892249885578)) ;
#86206=CARTESIAN_POINT('Ctrl Pts',(-18.7890091715742,24.8921860413854,124.796799294934)) ;
#86207=CARTESIAN_POINT('Ctrl Pts',(-18.4874128569439,24.9053844364946,124.617566260999)) ;
#86208=CARTESIAN_POINT('Ctrl Pts',(-18.2417575404836,24.918779878774,124.365456812483)) ;
#86209=CARTESIAN_POINT('Ctrl Pts',(-18.0954573193109,24.928655717013,124.151048711038)) ;
#86210=CARTESIAN_POINT('Ctrl Pts',(-17.9865203150819,24.9387171196107,123.910175250881)) ;
#86211=CARTESIAN_POINT('Ctrl Pts',(-17.9222460999715,24.9485821765459,123.658987057165)) ;
#86212=CARTESIAN_POINT('Ctrl Pts',(-17.9018079283208,24.9585942724947,123.396707820689)) ;
#86213=CARTESIAN_POINT('Ctrl Pts',(-17.9355686586318,24.9718715816401,123.049393446101)) ;
#86214=CARTESIAN_POINT('Ctrl Pts',(-18.0899475407356,24.9884706071474,122.636126991343)) ;
#86215=CARTESIAN_POINT('Ctrl Pts',(-18.3760314708444,25.0050696551804,122.300327989926)) ;
#86216=CARTESIAN_POINT('Ctrl Pts',(-18.6623187112641,25.0183130672114,122.102384463216)) ;
#86217=CARTESIAN_POINT('Ctrl Pts',(-18.9019733035102,25.0283504948998,121.992225850964)) ;
#86218=CARTESIAN_POINT('Ctrl Pts',(-19.1537567559459,25.0382547968554,121.926273908146)) ;
#86219=CARTESIAN_POINT('Ctrl Pts',(-19.5011724762164,25.0515216368306,121.896923152544)) ;
#86220=CARTESIAN_POINT('Ctrl Pts',(-19.9361209211562,25.0681478349205,121.974892242463)) ;
#86221=CARTESIAN_POINT('Ctrl Pts',(-20.3941483506745,25.0880669503039,122.240432926128)) ;
#86222=CARTESIAN_POINT('Ctrl Pts',(-20.6778013141646,25.1046733734382,122.578575786354)) ;
#86223=CARTESIAN_POINT('Ctrl Pts',(-20.8254198064288,25.1179695939339,122.895276836921)) ;
#86224=CARTESIAN_POINT('Ctrl Pts',(-20.9163896664301,25.1312384262753,123.231970672834)) ;
#86225=CARTESIAN_POINT('Ctrl Pts',(-20.9167689419944,25.1479296743084,123.675492638632)) ;
#86226=CARTESIAN_POINT('Ctrl Pts',(-20.7380584204792,25.1677394059812,124.170815449789)) ;
#86227=CARTESIAN_POINT('Ctrl Pts',(-20.3990544179289,25.1877170133098,124.579453442232)) ;
#86228=CARTESIAN_POINT('Ctrl Pts',(-19.9416756734989,25.2076433223676,124.846325842365)) ;
#86229=CARTESIAN_POINT('Ctrl Pts',(-19.4236779184025,25.2274601825323,124.942437107342)) ;
#86230=CARTESIAN_POINT('Ctrl Pts',(-18.8970108487145,25.2475599981263,124.854014090052)) ;
#86231=CARTESIAN_POINT('Ctrl Pts',(-18.4395915110761,25.2673169620089,124.595686505518)) ;
#86232=CARTESIAN_POINT('Ctrl Pts',(-18.0924071157132,25.2873538880783,124.192105333411)) ;
#86233=CARTESIAN_POINT('Ctrl Pts',(-17.9060265000467,25.3072234704598,123.697842908581)) ;
#86234=CARTESIAN_POINT('Ctrl Pts',(-17.8981566895004,25.327128042213,123.168973851605)) ;
#86235=CARTESIAN_POINT('Ctrl Pts',(-18.0717642136479,25.3470806444115,122.667793933237)) ;
#86236=CARTESIAN_POINT('Ctrl Pts',(-18.4052645219479,25.3669901353818,122.257095727428)) ;
#86237=CARTESIAN_POINT('Ctrl Pts',(-18.8570067132281,25.3868415040812,121.984255857802)) ;
#86238=CARTESIAN_POINT('Ctrl Pts',(-19.3806239056403,25.4069217002172,121.881586989434)) ;
#86239=CARTESIAN_POINT('Ctrl Pts',(-19.9007576230194,25.4267226437926,121.962652492736)) ;
#86240=CARTESIAN_POINT('Ctrl Pts',(-20.3666506513675,25.4467066203021,122.217535832542)) ;
#86241=CARTESIAN_POINT('Ctrl Pts',(-20.7158407306792,25.4666225832777,122.615352102572)) ;
#86242=CARTESIAN_POINT('Ctrl Pts',(-20.9092753913654,25.4864930180996,123.10688621769)) ;
#86243=CARTESIAN_POINT('Ctrl Pts',(-20.9225933282135,25.5065433033327,123.63946964645)) ;
#86244=CARTESIAN_POINT('Ctrl Pts',(-20.7563011574428,25.526317272092,124.138248789555)) ;
#86245=CARTESIAN_POINT('Ctrl Pts',(-20.4256737839772,25.5463737302116,124.55612392467)) ;
#86246=CARTESIAN_POINT('Ctrl Pts',(-19.9778044990182,25.5661686132026,124.832472781124)) ;
#86247=CARTESIAN_POINT('Ctrl Pts',(-19.4586089000129,25.5861352685049,124.941740459474)) ;
#86248=CARTESIAN_POINT('Ctrl Pts',(-18.933405433002,25.6060942385814,124.866405585267)) ;
#86249=CARTESIAN_POINT('Ctrl Pts',(-18.4668441914665,25.6259903261715,124.617555781116)) ;
#86250=CARTESIAN_POINT('Ctrl Pts',(-18.1127144201242,25.6458884960831,124.224823959823)) ;
#86251=CARTESIAN_POINT('Ctrl Pts',(-17.9132301741929,25.6657943314502,123.734766837906)) ;
#86252=CARTESIAN_POINT('Ctrl Pts',(-17.8929228695584,25.6857442563881,123.204966867725)) ;
#86253=CARTESIAN_POINT('Ctrl Pts',(-18.0536111401075,25.7056234462985,122.701580140501)) ;
#86254=CARTESIAN_POINT('Ctrl Pts',(-18.377808589848,25.7256047705791,122.281003832198)) ;
#86255=CARTESIAN_POINT('Ctrl Pts',(-18.8251899843192,25.7455345547874,121.99718762822)) ;
#86256=CARTESIAN_POINT('Ctrl Pts',(-19.3420583616094,25.7654545441782,121.883074058097)) ;
#86257=CARTESIAN_POINT('Ctrl Pts',(-19.8655398108464,25.7853097395322,121.95081448643)) ;
#86258=CARTESIAN_POINT('Ctrl Pts',(-20.3385236962934,25.8053557411916,122.195787304325)) ;
#86259=CARTESIAN_POINT('Ctrl Pts',(-20.6359551620709,25.8218554884014,122.518224212841)) ;
#86260=CARTESIAN_POINT('Ctrl Pts',(-20.7997772299296,25.8352440928495,122.829543405343)) ;
#86261=CARTESIAN_POINT('Ctrl Pts',(-20.878806089281,25.8451059211844,123.076370301885)) ;
#86262=CARTESIAN_POINT('Ctrl Pts',(-20.9149660822381,25.855072063942,123.335767898469)) ;
#86263=CARTESIAN_POINT('Ctrl Pts',(-20.901681357157,25.8684338100669,123.686592876107)) ;
#86264=CARTESIAN_POINT('Ctrl Pts',(-20.7738066717889,25.884888139022,124.104963749759)) ;
#86265=CARTESIAN_POINT('Ctrl Pts',(-20.5060796437535,25.9016553840703,124.461005538212)) ;
#86266=CARTESIAN_POINT('Ctrl Pts',(-20.2328324341928,25.9148419493443,124.674328351222)) ;
#86267=CARTESIAN_POINT('Ctrl Pts',(-20.0014412245227,25.9248314080889,124.798165745444)) ;
#86268=CARTESIAN_POINT('Ctrl Pts',(-19.7528536304337,25.93478518057,124.879736163845)) ;
#86269=CARTESIAN_POINT('Ctrl Pts',(-19.4914876961368,25.9448329971027,124.917038232705)) ;
#86270=CARTESIAN_POINT('Ctrl Pts',(-19.2329656958291,25.9546745302252,124.908870993837)) ;
#86271=CARTESIAN_POINT('Ctrl Pts',(-18.9760196741983,25.9646607724449,124.85572458636)) ;
#86272=CARTESIAN_POINT('Ctrl Pts',(-18.7332872577401,25.9745973958698,124.759342505799)) ;
#86273=CARTESIAN_POINT('Ctrl Pts',(-18.5085731788918,25.9846472732528,124.620640269178)) ;
#86274=CARTESIAN_POINT('Ctrl Pts',(-18.3151059732975,25.9944977120304,124.448627307497)) ;
#86275=CARTESIAN_POINT('Ctrl Pts',(-18.1519582512238,26.0044697259991,124.243595958302)) ;
#86276=CARTESIAN_POINT('Ctrl Pts',(-18.0265942662714,26.0144648946252,124.012733796054)) ;
#86277=CARTESIAN_POINT('Ctrl Pts',(-17.94321575523,26.0244987778864,123.762605317723)) ;
#86278=CARTESIAN_POINT('Ctrl Pts',(-17.9048256332287,26.0343546479497,123.506445495096)) ;
#86279=CARTESIAN_POINT('Ctrl Pts',(-17.9111726656182,26.0443521938669,123.243825664362)) ;
#86280=CARTESIAN_POINT('Ctrl Pts',(-17.9624847437566,26.0542603207662,122.988545851874)) ;
#86281=CARTESIAN_POINT('Ctrl Pts',(-18.0578964910856,26.0642706922883,122.743382417585)) ;
#86282=CARTESIAN_POINT('Ctrl Pts',(-18.195192673543,26.0743011350357,122.518384012855)) ;
#86283=CARTESIAN_POINT('Ctrl Pts',(-18.3658649539483,26.084149087589,122.323819765035)) ;
#86284=CARTESIAN_POINT('Ctrl Pts',(-18.5719645952938,26.09421175661,122.158181340976)) ;
#86285=CARTESIAN_POINT('Ctrl Pts',(-18.7999511759967,26.1041061320739,122.033112687758)) ;
#86286=CARTESIAN_POINT('Ctrl Pts',(-19.0470918391407,26.1140479303921,121.948484295276)) ;
#86287=CARTESIAN_POINT('Ctrl Pts',(-19.3067989983835,26.1240504241194,121.907695937297)) ;
#86288=CARTESIAN_POINT('Ctrl Pts',(-19.5704318398782,26.1340852226263,121.913051573615)) ;
#86289=CARTESIAN_POINT('Ctrl Pts',(-19.824351246944,26.1439301066057,121.9627151315)) ;
#86290=CARTESIAN_POINT('Ctrl Pts',(-20.0693695516345,26.1539159634237,122.056561537333)) ;
#86291=CARTESIAN_POINT('Ctrl Pts',(-20.2933941815534,26.1638507775985,122.19072291664)) ;
#86292=CARTESIAN_POINT('Ctrl Pts',(-20.4929379375906,26.1739082773838,122.36397713695)) ;
#86293=CARTESIAN_POINT('Ctrl Pts',(-20.6558144439717,26.1837300358021,122.564237995494)) ;
#86294=CARTESIAN_POINT('Ctrl Pts',(-20.7848455998996,26.1937856935861,122.79482096552)) ;
#86295=CARTESIAN_POINT('Ctrl Pts',(-20.8704620781849,26.2037278757661,123.041679298249)) ;
#86296=CARTESIAN_POINT('Ctrl Pts',(-20.9125411179837,26.2136330844608,123.298550407497)) ;
#86297=CARTESIAN_POINT('Ctrl Pts',(-20.9092518862155,26.2236748754233,123.56241297677)) ;
#86298=CARTESIAN_POINT('Ctrl Pts',(-20.8608770737848,26.2335826498955,123.81825615933)) ;
#86299=CARTESIAN_POINT('Ctrl Pts',(-20.7683065805399,26.2435941501231,124.064531536108)) ;
#86300=CARTESIAN_POINT('Ctrl Pts',(-20.6336276204181,26.2536269105158,124.291186385178)) ;
#86301=CARTESIAN_POINT('Ctrl Pts',(-20.4651029134243,26.2634774796507,124.487687379059)) ;
#86302=CARTESIAN_POINT('Ctrl Pts',(-20.2625522855935,26.2734660891806,124.654609276642)) ;
#86303=CARTESIAN_POINT('Ctrl Pts',(-20.0354400287525,26.2833947452047,124.783063120699)) ;
#86304=CARTESIAN_POINT('Ctrl Pts',(-19.7881531187985,26.2933824913825,124.871070996956)) ;
#86305=CARTESIAN_POINT('Ctrl Pts',(-19.5280420904567,26.3034184803182,124.914573869556)) ;
#86306=CARTESIAN_POINT('Ctrl Pts',(-19.2690516259357,26.3132733501318,124.912723418728)) ;
#86307=CARTESIAN_POINT('Ctrl Pts',(-19.0105800370941,26.3232727913736,124.86560866309)) ;
#86308=CARTESIAN_POINT('Ctrl Pts',(-18.7666075707734,26.3331678655537,124.775514885921)) ;
#86309=CARTESIAN_POINT('Ctrl Pts',(-18.5383077888514,26.3432285213934,124.642249303302)) ;
#86310=CARTESIAN_POINT('Ctrl Pts',(-18.3407235540066,26.353077395589,124.475043878373)) ;
#86311=CARTESIAN_POINT('Ctrl Pts',(-18.1716552019844,26.3631061075523,124.272882308973)) ;
#86312=CARTESIAN_POINT('Ctrl Pts',(-18.040865209082,26.3731355081354,124.044055902173)) ;
#86313=CARTESIAN_POINT('Ctrl Pts',(-17.9529323432651,26.3829757017522,123.800871133778)) ;
#86314=CARTESIAN_POINT('Ctrl Pts',(-17.907349688925,26.3929791243274,123.542000520602)) ;
#86315=CARTESIAN_POINT('Ctrl Pts',(-17.9074933099312,26.4029646614205,123.279546917314)) ;
#86316=CARTESIAN_POINT('Ctrl Pts',(-17.9537071122485,26.4130056659073,123.019784028195)) ;
#86317=CARTESIAN_POINT('Ctrl Pts',(-18.0422247319121,26.4228492048485,122.776701044052)) ;
#86318=CARTESIAN_POINT('Ctrl Pts',(-18.172959280111,26.4328342358393,122.549236855608)) ;
#86319=CARTESIAN_POINT('Ctrl Pts',(-18.3404039267093,26.4427736983613,122.348721052526)) ;
#86320=CARTESIAN_POINT('Ctrl Pts',(-18.5421292540438,26.4528134305851,122.17870944488)) ;
#86321=CARTESIAN_POINT('Ctrl Pts',(-18.7668321702435,26.4627016109023,122.048175439295)) ;
#86322=CARTESIAN_POINT('Ctrl Pts',(-19.0130942013059,26.4726911266048,121.957267850095)) ;
#86323=CARTESIAN_POINT('Ctrl Pts',(-19.270636423452,26.4826496772595,121.910844672131)) ;
#86324=CARTESIAN_POINT('Ctrl Pts',(-19.5307953770956,26.4925490843645,121.909202223713)) ;
#86325=CARTESIAN_POINT('Ctrl Pts',(-19.7910846414141,26.5025976707808,121.953512811704)) ;
#86326=CARTESIAN_POINT('Ctrl Pts',(-20.0360368235489,26.5124904897453,122.040759031323)) ;
#86327=CARTESIAN_POINT('Ctrl Pts',(-20.2660528706653,26.5225616072751,122.171557281645)) ;
#86328=CARTESIAN_POINT('Ctrl Pts',(-20.4649953247139,26.5323773012411,122.335824675937)) ;
#86329=CARTESIAN_POINT('Ctrl Pts',(-20.6368891208767,26.5424436787384,122.536824123293)) ;
#86330=CARTESIAN_POINT('Ctrl Pts',(-20.7690314537872,26.5523426648203,122.760972791709)) ;
#86331=CARTESIAN_POINT('Ctrl Pts',(-20.8617289021231,26.5623968448138,123.008329329804)) ;
#86332=CARTESIAN_POINT('Ctrl Pts',(-20.9094601027412,26.5722676577465,123.263357508459)) ;
#86333=CARTESIAN_POINT('Ctrl Pts',(-20.9122321988059,26.5823415586003,123.528012047214)) ;
#86334=CARTESIAN_POINT('Ctrl Pts',(-20.8703917027367,26.592161713987,123.782723049251)) ;
#86335=CARTESIAN_POINT('Ctrl Pts',(-20.7829899901851,26.6022404209392,124.032674888992)) ;
#86336=CARTESIAN_POINT('Ctrl Pts',(-20.6564493553006,26.612092009478,124.25860286663)) ;
#86337=CARTESIAN_POINT('Ctrl Pts',(-20.4891684822601,26.622165126003,124.463697321808)) ;
#86338=CARTESIAN_POINT('Ctrl Pts',(-20.293323576881,26.6320076430988,124.632686826274)) ;
#86339=CARTESIAN_POINT('Ctrl Pts',(-20.0684805251643,26.6419881046528,124.76769750117)) ;
#86340=CARTESIAN_POINT('Ctrl Pts',(-19.8224939925488,26.6520063546435,124.861502416363)) ;
#86341=CARTESIAN_POINT('Ctrl Pts',(-19.5674893463834,26.6618905148373,124.91103746618)) ;
#86342=CARTESIAN_POINT('Ctrl Pts',(-19.3030567708649,26.6719556618123,124.915566855908)) ;
#86343=CARTESIAN_POINT('Ctrl Pts',(-19.0475793987206,26.6817974854531,124.875168472208)) ;
#86344=CARTESIAN_POINT('Ctrl Pts',(-18.7981276860572,26.6918269579139,124.79009847604)) ;
#86345=CARTESIAN_POINT('Ctrl Pts',(-18.5676426643981,26.701853813176,124.662390118096)) ;
#86346=CARTESIAN_POINT('Ctrl Pts',(-18.3661950342201,26.7116970632865,124.500120225689)) ;
#86347=CARTESIAN_POINT('Ctrl Pts',(-18.1921722448789,26.7217455028697,124.301522698417)) ;
#86348=CARTESIAN_POINT('Ctrl Pts',(-18.0569733160775,26.7316949971176,124.077726969622)) ;
#86349=CARTESIAN_POINT('Ctrl Pts',(-17.9623479206744,26.7416028528436,123.835146450497)) ;
#86350=CARTESIAN_POINT('Ctrl Pts',(-17.9107817759331,26.7516623294935,123.57590066682)) ;
#86351=CARTESIAN_POINT('Ctrl Pts',(-17.9047865023787,26.7615031389022,123.317331030199)) ;
#86352=CARTESIAN_POINT('Ctrl Pts',(-17.9443188755689,26.771565289203,123.055908426171)) ;
#86353=CARTESIAN_POINT('Ctrl Pts',(-18.0275281430875,26.7814624503255,122.809476370172)) ;
#86354=CARTESIAN_POINT('Ctrl Pts',(-18.1519197086005,26.7913936247296,122.580053321706)) ;
#86355=CARTESIAN_POINT('Ctrl Pts',(-18.3162992678989,26.8014358284546,122.373607725889)) ;
#86356=CARTESIAN_POINT('Ctrl Pts',(-18.5108502149347,26.8113224108851,122.201394321902)) ;
#86357=CARTESIAN_POINT('Ctrl Pts',(-18.7344911406208,26.8213158466334,122.063754577682)) ;
#86358=CARTESIAN_POINT('Ctrl Pts',(-18.9774833859817,26.8312603149915,121.96757970157)) ;
#86359=CARTESIAN_POINT('Ctrl Pts',(-19.2335820350933,26.8412121312371,121.91453316318)) ;
#86360=CARTESIAN_POINT('Ctrl Pts',(-19.4972322377189,26.8512495673516,121.906934424089)) ;
#86361=CARTESIAN_POINT('Ctrl Pts',(-19.754305398308,26.8611345265279,121.944403815041)) ;
#86362=CARTESIAN_POINT('Ctrl Pts',(-20.0038371906887,26.8711326447399,122.026561032475)) ;
#86363=CARTESIAN_POINT('Ctrl Pts',(-20.2336644999362,26.8810535772519,122.149706995992)) ;
#86364=CARTESIAN_POINT('Ctrl Pts',(-20.4411151613036,26.8910948774739,122.312763749208)) ;
#86365=CARTESIAN_POINT('Ctrl Pts',(-20.6146912031061,26.9010017958639,122.506803957199)) ;
#86366=CARTESIAN_POINT('Ctrl Pts',(-20.7529734778652,26.910937587573,122.728283521879)) ;
#86367=CARTESIAN_POINT('Ctrl Pts',(-20.8514823737436,26.9209784821509,122.973063068783)) ;
#86368=CARTESIAN_POINT('Ctrl Pts',(-20.9053481968387,26.9308656838647,123.227257943129)) ;
#86369=CARTESIAN_POINT('Ctrl Pts',(-20.9147883410893,26.9408579516263,123.489656489309)) ;
#86370=CARTESIAN_POINT('Ctrl Pts',(-20.8786067103794,26.9508064726481,123.74859249786)) ;
#86371=CARTESIAN_POINT('Ctrl Pts',(-20.7984720557952,26.9607432462258,123.997098137103)) ;
#86372=CARTESIAN_POINT('Ctrl Pts',(-20.676104628499,26.9707262943668,124.229192313943)) ;
#86373=CARTESIAN_POINT('Ctrl Pts',(-20.5139774785616,26.9807700019769,124.437430943901)) ;
#86374=CARTESIAN_POINT('Ctrl Pts',(-20.3227007873807,26.9905986951302,124.61104899263)) ;
#86375=CARTESIAN_POINT('Ctrl Pts',(-20.0988745919875,27.0006734442596,124.75238354413)) ;
#86376=CARTESIAN_POINT('Ctrl Pts',(-19.8589158285045,27.0105387700552,124.850593645606)) ;
#86377=CARTESIAN_POINT('Ctrl Pts',(-19.6017027315997,27.0205609444121,124.907173107382)) ;
#86378=CARTESIAN_POINT('Ctrl Pts',(-19.3384167298905,27.030586997619,124.917590734457)) ;
#86379=CARTESIAN_POINT('Ctrl Pts',(-19.0817902884042,27.0404406944653,124.883165473566)) ;
#86380=CARTESIAN_POINT('Ctrl Pts',(-18.8321269948554,27.0504000992183,124.804605397786)) ;
#86381=CARTESIAN_POINT('Ctrl Pts',(-18.5982965329107,27.0604383449232,124.682527849518)) ;
#86382=CARTESIAN_POINT('Ctrl Pts',(-18.3923088563404,27.0703125290852,124.524671749467)) ;
#86383=CARTESIAN_POINT('Ctrl Pts',(-18.213440473293,27.0803823122231,124.329704461917)) ;
#86384=CARTESIAN_POINT('Ctrl Pts',(-18.074335807759,27.0902155672439,124.111906520483)) ;
#86385=CARTESIAN_POINT('Ctrl Pts',(-17.9724962914812,27.1002459933756,123.868794804679)) ;
#86386=CARTESIAN_POINT('Ctrl Pts',(-17.9151518381184,27.1102776055626,123.61147237248)) ;
#86387=CARTESIAN_POINT('Ctrl Pts',(-17.9030590057314,27.1201073024172,123.353458137196)) ;
#86388=CARTESIAN_POINT('Ctrl Pts',(-17.9357095844985,27.1300967443197,123.092976875081)) ;
#86389=CARTESIAN_POINT('Ctrl Pts',(-18.0141505189305,27.1401406363354,122.840961680301)) ;
#86390=CARTESIAN_POINT('Ctrl Pts',(-18.1320070501894,27.1499621981046,122.611342543819)) ;
#86391=CARTESIAN_POINT('Ctrl Pts',(-18.2908176421164,27.1599977697288,122.400792255072)) ;
#86392=CARTESIAN_POINT('Ctrl Pts',(-18.4841896216697,27.1700270440106,122.221709205105)) ;
#86393=CARTESIAN_POINT('Ctrl Pts',(-18.7010325739723,27.1798608811293,122.08111845669)) ;
#86394=CARTESIAN_POINT('Ctrl Pts',(-18.9441365822861,27.1899132772174,121.97778844473)) ;
#86395=CARTESIAN_POINT('Ctrl Pts',(-19.1986307271689,27.1998500441679,121.919247113411)) ;
#86396=CARTESIAN_POINT('Ctrl Pts',(-19.4593067664465,27.2097842791472,121.905113637741)) ;
#86397=CARTESIAN_POINT('Ctrl Pts',(-19.7207933748905,27.219808042474,121.936899749053)) ;
#86398=CARTESIAN_POINT('Ctrl Pts',(-19.9693907811413,27.2296943838587,122.012371578883)) ;
#86399=CARTESIAN_POINT('Ctrl Pts',(-20.2037993675098,27.2396834326256,122.130541837784)) ;
#86400=CARTESIAN_POINT('Ctrl Pts',(-20.4148911017479,27.249724653323,122.288871926613)) ;
#86401=CARTESIAN_POINT('Ctrl Pts',(-20.5918449134471,27.2595572935009,122.477157471636)) ;
#86402=CARTESIAN_POINT('Ctrl Pts',(-20.7363711758217,27.2695512228089,122.696442446085)) ;
#86403=CARTESIAN_POINT('Ctrl Pts',(-20.8404837011343,27.2795804304894,122.938566164147)) ;
#86404=CARTESIAN_POINT('Ctrl Pts',(-20.9004632009322,27.2894562421935,123.191081286783)) ;
#86405=CARTESIAN_POINT('Ctrl Pts',(-20.9161620820543,27.2994554691649,123.453345856358)) ;
#86406=CARTESIAN_POINT('Ctrl Pts',(-20.8865937388302,27.3093649503206,123.712111167712)) ;
#86407=CARTESIAN_POINT('Ctrl Pts',(-20.8114565304405,27.3194181806215,123.9653601692)) ;
#86408=CARTESIAN_POINT('Ctrl Pts',(-20.695723180066,27.3292887971726,124.197519423031)) ;
#86409=CARTESIAN_POINT('Ctrl Pts',(-20.5395590565441,27.3393104589046,124.409577578881)) ;
#86410=CARTESIAN_POINT('Ctrl Pts',(-20.3484964827814,27.3493332720857,124.590894769313)) ;
#86411=CARTESIAN_POINT('Ctrl Pts',(-20.1325252181775,27.3592004365456,124.734373686293)) ;
#86412=CARTESIAN_POINT('Ctrl Pts',(-19.8921052555751,27.3691938787656,124.840061281651)) ;
#86413=CARTESIAN_POINT('Ctrl Pts',(-19.6358971489778,27.3792255523659,124.902135847813)) ;
#86414=CARTESIAN_POINT('Ctrl Pts',(-19.3771491513025,27.3890919874789,124.918905570282)) ;
#86415=CARTESIAN_POINT('Ctrl Pts',(-19.1162550336676,27.399079438012,124.890574288521)) ;
#86416=CARTESIAN_POINT('Ctrl Pts',(-18.8652095381394,27.4090243678399,124.817799802531)) ;
#86417=CARTESIAN_POINT('Ctrl Pts',(-18.6283777604426,27.4190692628951,124.701277213198)) ;
#86418=CARTESIAN_POINT('Ctrl Pts',(-18.4190826873744,27.4289313245809,124.548398528838)) ;
#86419=CARTESIAN_POINT('Ctrl Pts',(-18.23679990877,27.4389230473678,124.35943784464)) ;
#86420=CARTESIAN_POINT('Ctrl Pts',(-18.0910351330655,27.4488552616077,124.142920914045)) ;
#86421=CARTESIAN_POINT('Ctrl Pts',(-17.9844514742124,27.4587945801734,123.90445397346)) ;
#86422=CARTESIAN_POINT('Ctrl Pts',(-17.9204596210356,27.4688387549493,123.648382078966)) ;
#86423=CARTESIAN_POINT('Ctrl Pts',(-17.902082443692,27.4787093090143,123.389646586281)) ;
#86424=CARTESIAN_POINT('Ctrl Pts',(-17.9284117059881,27.4886742913685,123.129103791897)) ;
#86425=CARTESIAN_POINT('Ctrl Pts',(-18.0004358375775,27.4987049942583,122.875545886623)) ;
#86426=CARTESIAN_POINT('Ctrl Pts',(-18.1134828367361,27.5085973342835,122.641417708606)) ;
#86427=CARTESIAN_POINT('Ctrl Pts',(-18.2678736241984,27.5186505674435,122.427083046342)) ;
#86428=CARTESIAN_POINT('Ctrl Pts',(-18.4538449647151,27.5285318119202,122.245793517395)) ;
#86429=CARTESIAN_POINT('Ctrl Pts',(-18.6715808971833,27.5385649327912,122.097192547089)) ;
#86430=CARTESIAN_POINT('Ctrl Pts',(-18.9081664411668,27.5484461430663,121.990047207349)) ;
#86431=CARTESIAN_POINT('Ctrl Pts',(-19.1642609051452,27.5585082188356,121.924381854683)) ;
#86432=CARTESIAN_POINT('Ctrl Pts',(-19.4225664239136,27.5683652772174,121.904494754885)) ;
#86433=CARTESIAN_POINT('Ctrl Pts',(-19.6839699262157,27.5783598325064,121.929577621368)) ;
#86434=CARTESIAN_POINT('Ctrl Pts',(-19.9354082337427,27.5882857200419,121.999117799901)) ;
#86435=CARTESIAN_POINT('Ctrl Pts',(-20.1732877832902,27.5983107400372,122.112287014641)) ;
#86436=CARTESIAN_POINT('Ctrl Pts',(-20.3852469318587,27.6082081171408,122.263036295737)) ;
#86437=CARTESIAN_POINT('Ctrl Pts',(-20.5699322318413,27.6181983542217,122.44963382705)) ;
#86438=CARTESIAN_POINT('Ctrl Pts',(-20.7196829783269,27.6282349670305,122.666746029416)) ;
#86439=CARTESIAN_POINT('Ctrl Pts',(-20.8278068728803,27.6380848504485,122.901936609501)) ;
#86440=CARTESIAN_POINT('Ctrl Pts',(-20.8949783481644,27.648088467351,123.156067646929)) ;
#86441=CARTESIAN_POINT('Ctrl Pts',(-20.9168353812002,27.6580778791161,123.417709468201)) ;
#86442=CARTESIAN_POINT('Ctrl Pts',(-20.8927038903756,27.6680966404609,123.679858425827)) ;
#86443=CARTESIAN_POINT('Ctrl Pts',(-20.8017637690144,27.681315315842,124.015169943229)) ;
#86444=CARTESIAN_POINT('Ctrl Pts',(-20.624397640746,27.6946256230867,124.321149899939)) ;
#86445=CARTESIAN_POINT('Ctrl Pts',(-20.3779433771167,27.7078632893127,124.566721861766)) ;
#86446=CARTESIAN_POINT('Ctrl Pts',(-20.1646154796001,27.7177829847234,124.716537787326)) ;
#86447=CARTESIAN_POINT('Ctrl Pts',(-19.9252314219541,27.727835851722,124.828242513711)) ;
#86448=CARTESIAN_POINT('Ctrl Pts',(-19.6751407014436,27.7376912600512,124.895632476655)) ;
#86449=CARTESIAN_POINT('Ctrl Pts',(-19.412428193496,27.7477298917278,124.919430792106)) ;
#86450=CARTESIAN_POINT('Ctrl Pts',(-19.0641209038591,27.7610320739948,124.889619359484)) ;
#86451=CARTESIAN_POINT('Ctrl Pts',(-18.6502903905597,27.7775770870777,124.740836279188)) ;
#86452=CARTESIAN_POINT('Ctrl Pts',(-18.3098859245536,27.7942291031539,124.458090863763)) ;
#86453=CARTESIAN_POINT('Ctrl Pts',(-18.1090493187269,27.8074521940591,124.17447204272)) ;
#86454=CARTESIAN_POINT('Ctrl Pts',(-17.9965232918457,27.8174131536185,123.938133979673)) ;
#86455=CARTESIAN_POINT('Ctrl Pts',(-17.9266087730233,27.8274379503696,123.684145144491)) ;
#86456=CARTESIAN_POINT('Ctrl Pts',(-17.8934656932994,27.8406623977654,123.338168391895)) ;
#86457=CARTESIAN_POINT('Ctrl Pts',(-17.9661155358838,27.8572961824645,122.902139051415)) ;
#86458=CARTESIAN_POINT('Ctrl Pts',(-18.2260073081097,27.8771988491894,122.441354547989)) ;
#86459=CARTESIAN_POINT('Ctrl Pts',(-18.6269746119238,27.8970990769713,122.096481259438)) ;
#86460=CARTESIAN_POINT('Ctrl Pts',(-19.1218890723207,27.9170165645028,121.908622605301)) ;
#86461=CARTESIAN_POINT('Ctrl Pts',(-19.6515477387723,27.9369460903197,121.90059571952)) ;
#86462=CARTESIAN_POINT('Ctrl Pts',(-20.1529442502027,27.956908358206,122.07417484712)) ;
#86463=CARTESIAN_POINT('Ctrl Pts',(-20.5634708106491,27.9767985531582,122.407134552226)) ;
#86464=CARTESIAN_POINT('Ctrl Pts',(-20.8369751729256,27.9966887979044,122.859670241796)) ;
#86465=CARTESIAN_POINT('Ctrl Pts',(-20.9394668766951,28.0167631704669,123.383205991598)) ;
#86466=CARTESIAN_POINT('Ctrl Pts',(-20.8584842588624,28.0365485478272,123.902864524186)) ;
#86467=CARTESIAN_POINT('Ctrl Pts',(-20.6042776799615,28.0565104218943,124.368499119697)) ;
#86468=CARTESIAN_POINT('Ctrl Pts',(-20.2051858780569,28.0764903973848,124.718841264619)) ;
#86469=CARTESIAN_POINT('Ctrl Pts',(-19.7150043467851,28.0963028272628,124.911309469325)) ;
#86470=CARTESIAN_POINT('Ctrl Pts',(-19.1842604378428,28.1162829353531,124.925752106115)) ;
#86471=CARTESIAN_POINT('Ctrl Pts',(-18.6824773897549,28.1361773189503,124.758643613806)) ;
#86472=CARTESIAN_POINT('Ctrl Pts',(-18.2670496367191,28.1561042469275,124.430319759425)) ;
#86473=CARTESIAN_POINT('Ctrl Pts',(-17.9883198062167,28.1759991042288,123.980833693048)) ;
#86474=CARTESIAN_POINT('Ctrl Pts',(-17.8794805614305,28.1960382978324,123.459516608282)) ;
#86475=CARTESIAN_POINT('Ctrl Pts',(-17.9544486755063,28.2158782657432,122.937505697659)) ;
#86476=CARTESIAN_POINT('Ctrl Pts',(-18.2027332815713,28.2357930827073,122.470098177361)) ;
#86477=CARTESIAN_POINT('Ctrl Pts',(-18.5964066329864,28.2557353281035,122.115256848635)) ;
#86478=CARTESIAN_POINT('Ctrl Pts',(-19.0856168086369,28.275607376218,121.915866271612)) ;
#86479=CARTESIAN_POINT('Ctrl Pts',(-19.6169218061426,28.2956184411721,121.895642781133)) ;
#86480=CARTESIAN_POINT('Ctrl Pts',(-20.1188292935515,28.3154299654757,122.055652903489)) ;
#86481=CARTESIAN_POINT('Ctrl Pts',(-20.5414244265229,28.3355251774391,122.381920562138)) ;
#86482=CARTESIAN_POINT('Ctrl Pts',(-20.8229842740963,28.3553059013589,122.826156087312)) ;
#86483=CARTESIAN_POINT('Ctrl Pts',(-20.9383586766976,28.3752969770017,123.344606135062)) ;
#86484=CARTESIAN_POINT('Ctrl Pts',(-20.8698588440805,28.3951789160447,123.868727080192)) ;
#86485=CARTESIAN_POINT('Ctrl Pts',(-20.6263861212141,28.415131520548,124.33974290189)) ;
#86486=CARTESIAN_POINT('Ctrl Pts',(-20.2377379988083,28.4350303892786,124.69852394791)) ;
#86487=CARTESIAN_POINT('Ctrl Pts',(-19.7505120225895,28.4549237890882,124.903632562329)) ;
#86488=CARTESIAN_POINT('Ctrl Pts',(-19.2219604499456,28.4748329199282,124.931009679036)) ;
#86489=CARTESIAN_POINT('Ctrl Pts',(-18.7130412720916,28.4948650196918,124.774779736929)) ;
#86490=CARTESIAN_POINT('Ctrl Pts',(-18.3620584933981,28.5113970928613,124.510284590691)) ;
#86491=CARTESIAN_POINT('Ctrl Pts',(-18.1460674126106,28.5247324334672,124.234383966013)) ;
#86492=CARTESIAN_POINT('Ctrl Pts',(-18.0239856925731,28.5345749920069,124.006320082283)) ;
#86493=CARTESIAN_POINT('Ctrl Pts',(-17.9414030192515,28.5446268988568,123.755444503094)) ;
#86494=CARTESIAN_POINT('Ctrl Pts',(-17.8916917870985,28.5578754132477,123.410803822859)) ;
#86495=CARTESIAN_POINT('Ctrl Pts',(-17.9431871506201,28.5744745881955,122.972697293955)) ;
#86496=CARTESIAN_POINT('Ctrl Pts',(-18.1408539621108,28.5910633739905,122.578582469759)) ;
#86497=CARTESIAN_POINT('Ctrl Pts',(-18.3723983221645,28.6043391903325,122.317615113724)) ;
#86498=CARTESIAN_POINT('Ctrl Pts',(-18.577527292145,28.6143130411263,122.154436808147)) ;
#86499=CARTESIAN_POINT('Ctrl Pts',(-18.8092646056395,28.6243420732187,122.028922034954)) ;
#86500=CARTESIAN_POINT('Ctrl Pts',(-19.0557478273817,28.6342321987206,121.946437772454)) ;
#86501=CARTESIAN_POINT('Ctrl Pts',(-19.3153706733146,28.6442246769921,121.907264160908)) ;
#86502=CARTESIAN_POINT('Ctrl Pts',(-19.5768427425273,28.6541758920895,121.913598624698)) ;
#86503=CARTESIAN_POINT('Ctrl Pts',(-19.8356388835886,28.6642243938445,121.9659387871)) ;
#86504=CARTESIAN_POINT('Ctrl Pts',(-20.0765080850792,28.6740657434613,122.060169659542)) ;
#86505=CARTESIAN_POINT('Ctrl Pts',(-20.300843510358,28.6840520344815,122.196258449548)) ;
#86506=CARTESIAN_POINT('Ctrl Pts',(-20.4973109441294,28.6939886462101,122.368330827901)) ;
#86507=CARTESIAN_POINT('Ctrl Pts',(-20.6626341566035,28.7040385215777,122.57425065372)) ;
#86508=CARTESIAN_POINT('Ctrl Pts',(-20.7873624065296,28.7138889801131,122.801100887893)) ;
#86509=CARTESIAN_POINT('Ctrl Pts',(-20.8724691047688,28.7238609170659,123.048913631883)) ;
#86510=CARTESIAN_POINT('Ctrl Pts',(-20.9133208956479,28.733856373998,123.308428140769)) ;
#86511=CARTESIAN_POINT('Ctrl Pts',(-20.9081765057666,28.7438891810511,123.572012092005)) ;
#86512=CARTESIAN_POINT('Ctrl Pts',(-20.8585590805843,28.7537490676411,123.826338311456)) ;
#86513=CARTESIAN_POINT('Ctrl Pts',(-20.764789229398,28.7637381482063,124.071497059533)) ;
#86514=CARTESIAN_POINT('Ctrl Pts',(-20.6306361728563,28.7736696274155,124.295376547867)) ;
#86515=CARTESIAN_POINT('Ctrl Pts',(-20.4590320836787,28.7836554868614,124.493932716745)) ;
#86516=CARTESIAN_POINT('Ctrl Pts',(-20.2542272972785,28.7936936375086,124.660161314307)) ;
#86517=CARTESIAN_POINT('Ctrl Pts',(-20.0282560662824,28.803541728013,124.78635916123)) ;
#86518=CARTESIAN_POINT('Ctrl Pts',(-19.7786454124,28.813602636531,124.873435806326)) ;
#86519=CARTESIAN_POINT('Ctrl Pts',(-19.5219342752848,28.8234974836889,124.914980277803)) ;
#86520=CARTESIAN_POINT('Ctrl Pts',(-19.26072567087,28.833439155734,124.911999560869)) ;
#86521=CARTESIAN_POINT('Ctrl Pts',(-19.0023461124135,28.8434416828595,124.863503088264)) ;
#86522=CARTESIAN_POINT('Ctrl Pts',(-18.7557142855735,28.8534764740469,124.770209950683)) ;
#86523=CARTESIAN_POINT('Ctrl Pts',(-18.5330665031705,28.863321353906,124.638416591467)) ;
#86524=CARTESIAN_POINT('Ctrl Pts',(-18.3335959771311,28.8733072345245,124.467967806184)) ;
#86525=CARTESIAN_POINT('Ctrl Pts',(-18.1674022200289,28.8832419576177,124.266559871745)) ;
#86526=CARTESIAN_POINT('Ctrl Pts',(-18.0373647499672,28.8932997979289,124.036497815317)) ;
#86527=CARTESIAN_POINT('Ctrl Pts',(-17.950911814326,28.9031202853254,123.793301563566)) ;
#86528=CARTESIAN_POINT('Ctrl Pts',(-17.9065295280347,28.9131806866705,123.532709133583)) ;
#86529=CARTESIAN_POINT('Ctrl Pts',(-17.9084022908856,28.9231116522234,123.271710634104)) ;
#86530=CARTESIAN_POINT('Ctrl Pts',(-17.9550199869084,28.9330505145599,123.014749249068)) ;
#86531=CARTESIAN_POINT('Ctrl Pts',(-18.0458283672377,28.9430362454861,122.768516340365)) ;
#86532=CARTESIAN_POINT('Ctrl Pts',(-18.1787394441072,28.9530606309135,122.541096570347)) ;
#86533=CARTESIAN_POINT('Ctrl Pts',(-18.3467919785273,28.9629639152668,122.342338042519)) ;
#86534=CARTESIAN_POINT('Ctrl Pts',(-18.5499731696622,28.9730239198448,122.173252013428)) ;
#86535=CARTESIAN_POINT('Ctrl Pts',(-18.7744434743641,28.9828671889139,122.044654486055)) ;
#86536=CARTESIAN_POINT('Ctrl Pts',(-19.0212126462486,28.9928577545216,121.955119711378)) ;
#86537=CARTESIAN_POINT('Ctrl Pts',(-19.2782134163419,29.0027858863004,121.910108935023)) ;
#86538=CARTESIAN_POINT('Ctrl Pts',(-19.5406963148018,29.0127737733813,121.909949720142)) ;
#86539=CARTESIAN_POINT('Ctrl Pts',(-19.8003636387641,29.02280972295,121.956024596532)) ;
#86540=CARTESIAN_POINT('Ctrl Pts',(-20.0437946869578,29.0326646093288,122.0444605937)) ;
#86541=CARTESIAN_POINT('Ctrl Pts',(-20.2715846639012,29.0426640236767,122.175375625611)) ;
#86542=CARTESIAN_POINT('Ctrl Pts',(-20.4713275194905,29.0525591888672,122.34193965665)) ;
#86543=CARTESIAN_POINT('Ctrl Pts',(-20.6418433631902,29.0626195075592,122.543928922245)) ;
#86544=CARTESIAN_POINT('Ctrl Pts',(-20.7720825546946,29.0724696393352,122.767656038512)) ;
#86545=CARTESIAN_POINT('Ctrl Pts',(-20.8637061447357,29.0825002097855,123.014799627036)) ;
#86546=CARTESIAN_POINT('Ctrl Pts',(-20.9103762630913,29.0925143604583,123.273804452751)) ;
#86547=CARTESIAN_POINT('Ctrl Pts',(-20.9117741336975,29.1024072940037,123.53378141723)) ;
#86548=CARTESIAN_POINT('Ctrl Pts',(-20.867883240844,29.112396807994,123.792574654758)) ;
#86549=CARTESIAN_POINT('Ctrl Pts',(-20.7801810778798,29.1223505786464,124.039048417847)) ;
#86550=CARTESIAN_POINT('Ctrl Pts',(-20.6496213778519,29.132398347307,124.268526107138)) ;
#86551=CARTESIAN_POINT('Ctrl Pts',(-20.4848587379141,29.1422400737468,124.46791155322)) ;
#86552=CARTESIAN_POINT('Ctrl Pts',(-20.2855219341304,29.1522255905695,124.638505213354)) ;
#86553=CARTESIAN_POINT('Ctrl Pts',(-20.0606187506956,29.1621649222651,124.771401656305)) ;
#86554=CARTESIAN_POINT('Ctrl Pts',(-19.8136216179253,29.1722046919626,124.864082795799)) ;
#86555=CARTESIAN_POINT('Ctrl Pts',(-19.558187368143,29.1820928532114,124.911871502229)) ;
#86556=CARTESIAN_POINT('Ctrl Pts',(-19.2957011783519,29.1920824077138,124.915102448404)) ;
#86557=CARTESIAN_POINT('Ctrl Pts',(-19.0374781818425,29.2020408222374,124.872643060304)) ;
#86558=CARTESIAN_POINT('Ctrl Pts',(-18.7917703837319,29.2119407350668,124.787095968834)) ;
#86559=CARTESIAN_POINT('Ctrl Pts',(-18.5613536456222,29.2219874347167,124.65825660223)) ;
#86560=CARTESIAN_POINT('Ctrl Pts',(-18.3596420924881,29.2318872950223,124.493892512925)) ;
#86561=CARTESIAN_POINT('Ctrl Pts',(-18.1869148909575,29.2419386992278,124.294103199834)) ;
#86562=CARTESIAN_POINT('Ctrl Pts',(-18.0536769669931,29.2518197361489,124.071184737114)) ;
#86563=CARTESIAN_POINT('Ctrl Pts',(-17.9597521892141,29.2618195683264,123.825804732125)) ;
#86564=CARTESIAN_POINT('Ctrl Pts',(-17.9100403484687,29.2717375713113,123.569907928987)) ;
#86565=CARTESIAN_POINT('Ctrl Pts',(-17.9055429199268,29.2817888771858,123.305853384214)) ;
#86566=CARTESIAN_POINT('Ctrl Pts',(-17.9459174143974,29.2916587005774,123.049589465829)) ;
#86567=CARTESIAN_POINT('Ctrl Pts',(-18.0318972364498,29.3017328666277,122.799266072468)) ;
#86568=CARTESIAN_POINT('Ctrl Pts',(-18.1565829873438,29.3115529507693,122.573255953319)) ;
#86569=CARTESIAN_POINT('Ctrl Pts',(-18.3226099186623,29.3216316775052,122.36697855623)) ;
#86570=CARTESIAN_POINT('Ctrl Pts',(-18.5174760158988,29.3314832581547,122.196440883835)) ;
#86571=CARTESIAN_POINT('Ctrl Pts',(-18.7437589213341,29.3415563864531,122.059171973647)) ;
#86572=CARTESIAN_POINT('Ctrl Pts',(-18.9848715208291,29.3513988643445,121.965485865843)) ;
#86573=CARTESIAN_POINT('Ctrl Pts',(-19.2419396876553,29.3613794709426,121.913527744618)) ;
#86574=CARTESIAN_POINT('Ctrl Pts',(-19.5051237744955,29.3713971799614,121.907465724619)) ;
#86575=CARTESIAN_POINT('Ctrl Pts',(-19.7620431375332,29.3812833589988,121.946175909808)) ;
#86576=CARTESIAN_POINT('Ctrl Pts',(-20.0125730392579,29.3913409715712,122.030311528781)) ;
#86577=CARTESIAN_POINT('Ctrl Pts',(-20.2405533557099,29.4012173649433,122.154388504609)) ;
#86578=CARTESIAN_POINT('Ctrl Pts',(-20.4463541851592,29.4112123930937,122.317580930784)) ;
#86579=CARTESIAN_POINT('Ctrl Pts',(-20.6208172138511,29.4212331399397,122.514846934847)) ;
#86580=CARTESIAN_POINT('Ctrl Pts',(-20.7570016708868,29.4311352086061,122.736578720449)) ;
#86581=CARTESIAN_POINT('Ctrl Pts',(-20.8538352390123,29.4411259484258,122.980616710616)) ;
#86582=CARTESIAN_POINT('Ctrl Pts',(-20.9064868502557,29.4510891446361,123.23707769916)) ;
#86583=CARTESIAN_POINT('Ctrl Pts',(-20.914410419633,29.4609933289362,123.497253000178)) ;
#86584=CARTESIAN_POINT('Ctrl Pts',(-20.8762358005154,29.4710537893271,123.758827580412)) ;
#86585=CARTESIAN_POINT('Ctrl Pts',(-20.7953305897781,29.4808943351979,124.004481871684)) ;
#86586=CARTESIAN_POINT('Ctrl Pts',(-20.6705730749621,29.4909565559097,124.237592816873)) ;
#86587=CARTESIAN_POINT('Ctrl Pts',(-20.5096749757579,29.5008536989262,124.441955772106)) ;
#86588=CARTESIAN_POINT('Ctrl Pts',(-20.3156640114165,29.5107848753434,124.616506656617)) ;
#86589=CARTESIAN_POINT('Ctrl Pts',(-20.0916629418475,29.520827089122,124.756019382219)) ;
#86590=CARTESIAN_POINT('Ctrl Pts',(-19.8506899321232,29.5307136293248,124.853178323577)) ;
#86591=CARTESIAN_POINT('Ctrl Pts',(-19.5938766834909,29.5407072239302,124.908009663912)) ;
#86592=CARTESIAN_POINT('Ctrl Pts',(-19.332712747215,29.5506510990877,124.917331744836)) ;
#86593=CARTESIAN_POINT('Ctrl Pts',(-19.0734479879124,29.5606116352025,124.881449299093)) ;
#86594=CARTESIAN_POINT('Ctrl Pts',(-18.8233593876915,29.5706082385252,124.800941689882)) ;
#86595=CARTESIAN_POINT('Ctrl Pts',(-18.5904051560722,29.5806413214798,124.677470404879)) ;
#86596=CARTESIAN_POINT('Ctrl Pts',(-18.3859961074744,29.5904924901813,124.518621309858)) ;
#86597=CARTESIAN_POINT('Ctrl Pts',(-18.2097416401463,29.6004549808802,124.325047682833)) ;
#86598=CARTESIAN_POINT('Ctrl Pts',(-18.0691118335263,29.6104834092979,124.102151585275)) ;
#86599=CARTESIAN_POINT('Ctrl Pts',(-17.9704269675126,29.6203937766625,123.861151262509)) ;
#86600=CARTESIAN_POINT('Ctrl Pts',(-17.9142776230811,29.6303286442776,123.606174600459)) ;
#86601=CARTESIAN_POINT('Ctrl Pts',(-17.9033816131702,29.6403697862566,123.342537736076)) ;
#86602=CARTESIAN_POINT('Ctrl Pts',(-17.9377116774726,29.6502569224598,123.084976886491)) ;
#86603=CARTESIAN_POINT('Ctrl Pts',(-18.0166487960382,29.6602492048632,122.834555046718)) ;
#86604=CARTESIAN_POINT('Ctrl Pts',(-18.1374177643865,29.6701977328284,122.60266731771)) ;
#86605=CARTESIAN_POINT('Ctrl Pts',(-18.2961113277449,29.6801344639905,122.395320977446)) ;
#86606=CARTESIAN_POINT('Ctrl Pts',(-18.4891133100422,29.6901176748505,122.217574840443)) ;
#86607=CARTESIAN_POINT('Ctrl Pts',(-18.7115763555757,29.7001607740004,122.075621485712)) ;
#86608=CARTESIAN_POINT('Ctrl Pts',(-18.949992826985,29.7099917382753,121.976031903192)) ;
#86609=CARTESIAN_POINT('Ctrl Pts',(-19.2081671628499,29.7200645906612,121.917784053486)) ;
#86610=CARTESIAN_POINT('Ctrl Pts',(-19.467127300379,29.729928718373,121.905550210389)) ;
#86611=CARTESIAN_POINT('Ctrl Pts',(-19.7284409010787,29.7399509205079,121.938343116302)) ;
#86612=CARTESIAN_POINT('Ctrl Pts',(-19.9800566224885,29.7499781134763,122.016652854863)) ;
#86613=CARTESIAN_POINT('Ctrl Pts',(-20.210400702207,29.7598337074433,122.135017062282)) ;
#86614=CARTESIAN_POINT('Ctrl Pts',(-20.4193129127433,29.7697908793086,122.292588450327)) ;
#86615=CARTESIAN_POINT('Ctrl Pts',(-20.5988052662756,29.779829723307,122.485901523046)) ;
#86616=CARTESIAN_POINT('Ctrl Pts',(-20.740066998357,29.7897037471826,122.703600137925)) ;
#86617=CARTESIAN_POINT('Ctrl Pts',(-20.8433563231969,29.799773573173,122.947193893449)) ;
#86618=CARTESIAN_POINT('Ctrl Pts',(-20.9015323318944,29.8096068170702,123.198990450446)) ;
#86619=CARTESIAN_POINT('Ctrl Pts',(-20.9161199372986,29.8196372448433,123.462166811631)) ;
#86620=CARTESIAN_POINT('Ctrl Pts',(-20.8840222579638,29.8296688615884,123.723840344967)) ;
#86621=CARTESIAN_POINT('Ctrl Pts',(-20.8090522677205,29.8394985385691,123.971017934646)) ;
#86622=CARTESIAN_POINT('Ctrl Pts',(-20.6910925085159,29.8494880554091,124.205545773944)) ;
#86623=CARTESIAN_POINT('Ctrl Pts',(-20.5328239158274,29.8595316675488,124.416758785664)) ;
#86624=CARTESIAN_POINT('Ctrl Pts',(-20.3448871273158,29.8693542738841,124.593710045622)) ;
#86625=CARTESIAN_POINT('Ctrl Pts',(-20.1246838233644,29.8793925037834,124.738944315077)) ;
#86626=CARTESIAN_POINT('Ctrl Pts',(-19.8829956359094,29.8894035385753,124.842903601253)) ;
#86627=CARTESIAN_POINT('Ctrl Pts',(-19.629944134694,29.8993012695424,124.903033941421)) ;
#86628=CARTESIAN_POINT('Ctrl Pts',(-19.3679037961103,29.9092908973929,124.918797744218)) ;
#86629=CARTESIAN_POINT('Ctrl Pts',(-19.1080010949963,29.9192466878389,124.88883390131)) ;
#86630=CARTESIAN_POINT('Ctrl Pts',(-18.857809354991,29.929174086401,124.814884890953)) ;
#86631=CARTESIAN_POINT('Ctrl Pts',(-18.6219992187214,29.9391996815108,124.697407355649)) ;
#86632=CARTESIAN_POINT('Ctrl Pts',(-18.4130181328675,29.9490855321804,124.543075003642)) ;
#86633=CARTESIAN_POINT('Ctrl Pts',(-18.2316836984906,29.9590747120246,124.353257774373)) ;
#86634=CARTESIAN_POINT('Ctrl Pts',(-18.0857681933595,29.9691158991282,124.133401993258)) ;
#86635=CARTESIAN_POINT('Ctrl Pts',(-17.9820470555373,29.9789485426041,123.896746050801)) ;
#86636=CARTESIAN_POINT('Ctrl Pts',(-17.9192601596466,29.9889424923136,123.641732893525)) ;
#86637=CARTESIAN_POINT('Ctrl Pts',(-17.9021985043466,29.9989716150901,123.378728309774)) ;
#86638=CARTESIAN_POINT('Ctrl Pts',(-17.9302095800825,30.0088477460088,123.120696813041)) ;
#86639=CARTESIAN_POINT('Ctrl Pts',(-18.0031833304748,30.0188457810258,122.868329081507)) ;
#86640=CARTESIAN_POINT('Ctrl Pts',(-18.1177424147025,30.0287597107845,122.634304146691)) ;
#86641=CARTESIAN_POINT('Ctrl Pts',(-18.2731207173211,30.0388028985223,122.420990591887)) ;
#86642=CARTESIAN_POINT('Ctrl Pts',(-18.460477880612,30.0487027406627,122.240473905107)) ;
#86643=CARTESIAN_POINT('Ctrl Pts',(-18.6780038327348,30.0586940074707,122.093431755788)) ;
#86644=CARTESIAN_POINT('Ctrl Pts',(-18.9189236827015,30.0687261096027,121.986371546732)) ;
#86645=CARTESIAN_POINT('Ctrl Pts',(-19.170468246111,30.0785929905574,121.92348620404)) ;
#86646=CARTESIAN_POINT('Ctrl Pts',(-19.4323508510835,30.0885847818456,121.904376081853)) ;
#86647=CARTESIAN_POINT('Ctrl Pts',(-19.6945696776365,30.0986168977571,121.931642192667)) ;
#86648=CARTESIAN_POINT('Ctrl Pts',(-19.9440014901615,30.1084832145571,122.002451382793)) ;
#86649=CARTESIAN_POINT('Ctrl Pts',(-20.1803630188248,30.1184706960307,122.116477795654)) ;
#86650=CARTESIAN_POINT('Ctrl Pts',(-20.392566350984,30.1284156204096,122.269087188915)) ;
#86651=CARTESIAN_POINT('Ctrl Pts',(-20.5767324875527,30.1384605063203,122.458162856591)) ;
#86652=CARTESIAN_POINT('Ctrl Pts',(-20.7227801654869,30.1483226100329,122.67228121434)) ;
#86653=CARTESIAN_POINT('Ctrl Pts',(-20.8312983726913,30.1583141738574,122.911353552395)) ;
#86654=CARTESIAN_POINT('Ctrl Pts',(-20.8961724450446,30.1682469819203,123.164186294995)) ;
#86655=CARTESIAN_POINT('Ctrl Pts',(-20.916810994507,30.1781840841566,123.424522266059)) ;
#86656=CARTESIAN_POINT('Ctrl Pts',(-20.8912996042722,30.188236530427,123.687434835979)) ;
#86657=CARTESIAN_POINT('Ctrl Pts',(-20.8223241947769,30.1980826460086,123.936840767883)) ;
#86658=CARTESIAN_POINT('Ctrl Pts',(-20.7091987850365,30.2081306657235,124.17541152145)) ;
#86659=CARTESIAN_POINT('Ctrl Pts',(-20.5576650602483,30.2180726173524,124.388259700238)) ;
#86660=CARTESIAN_POINT('Ctrl Pts',(-20.3719976932811,30.2280113983515,124.57195695698)) ;
#86661=CARTESIAN_POINT('Ctrl Pts',(-20.1552718930415,30.2380374470776,124.721755575099)) ;
#86662=CARTESIAN_POINT('Ctrl Pts',(-19.9192454996909,30.2479243074858,124.830442864662)) ;
#86663=CARTESIAN_POINT('Ctrl Pts',(-19.6643659591417,30.2579555826176,124.897557475444)) ;
#86664=CARTESIAN_POINT('Ctrl Pts',(-19.4055132729224,30.267838559918,124.919346689653)) ;
#86665=CARTESIAN_POINT('Ctrl Pts',(-19.1423742851105,30.2778954133252,124.895462225033)) ;
#86666=CARTESIAN_POINT('Ctrl Pts',(-18.8081585492134,30.2910636544011,124.805348478367)) ;
#86667=CARTESIAN_POINT('Ctrl Pts',(-18.4999606060616,30.3044646836276,124.627109350704)) ;
#86668=CARTESIAN_POINT('Ctrl Pts',(-18.2548402508357,30.3176776003585,124.381034742561)) ;
#86669=CARTESIAN_POINT('Ctrl Pts',(-18.1049154570646,30.3276059948117,124.167570645998)) ;
#86670=CARTESIAN_POINT('Ctrl Pts',(-17.9935223888196,30.3375874949398,123.930052646589)) ;
#86671=CARTESIAN_POINT('Ctrl Pts',(-17.9250251231697,30.3476280382099,123.675258459608)) ;
#86672=CARTESIAN_POINT('Ctrl Pts',(-17.9019089621538,30.357477369993,123.417459308466)) ;
#86673=CARTESIAN_POINT('Ctrl Pts',(-17.9235593814897,30.3674727744647,123.155687344675)) ;
#86674=CARTESIAN_POINT('Ctrl Pts',(-17.9909293206155,30.3774891019133,122.901233828562)) ;
#86675=CARTESIAN_POINT('Ctrl Pts',(-18.1363619700471,30.3907127590798,122.585590307536)) ;
#86676=CARTESIAN_POINT('Ctrl Pts',(-18.3617445260575,30.4040070504692,122.313580619713)) ;
#86677=CARTESIAN_POINT('Ctrl Pts',(-18.6465310373536,30.4172914014007,122.111548083525)) ;
#86678=CARTESIAN_POINT('Ctrl Pts',(-18.8832363601411,30.4272637824625,121.999174549586)) ;
#86679=CARTESIAN_POINT('Ctrl Pts',(-19.1341844428468,30.4371721620881,121.929596295639)) ;
#86680=CARTESIAN_POINT('Ctrl Pts',(-19.3971607833827,30.4472261608362,121.904405542938)) ;
#86681=CARTESIAN_POINT('Ctrl Pts',(-19.6555624151399,30.4570883579525,121.924666180462)) ;
#86682=CARTESIAN_POINT('Ctrl Pts',(-19.9952854684949,30.4704354843266,122.01183022792)) ;
#86683=CARTESIAN_POINT('Ctrl Pts',(-20.3783427936636,30.486972449968,122.227450317524)) ;
#86684=CARTESIAN_POINT('Ctrl Pts',(-20.6669629084573,30.5036070541419,122.562246315872)) ;
#86685=CARTESIAN_POINT('Ctrl Pts',(-20.8186251415275,30.5168968473846,122.876913691283)) ;
#86686=CARTESIAN_POINT('Ctrl Pts',(-20.8898702450345,30.526849478644,123.128536989928)) ;
#86687=CARTESIAN_POINT('Ctrl Pts',(-20.9166526278365,30.5368014459487,123.388718812429)) ;
#86688=CARTESIAN_POINT('Ctrl Pts',(-20.8911983771875,30.5501687044125,123.739033428064)) ;
#86689=CARTESIAN_POINT('Ctrl Pts',(-20.7477475189037,30.5666855163617,124.154053346653)) ;
#86690=CARTESIAN_POINT('Ctrl Pts',(-20.4126988443248,30.586711411368,124.567435413989)) ;
#86691=CARTESIAN_POINT('Ctrl Pts',(-19.9614671654052,30.6065221414982,124.838987072851)) ;
#86692=CARTESIAN_POINT('Ctrl Pts',(-19.4406806653169,30.626499357628,124.942199667842)) ;
#86693=CARTESIAN_POINT('Ctrl Pts',(-18.9173904837054,30.6464262330233,124.86074682562)) ;
#86694=CARTESIAN_POINT('Ctrl Pts',(-18.4548551754709,30.6662476944996,124.608403042469)) ;
#86695=CARTESIAN_POINT('Ctrl Pts',(-18.1021138578036,30.6863220123089,124.208208372338)) ;
#86696=CARTESIAN_POINT('Ctrl Pts',(-17.9097086793361,30.7061699813168,123.716866447982)) ;
#86697=CARTESIAN_POINT('Ctrl Pts',(-17.8953715490996,30.72611701538,123.187016557676)) ;
#86698=CARTESIAN_POINT('Ctrl Pts',(-18.0624519723751,30.7460129663522,122.685261153681)) ;
#86699=CARTESIAN_POINT('Ctrl Pts',(-18.3899873246686,30.7659084459704,122.270164037835)) ;
#86700=CARTESIAN_POINT('Ctrl Pts',(-18.8408813750857,30.7858645569352,121.990764998331)) ;
#86701=CARTESIAN_POINT('Ctrl Pts',(-19.3586318139167,30.8057691049752,121.882458783378)) ;
#86702=CARTESIAN_POINT('Ctrl Pts',(-19.8818185744041,30.8256432292943,121.955925643777)) ;
#86703=CARTESIAN_POINT('Ctrl Pts',(-20.3522474723433,30.8456977592933,122.206355579186)) ;
#86704=CARTESIAN_POINT('Ctrl Pts',(-20.7048311303731,30.8655052730533,122.59744630561)) ;
#86705=CARTESIAN_POINT('Ctrl Pts',(-20.9055172328141,30.885488628821,123.089116826482)) ;
#86706=CARTESIAN_POINT('Ctrl Pts',(-20.9255113800788,30.905406931405,123.618128166974)) ;
#86707=CARTESIAN_POINT('Ctrl Pts',(-20.7655078140649,30.9252751468507,124.121480433858)) ;
#86708=CARTESIAN_POINT('Ctrl Pts',(-20.4398813109932,30.945325463647,124.543131309097)) ;
#86709=CARTESIAN_POINT('Ctrl Pts',(-19.9961416301673,30.9651015255295,124.825243045067)) ;
#86710=CARTESIAN_POINT('Ctrl Pts',(-19.4760428857146,30.9851561312219,124.940890724397)) ;
#86711=CARTESIAN_POINT('Ctrl Pts',(-18.9542245242808,31.0049498203778,124.872803577724)) ;
#86712=CARTESIAN_POINT('Ctrl Pts',(-18.4824553574321,31.0249165119722,124.630033633571)) ;
#86713=CARTESIAN_POINT('Ctrl Pts',(-18.1224338999949,31.0448765577232,124.240259071478)) ;
#86714=CARTESIAN_POINT('Ctrl Pts',(-17.9173964213131,31.0647748178734,123.752794316431)) ;
#86715=CARTESIAN_POINT('Ctrl Pts',(-17.8903757638579,31.0846697334226,123.22473469265)) ;
#86716=CARTESIAN_POINT('Ctrl Pts',(-18.0448284170245,31.1045799138362,122.718600932171)) ;
#86717=CARTESIAN_POINT('Ctrl Pts',(-18.3629565328079,31.1245157129505,122.29484956572)) ;
#86718=CARTESIAN_POINT('Ctrl Pts',(-18.8066023023989,31.1444535746046,122.005048043472)) ;
#86719=CARTESIAN_POINT('Ctrl Pts',(-19.3219837707938,31.1643726212422,121.883821949317)) ;
#86720=CARTESIAN_POINT('Ctrl Pts',(-19.8485586474663,31.1843215192964,121.945761987751)) ;
#86721=CARTESIAN_POINT('Ctrl Pts',(-20.3214530576657,31.2042273467395,122.183047702527)) ;
#86722=CARTESIAN_POINT('Ctrl Pts',(-20.62457405632,31.2208100421048,122.502904725448)) ;
#86723=CARTESIAN_POINT('Ctrl Pts',(-20.7912398187945,31.2340842558284,122.809407390215)) ;
#86724=CARTESIAN_POINT('Ctrl Pts',(-20.8750277230681,31.2441309750277,123.059747682737)) ;
#86725=CARTESIAN_POINT('Ctrl Pts',(-20.9135794146644,31.2539750096734,123.315566077138)) ;
#86726=CARTESIAN_POINT('Ctrl Pts',(-20.9056166911276,31.267309394578,123.665879105346)) ;
#86727=CARTESIAN_POINT('Ctrl Pts',(-20.7817240069621,31.2838966118777,124.089024590941)) ;
#86728=CARTESIAN_POINT('Ctrl Pts',(-20.5204927418564,31.3005298239156,124.44560763796)) ;
#86729=CARTESIAN_POINT('Ctrl Pts',(-20.2482842473179,31.3138122661878,124.664159228814)) ;
#86730=CARTESIAN_POINT('Ctrl Pts',(-20.0203552489676,31.323718154102,124.789870365395)) ;
#86731=CARTESIAN_POINT('Ctrl Pts',(-19.7720861356419,31.3337065722071,124.875118114952)) ;
#86732=CARTESIAN_POINT('Ctrl Pts',(-19.5118369240493,31.3437299994459,124.915827009597)) ;
#86733=CARTESIAN_POINT('Ctrl Pts',(-19.2516219194721,31.3536344305629,124.910938614496)) ;
#86734=CARTESIAN_POINT('Ctrl Pts',(-18.9093544512018,31.3668975831733,124.844874070695)) ;
#86735=CARTESIAN_POINT('Ctrl Pts',(-18.5909341743351,31.3802224810772,124.689988959161)) ;
#86736=CARTESIAN_POINT('Ctrl Pts',(-18.3276472878309,31.3934782246928,124.461818204276)) ;
#86737=CARTESIAN_POINT('Ctrl Pts',(-18.1623509832731,31.4034375981401,124.258944934311)) ;
#86738=CARTESIAN_POINT('Ctrl Pts',(-18.0346692467731,31.4133814220671,124.030912426066)) ;
#86739=CARTESIAN_POINT('Ctrl Pts',(-17.9478499345261,31.4234293662144,123.781565182109)) ;
#86740=CARTESIAN_POINT('Ctrl Pts',(-17.9062405916385,31.4332803374325,123.526042263013)) ;
#86741=CARTESIAN_POINT('Ctrl Pts',(-17.9089961332649,31.4432521548746,123.264037869211)) ;
#86742=CARTESIAN_POINT('Ctrl Pts',(-17.9573713255669,31.4532475771667,123.0058246328)) ;
#86743=CARTESIAN_POINT('Ctrl Pts',(-18.0504365475839,31.4632806422904,122.759146467247)) ;
#86744=CARTESIAN_POINT('Ctrl Pts',(-18.182455819894,31.4731459749556,122.53603494168)) ;
#86745=CARTESIAN_POINT('Ctrl Pts',(-18.3522600986835,31.4831065175532,122.336826203529)) ;
#86746=CARTESIAN_POINT('Ctrl Pts',(-18.555825302581,31.4931402030549,122.169258613365)) ;
#86747=CARTESIAN_POINT('Ctrl Pts',(-18.7818081775691,31.5030250350452,122.04108939127)) ;
#86748=CARTESIAN_POINT('Ctrl Pts',(-19.0310789742768,31.513092461805,121.952582039014)) ;
#86749=CARTESIAN_POINT('Ctrl Pts',(-19.2860425398375,31.5229309509638,121.909432534115)) ;
#86750=CARTESIAN_POINT('Ctrl Pts',(-19.5504588373335,31.532994432154,121.910897207184)) ;
#86751=CARTESIAN_POINT('Ctrl Pts',(-19.806252038689,31.5428885899691,121.957687925717)) ;
#86752=CARTESIAN_POINT('Ctrl Pts',(-20.0513987980626,31.5528304467134,122.047929059202)) ;
#86753=CARTESIAN_POINT('Ctrl Pts',(-20.2786389120805,31.5628329243848,122.180116472421)) ;
#86754=CARTESIAN_POINT('Ctrl Pts',(-20.4798154738035,31.5728677286891,122.350583181619)) ;
#86755=CARTESIAN_POINT('Ctrl Pts',(-20.6455040679005,31.5827126055348,122.549301249805)) ;
#86756=CARTESIAN_POINT('Ctrl Pts',(-20.7764127766709,31.5926984850903,122.776686313643)) ;
#86757=CARTESIAN_POINT('Ctrl Pts',(-20.8656033287989,31.6026332154488,123.022106958682)) ;
#86758=CARTESIAN_POINT('Ctrl Pts',(-20.9111243111444,31.6126910277617,123.282421856098)) ;
#86759=CARTESIAN_POINT('Ctrl Pts',(-20.9112068367647,31.6225116198861,123.540539997943)) ;
#86760=CARTESIAN_POINT('Ctrl Pts',(-20.865687331279,31.6325782054958,123.801079440899)) ;
#86761=CARTESIAN_POINT('Ctrl Pts',(-20.7770317266897,31.6424777860777,124.045722854565)) ;
#86762=CARTESIAN_POINT('Ctrl Pts',(-20.6453936142839,31.6525293857559,124.274672946805)) ;
#86763=CARTESIAN_POINT('Ctrl Pts',(-20.4790792984421,31.6624035721729,124.473913961419)) ;
#86764=CARTESIAN_POINT('Ctrl Pts',(-20.2772197656373,31.6724600480538,124.644405849723)) ;
#86765=CARTESIAN_POINT('Ctrl Pts',(-20.0524976022664,31.6823529793564,124.775234014397)) ;
#86766=CARTESIAN_POINT('Ctrl Pts',(-19.8043940631741,31.692415758069,124.866611670972)) ;
#86767=CARTESIAN_POINT('Ctrl Pts',(-19.5498389701363,31.7022582836502,124.912638260607)) ;
#86768=CARTESIAN_POINT('Ctrl Pts',(-19.287331714963,31.7122490490751,124.914410642322)) ;
#86769=CARTESIAN_POINT('Ctrl Pts',(-19.0300907670381,31.7221771250731,124.870797527224)) ;
#86770=CARTESIAN_POINT('Ctrl Pts',(-18.7826960536114,31.7321650354601,124.783086226261)) ;
#86771=CARTESIAN_POINT('Ctrl Pts',(-18.5534309522588,31.7422009475851,124.652751134591)) ;
#86772=CARTESIAN_POINT('Ctrl Pts',(-18.353644514985,31.7520559604328,124.487929296874)) ;
#86773=CARTESIAN_POINT('Ctrl Pts',(-18.1828179715406,31.762054906349,124.288330075696)) ;
#86774=CARTESIAN_POINT('Ctrl Pts',(-18.0503460097519,31.771951818797,124.064468215422)) ;
#86775=CARTESIAN_POINT('Ctrl Pts',(-17.9573008027146,31.7820056168905,123.817225770989)) ;
#86776=CARTESIAN_POINT('Ctrl Pts',(-17.9093501306192,31.7918865377172,123.562001493347)) ;
#86777=CARTESIAN_POINT('Ctrl Pts',(-17.9059334517401,31.8018910637149,123.299145753374)) ;
#86778=CARTESIAN_POINT('Ctrl Pts',(-17.9482120491376,31.8118750273324,123.040161685246)) ;
#86779=CARTESIAN_POINT('Ctrl Pts',(-18.0355138245975,31.8219146678837,122.791213968382)) ;
#86780=CARTESIAN_POINT('Ctrl Pts',(-18.1619308507885,31.8317586934984,122.565514127231)) ;
#86781=CARTESIAN_POINT('Ctrl Pts',(-18.3274742184349,31.8417496993158,122.361724868883)) ;
#86782=CARTESIAN_POINT('Ctrl Pts',(-18.5272092718872,31.8517874908479,122.189426042634)) ;
#86783=CARTESIAN_POINT('Ctrl Pts',(-18.7492365418585,31.8616318906363,122.05662983357)) ;
#86784=CARTESIAN_POINT('Ctrl Pts',(-18.9941697641335,31.8716166911931,121.962618647792)) ;
#86785=CARTESIAN_POINT('Ctrl Pts',(-19.2505857843533,31.8815562146042,121.912666206365)) ;
#86786=CARTESIAN_POINT('Ctrl Pts',(-19.5143572467387,31.8915959337052,121.908010594915)) ;
#86787=CARTESIAN_POINT('Ctrl Pts',(-19.771053035124,31.9014841056245,121.94848018403)) ;
#86788=CARTESIAN_POINT('Ctrl Pts',(-20.0194783206586,31.9114736680415,122.033298650539)) ;
#86789=CARTESIAN_POINT('Ctrl Pts',(-20.2485944427228,31.9214320402362,122.159742447755)) ;
#86790=CARTESIAN_POINT('Ctrl Pts',(-20.4514867933735,31.9313321144669,122.322607169725)) ;
#86791=CARTESIAN_POINT('Ctrl Pts',(-20.6255075792033,31.9413782108405,122.521118480551)) ;
#86792=CARTESIAN_POINT('Ctrl Pts',(-20.7605689119132,31.9512867948376,122.743753647204)) ;
#86793=CARTESIAN_POINT('Ctrl Pts',(-20.8563432165643,31.9612973734285,122.988771599216)) ;
#86794=CARTESIAN_POINT('Ctrl Pts',(-20.9076937965973,31.9713265315413,123.247285998441)) ;
#86795=CARTESIAN_POINT('Ctrl Pts',(-20.9136494977614,31.9811794133794,123.506125048581)) ;
#86796=CARTESIAN_POINT('Ctrl Pts',(-20.8749431252904,31.9911389745304,123.764982177503)) ;
#86797=CARTESIAN_POINT('Ctrl Pts',(-20.7907719543159,32.0011774091195,124.014974716044)) ;
#86798=CARTESIAN_POINT('Ctrl Pts',(-20.66695264249,32.0110506813466,124.243030789615)) ;
#86799=CARTESIAN_POINT('Ctrl Pts',(-20.5021399302121,32.0211239233402,124.450109642599)) ;
#86800=CARTESIAN_POINT('Ctrl Pts',(-20.3089945095504,32.0309442548732,124.621352168166)) ;
#86801=CARTESIAN_POINT('Ctrl Pts',(-20.0834973590324,32.0410229161,124.760153885266)) ;
#86802=CARTESIAN_POINT('Ctrl Pts',(-19.8427881240408,32.0508745113942,124.855626446842)) ;
#86803=CARTESIAN_POINT('Ctrl Pts',(-19.5836101770202,32.060947646623,124.909232373603)) ;
#86804=CARTESIAN_POINT('Ctrl Pts',(-19.3250477235278,32.0707900821481,124.91680672433)) ;
#86805=CARTESIAN_POINT('Ctrl Pts',(-19.0654135129984,32.0807708512815,124.879716005305)) ;
#86806=CARTESIAN_POINT('Ctrl Pts',(-18.8153951069858,32.0907879525253,124.797342091289)) ;
#86807=CARTESIAN_POINT('Ctrl Pts',(-18.5862068913827,32.1006764001272,124.674829079308)) ;
#86808=CARTESIAN_POINT('Ctrl Pts',(-18.3783323865825,32.110732114308,124.511717380021)) ;
#86809=CARTESIAN_POINT('Ctrl Pts',(-18.20504643639,32.1206073207219,124.318515886017)) ;
#86810=CARTESIAN_POINT('Ctrl Pts',(-18.0657523054065,32.1306023731946,124.095843008576)) ;
#86811=CARTESIAN_POINT('Ctrl Pts',(-17.9673624393521,32.1406242571567,123.851536926118)) ;
#86812=CARTESIAN_POINT('Ctrl Pts',(-17.9132447511668,32.150528229686,123.596960929366)) ;
#86813=CARTESIAN_POINT('Ctrl Pts',(-17.9036966014167,32.1605167263469,123.334645288358)) ;
#86814=CARTESIAN_POINT('Ctrl Pts',(-17.939924691972,32.1704805235949,123.07533896734)) ;
#86815=CARTESIAN_POINT('Ctrl Pts',(-18.0195480393415,32.1803845469029,122.827524176256)) ;
#86816=CARTESIAN_POINT('Ctrl Pts',(-18.1430776002173,32.1904450502245,122.593816083373)) ;
#86817=CARTESIAN_POINT('Ctrl Pts',(-18.3015440658301,32.2002855853644,122.389414603507)) ;
#86818=CARTESIAN_POINT('Ctrl Pts',(-18.4971343102704,32.210347806069,122.211511240556)) ;
#86819=CARTESIAN_POINT('Ctrl Pts',(-18.7171578358292,32.2202449598452,122.072795116102)) ;
#86820=CARTESIAN_POINT('Ctrl Pts',(-18.9584036223106,32.2301760932307,121.973254778566)) ;
#86821=CARTESIAN_POINT('Ctrl Pts',(-19.2161862551315,32.2402184683764,121.916771627792)) ;
#86822=CARTESIAN_POINT('Ctrl Pts',(-19.4757653790532,32.2501044061426,121.905874060276)) ;
#86823=CARTESIAN_POINT('Ctrl Pts',(-19.7361743618916,32.2601002491274,121.940186996512)) ;
#86824=CARTESIAN_POINT('Ctrl Pts',(-19.9853445011283,32.270042227006,122.01880797192)) ;
#86825=CARTESIAN_POINT('Ctrl Pts',(-20.2176224237473,32.280001601487,122.139380240724)) ;
#86826=CARTESIAN_POINT('Ctrl Pts',(-20.4263292540062,32.2899982173208,122.298965348353)) ;
#86827=CARTESIAN_POINT('Ctrl Pts',(-20.6045437074103,32.3000324358943,122.49330330733)) ;
#86828=CARTESIAN_POINT('Ctrl Pts',(-20.7440160089712,32.3098855031049,122.711454247693)) ;
#86829=CARTESIAN_POINT('Ctrl Pts',(-20.8452761241106,32.3198457609825,122.952809541801)) ;
#86830=CARTESIAN_POINT('Ctrl Pts',(-20.9031915155856,32.3298747876881,123.209934123648)) ;
#86831=CARTESIAN_POINT('Ctrl Pts',(-20.9155108381836,32.3397849947225,123.470061362045)) ;
#86832=CARTESIAN_POINT('Ctrl Pts',(-20.8830729146311,32.3497199053701,123.729125220497)) ;
#86833=CARTESIAN_POINT('Ctrl Pts',(-20.8050925575432,32.3597610355494,123.98120077394)) ;
#86834=CARTESIAN_POINT('Ctrl Pts',(-20.6865290803088,32.3696481759193,124.212412477173)) ;
#86835=CARTESIAN_POINT('Ctrl Pts',(-20.5283214706852,32.3796404534553,124.421965720278)) ;
#86836=CARTESIAN_POINT('Ctrl Pts',(-20.3368987653535,32.3895889967236,124.600050795474)) ;
#86837=CARTESIAN_POINT('Ctrl Pts',(-20.1179553075885,32.3995256715408,124.742318590014)) ;
#86838=CARTESIAN_POINT('Ctrl Pts',(-19.8765857645309,32.4095090924772,124.845198491733)) ;
#86839=CARTESIAN_POINT('Ctrl Pts',(-19.6194540624684,32.4195514076664,124.904530262006)) ;
#86840=CARTESIAN_POINT('Ctrl Pts',(-19.3612323588906,32.4293917251056,124.918456384701)) ;
#86841=CARTESIAN_POINT('Ctrl Pts',(-19.0995012622624,32.4394214291631,124.887349726659)) ;
#86842=CARTESIAN_POINT('Ctrl Pts',(-18.8475761386304,32.4494423858856,124.81065894568)) ;
#86843=CARTESIAN_POINT('Ctrl Pts',(-18.6160938856141,32.4593089281892,124.693811732837)) ;
#86844=CARTESIAN_POINT('Ctrl Pts',(-18.4041445829569,32.4693800281344,124.535355939284)) ;
#86845=CARTESIAN_POINT('Ctrl Pts',(-18.2270297897121,32.4792221023119,124.346861724585)) ;
#86846=CARTESIAN_POINT('Ctrl Pts',(-18.0828270949522,32.489182896899,124.128411540511)) ;
#86847=CARTESIAN_POINT('Ctrl Pts',(-17.978420138532,32.4992207697998,123.88617867698)) ;
#86848=CARTESIAN_POINT('Ctrl Pts',(-17.918171831887,32.5090950553439,123.633750736518)) ;
#86849=CARTESIAN_POINT('Ctrl Pts',(-17.9023810135821,32.5191648057578,123.369635645094)) ;
#86850=CARTESIAN_POINT('Ctrl Pts',(-17.9318454096663,32.5289980902925,123.112890613939)) ;
#86851=CARTESIAN_POINT('Ctrl Pts',(-18.0061909068655,32.5390284310925,122.860013828916)) ;
#86852=CARTESIAN_POINT('Ctrl Pts',(-18.1240350153628,32.5490603550921,122.624176778822)) ;
#86853=CARTESIAN_POINT('Ctrl Pts',(-18.2773901023668,32.558888890028,122.416362824848)) ;
#86854=CARTESIAN_POINT('Ctrl Pts',(-18.4671549519202,32.5688826677927,122.234811814169)) ;
#86855=CARTESIAN_POINT('Ctrl Pts',(-18.6865982599419,32.5789103782782,122.088899208413)) ;
#86856=CARTESIAN_POINT('Ctrl Pts',(-18.9245545564035,32.5887987891122,121.984478210373)) ;
#86857=CARTESIAN_POINT('Ctrl Pts',(-19.179155033595,32.5987756396477,121.921970498854)) ;
#86858=CARTESIAN_POINT('Ctrl Pts',(-19.4411893341139,32.6087674361982,121.904567510373)) ;
#86859=CARTESIAN_POINT('Ctrl Pts',(-19.703326580114,32.6188034422919,121.933365758691)) ;
#86860=CARTESIAN_POINT('Ctrl Pts',(-19.9519587960283,32.6286541765547,122.005505794216)) ;
#86861=CARTESIAN_POINT('Ctrl Pts',(-20.1877508005523,32.6386454350829,122.120918680607)) ;
#86862=CARTESIAN_POINT('Ctrl Pts',(-20.3985123625034,32.6485633299861,122.274300781478)) ;
#86863=CARTESIAN_POINT('Ctrl Pts',(-20.5814614274393,32.6585914716491,122.463947516891)) ;
#86864=CARTESIAN_POINT('Ctrl Pts',(-20.7267096138185,32.668476639765,122.679326125919)) ;
#86865=CARTESIAN_POINT('Ctrl Pts',(-20.8340502982722,32.678466003271,122.918892802554)) ;
#86866=CARTESIAN_POINT('Ctrl Pts',(-20.8979545030379,32.6885071382811,123.174908117759)) ;
#86867=CARTESIAN_POINT('Ctrl Pts',(-20.9164761609195,32.6983398064691,123.432631238316)) ;
#86868=CARTESIAN_POINT('Ctrl Pts',(-20.8902807920564,32.7083337094236,123.693949516132)) ;
#86869=CARTESIAN_POINT('Ctrl Pts',(-20.8183191956796,32.7183629945081,123.947496333409)) ;
#86870=CARTESIAN_POINT('Ctrl Pts',(-20.7055639452945,32.72823852295,124.181255541168)) ;
#86871=CARTESIAN_POINT('Ctrl Pts',(-20.5522820009705,32.7382388055661,124.394679958423)) ;
#86872=CARTESIAN_POINT('Ctrl Pts',(-20.366031988061,32.7481508216231,124.57682210646)) ;
#86873=CARTESIAN_POINT('Ctrl Pts',(-20.1482437968875,32.7581928969621,124.725815001188)) ;
#86874=CARTESIAN_POINT('Ctrl Pts',(-19.9112655719754,32.7680927296182,124.8331936985)) ;
#86875=CARTESIAN_POINT('Ctrl Pts',(-19.65704415951,32.7780851301962,124.898959513189)) ;
#86876=CARTESIAN_POINT('Ctrl Pts',(-19.3941345542646,32.7881191519556,124.919203661167)) ;
#86877=CARTESIAN_POINT('Ctrl Pts',(-19.1361107148346,32.7979837627968,124.894256925511)) ;
#86878=CARTESIAN_POINT('Ctrl Pts',(-18.8829224544705,32.807976162258,124.824605397838)) ;
#86879=CARTESIAN_POINT('Ctrl Pts',(-18.6449612635533,32.8180081155909,124.711138853319)) ;
#86880=CARTESIAN_POINT('Ctrl Pts',(-18.4336192368535,32.8278744745325,124.560921747617)) ;
#86881=CARTESIAN_POINT('Ctrl Pts',(-18.2490612673754,32.8378619500183,124.374355254994)) ;
#86882=CARTESIAN_POINT('Ctrl Pts',(-18.1001820205622,32.8478068562068,124.159518606616)) ;
#86883=CARTESIAN_POINT('Ctrl Pts',(-17.9899307415803,32.857851820867,123.919702152225)) ;
#86884=CARTESIAN_POINT('Ctrl Pts',(-17.9239755325999,32.8677136277719,123.669054864759)) ;
#86885=CARTESIAN_POINT('Ctrl Pts',(-17.9017602263012,32.8777063000777,123.407426433999)) ;
#86886=CARTESIAN_POINT('Ctrl Pts',(-17.9251935246742,32.887634971023,123.147548631717)) ;
#86887=CARTESIAN_POINT('Ctrl Pts',(-17.9931352135227,32.8975875132483,122.895003816011)) ;
#86888=CARTESIAN_POINT('Ctrl Pts',(-18.1043312287972,32.9075888692442,122.656829799846)) ;
#86889=CARTESIAN_POINT('Ctrl Pts',(-18.2558767004374,32.9176174815189,122.441233493131)) ;
#86890=CARTESIAN_POINT('Ctrl Pts',(-18.4392492938704,32.9274818160684,122.257982555295)) ;
#86891=CARTESIAN_POINT('Ctrl Pts',(-18.6541333399341,32.937474140145,122.107122522269)) ;
#86892=CARTESIAN_POINT('Ctrl Pts',(-18.8904036310431,32.9474016325109,121.996414241407)) ;
#86893=CARTESIAN_POINT('Ctrl Pts',(-19.144776160248,32.9574289910617,121.927756331862)) ;
#86894=CARTESIAN_POINT('Ctrl Pts',(-19.4035634233285,32.9673154091128,121.904356292453)) ;
#86895=CARTESIAN_POINT('Ctrl Pts',(-19.6662173972518,32.9773471438482,121.926427682475)) ;
#86896=CARTESIAN_POINT('Ctrl Pts',(-19.9173873207107,32.9872287250915,121.992537401162)) ;
#86897=CARTESIAN_POINT('Ctrl Pts',(-20.1575155915266,32.9972907031238,122.103143972169)) ;
#86898=CARTESIAN_POINT('Ctrl Pts',(-20.370483550717,33.0071477814855,122.250663584042)) ;
#86899=CARTESIAN_POINT('Ctrl Pts',(-20.5574852732715,33.0171423545915,122.435031329392)) ;
#86900=CARTESIAN_POINT('Ctrl Pts',(-20.7087098909113,33.0270681508791,122.647604267584)) ;
#86901=CARTESIAN_POINT('Ctrl Pts',(-20.8218893770371,33.0370935180488,122.885487342572)) ;
#86902=CARTESIAN_POINT('Ctrl Pts',(-20.8912556584646,33.0469895977027,123.136134795138)) ;
#86903=CARTESIAN_POINT('Ctrl Pts',(-20.9168234356785,33.0569846774083,123.397550614612)) ;
#86904=CARTESIAN_POINT('Ctrl Pts',(-20.8961029605947,33.0670097652241,123.660183142044)) ;
#86905=CARTESIAN_POINT('Ctrl Pts',(-20.8098991145045,33.0801935875914,123.99574300305)) ;
#86906=CARTESIAN_POINT('Ctrl Pts',(-20.6369446858756,33.0935157057373,124.304678709047)) ;
#86907=CARTESIAN_POINT('Ctrl Pts',(-20.3908204960889,33.1068949153649,124.555834602614)) ;
#86908=CARTESIAN_POINT('Ctrl Pts',(-20.1809494793358,33.1167331526091,124.706837071298)) ;
#86909=CARTESIAN_POINT('Ctrl Pts',(-19.942577781835,33.1268060758678,124.821869252031)) ;
#86910=CARTESIAN_POINT('Ctrl Pts',(-19.693263181732,33.1366627173229,124.892205355517)) ;
#86911=CARTESIAN_POINT('Ctrl Pts',(-19.4322613230798,33.146648092829,124.919218109963)) ;
#86912=CARTESIAN_POINT('Ctrl Pts',(-19.0841401970618,33.1599321242894,124.89401589364)) ;
#86913=CARTESIAN_POINT('Ctrl Pts',(-18.6686887473864,33.1764509161598,124.751538820693)) ;
#86914=CARTESIAN_POINT('Ctrl Pts',(-18.322123263724,33.1932366331664,124.470796884464)) ;
#86915=CARTESIAN_POINT('Ctrl Pts',(-18.1195228019478,33.2063497816754,124.191941939277)) ;
#86916=CARTESIAN_POINT('Ctrl Pts',(-18.0029823657326,33.2163853307556,123.955407109914)) ;
#86917=CARTESIAN_POINT('Ctrl Pts',(-17.9301367991554,33.226401386935,123.70244375215)) ;
#86918=CARTESIAN_POINT('Ctrl Pts',(-17.8928038233433,33.239579422801,123.358205398184)) ;
#86919=CARTESIAN_POINT('Ctrl Pts',(-17.9589484139631,33.2561812999881,122.921862723111)) ;
#86920=CARTESIAN_POINT('Ctrl Pts',(-18.2153509315473,33.276244444604,122.454328572859)) ;
#86921=CARTESIAN_POINT('Ctrl Pts',(-18.610517617413,33.2960453346877,122.106659477122)) ;
#86922=CARTESIAN_POINT('Ctrl Pts',(-19.1034981315604,33.3159884599664,121.912149478104)) ;
#86923=CARTESIAN_POINT('Ctrl Pts',(-19.6321521720369,33.335886505086,121.897927841427)) ;
#86924=CARTESIAN_POINT('Ctrl Pts',(-20.1341123261989,33.3557722647127,122.063632571961)) ;
#86925=CARTESIAN_POINT('Ctrl Pts',(-20.5525339489159,33.3758374398926,122.394216721666)) ;
#86926=CARTESIAN_POINT('Ctrl Pts',(-20.8296056794486,33.3956640829954,122.842560084467)) ;
#86927=CARTESIAN_POINT('Ctrl Pts',(-20.9388743874097,33.4155727924438,123.360152546638)) ;
#86928=CARTESIAN_POINT('Ctrl Pts',(-20.8648847574417,33.4355246294756,123.885402002908)) ;
#86929=CARTESIAN_POINT('Ctrl Pts',(-20.6147318866576,33.4555331041787,124.35462141048)) ;
#86930=CARTESIAN_POINT('Ctrl Pts',(-20.2239322170856,33.4753345629402,124.707141469447)) ;
#86931=CARTESIAN_POINT('Ctrl Pts',(-19.7330000970732,33.4952914511762,124.907967316448)) ;
#86932=CARTESIAN_POINT('Ctrl Pts',(-19.2022616264228,33.5152752885903,124.92803419319)) ;
#86933=CARTESIAN_POINT('Ctrl Pts',(-18.7005637331334,33.5350837278112,124.768198422526)) ;
#86934=CARTESIAN_POINT('Ctrl Pts',(-18.2796383911774,33.5550694371914,124.44444941678)) ;
#86935=CARTESIAN_POINT('Ctrl Pts',(-17.9957682334727,33.5749389602067,123.998878153294)) ;
#86936=CARTESIAN_POINT('Ctrl Pts',(-17.8804168309484,33.5949596993239,123.479617978128)) ;
#86937=CARTESIAN_POINT('Ctrl Pts',(-17.9478193704265,33.6147637643009,122.957391827928)) ;
#86938=CARTESIAN_POINT('Ctrl Pts',(-18.1922075876265,33.6348257280316,122.483648094758)) ;
#86939=CARTESIAN_POINT('Ctrl Pts',(-18.5796761414085,33.6546589083201,122.126063706925)) ;
#86940=CARTESIAN_POINT('Ctrl Pts',(-19.0672471785734,33.6745781056462,121.919993572332)) ;
#86941=CARTESIAN_POINT('Ctrl Pts',(-19.5964794361335,33.6945161307595,121.892984850209)) ;
#86942=CARTESIAN_POINT('Ctrl Pts',(-20.1019033803434,33.7143941768156,122.047027331049)) ;
#86943=CARTESIAN_POINT('Ctrl Pts',(-20.5266212368,33.7343789111036,122.365892503823)) ;
#86944=CARTESIAN_POINT('Ctrl Pts',(-20.8161596894946,33.7542897277821,122.809038474966)) ;
#86945=CARTESIAN_POINT('Ctrl Pts',(-20.9372320691971,33.7742887033008,123.326476372936)) ;
#86946=CARTESIAN_POINT('Ctrl Pts',(-20.8757063920879,33.794093623946,123.849357303765)) ;
#86947=CARTESIAN_POINT('Ctrl Pts',(-20.6381117871144,33.8140775842373,124.324253054695)) ;
#86948=CARTESIAN_POINT('Ctrl Pts',(-20.2542831223755,33.8339637879612,124.68776744017)) ;
#86949=CARTESIAN_POINT('Ctrl Pts',(-19.7682875774795,33.8539129662844,124.899638859617)) ;
#86950=CARTESIAN_POINT('Ctrl Pts',(-19.2403826918121,33.8738147655239,124.932749323291)) ;
#86951=CARTESIAN_POINT('Ctrl Pts',(-18.7331049966278,33.8936933705763,124.784958195481)) ;
#86952=CARTESIAN_POINT('Ctrl Pts',(-18.3035554846274,33.913725730302,124.470321163056)) ;
#86953=CARTESIAN_POINT('Ctrl Pts',(-18.0587986989934,33.9303074562581,124.103799046386)) ;
#86954=CARTESIAN_POINT('Ctrl Pts',(-17.9464440989299,33.943501626556,123.775801865132)) ;
#86955=CARTESIAN_POINT('Ctrl Pts',(-17.891701854277,33.9568138046492,123.430280794334)) ;
#86956=CARTESIAN_POINT('Ctrl Pts',(-17.937495113229,33.9733799842425,122.992341681738)) ;
#86957=CARTESIAN_POINT('Ctrl Pts',(-18.1302774467429,33.9900081791027,122.594720028889)) ;
#86958=CARTESIAN_POINT('Ctrl Pts',(-18.3588197435753,34.0032967608125,122.330608010279)) ;
#86959=CARTESIAN_POINT('Ctrl Pts',(-18.5618595656554,34.0132650089161,122.165129183368)) ;
#86960=CARTESIAN_POINT('Ctrl Pts',(-18.7891847096601,34.0231797651722,122.037806845521)) ;
#86961=CARTESIAN_POINT('Ctrl Pts',(-19.0375192291355,34.0331929158234,121.950759748817)) ;
#86962=CARTESIAN_POINT('Ctrl Pts',(-19.2972286630396,34.0432056230254,121.908570343025)) ;
#86963=CARTESIAN_POINT('Ctrl Pts',(-19.6446460039,34.0564249117167,121.912596021897)) ;
#86964=CARTESIAN_POINT('Ctrl Pts',(-20.0699254705713,34.0730435927147,122.03142792988)) ;
#86965=CARTESIAN_POINT('Ctrl Pts',(-20.4284671618756,34.0896085004882,122.287092857787)) ;
#86966=CARTESIAN_POINT('Ctrl Pts',(-20.6522378081821,34.103006972099,122.558923682417)) ;
#86967=CARTESIAN_POINT('Ctrl Pts',(-20.779673548747,34.112848227586,122.78398886291)) ;
#86968=CARTESIAN_POINT('Ctrl Pts',(-20.8678897526762,34.1228345431742,123.031102300472)) ;
#86969=CARTESIAN_POINT('Ctrl Pts',(-20.9117788511624,34.1327711507606,123.288555336312)) ;
#86970=CARTESIAN_POINT('Ctrl Pts',(-20.9101514532125,34.1428210181289,123.552623293535)) ;
#86971=CARTESIAN_POINT('Ctrl Pts',(-20.863821952132,34.1526715128037,123.807324091934)) ;
#86972=CARTESIAN_POINT('Ctrl Pts',(-20.7735256213535,34.1626433131982,124.053287870522)) ;
#86973=CARTESIAN_POINT('Ctrl Pts',(-20.6415098394546,34.172639280224,124.280439245738)) ;
#86974=CARTESIAN_POINT('Ctrl Pts',(-20.4711254085416,34.1826767396052,124.481765931649)) ;
#86975=CARTESIAN_POINT('Ctrl Pts',(-20.2726263760509,34.1925174405059,124.647547741897)) ;
#86976=CARTESIAN_POINT('Ctrl Pts',(-20.0438538007464,34.2025654617733,124.779381747442)) ;
#86977=CARTESIAN_POINT('Ctrl Pts',(-19.7979948387222,34.212512854856,124.868199817644)) ;
#86978=CARTESIAN_POINT('Ctrl Pts',(-19.5415398597008,34.2224230009024,124.913598266864)) ;
#86979=CARTESIAN_POINT('Ctrl Pts',(-19.2772295562355,34.232481914752,124.913481740672)) ;
#86980=CARTESIAN_POINT('Ctrl Pts',(-19.0224749494035,34.2423226850413,124.868818922004)) ;
#86981=CARTESIAN_POINT('Ctrl Pts',(-18.7738170634932,34.2523855546199,124.778924498811)) ;
#86982=CARTESIAN_POINT('Ctrl Pts',(-18.5484380725391,34.2622798777504,124.649212333765)) ;
#86983=CARTESIAN_POINT('Ctrl Pts',(-18.3476405758638,34.2722216848449,124.482118201079)) ;
#86984=CARTESIAN_POINT('Ctrl Pts',(-18.1777564580938,34.2822241958002,124.281491322928)) ;
#86985=CARTESIAN_POINT('Ctrl Pts',(-18.0452449011872,34.2922589166186,124.053519923631)) ;
#86986=CARTESIAN_POINT('Ctrl Pts',(-17.9556349074693,34.3021040941243,123.810796881849)) ;
#86987=CARTESIAN_POINT('Ctrl Pts',(-17.9083784162444,34.3120888545254,123.552736052031)) ;
#86988=CARTESIAN_POINT('Ctrl Pts',(-17.9065296697451,34.3220277608418,123.291519123483)) ;
#86989=CARTESIAN_POINT('Ctrl Pts',(-17.9505964036269,34.3320699884775,123.031352463089)) ;
#86990=CARTESIAN_POINT('Ctrl Pts',(-18.037624931531,34.3419552000619,122.786560063066)) ;
#86991=CARTESIAN_POINT('Ctrl Pts',(-18.1669823934787,34.3519541302638,122.557890019545)) ;
#86992=CARTESIAN_POINT('Ctrl Pts',(-18.3326161325234,34.3618715531743,122.356617211244)) ;
#86993=CARTESIAN_POINT('Ctrl Pts',(-18.5332582552476,34.371919485253,122.185024436481)) ;
#86994=CARTESIAN_POINT('Ctrl Pts',(-18.7567288565943,34.3817968610624,122.052891702144)) ;
#86995=CARTESIAN_POINT('Ctrl Pts',(-19.0039582074564,34.3918507542303,121.959841830907)) ;
#86996=CARTESIAN_POINT('Ctrl Pts',(-19.2595239194454,34.4017443774836,121.911772148145)) ;
#86997=CARTESIAN_POINT('Ctrl Pts',(-19.5238983005659,34.4118069711066,121.908716657906)) ;
#86998=CARTESIAN_POINT('Ctrl Pts',(-19.7791766052678,34.4216495450957,121.950552116811)) ;
#86999=CARTESIAN_POINT('Ctrl Pts',(-20.0271336820024,34.4316403019786,122.036751836133)) ;
#87000=CARTESIAN_POINT('Ctrl Pts',(-20.254936747224,34.4415683637365,122.163955290834)) ;
#87001=CARTESIAN_POINT('Ctrl Pts',(-20.4586999823896,34.4515563396257,122.329419432095)) ;
#87002=CARTESIAN_POINT('Ctrl Pts',(-20.6311135230344,34.4615920039821,122.528971921844)) ;
#87003=CARTESIAN_POINT('Ctrl Pts',(-20.7641991432005,34.4714479424018,122.751184316972)) ;
#87004=CARTESIAN_POINT('Ctrl Pts',(-20.8583766148853,34.4814434337987,122.996362053338)) ;
#87005=CARTESIAN_POINT('Ctrl Pts',(-20.9082075537525,34.4913532387521,123.251982490847)) ;
#87006=CARTESIAN_POINT('Ctrl Pts',(-20.9133731041675,34.5013654610189,123.515048494353)) ;
#87007=CARTESIAN_POINT('Ctrl Pts',(-20.8722117287927,34.5113933417117,123.775338285339)) ;
#87008=CARTESIAN_POINT('Ctrl Pts',(-20.7883656546394,34.5212497376943,124.020406248148)) ;
#87009=CARTESIAN_POINT('Ctrl Pts',(-20.6615835386418,34.5312745348743,124.251337874107)) ;
#87010=CARTESIAN_POINT('Ctrl Pts',(-20.4960213753757,34.5413054648581,124.456471359235)) ;
#87011=CARTESIAN_POINT('Ctrl Pts',(-20.3013678063014,34.5511500673668,124.626861391942)) ;
#87012=CARTESIAN_POINT('Ctrl Pts',(-20.0771540029309,34.5611409185909,124.763475181664)) ;
#87013=CARTESIAN_POINT('Ctrl Pts',(-19.8312684979688,34.5711787516021,124.858978848205)) ;
#87014=CARTESIAN_POINT('Ctrl Pts',(-19.577597721108,34.5810231400675,124.909794407279)) ;
#87015=CARTESIAN_POINT('Ctrl Pts',(-19.3153254135936,34.5910079444371,124.916395570921)) ;
#87016=CARTESIAN_POINT('Ctrl Pts',(-19.0569804860377,34.6009474639199,124.87763585839)) ;
#87017=CARTESIAN_POINT('Ctrl Pts',(-18.806866607614,34.6109871949213,124.793729916711)) ;
#87018=CARTESIAN_POINT('Ctrl Pts',(-18.5785256075441,34.6208753231676,124.669671687923)) ;
#87019=CARTESIAN_POINT('Ctrl Pts',(-18.3728209709373,34.6308650483761,124.506586268412)) ;
#87020=CARTESIAN_POINT('Ctrl Pts',(-18.1992525056931,34.6408228130776,124.31075898755)) ;
#87021=CARTESIAN_POINT('Ctrl Pts',(-18.0625580666762,34.6507251544896,124.089319343284)) ;
#87022=CARTESIAN_POINT('Ctrl Pts',(-17.9650433992383,34.660769350196,123.844056094203)) ;
#87023=CARTESIAN_POINT('Ctrl Pts',(-17.9122901221407,34.6706767509553,123.589085907757)) ;
#87024=CARTESIAN_POINT('Ctrl Pts',(-17.9040671219944,34.6806873508296,123.326142620746)) ;
#87025=CARTESIAN_POINT('Ctrl Pts',(-17.942203265216,34.6907176467418,123.065322697016)) ;
#87026=CARTESIAN_POINT('Ctrl Pts',(-18.0232493114111,34.7005724263915,122.819373677744)) ;
#87027=CARTESIAN_POINT('Ctrl Pts',(-18.1463519672124,34.710529754609,122.588461269854)) ;
#87028=CARTESIAN_POINT('Ctrl Pts',(-18.309353042108,34.7205687875159,122.381049743484)) ;
#87029=CARTESIAN_POINT('Ctrl Pts',(-18.5023659383517,34.7304418994052,122.207599723295)) ;
#87030=CARTESIAN_POINT('Ctrl Pts',(-18.7269874138073,34.7405151844323,122.06763353317)) ;
#87031=CARTESIAN_POINT('Ctrl Pts',(-18.966311174259,34.7503355041691,121.970921603636)) ;
#87032=CARTESIAN_POINT('Ctrl Pts',(-19.2252615250139,34.7604141695475,121.915607928114)) ;
#87033=CARTESIAN_POINT('Ctrl Pts',(-19.4840428530472,34.7702657600313,121.906215757302)) ;
#87034=CARTESIAN_POINT('Ctrl Pts',(-19.7462130095486,34.7803389103502,121.942457891797)) ;
#87035=CARTESIAN_POINT('Ctrl Pts',(-19.9923964312408,34.7901812903253,122.021867293698)) ;
#87036=CARTESIAN_POINT('Ctrl Pts',(-20.224633402004,34.8001622665683,122.143734711503)) ;
#87037=CARTESIAN_POINT('Ctrl Pts',(-20.4326722972678,34.8101785949236,122.305014175264)) ;
#87038=CARTESIAN_POINT('Ctrl Pts',(-20.6076836467507,34.8200763919147,122.497420427446)) ;
#87039=CARTESIAN_POINT('Ctrl Pts',(-20.7486352078836,34.8300889486468,122.719624524635)) ;
#87040=CARTESIAN_POINT('Ctrl Pts',(-20.8484693509522,34.8401209834933,122.963608083388)) ;
#87041=CARTESIAN_POINT('Ctrl Pts',(-20.9039852822509,34.8499603843087,123.216169118791)) ;
#87042=CARTESIAN_POINT('Ctrl Pts',(-20.915252015336,34.8600261699603,123.480416453755)) ;
#87043=CARTESIAN_POINT('Ctrl Pts',(-20.8809428954112,34.8699166250749,123.738080890662)) ;
#87044=CARTESIAN_POINT('Ctrl Pts',(-20.8021590268459,34.8799087437107,123.988551842107)) ;
#87045=CARTESIAN_POINT('Ctrl Pts',(-20.6812162451853,34.8898715704737,124.220748500845)) ;
#87046=CARTESIAN_POINT('Ctrl Pts',(-20.5232363311893,34.8997758537466,124.427621791333)) ;
#87047=CARTESIAN_POINT('Ctrl Pts',(-20.328602748606,34.9098362876937,124.606497029424)) ;
#87048=CARTESIAN_POINT('Ctrl Pts',(-20.1108581510111,34.9196768403669,124.746063981003)) ;
#87049=CARTESIAN_POINT('Ctrl Pts',(-19.8670007279919,34.9297390603126,124.848234310547)) ;
#87050=CARTESIAN_POINT('Ctrl Pts',(-19.6132374871759,34.9396361995912,124.9052994767)) ;
#87051=CARTESIAN_POINT('Ctrl Pts',(-19.352586866818,34.9495673917262,124.918345206172)) ;
#87052=CARTESIAN_POINT('Ctrl Pts',(-19.0907761598874,34.9596095463713,124.885281266899)) ;
#87053=CARTESIAN_POINT('Ctrl Pts',(-18.8424935087745,34.9694963073906,124.808663455936)) ;
#87054=CARTESIAN_POINT('Ctrl Pts',(-18.6085514013706,34.9794956091078,124.689074670539)) ;
#87055=CARTESIAN_POINT('Ctrl Pts',(-18.4004100503073,34.9894164072746,124.532024155764)) ;
#87056=CARTESIAN_POINT('Ctrl Pts',(-18.220695374879,34.9994504608713,124.339108184459)) ;
#87057=CARTESIAN_POINT('Ctrl Pts',(-18.0786234259347,35.0093735784377,124.120391230864)) ;
#87058=CARTESIAN_POINT('Ctrl Pts',(-17.9753990929057,35.0194297019368,123.877150159267)) ;
#87059=CARTESIAN_POINT('Ctrl Pts',(-17.917104068257,35.0292751435917,123.62506345845)) ;
#87060=CARTESIAN_POINT('Ctrl Pts',(-17.9024452588224,35.0392374447158,123.36369174523)) ;
#87061=CARTESIAN_POINT('Ctrl Pts',(-17.933946461117,35.0492659239909,123.102025569632)) ;
#87062=CARTESIAN_POINT('Ctrl Pts',(-18.0094085575674,35.0591762775006,122.852777323591)) ;
#87063=CARTESIAN_POINT('Ctrl Pts',(-18.1266927602278,35.0691111496778,122.619516835167)) ;
#87064=CARTESIAN_POINT('Ctrl Pts',(-18.2845521812503,35.0791522872635,122.408084929037)) ;
#87065=CARTESIAN_POINT('Ctrl Pts',(-18.4736704054688,35.0890394364781,122.22989810543)) ;
#87066=CARTESIAN_POINT('Ctrl Pts',(-18.6928945527343,35.0990316712291,122.085390254205)) ;
#87067=CARTESIAN_POINT('Ctrl Pts',(-18.932889746988,35.1089803767921,121.9816540539)) ;
#87068=CARTESIAN_POINT('Ctrl Pts',(-19.1868087710443,35.1189164452158,121.92087877605)) ;
#87069=CARTESIAN_POINT('Ctrl Pts',(-19.4487510389459,35.1289021294316,121.904734357307)) ;
#87070=CARTESIAN_POINT('Ctrl Pts',(-19.7108597155161,35.1389425560002,121.934890399688)) ;
#87071=CARTESIAN_POINT('Ctrl Pts',(-19.9588218803458,35.148781669464,122.008182230702)) ;
#87072=CARTESIAN_POINT('Ctrl Pts',(-20.195037968623,35.1588114036398,122.125114451366)) ;
#87073=CARTESIAN_POINT('Ctrl Pts',(-20.4067898564085,35.1688335031457,122.281715086655)) ;
#87074=CARTESIAN_POINT('Ctrl Pts',(-20.5858406931206,35.1787019430391,122.46934344386)) ;
#87075=CARTESIAN_POINT('Ctrl Pts',(-20.7324825930465,35.1887708077248,122.689561854867)) ;
#87076=CARTESIAN_POINT('Ctrl Pts',(-20.8362960938539,35.1986134808234,122.926479912635)) ;
#87077=CARTESIAN_POINT('Ctrl Pts',(-20.899055079425,35.2085741149858,123.180594616481)) ;
#87078=CARTESIAN_POINT('Ctrl Pts',(-20.9163568869125,35.2186120306639,123.44380305098)) ;
#87079=CARTESIAN_POINT('Ctrl Pts',(-20.8886337721967,35.2284863055234,123.701836099716)) ;
#87080=CARTESIAN_POINT('Ctrl Pts',(-20.815106074293,35.2385560558985,123.956001024207)) ;
#87081=CARTESIAN_POINT('Ctrl Pts',(-20.701400325098,35.248389351273,124.188072701268)) ;
#87082=CARTESIAN_POINT('Ctrl Pts',(-20.5466987675831,35.2584196487526,124.401475805769)) ;
#87083=CARTESIAN_POINT('Ctrl Pts',(-20.3567063540923,35.2684517351941,124.584263100217)) ;
#87084=CARTESIAN_POINT('Ctrl Pts',(-20.1426513521819,35.278279663683,124.72875221101)) ;
#87085=CARTESIAN_POINT('Ctrl Pts',(-19.9030046171071,35.2882757047938,124.836324512499)) ;
#87086=CARTESIAN_POINT('Ctrl Pts',(-19.6474276615906,35.298301516895,124.900352262788)) ;
#87087=CARTESIAN_POINT('Ctrl Pts',(-19.3882751938659,35.3081887517898,124.919108279541)) ;
#87088=CARTESIAN_POINT('Ctrl Pts',(-19.1274391236298,35.3181656180008,124.892776277121)) ;
#87089=CARTESIAN_POINT('Ctrl Pts',(-18.8746646646945,35.3281585618726,124.821468377364)) ;
#87090=CARTESIAN_POINT('Ctrl Pts',(-18.6372430900327,35.338196484544,124.706562893995)) ;
#87091=CARTESIAN_POINT('Ctrl Pts',(-18.4271550056594,35.3480449488057,124.555385469111)) ;
#87092=CARTESIAN_POINT('Ctrl Pts',(-18.2435829818069,35.3580368155497,124.367696236912)) ;
#87093=CARTESIAN_POINT('Ctrl Pts',(-18.0963252747795,35.3679545475909,124.152615497661)) ;
#87094=CARTESIAN_POINT('Ctrl Pts',(-17.9874096726993,35.3779827324862,123.912669454081)) ;
#87095=CARTESIAN_POINT('Ctrl Pts',(-17.9226347534564,35.387867890535,123.66109622289)) ;
#87096=CARTESIAN_POINT('Ctrl Pts',(-17.9016765666423,35.3978572510767,123.39941901094)) ;
#87097=CARTESIAN_POINT('Ctrl Pts',(-17.9271558083283,35.4078984080111,123.136781335397)) ;
#87098=CARTESIAN_POINT('Ctrl Pts',(-17.9959687525466,35.4177309914662,122.88772650032)) ;
#87099=CARTESIAN_POINT('Ctrl Pts',(-18.1081319471754,35.4277252114282,122.650247800051)) ;
#87100=CARTESIAN_POINT('Ctrl Pts',(-18.2607849253877,35.4377533132155,122.435427774985)) ;
#87101=CARTESIAN_POINT('Ctrl Pts',(-18.4453853520115,35.4476332578386,122.252848690864)) ;
#87102=CARTESIAN_POINT('Ctrl Pts',(-18.6610214269731,35.4576235843956,122.103123520847)) ;
#87103=CARTESIAN_POINT('Ctrl Pts',(-18.8982196683709,35.4675645160499,121.993647605999)) ;
#87104=CARTESIAN_POINT('Ctrl Pts',(-19.1519136468404,35.4775516345528,121.926344805637)) ;
#87105=CARTESIAN_POINT('Ctrl Pts',(-19.4146479680384,35.48758496745,121.904428438846)) ;
#87106=CARTESIAN_POINT('Ctrl Pts',(-19.6729148068661,35.4974510718947,121.927562236653)) ;
#87107=CARTESIAN_POINT('Ctrl Pts',(-19.9282737618614,35.5075171857751,121.996483449793)) ;
#87108=CARTESIAN_POINT('Ctrl Pts',(-20.1628377208178,35.5173731975435,122.106361679407)) ;
#87109=CARTESIAN_POINT('Ctrl Pts',(-20.3781660934209,35.5273679011748,122.256744946492)) ;
#87110=CARTESIAN_POINT('Ctrl Pts',(-20.5644031071723,35.5373992368997,122.443319308297)) ;
#87111=CARTESIAN_POINT('Ctrl Pts',(-20.7132753997824,35.5472657621033,122.655613795221)) ;
#87112=CARTESIAN_POINT('Ctrl Pts',(-20.824735991116,35.5572531901491,122.893195278124)) ;
#87113=CARTESIAN_POINT('Ctrl Pts',(-20.8931143715501,35.5671981198355,123.145473611636)) ;
#87114=CARTESIAN_POINT('Ctrl Pts',(-20.916731989703,35.5772430379441,123.408359549251)) ;
#87115=CARTESIAN_POINT('Ctrl Pts',(-20.8949804435051,35.587105007558,123.66662867698)) ;
#87116=CARTESIAN_POINT('Ctrl Pts',(-20.8283478671713,35.5970970755792,123.920587710675)) ;
#87117=CARTESIAN_POINT('Ctrl Pts',(-20.719243324381,35.6070280009538,124.157679141684)) ;
#87118=CARTESIAN_POINT('Ctrl Pts',(-20.5707147508326,35.6169786291772,124.372871095378)) ;
#87119=CARTESIAN_POINT('Ctrl Pts',(-20.3862369565019,35.6269788682363,124.560073078809)) ;
#87120=CARTESIAN_POINT('Ctrl Pts',(-20.1712640574126,35.6370073236055,124.712497104667)) ;
#87121=CARTESIAN_POINT('Ctrl Pts',(-19.9370958263856,35.6468733581888,124.823815964018)) ;
#87122=CARTESIAN_POINT('Ctrl Pts',(-19.6841078343026,35.6568656799362,124.894073754451)) ;
#87123=CARTESIAN_POINT('Ctrl Pts',(-19.4242931282444,35.6667979696132,124.919232541197)) ;
#87124=CARTESIAN_POINT('Ctrl Pts',(-19.1622457507477,35.676799614584,124.89901214049)) ;
#87125=CARTESIAN_POINT('Ctrl Pts',(-18.8234350299955,35.690112248,124.811793581749)) ;
#87126=CARTESIAN_POINT('Ctrl Pts',(-18.5168964604078,35.7033439973816,124.639445590766)) ;
#87127=CARTESIAN_POINT('Ctrl Pts',(-18.2664225908945,35.7166672621986,124.394805388771)) ;
#87128=CARTESIAN_POINT('Ctrl Pts',(-18.1147450135693,35.7265429684163,124.184207203932)) ;
#87129=CARTESIAN_POINT('Ctrl Pts',(-18.0003454842561,35.7365325595163,123.947960343234)) ;
#87130=CARTESIAN_POINT('Ctrl Pts',(-17.9289701667244,35.7464596559717,123.697008534527)) ;
#87131=CARTESIAN_POINT('Ctrl Pts',(-17.9019627690378,35.7564848044763,123.434969684401)) ;
#87132=CARTESIAN_POINT('Ctrl Pts',(-17.9204625057985,35.766380458623,123.175558526549)) ;
#87133=CARTESIAN_POINT('Ctrl Pts',(-17.9840399510721,35.7763839930012,122.920505986074)) ;
#87134=CARTESIAN_POINT('Ctrl Pts',(-18.0907912526402,35.7863691314413,122.680759611974)) ;
#87135=CARTESIAN_POINT('Ctrl Pts',(-18.2384845563749,35.7964050560366,122.462276828214)) ;
#87136=CARTESIAN_POINT('Ctrl Pts',(-18.4182832581623,35.8062563314643,122.276022071899)) ;
#87137=CARTESIAN_POINT('Ctrl Pts',(-18.6302545916797,35.8162485926257,122.121024656498)) ;
#87138=CARTESIAN_POINT('Ctrl Pts',(-18.8673155093982,35.8262884766433,122.005244450248)) ;
#87139=CARTESIAN_POINT('Ctrl Pts',(-19.1155599860478,35.8361232511457,121.93323039927)) ;
#87140=CARTESIAN_POINT('Ctrl Pts',(-19.3787662820051,35.846199632166,121.90464170685)) ;
#87141=CARTESIAN_POINT('Ctrl Pts',(-19.6369856027935,35.8560459053166,121.921721200336)) ;
#87142=CARTESIAN_POINT('Ctrl Pts',(-19.9782318745606,35.8694104266019,122.004755386422)) ;
#87143=CARTESIAN_POINT('Ctrl Pts',(-20.2860781894191,35.8826166710363,122.173358222392)) ;
#87144=CARTESIAN_POINT('Ctrl Pts',(-20.5388194305417,35.8958816257135,122.413415383819)) ;
#87145=CARTESIAN_POINT('Ctrl Pts',(-20.6954518663001,35.9059139062652,122.625487616004)) ;
#87146=CARTESIAN_POINT('Ctrl Pts',(-20.8114494728934,35.9158226397831,122.858608403369)) ;
#87147=CARTESIAN_POINT('Ctrl Pts',(-20.8860782708486,35.9257601906506,123.108875396054)) ;
#87148=CARTESIAN_POINT('Ctrl Pts',(-20.9161752733181,35.9357900382445,123.370700554843)) ;
#87149=CARTESIAN_POINT('Ctrl Pts',(-20.8957731929268,35.949025178165,123.717991080168)) ;
#87150=CARTESIAN_POINT('Ctrl Pts',(-20.7562782646861,35.9656936425361,124.138331425498)) ;
#87151=CARTESIAN_POINT('Ctrl Pts',(-20.4290918169683,35.98556465441,124.553143935095)) ;
#87152=CARTESIAN_POINT('Ctrl Pts',(-20.0516669376428,36.002271738793,124.786848654509)) ;
#87153=CARTESIAN_POINT('Ctrl Pts',(-19.7200488034031,36.0154490201036,124.886772678737)) ;
#87154=CARTESIAN_POINT('Ctrl Pts',(-19.3739896601812,36.0287164806177,124.929104605177)) ;
#87155=CARTESIAN_POINT('Ctrl Pts',(-18.9367256618785,36.0453303713049,124.867571649377)) ;
#87156=CARTESIAN_POINT('Ctrl Pts',(-18.4683585867537,36.0652791707323,124.618963683723)) ;
#87157=CARTESIAN_POINT('Ctrl Pts',(-18.1135879764182,36.0852002822632,124.2260271695)) ;
#87158=CARTESIAN_POINT('Ctrl Pts',(-17.9136719684102,36.1050667304361,123.737230065052)) ;
#87159=CARTESIAN_POINT('Ctrl Pts',(-17.8927126209991,36.1250930770532,123.205433374261)) ;
#87160=CARTESIAN_POINT('Ctrl Pts',(-18.0533007215964,36.1449551214427,122.702455916173)) ;
#87161=CARTESIAN_POINT('Ctrl Pts',(-18.3764776353452,36.1649004241238,122.282339628229)) ;
#87162=CARTESIAN_POINT('Ctrl Pts',(-18.8226158877263,36.1847957311827,121.998462474444)) ;
#87163=CARTESIAN_POINT('Ctrl Pts',(-19.3385842783177,36.2046890013503,121.882951679264)) ;
#87164=CARTESIAN_POINT('Ctrl Pts',(-19.8648495105545,36.2246545940308,121.950798037064)) ;
#87165=CARTESIAN_POINT('Ctrl Pts',(-20.334465653922,36.2445299177156,122.192756268591)) ;
#87166=CARTESIAN_POINT('Ctrl Pts',(-20.6955169132806,36.2645049802905,122.582020760569)) ;
#87167=CARTESIAN_POINT('Ctrl Pts',(-20.9010738348726,36.2844573899217,123.070861900805)) ;
#87168=CARTESIAN_POINT('Ctrl Pts',(-20.9283436001929,36.3042934441578,123.597363126459)) ;
#87169=CARTESIAN_POINT('Ctrl Pts',(-20.7737705212242,36.3242713555753,124.10534582472)) ;
#87170=CARTESIAN_POINT('Ctrl Pts',(-20.4556033727974,36.3441894050788,124.528410951894)) ;
#87171=CARTESIAN_POINT('Ctrl Pts',(-20.0139153720363,36.3640575488469,124.818025234808)) ;
#87172=CARTESIAN_POINT('Ctrl Pts',(-19.4952301669597,36.3841084054342,124.939796977761)) ;
#87173=CARTESIAN_POINT('Ctrl Pts',(-18.9729215440468,36.4038888418901,124.878628473693)) ;
#87174=CARTESIAN_POINT('Ctrl Pts',(-18.4967651240595,36.4239188975679,124.640802577976)) ;
#87175=CARTESIAN_POINT('Ctrl Pts',(-18.1335848516454,36.4438000027427,124.25686352696)) ;
#87176=CARTESIAN_POINT('Ctrl Pts',(-17.9219195474901,36.4636804651105,123.77277946085)) ;
#87177=CARTESIAN_POINT('Ctrl Pts',(-17.8881151233781,36.4836656122549,123.242666380459)) ;
#87178=CARTESIAN_POINT('Ctrl Pts',(-18.0366553794252,36.5035561907912,122.73529278596)) ;
#87179=CARTESIAN_POINT('Ctrl Pts',(-18.3487072158258,36.5234502106656,122.308453160384)) ;
#87180=CARTESIAN_POINT('Ctrl Pts',(-18.7881486981132,36.543371655392,122.013243316393)) ;
#87181=CARTESIAN_POINT('Ctrl Pts',(-19.3013483876729,36.5632697934474,121.884892286894)) ;
#87182=CARTESIAN_POINT('Ctrl Pts',(-19.8317595038524,36.5833405486635,121.940839429391)) ;
#87183=CARTESIAN_POINT('Ctrl Pts',(-20.3047244450388,36.6031260987147,122.170976388332)) ;
#87184=CARTESIAN_POINT('Ctrl Pts',(-20.6751961018729,36.6231091735921,122.551414789717)) ;
#87185=CARTESIAN_POINT('Ctrl Pts',(-20.8920876251874,36.643018256238,123.034079238211)) ;
#87186=CARTESIAN_POINT('Ctrl Pts',(-20.9326736949197,36.6628768153608,123.560393777446)) ;
#87187=CARTESIAN_POINT('Ctrl Pts',(-20.7893507745121,36.6829202591995,124.073361851782)) ;
#87188=CARTESIAN_POINT('Ctrl Pts',(-20.5344135959182,36.6994203239287,124.430349947457)) ;
#87189=CARTESIAN_POINT('Ctrl Pts',(-20.2630412458369,36.7128100637776,124.654248532504)) ;
#87190=CARTESIAN_POINT('Ctrl Pts',(-20.0376657911243,36.722666964986,124.781998493706)) ;
#87191=CARTESIAN_POINT('Ctrl Pts',(-19.790451891043,36.7326584908325,124.870339079412)) ;
#87192=CARTESIAN_POINT('Ctrl Pts',(-19.5333205208731,36.7425831712835,124.914226210988)) ;
#87193=CARTESIAN_POINT('Ctrl Pts',(-19.2702961550599,36.7525937613279,124.912889798325)) ;
#87194=CARTESIAN_POINT('Ctrl Pts',(-18.9272992756477,36.7658530220315,124.851022900053)) ;
#87195=CARTESIAN_POINT('Ctrl Pts',(-18.6064416437255,36.7792040971818,124.699737523157)) ;
#87196=CARTESIAN_POINT('Ctrl Pts',(-18.3413179144251,36.7924104064166,124.475682143339)) ;
#87197=CARTESIAN_POINT('Ctrl Pts',(-18.1729500479038,36.8023972400069,124.274423037726)) ;
#87198=CARTESIAN_POINT('Ctrl Pts',(-18.0423739740692,36.812349967503,124.047750299169)) ;
#87199=CARTESIAN_POINT('Ctrl Pts',(-17.952518013425,36.8223980643446,123.799486638763)) ;
#87200=CARTESIAN_POINT('Ctrl Pts',(-17.907757267272,36.8322395212164,123.544740945739)) ;
#87201=CARTESIAN_POINT('Ctrl Pts',(-17.9073502062391,36.8422257881299,123.282355578864)) ;
#87202=CARTESIAN_POINT('Ctrl Pts',(-17.9521694205823,36.8521623890303,123.025063136411)) ;
#87203=CARTESIAN_POINT('Ctrl Pts',(-18.0420963058471,36.8622123318174,122.776771029239)) ;
#87204=CARTESIAN_POINT('Ctrl Pts',(-18.1710052785227,36.8720625315031,122.552279193621)) ;
#87205=CARTESIAN_POINT('Ctrl Pts',(-18.3384408575299,36.8820354364352,122.350698607091)) ;
#87206=CARTESIAN_POINT('Ctrl Pts',(-18.5389463808558,36.8920338109148,122.18084427361)) ;
#87207=CARTESIAN_POINT('Ctrl Pts',(-18.7664541058527,36.9020539847848,122.048279786072)) ;
#87208=CARTESIAN_POINT('Ctrl Pts',(-19.0105222002321,36.9119550287268,121.95809778858)) ;
#87209=CARTESIAN_POINT('Ctrl Pts',(-19.268728383313,36.9219438324511,121.910847088745)) ;
#87210=CARTESIAN_POINT('Ctrl Pts',(-19.5305939085291,36.9319092992829,121.909337770446)) ;
#87211=CARTESIAN_POINT('Ctrl Pts',(-19.7872824216961,36.9418128615559,121.95243202349)) ;
#87212=CARTESIAN_POINT('Ctrl Pts',(-20.0363517848326,36.9518735394339,122.041006819332)) ;
#87213=CARTESIAN_POINT('Ctrl Pts',(-20.2614482794892,36.9617138373834,122.1683698474)) ;
#87214=CARTESIAN_POINT('Ctrl Pts',(-20.4656746860891,36.9717768322928,122.336311677907)) ;
#87215=CARTESIAN_POINT('Ctrl Pts',(-20.6346325844978,36.9816711264399,122.533982970242)) ;
#87216=CARTESIAN_POINT('Ctrl Pts',(-20.7679155889213,36.9916129241368,122.758650934849)) ;
#87217=CARTESIAN_POINT('Ctrl Pts',(-20.8608421966797,37.0016155016659,123.004571300072)) ;
#87218=CARTESIAN_POINT('Ctrl Pts',(-20.9094048501918,37.011649965587,123.26374268831)) ;
#87219=CARTESIAN_POINT('Ctrl Pts',(-20.9125815920894,37.0214961041081,123.522477689503)) ;
#87220=CARTESIAN_POINT('Ctrl Pts',(-20.8707936127288,37.0314772773451,123.781401079755)) ;
#87221=CARTESIAN_POINT('Ctrl Pts',(-20.7848638119868,37.0414295713023,124.028425816195)) ;
#87222=CARTESIAN_POINT('Ctrl Pts',(-20.6570438981956,37.0514283664369,124.258022088148)) ;
#87223=CARTESIAN_POINT('Ctrl Pts',(-20.4902612991329,37.0614674746977,124.462411340172)) ;
#87224=CARTESIAN_POINT('Ctrl Pts',(-20.2951235539568,37.0712924161369,124.631500866346)) ;
#87225=CARTESIAN_POINT('Ctrl Pts',(-20.0686616200432,37.0813471032113,124.767597084672)) ;
#87226=CARTESIAN_POINT('Ctrl Pts',(-19.8245710827869,37.0912899081514,124.860842297865)) ;
#87227=CARTESIAN_POINT('Ctrl Pts',(-19.5691588004271,37.1011936941479,124.910878499083)) ;
#87228=CARTESIAN_POINT('Ctrl Pts',(-19.3052063233042,37.1112405107127,124.915717087351)) ;
#87229=CARTESIAN_POINT('Ctrl Pts',(-19.0482495106725,37.1211360301914,124.875491392646)) ;
#87230=CARTESIAN_POINT('Ctrl Pts',(-18.7981148297119,37.1311981155158,124.789869782215)) ;
#87231=CARTESIAN_POINT('Ctrl Pts',(-18.5715632075335,37.1410408264737,124.664999559399)) ;
#87232=CARTESIAN_POINT('Ctrl Pts',(-18.3667645398744,37.1510315437798,124.500772902301)) ;
#87233=CARTESIAN_POINT('Ctrl Pts',(-18.1946815226206,37.1609596268764,124.304654257152)) ;
#87234=CARTESIAN_POINT('Ctrl Pts',(-18.0580587042926,37.1709475569881,124.080530224495)) ;
#87235=CARTESIAN_POINT('Ctrl Pts',(-17.9623882859192,37.1809833831154,123.834772735687)) ;
#87236=CARTESIAN_POINT('Ctrl Pts',(-17.9113591892937,37.190838720229,123.580846703996)) ;
#87237=CARTESIAN_POINT('Ctrl Pts',(-17.9046918793828,37.2008364550792,123.318229679078)) ;
#87238=CARTESIAN_POINT('Ctrl Pts',(-17.9432929783789,37.2107443590637,123.060725439739)) ;
#87239=CARTESIAN_POINT('Ctrl Pts',(-18.0264609446868,37.2207554336121,122.811128639324)) ;
#87240=CARTESIAN_POINT('Ctrl Pts',(-18.1523845768401,37.2307832891477,122.579637946315)) ;
#87241=CARTESIAN_POINT('Ctrl Pts',(-18.313434602913,37.240640883053,122.376742009224)) ;
#87242=CARTESIAN_POINT('Ctrl Pts',(-18.510241481172,37.2506675698911,122.201537057415)) ;
#87243=CARTESIAN_POINT('Ctrl Pts',(-18.7348729634303,37.2606962390448,122.063695449204)) ;
#87244=CARTESIAN_POINT('Ctrl Pts',(-18.9753445770678,37.2705414473262,121.96828080011)) ;
#87245=CARTESIAN_POINT('Ctrl Pts',(-19.2323500330995,37.2805321362893,121.914602131553)) ;
#87246=CARTESIAN_POINT('Ctrl Pts',(-19.4960202224024,37.2905700125716,121.9069126897)) ;
#87247=CARTESIAN_POINT('Ctrl Pts',(-19.7520669609929,37.3004143902138,121.943940420464)) ;
#87248=CARTESIAN_POINT('Ctrl Pts',(-20.0014193408441,37.3103991946052,122.025510816322)) ;
#87249=CARTESIAN_POINT('Ctrl Pts',(-20.2318871717339,37.3203387248238,122.148511202845)) ;
#87250=CARTESIAN_POINT('Ctrl Pts',(-20.4394866075736,37.3303784128607,122.311296862849)) ;
#87251=CARTESIAN_POINT('Ctrl Pts',(-20.6131300585679,37.340266702229,122.504635758308)) ;
#87252=CARTESIAN_POINT('Ctrl Pts',(-20.7523750420527,37.3502558259138,122.727153728378)) ;
#87253=CARTESIAN_POINT('Ctrl Pts',(-20.8503938939143,37.3602158355884,122.969841158144)) ;
#87254=CARTESIAN_POINT('Ctrl Pts',(-20.9050687368293,37.3701162652927,123.224212899945)) ;
#87255=CARTESIAN_POINT('Ctrl Pts',(-20.9148721088486,37.3801593466994,123.487941036205)) ;
#87256=CARTESIAN_POINT('Ctrl Pts',(-20.8792246033343,37.390066740607,123.745859387518)) ;
#87257=CARTESIAN_POINT('Ctrl Pts',(-20.7989609173973,37.4000784715962,123.996417274373)) ;
#87258=CARTESIAN_POINT('Ctrl Pts',(-20.6756955451906,37.410110689311,124.22947112403)) ;
#87259=CARTESIAN_POINT('Ctrl Pts',(-20.51702591384,37.4199631985572,124.434050623572)) ;
#87260=CARTESIAN_POINT('Ctrl Pts',(-20.3237233572184,37.4299211351002,124.610450271903)) ;
#87261=CARTESIAN_POINT('Ctrl Pts',(-20.1007000293467,37.4399600051085,124.751331487019)) ;
#87262=CARTESIAN_POINT('Ctrl Pts',(-19.8607616035958,37.4498331602667,124.850169231509)) ;
#87263=CARTESIAN_POINT('Ctrl Pts',(-19.602246757542,37.4599064351164,124.906872980276)) ;
#87264=CARTESIAN_POINT('Ctrl Pts',(-19.3443562287078,37.4697267522938,124.917896850224)) ;
#87265=CARTESIAN_POINT('Ctrl Pts',(-19.0818283552624,37.4798054380873,124.883340221226)) ;
#87266=CARTESIAN_POINT('Ctrl Pts',(-18.8348322832029,37.4896569494704,124.805570098911)) ;
#87267=CARTESIAN_POINT('Ctrl Pts',(-18.599913832951,37.499730395777,124.683655014206)) ;
#87268=CARTESIAN_POINT('Ctrl Pts',(-18.3945253990698,37.5095716709017,124.526446904205)) ;
#87269=CARTESIAN_POINT('Ctrl Pts',(-18.2164310699433,37.5195567705585,124.333775949038)) ;
#87270=CARTESIAN_POINT('Ctrl Pts',(-18.0744621012236,37.5295642466928,124.11237858257)) ;
#87271=CARTESIAN_POINT('Ctrl Pts',(-17.9737434063258,37.5394868344017,123.871874033015)) ;
#87272=CARTESIAN_POINT('Ctrl Pts',(-17.9155198712875,37.5494734386751,123.615951736417)) ;
#87273=CARTESIAN_POINT('Ctrl Pts',(-17.9030442398782,37.5595135670092,123.352424180443)) ;
#87274=CARTESIAN_POINT('Ctrl Pts',(-17.9352929472443,37.5693530015426,123.095845830502)) ;
#87275=CARTESIAN_POINT('Ctrl Pts',(-18.0131166461626,37.5794170560336,122.843116592569)) ;
#87276=CARTESIAN_POINT('Ctrl Pts',(-18.1316981730949,37.5893079752708,122.611787994209)) ;
#87277=CARTESIAN_POINT('Ctrl Pts',(-18.2897770295622,37.5992999685768,122.402140602484)) ;
#87278=CARTESIAN_POINT('Ctrl Pts',(-18.4814669497025,37.6092628325361,122.223821161659)) ;
#87279=CARTESIAN_POINT('Ctrl Pts',(-18.6995802858491,37.6191670923539,122.081762570876)) ;
#87280=CARTESIAN_POINT('Ctrl Pts',(-18.9428624159537,37.6292275829253,121.978356993375)) ;
#87281=CARTESIAN_POINT('Ctrl Pts',(-19.1947597030667,37.6390679325563,121.919723653256)) ;
#87282=CARTESIAN_POINT('Ctrl Pts',(-19.4587639337918,37.6491309080463,121.905087450184)) ;
#87283=CARTESIAN_POINT('Ctrl Pts',(-19.7169360685854,37.6590252281897,121.936206707452)) ;
#87284=CARTESIAN_POINT('Ctrl Pts',(-19.9671186320429,37.6689669413213,122.011348625595)) ;
#87285=CARTESIAN_POINT('Ctrl Pts',(-20.2020080675906,37.6789698311154,122.129443636696)) ;
#87286=CARTESIAN_POINT('Ctrl Pts',(-20.4132615576,37.6890096882759,122.287457794107)) ;
#87287=CARTESIAN_POINT('Ctrl Pts',(-20.5904502427968,37.6988338691135,122.475251891521)) ;
#87288=CARTESIAN_POINT('Ctrl Pts',(-20.735982916264,37.7088908426167,122.69583339334)) ;
#87289=CARTESIAN_POINT('Ctrl Pts',(-20.8393694687883,37.7188189668038,122.93539179218)) ;
#87290=CARTESIAN_POINT('Ctrl Pts',(-20.9004226762574,37.7287726618772,123.18974167518)) ;
#87291=CARTESIAN_POINT('Ctrl Pts',(-20.9161571182402,37.7388188554525,123.453273135493)) ;
#87292=CARTESIAN_POINT('Ctrl Pts',(-20.8867385875313,37.7486669578124,123.710392738064)) ;
#87293=CARTESIAN_POINT('Ctrl Pts',(-20.8130541065125,37.75862854604,123.96157704454)) ;
#87294=CARTESIAN_POINT('Ctrl Pts',(-20.6957843077402,37.7686572161963,124.197608569847)) ;
#87295=CARTESIAN_POINT('Ctrl Pts',(-20.5412434271641,37.778567519078,124.407217781717)) ;
#87296=CARTESIAN_POINT('Ctrl Pts',(-20.352645450369,37.7885024028859,124.58776383537)) ;
#87297=CARTESIAN_POINT('Ctrl Pts',(-20.133119143806,37.7985435445765,124.734158279139)) ;
#87298=CARTESIAN_POINT('Ctrl Pts',(-19.895266526059,37.8084306657405,124.838762309883)) ;
#87299=CARTESIAN_POINT('Ctrl Pts',(-19.6403142341081,37.818423008589,124.901552440905)) ;
#87300=CARTESIAN_POINT('Ctrl Pts',(-19.3794511200074,37.828371309813,124.918971337681)) ;
#87301=CARTESIAN_POINT('Ctrl Pts',(-19.1197938910939,37.8383088874951,124.891242488897)) ;
#87302=CARTESIAN_POINT('Ctrl Pts',(-18.8675519902502,37.8482954619457,124.818740589761)) ;
#87303=CARTESIAN_POINT('Ctrl Pts',(-18.6308845594972,37.8583242718541,124.702791487369)) ;
#87304=CARTESIAN_POINT('Ctrl Pts',(-18.4209911500482,37.8682025931609,124.550044711612)) ;
#87305=CARTESIAN_POINT('Ctrl Pts',(-18.2382893834789,37.8781942405083,124.361450555223)) ;
#87306=CARTESIAN_POINT('Ctrl Pts',(-18.0909361216224,37.8882287639461,124.142780458619)) ;
#87307=CARTESIAN_POINT('Ctrl Pts',(-17.9851082426078,37.8980921208247,123.90613973582)) ;
#87308=CARTESIAN_POINT('Ctrl Pts',(-17.9206158973704,37.908162347505,123.649512993499)) ;
#87309=CARTESIAN_POINT('Ctrl Pts',(-17.9021014477694,37.9180046556397,123.391519278401)) ;
#87310=CARTESIAN_POINT('Ctrl Pts',(-17.9280213893312,37.9279653876631,123.131054268142)) ;
#87311=CARTESIAN_POINT('Ctrl Pts',(-17.9998223639555,37.9380032768612,122.877238454483)) ;
#87312=CARTESIAN_POINT('Ctrl Pts',(-18.1123180047447,37.94787755978,122.643370168163)) ;
#87313=CARTESIAN_POINT('Ctrl Pts',(-18.2666811956989,37.9579473043975,122.428479079685)) ;
#87314=CARTESIAN_POINT('Ctrl Pts',(-18.4515097019627,37.9677806147431,122.247856374346)) ;
#87315=CARTESIAN_POINT('Ctrl Pts',(-18.6687188341038,37.9778108580958,122.098544975013)) ;
#87316=CARTESIAN_POINT('Ctrl Pts',(-18.9089398495734,37.9878431460742,121.989907265577)) ;
#87317=CARTESIAN_POINT('Ctrl Pts',(-19.1589973603507,37.9976703225423,121.925371796745)) ;
#87318=CARTESIAN_POINT('Ctrl Pts',(-19.4210528476622,38.0076757054092,121.904329796489)) ;
#87319=CARTESIAN_POINT('Ctrl Pts',(-19.6822603276462,38.0176583444019,121.929146579502)) ;
#87320=CARTESIAN_POINT('Ctrl Pts',(-19.9365866650456,38.0277024115385,121.999661380241)) ;
#87321=CARTESIAN_POINT('Ctrl Pts',(-20.1697455284941,38.0375236303425,122.110354265076)) ;
#87322=CARTESIAN_POINT('Ctrl Pts',(-20.3851407356152,38.0475604692805,122.262573522578)) ;
#87323=CARTESIAN_POINT('Ctrl Pts',(-20.5700791380799,38.0575848813783,122.450185779491)) ;
#87324=CARTESIAN_POINT('Ctrl Pts',(-20.7175310391498,38.0674369657836,122.663002255422)) ;
#87325=CARTESIAN_POINT('Ctrl Pts',(-20.8276645507075,38.0774278625268,122.901301885871)) ;
#87326=CARTESIAN_POINT('Ctrl Pts',(-20.8944393360025,38.0873458544277,123.153269837169)) ;
#87327=CARTESIAN_POINT('Ctrl Pts',(-20.916752709306,38.0973739698847,123.415831037644)) ;
#87328=CARTESIAN_POINT('Ctrl Pts',(-20.89358187262,38.1072591458268,123.674574253975)) ;
#87329=CARTESIAN_POINT('Ctrl Pts',(-20.8257391871181,38.1172485042337,123.928171654191)) ;
#87330=CARTESIAN_POINT('Ctrl Pts',(-20.7138167717013,38.127289651814,124.167129479311)) ;
#87331=CARTESIAN_POINT('Ctrl Pts',(-20.5656061454427,38.1371222748204,124.378785103182)) ;
#87332=CARTESIAN_POINT('Ctrl Pts',(-20.3804240799344,38.1471163459312,124.565013167833)) ;
#87333=CARTESIAN_POINT('Ctrl Pts',(-20.1646606886898,38.1571450035721,124.716368185705)) ;
#87334=CARTESIAN_POINT('Ctrl Pts',(-19.9294754177371,38.1670293297649,124.826601817947)) ;
#87335=CARTESIAN_POINT('Ctrl Pts',(-19.6768051124309,38.1769950732555,124.89551183432)) ;
#87336=CARTESIAN_POINT('Ctrl Pts',(-19.4143545698229,38.1870234523867,124.919272831667)) ;
#87337=CARTESIAN_POINT('Ctrl Pts',(-19.155026247405,38.1969242985936,124.897774472843)) ;
#87338=CARTESIAN_POINT('Ctrl Pts',(-18.899449911136,38.2069829560107,124.830469885562)) ;
#87339=CARTESIAN_POINT('Ctrl Pts',(-18.6640472589483,38.2168405187926,124.72223521876)) ;
#87340=CARTESIAN_POINT('Ctrl Pts',(-18.4464297173287,38.2269089213458,124.571809104608)) ;
#87341=CARTESIAN_POINT('Ctrl Pts',(-18.262192640318,38.2367643200854,124.389754401548)) ;
#87342=CARTESIAN_POINT('Ctrl Pts',(-18.1096196037123,38.2467591871593,124.175968694404)) ;
#87343=CARTESIAN_POINT('Ctrl Pts',(-17.9965795627306,38.2567904821428,123.937817735641)) ;
#87344=CARTESIAN_POINT('Ctrl Pts',(-17.9273563602029,38.2666570068693,123.687937654047)) ;
#87345=CARTESIAN_POINT('Ctrl Pts',(-17.9018527032758,38.276644477565,123.426751350671)) ;
#87346=CARTESIAN_POINT('Ctrl Pts',(-17.9218607437343,38.2865892371289,123.166140198543)) ;
#87347=CARTESIAN_POINT('Ctrl Pts',(-17.9876155290226,38.2966347930777,122.910504235427)) ;
#87348=CARTESIAN_POINT('Ctrl Pts',(-18.0945121468168,38.3064943814529,122.674449960714)) ;
#87349=CARTESIAN_POINT('Ctrl Pts',(-18.2424996480843,38.3164953365889,122.457313423853)) ;
#87350=CARTESIAN_POINT('Ctrl Pts',(-18.4240798301571,38.3263995638665,122.270788969546)) ;
#87351=CARTESIAN_POINT('Ctrl Pts',(-18.6381236155899,38.3364416407616,122.116493175448)) ;
#87352=CARTESIAN_POINT('Ctrl Pts',(-18.8725441547087,38.3463492534478,122.003091772094)) ;
#87353=CARTESIAN_POINT('Ctrl Pts',(-19.1267212481479,38.3564037840635,121.931068647469)) ;
#87354=CARTESIAN_POINT('Ctrl Pts',(-19.3845339848272,38.3662645706124,121.904631230091)) ;
#87355=CARTESIAN_POINT('Ctrl Pts',(-19.6464652984615,38.3762583256834,121.92312229318)) ;
#87356=CARTESIAN_POINT('Ctrl Pts',(-19.8995750129763,38.3861836859234,121.986273003471)) ;
#87357=CARTESIAN_POINT('Ctrl Pts',(-20.140272020409,38.3962116153187,122.093470120755)) ;
#87358=CARTESIAN_POINT('Ctrl Pts',(-20.3558252995868,38.406097882118,122.238568442777)) ;
#87359=CARTESIAN_POINT('Ctrl Pts',(-20.5456984409777,38.4161296510163,122.42138753169)) ;
#87360=CARTESIAN_POINT('Ctrl Pts',(-20.698877922451,38.4260112468599,122.631132419724)) ;
#87361=CARTESIAN_POINT('Ctrl Pts',(-20.8154213762224,38.4360731323278,122.8684346522)) ;
#87362=CARTESIAN_POINT('Ctrl Pts',(-20.8875986677405,38.4459305663467,123.117253823727)) ;
#87363=CARTESIAN_POINT('Ctrl Pts',(-20.9164045121782,38.4559238093887,123.378246907377)) ;
#87364=CARTESIAN_POINT('Ctrl Pts',(-20.8995775457113,38.465854570275,123.638690081529)) ;
#87365=CARTESIAN_POINT('Ctrl Pts',(-20.816850334482,38.4792035624722,123.979625573362)) ;
#87366=CARTESIAN_POINT('Ctrl Pts',(-20.6476612787041,38.4924719352886,124.289010646964)) ;
#87367=CARTESIAN_POINT('Ctrl Pts',(-20.4070708455003,38.505754876673,124.541958141041)) ;
#87368=CARTESIAN_POINT('Ctrl Pts',(-20.1946437063502,38.5157976625152,124.698532719528)) ;
#87369=CARTESIAN_POINT('Ctrl Pts',(-19.9628978193437,38.5256476050673,124.813858968729)) ;
#87370=CARTESIAN_POINT('Ctrl Pts',(-19.7111423066587,38.5356448379863,124.888916493239)) ;
#87371=CARTESIAN_POINT('Ctrl Pts',(-19.4496444734046,38.5456597333208,124.918770576671)) ;
#87372=CARTESIAN_POINT('Ctrl Pts',(-19.102347554309,38.558899409959,124.897958325602)) ;
#87373=CARTESIAN_POINT('Ctrl Pts',(-18.6847987628518,38.5754466343643,124.759928991449)) ;
#87374=CARTESIAN_POINT('Ctrl Pts',(-18.3371659709119,38.5920940714954,124.486215378783)) ;
#87375=CARTESIAN_POINT('Ctrl Pts',(-18.1282833266673,38.6053835689736,124.206304846633)) ;
#87376=CARTESIAN_POINT('Ctrl Pts',(-18.0108766480719,38.615256976796,123.974924396754)) ;
#87377=CARTESIAN_POINT('Ctrl Pts',(-17.9340194463027,38.6253093543887,123.722198205263)) ;
#87378=CARTESIAN_POINT('Ctrl Pts',(-17.9027887073884,38.6352130079296,123.463801752552)) ;
#87379=CARTESIAN_POINT('Ctrl Pts',(-17.9163242119673,38.6451572769249,123.202860594878)) ;
#87380=CARTESIAN_POINT('Ctrl Pts',(-17.9947872688244,38.6584882852576,122.861360560677)) ;
#87381=CARTESIAN_POINT('Ctrl Pts',(-18.2021257874539,38.6751098657819,122.471340515978)) ;
#87382=CARTESIAN_POINT('Ctrl Pts',(-18.5280196716949,38.6916525364803,122.176175599121)) ;
#87383=CARTESIAN_POINT('Ctrl Pts',(-18.84008875281,38.7050016960432,122.015952826464)) ;
#87384=CARTESIAN_POINT('Ctrl Pts',(-19.1721179105993,38.7182298462027,121.912874830925)) ;
#87385=CARTESIAN_POINT('Ctrl Pts',(-19.6137093351474,38.7348605233402,121.89504706836)) ;
#87386=CARTESIAN_POINT('Ctrl Pts',(-20.1178745686584,38.7547634626283,122.055405875493)) ;
#87387=CARTESIAN_POINT('Ctrl Pts',(-20.5372564996866,38.7746663292316,122.377645054216)) ;
#87388=CARTESIAN_POINT('Ctrl Pts',(-20.8224486031123,38.7945794943364,122.823633412691)) ;
#87389=CARTESIAN_POINT('Ctrl Pts',(-20.9381893408,38.8146153234777,123.343346667635)) ;
#87390=CARTESIAN_POINT('Ctrl Pts',(-20.8706660685584,38.8344338983558,123.865874261203)) ;
#87391=CARTESIAN_POINT('Ctrl Pts',(-20.627922443163,38.8544041993978,124.337692899044)) ;
#87392=CARTESIAN_POINT('Ctrl Pts',(-20.2401234229137,38.8742957317623,124.69730681963)) ;
#87393=CARTESIAN_POINT('Ctrl Pts',(-19.7497967047093,38.8943188295789,124.903871868757)) ;
#87394=CARTESIAN_POINT('Ctrl Pts',(-19.2242573161077,38.9141155824988,124.930795625851)) ;
#87395=CARTESIAN_POINT('Ctrl Pts',(-18.7165907441389,38.9340766709876,124.776879006077)) ;
#87396=CARTESIAN_POINT('Ctrl Pts',(-18.2921488184441,38.9540549399198,124.457746589565)) ;
#87397=CARTESIAN_POINT('Ctrl Pts',(-18.0037947360342,38.9738749547108,124.016952429214)) ;
#87398=CARTESIAN_POINT('Ctrl Pts',(-17.8810979198861,38.9938133639626,123.501394794737)) ;
#87399=CARTESIAN_POINT('Ctrl Pts',(-17.9432262389664,39.013860481355,122.972141220867)) ;
#87400=CARTESIAN_POINT('Ctrl Pts',(-18.179999474083,39.0337067271889,122.500852961374)) ;
#87401=CARTESIAN_POINT('Ctrl Pts',(-18.5620692319856,39.0535556957009,122.137036795423)) ;
#87402=CARTESIAN_POINT('Ctrl Pts',(-19.0504584844477,39.0736059980122,121.923948334636)) ;
#87403=CARTESIAN_POINT('Ctrl Pts',(-19.5767211389698,39.0934409204434,121.8907738155)) ;
#87404=CARTESIAN_POINT('Ctrl Pts',(-20.0851205819504,39.1133713216693,122.038805273945)) ;
#87405=CARTESIAN_POINT('Ctrl Pts',(-20.5122385328754,39.1332562670282,122.350424357377)) ;
#87406=CARTESIAN_POINT('Ctrl Pts',(-20.8092718181263,39.1533288751795,122.793463019832)) ;
#87407=CARTESIAN_POINT('Ctrl Pts',(-20.9356236783323,39.1731201915077,123.304163853874)) ;
#87408=CARTESIAN_POINT('Ctrl Pts',(-20.8812715084831,39.1930849812749,123.831959781897)) ;
#87409=CARTESIAN_POINT('Ctrl Pts',(-20.6486431634336,39.2130679370252,124.309427208045)) ;
#87410=CARTESIAN_POINT('Ctrl Pts',(-20.2711039549004,39.2328764590014,124.676430038506)) ;
#87411=CARTESIAN_POINT('Ctrl Pts',(-19.7870902404589,39.2528620337372,124.894984520865)) ;
#87412=CARTESIAN_POINT('Ctrl Pts',(-19.2600307895484,39.2727446738056,124.934952427669)) ;
#87413=CARTESIAN_POINT('Ctrl Pts',(-18.7492190934437,39.2926999859375,124.792610565746)) ;
#87414=CARTESIAN_POINT('Ctrl Pts',(-18.3190388924115,39.3125743425453,124.485911249285)) ;
#87415=CARTESIAN_POINT('Ctrl Pts',(-18.0175162438669,39.3325565494064,124.048781584885)) ;
#87416=CARTESIAN_POINT('Ctrl Pts',(-17.8838364996547,39.3524876273563,123.536075517646)) ;
#87417=CARTESIAN_POINT('Ctrl Pts',(-17.9330377132969,39.3724146022113,123.008847051512)) ;
#87418=CARTESIAN_POINT('Ctrl Pts',(-18.1572602607085,39.3922470611602,122.531726093143)) ;
#87419=CARTESIAN_POINT('Ctrl Pts',(-18.4706715836701,39.4089047453354,122.219175253551)) ;
#87420=CARTESIAN_POINT('Ctrl Pts',(-18.7724853140679,39.4221539692425,122.045409139846)) ;
#87421=CARTESIAN_POINT('Ctrl Pts',(-19.0206746467771,39.4322029906937,121.95528639923)) ;
#87422=CARTESIAN_POINT('Ctrl Pts',(-19.2758714027625,39.4420629989242,121.910414373671)) ;
#87423=CARTESIAN_POINT('Ctrl Pts',(-19.6249850662901,39.4553465121488,121.909430053781)) ;
#87424=CARTESIAN_POINT('Ctrl Pts',(-20.0524695157253,39.4719924311496,122.023204765113)) ;
#87425=CARTESIAN_POINT('Ctrl Pts',(-20.4138864148045,39.4885464089657,122.274186137911)) ;
#87426=CARTESIAN_POINT('Ctrl Pts',(-20.6406300091737,39.5019061379373,122.542218010001)) ;
#87427=CARTESIAN_POINT('Ctrl Pts',(-20.7717096169385,39.511799189734,122.766754046185)) ;
#87428=CARTESIAN_POINT('Ctrl Pts',(-20.8630087660866,39.521789155015,123.012860662966)) ;
#87429=CARTESIAN_POINT('Ctrl Pts',(-20.9101748143691,39.5317410358759,123.270138684946)) ;
#87430=CARTESIAN_POINT('Ctrl Pts',(-20.9117456673708,39.5417893875677,123.534165997582)) ;
#87431=CARTESIAN_POINT('Ctrl Pts',(-20.8686552536552,39.5516306716739,123.789195920828)) ;
#87432=CARTESIAN_POINT('Ctrl Pts',(-20.7812002337361,39.5616173747996,124.036586790097)) ;
#87433=CARTESIAN_POINT('Ctrl Pts',(-20.6528795142412,39.571552403617,124.264016264375)) ;
#87434=CARTESIAN_POINT('Ctrl Pts',(-20.4848907700779,39.5816081985239,124.46795141361)) ;
#87435=CARTESIAN_POINT('Ctrl Pts',(-20.2887891671277,39.5914365618132,124.636091146284)) ;
#87436=CARTESIAN_POINT('Ctrl Pts',(-20.0614641234576,39.6014975317111,124.771025787529)) ;
#87437=CARTESIAN_POINT('Ctrl Pts',(-19.8176332037188,39.6114118106009,124.862898597772)) ;
#87438=CARTESIAN_POINT('Ctrl Pts',(-19.5592282819904,39.6214208050691,124.912002571716)) ;
#87439=CARTESIAN_POINT('Ctrl Pts',(-19.2956754516133,39.6314506396329,124.914961194742)) ;
#87440=CARTESIAN_POINT('Ctrl Pts',(-19.0399610301937,39.6413088697051,124.873328894269)) ;
#87441=CARTESIAN_POINT('Ctrl Pts',(-18.7918272427075,39.6513075754475,124.787030713098)) ;
#87442=CARTESIAN_POINT('Ctrl Pts',(-18.5646041239284,39.6612022313663,124.660518202869)) ;
#87443=CARTESIAN_POINT('Ctrl Pts',(-18.3594891226658,39.6712652957503,124.493676816178)) ;
#87444=CARTESIAN_POINT('Ctrl Pts',(-18.1900268540481,39.6811049540302,124.298315227073)) ;
#87445=CARTESIAN_POINT('Ctrl Pts',(-18.053792583236,39.691168121112,124.071699946612)) ;
#87446=CARTESIAN_POINT('Ctrl Pts',(-17.960749315,39.7010623662391,123.828876199066)) ;
#87447=CARTESIAN_POINT('Ctrl Pts',(-17.9103583441189,39.7110041878437,123.572554229599)) ;
#87448=CARTESIAN_POINT('Ctrl Pts',(-17.9051091078073,39.7210067187618,123.309715572966)) ;
#87449=CARTESIAN_POINT('Ctrl Pts',(-17.9461034213345,39.7310413452193,123.049236091637)) ;
#87450=CARTESIAN_POINT('Ctrl Pts',(-18.0297068679523,39.7408868802057,122.804375715976)) ;
#87451=CARTESIAN_POINT('Ctrl Pts',(-18.1557911659349,39.7508703050448,122.574330051635)) ;
#87452=CARTESIAN_POINT('Ctrl Pts',(-18.3194197366641,39.7608206954098,122.370358879002)) ;
#87453=CARTESIAN_POINT('Ctrl Pts',(-18.5166895154144,39.7708183357069,122.1968019572)) ;
#87454=CARTESIAN_POINT('Ctrl Pts',(-18.7422717110751,39.7808574162701,122.06004045278)) ;
#87455=CARTESIAN_POINT('Ctrl Pts',(-18.9827757053251,39.7906835670392,121.966001404595)) ;
#87456=CARTESIAN_POINT('Ctrl Pts',(-19.241779151991,39.8007401419683,121.913550884301)) ;
#87457=CARTESIAN_POINT('Ctrl Pts',(-19.5029424763994,39.8106806813486,121.907401203059)) ;
#87458=CARTESIAN_POINT('Ctrl Pts',(-19.7603853137432,39.820585074325,121.945742920367)) ;
#87459=CARTESIAN_POINT('Ctrl Pts',(-20.0107266937267,39.8306317285299,122.029537599121)) ;
#87460=CARTESIAN_POINT('Ctrl Pts',(-20.2393968682051,39.8405272904683,122.153454191526)) ;
#87461=CARTESIAN_POINT('Ctrl Pts',(-20.4464414983218,39.8505893683139,122.317864784386)) ;
#87462=CARTESIAN_POINT('Ctrl Pts',(-20.6181263774124,39.8604320667276,122.511365345899)) ;
#87463=CARTESIAN_POINT('Ctrl Pts',(-20.7561382322086,39.8704228416891,122.734672291079)) ;
#87464=CARTESIAN_POINT('Ctrl Pts',(-20.8526500680807,39.8803507067082,122.97707426249)) ;
#87465=CARTESIAN_POINT('Ctrl Pts',(-20.9063594910296,39.8903394514744,123.234019741878)) ;
#87466=CARTESIAN_POINT('Ctrl Pts',(-20.9142878541207,39.9003722370613,123.497555642552)) ;
#87467=CARTESIAN_POINT('Ctrl Pts',(-20.8772279525817,39.910238921682,123.754170693425)) ;
#87468=CARTESIAN_POINT('Ctrl Pts',(-20.7961043668712,39.9202008138451,124.003076881027)) ;
#87469=CARTESIAN_POINT('Ctrl Pts',(-20.6717493071348,39.9302342907577,124.2355665129)) ;
#87470=CARTESIAN_POINT('Ctrl Pts',(-20.5116325782537,39.940118632006,124.440138606861)) ;
#87471=CARTESIAN_POINT('Ctrl Pts',(-20.3149883606172,39.9501815741271,124.61689780952)) ;
#87472=CARTESIAN_POINT('Ctrl Pts',(-20.0953995131372,39.9600319757467,124.754007658767)) ;
#87473=CARTESIAN_POINT('Ctrl Pts',(-19.8513143447031,39.9700588645364,124.853250471539)) ;
#87474=CARTESIAN_POINT('Ctrl Pts',(-19.5934970141475,39.9800874794926,124.907943166141)) ;
#87475=CARTESIAN_POINT('Ctrl Pts',(-19.3349601607156,39.9899327026126,124.917361759063)) ;
#87476=CARTESIAN_POINT('Ctrl Pts',(-19.0748122096571,39.9999233864186,124.881915578707)) ;
#87477=CARTESIAN_POINT('Ctrl Pts',(-18.8237784515497,40.009961268491,124.800902625927)) ;
#87478=CARTESIAN_POINT('Ctrl Pts',(-18.5948964274932,40.0198056281299,124.68030432098)) ;
#87479=CARTESIAN_POINT('Ctrl Pts',(-18.3872328665451,40.0297904987446,124.519971576075)) ;
#87480=CARTESIAN_POINT('Ctrl Pts',(-18.2112308942488,40.0397297820733,124.326928042325)) ;
#87481=CARTESIAN_POINT('Ctrl Pts',(-18.0701011370966,40.0497703914464,124.10401924585)) ;
#87482=CARTESIAN_POINT('Ctrl Pts',(-17.9711747293191,40.0596552423596,123.863797270785)) ;
#87483=CARTESIAN_POINT('Ctrl Pts',(-17.914507891847,40.0696571985284,123.607177988291)) ;
#87484=CARTESIAN_POINT('Ctrl Pts',(-17.9031408318448,40.0795757952489,123.346733888948)) ;
#87485=CARTESIAN_POINT('Ctrl Pts',(-17.9376487606401,40.0896226173247,123.085016388873)) ;
#87486=CARTESIAN_POINT('Ctrl Pts',(-18.0155031495141,40.0994968984374,122.837438413162)) ;
#87487=CARTESIAN_POINT('Ctrl Pts',(-18.1371591486748,40.109551098482,122.602950598639)) ;
#87488=CARTESIAN_POINT('Ctrl Pts',(-18.2951196454476,40.1194465281173,122.396320882415)) ;
#87489=CARTESIAN_POINT('Ctrl Pts',(-18.4896702718675,40.1295081564346,122.217309891194)) ;
#87490=CARTESIAN_POINT('Ctrl Pts',(-18.7075627861497,40.1393527852645,122.077821066016)) ;
#87491=CARTESIAN_POINT('Ctrl Pts',(-18.9487886325186,40.1493128328701,121.976254285154)) ;
#87492=CARTESIAN_POINT('Ctrl Pts',(-19.2060965362213,40.1593511390442,121.918165822933)) ;
#87493=CARTESIAN_POINT('Ctrl Pts',(-19.4652798129029,40.1692244384768,121.905341126692)) ;
#87494=CARTESIAN_POINT('Ctrl Pts',(-19.7278620306309,40.1792977000631,121.938443177458)) ;
#87495=CARTESIAN_POINT('Ctrl Pts',(-19.9745652121543,40.1891179260198,122.014376604329)) ;
#87496=CARTESIAN_POINT('Ctrl Pts',(-20.210384152523,40.1991969899593,122.134825848413)) ;
#87497=CARTESIAN_POINT('Ctrl Pts',(-20.4170898719692,40.2090470799791,122.290751429487)) ;
#87498=CARTESIAN_POINT('Ctrl Pts',(-20.5976846428322,40.2191258335929,122.484401518764)) ;
#87499=CARTESIAN_POINT('Ctrl Pts',(-20.7384649199968,40.2289473008524,122.700793862279)) ;
#87500=CARTESIAN_POINT('Ctrl Pts',(-20.8423732928383,40.23901289921,122.943977873275)) ;
#87501=CARTESIAN_POINT('Ctrl Pts',(-20.9014655130511,40.2489155549847,123.197477874162)) ;
#87502=CARTESIAN_POINT('Ctrl Pts',(-20.9159315140315,40.2589663808143,123.461152741984)) ;
#87503=CARTESIAN_POINT('Ctrl Pts',(-20.8851862687562,40.2688405851532,123.718866407652)) ;
#87504=CARTESIAN_POINT('Ctrl Pts',(-20.8087033848994,40.2789130351923,123.972210529531)) ;
#87505=CARTESIAN_POINT('Ctrl Pts',(-20.6924508708633,40.2887420519658,124.202923123241)) ;
#87506=CARTESIAN_POINT('Ctrl Pts',(-20.534514449587,40.2988088978806,124.415095541138)) ;
#87507=CARTESIAN_POINT('Ctrl Pts',(-20.3453419288887,40.3086990691824,124.593367187674)) ;
#87508=CARTESIAN_POINT('Ctrl Pts',(-20.126206043176,40.3186912628062,124.738011905012)) ;
#87509=CARTESIAN_POINT('Ctrl Pts',(-19.8858849575961,40.3286540734297,124.841878589706)) ;
#87510=CARTESIAN_POINT('Ctrl Pts',(-19.6328023115127,40.3385583462731,124.902733214097)) ;
#87511=CARTESIAN_POINT('Ctrl Pts',(-19.368941004048,40.3486188380777,124.918739240953)) ;
#87512=CARTESIAN_POINT('Ctrl Pts',(-19.111948949925,40.3584591697501,124.889672424697)) ;
#87513=CARTESIAN_POINT('Ctrl Pts',(-18.8582728174585,40.3685222158418,124.815092864794)) ;
#87514=CARTESIAN_POINT('Ctrl Pts',(-18.6254185641157,40.3784162715369,124.699353388829)) ;
#87515=CARTESIAN_POINT('Ctrl Pts',(-18.414789936686,40.3883589718599,124.544790683395)) ;
#87516=CARTESIAN_POINT('Ctrl Pts',(-18.2329762001901,40.3983647127875,124.354801620633)) ;
#87517=CARTESIAN_POINT('Ctrl Pts',(-18.0869571139645,40.408385623303,124.135661151696)) ;
#87518=CARTESIAN_POINT('Ctrl Pts',(-17.982299068752,40.418276358753,123.897735676412)) ;
#87519=CARTESIAN_POINT('Ctrl Pts',(-17.9195403076832,40.4282678994818,123.64278976609)) ;
#87520=CARTESIAN_POINT('Ctrl Pts',(-17.9021523398952,40.4382157599035,123.381951195381)) ;
#87521=CARTESIAN_POINT('Ctrl Pts',(-17.9298041725074,40.4481624290898,123.122015017719)) ;
#87522=CARTESIAN_POINT('Ctrl Pts',(-18.0031779584756,40.4582105052254,122.868371382531)) ;
#87523=CARTESIAN_POINT('Ctrl Pts',(-18.1169687224454,40.468058103231,122.635944200235)) ;
#87524=CARTESIAN_POINT('Ctrl Pts',(-18.2704811318407,40.4780198263155,122.423910978732)) ;
#87525=CARTESIAN_POINT('Ctrl Pts',(-18.4599935581485,40.4880484613985,122.240750173216)) ;
#87526=CARTESIAN_POINT('Ctrl Pts',(-18.6757822343563,40.4979587697165,122.094962047602)) ;
#87527=CARTESIAN_POINT('Ctrl Pts',(-18.9139355025239,40.5078936668524,121.987961124184)) ;
#87528=CARTESIAN_POINT('Ctrl Pts',(-19.1697997287511,40.517934749795,121.923493244547)) ;
#87529=CARTESIAN_POINT('Ctrl Pts',(-19.428950366049,40.5278220926232,121.904543523959)) ;
#87530=CARTESIAN_POINT('Ctrl Pts',(-19.6901959445774,40.5378136075626,121.930704214457)) ;
#87531=CARTESIAN_POINT('Ctrl Pts',(-19.9419057770973,40.5477649987591,122.001654050665)) ;
#87532=CARTESIAN_POINT('Ctrl Pts',(-20.1772160470658,40.5576975320917,122.114605806638)) ;
#87533=CARTESIAN_POINT('Ctrl Pts',(-20.390773351119,40.5676946899911,122.267599496389)) ;
#87534=CARTESIAN_POINT('Ctrl Pts',(-20.5744051539528,40.5776797001546,122.455089020715)) ;
#87535=CARTESIAN_POINT('Ctrl Pts',(-20.723188468568,40.5877225267244,122.673023900318)) ;
#87536=CARTESIAN_POINT('Ctrl Pts',(-20.8301426365293,40.5975527610294,122.908217068064)) ;
#87537=CARTESIAN_POINT('Ctrl Pts',(-20.8963379142863,40.607628786264,123.164540306248)) ;
#87538=CARTESIAN_POINT('Ctrl Pts',(-20.9167055563444,40.6174810227549,123.422701150021)) ;
#87539=CARTESIAN_POINT('Ctrl Pts',(-20.891615051151,40.627554229189,123.686179366379)) ;
#87540=CARTESIAN_POINT('Ctrl Pts',(-20.8226924038434,40.6373957386962,123.935469529968)) ;
#87541=CARTESIAN_POINT('Ctrl Pts',(-20.7110845119955,40.647356685476,124.172237837628)) ;
#87542=CARTESIAN_POINT('Ctrl Pts',(-20.5584645897465,40.657394514276,124.387376516039)) ;
#87543=CARTESIAN_POINT('Ctrl Pts',(-20.3741751702042,40.6672688240305,124.570098190474)) ;
#87544=CARTESIAN_POINT('Ctrl Pts',(-20.1567868434197,40.6773385217037,124.720922673687)) ;
#87545=CARTESIAN_POINT('Ctrl Pts',(-19.9221561017423,40.6871719929911,124.829257549577)) ;
#87546=CARTESIAN_POINT('Ctrl Pts',(-19.6675134133936,40.697201639521,124.897250208865)) ;
#87547=CARTESIAN_POINT('Ctrl Pts',(-19.404726915787,40.7072361538484,124.919206335434)) ;
#87548=CARTESIAN_POINT('Ctrl Pts',(-19.1475426653616,40.7170614393193,124.896320551621)) ;
#87549=CARTESIAN_POINT('Ctrl Pts',(-18.8935848410147,40.7270656808678,124.828449926807)) ;
#87550=CARTESIAN_POINT('Ctrl Pts',(-18.6557571219536,40.7370483259469,124.717619979883)) ;
#87551=CARTESIAN_POINT('Ctrl Pts',(-18.4396753878514,40.7470935230384,124.566036174496)) ;
#87552=CARTESIAN_POINT('Ctrl Pts',(-18.2569837011254,40.7569166387985,124.383646814928)) ;
#87553=CARTESIAN_POINT('Ctrl Pts',(-18.1050079926846,40.7669512505988,124.168150561838)) ;
#87554=CARTESIAN_POINT('Ctrl Pts',(-17.9935267427077,40.776976259372,123.929445084339)) ;
#87555=CARTESIAN_POINT('Ctrl Pts',(-17.9258202753636,40.7868281842135,123.679551402899)) ;
#87556=CARTESIAN_POINT('Ctrl Pts',(-17.9018056354857,40.7968191225363,123.418132469691)) ;
#87557=CARTESIAN_POINT('Ctrl Pts',(-17.9232248951131,40.8067371076827,123.158348244679)) ;
#87558=CARTESIAN_POINT('Ctrl Pts',(-17.9900857838276,40.8167652085782,122.903464281987)) ;
#87559=CARTESIAN_POINT('Ctrl Pts',(-18.0985313024471,40.8266504495208,122.667402977687)) ;
#87560=CARTESIAN_POINT('Ctrl Pts',(-18.2473410925538,40.8366395624874,122.451144336104)) ;
#87561=CARTESIAN_POINT('Ctrl Pts',(-18.4328177933568,40.8466816268282,122.263433343905)) ;
#87562=CARTESIAN_POINT('Ctrl Pts',(-18.6432373021323,40.8565108282327,122.113605035665)) ;
#87563=CARTESIAN_POINT('Ctrl Pts',(-18.8804063338663,40.8665176689909,122.000080751744)) ;
#87564=CARTESIAN_POINT('Ctrl Pts',(-19.1333087574883,40.8765051931828,121.929728664348)) ;
#87565=CARTESIAN_POINT('Ctrl Pts',(-19.3956374933461,40.8865348389914,121.904438993338)) ;
#87566=CARTESIAN_POINT('Ctrl Pts',(-19.6543707145139,40.8964088697302,121.924454848222)) ;
#87567=CARTESIAN_POINT('Ctrl Pts',(-19.9089008937694,40.9064081925943,121.989579416378)) ;
#87568=CARTESIAN_POINT('Ctrl Pts',(-20.1463240582721,40.9163190281699,122.096753063302)) ;
#87569=CARTESIAN_POINT('Ctrl Pts',(-20.3645193729387,40.9263732761439,122.245676406375)) ;
#87570=CARTESIAN_POINT('Ctrl Pts',(-20.5501419901856,40.9362320204066,122.42647707007)) ;
#87571=CARTESIAN_POINT('Ctrl Pts',(-20.7048457015326,40.9463001064796,122.641065679255)) ;
#87572=CARTESIAN_POINT('Ctrl Pts',(-20.8175173641889,40.9561555896591,122.874289210237)) ;
#87573=CARTESIAN_POINT('Ctrl Pts',(-20.8897275055665,40.9661504354533,123.126813177261)) ;
#87574=CARTESIAN_POINT('Ctrl Pts',(-20.9165302141604,40.9761817311159,123.389064120819)) ;
#87575=CARTESIAN_POINT('Ctrl Pts',(-20.898116848103,40.9860482744057,123.647700931821)) ;
#87576=CARTESIAN_POINT('Ctrl Pts',(-20.8347236238339,40.9960356701691,123.902356200774)) ;
#87577=CARTESIAN_POINT('Ctrl Pts',(-20.7286285702455,41.0059807108991,124.141239921477)) ;
#87578=CARTESIAN_POINT('Ctrl Pts',(-20.5811211598771,41.0160252171158,124.360105227099)) ;
#87579=CARTESIAN_POINT('Ctrl Pts',(-20.4012876880261,41.0258887232531,124.546811663943)) ;
#87580=CARTESIAN_POINT('Ctrl Pts',(-20.1893463018213,41.0358815840892,124.701796997942)) ;
#87581=CARTESIAN_POINT('Ctrl Pts',(-19.9552720707621,41.0458077778081,124.816998522553)) ;
#87582=CARTESIAN_POINT('Ctrl Pts',(-19.7024899327944,41.0558267038407,124.890516309692)) ;
#87583=CARTESIAN_POINT('Ctrl Pts',(-19.4434540809893,41.0657417032083,124.918982353563)) ;
#87584=CARTESIAN_POINT('Ctrl Pts',(-19.179821038914,41.0757964747656,124.901749795245)) ;
#87585=CARTESIAN_POINT('Ctrl Pts',(-18.9280800412219,41.0856554370632,124.840372296681)) ;
#87586=CARTESIAN_POINT('Ctrl Pts',(-18.6874351062413,41.095649680901,124.735268941808)) ;
#87587=CARTESIAN_POINT('Ctrl Pts',(-18.4700684891871,41.1055749103252,124.591037888929)) ;
#87588=CARTESIAN_POINT('Ctrl Pts',(-18.2791378076578,41.1156028742167,124.409455504001)) ;
#87589=CARTESIAN_POINT('Ctrl Pts',(-18.1245883806122,41.1254891338471,124.20057485489)) ;
#87590=CARTESIAN_POINT('Ctrl Pts',(-18.0068635292268,41.1355208969249,123.964745548738)) ;
#87591=CARTESIAN_POINT('Ctrl Pts',(-17.9327293076382,41.1454025232191,123.715825423128)) ;
#87592=CARTESIAN_POINT('Ctrl Pts',(-17.9023394171472,41.1554642927052,123.453203976772)) ;
#87593=CARTESIAN_POINT('Ctrl Pts',(-17.9176211064176,41.1653221602007,123.194569188612)) ;
#87594=CARTESIAN_POINT('Ctrl Pts',(-17.9778112462982,41.1753137853181,122.939023648064)) ;
#87595=CARTESIAN_POINT('Ctrl Pts',(-18.0809522301768,41.1852505844263,122.699110258918)) ;
#87596=CARTESIAN_POINT('Ctrl Pts',(-18.2246372961258,41.1952414139836,122.479365383899)) ;
#87597=CARTESIAN_POINT('Ctrl Pts',(-18.4051031632681,41.2052646496968,122.287492545493)) ;
#87598=CARTESIAN_POINT('Ctrl Pts',(-18.6133310445568,41.215160997726,122.131695698258)) ;
#87599=CARTESIAN_POINT('Ctrl Pts',(-18.8473975521708,41.2251505602285,122.012807543813)) ;
#87600=CARTESIAN_POINT('Ctrl Pts',(-19.0999569107167,41.235190867913,121.936495551711)) ;
#87601=CARTESIAN_POINT('Ctrl Pts',(-19.35673862267,41.2450331712602,121.905316610654)) ;
#87602=CARTESIAN_POINT('Ctrl Pts',(-19.619750139844,41.2550568795393,121.919098001981)) ;
#87603=CARTESIAN_POINT('Ctrl Pts',(-19.9583979422888,41.268279057007,121.997129854709)) ;
#87604=CARTESIAN_POINT('Ctrl Pts',(-20.2706317559911,41.2815716420663,122.162222495001)) ;
#87605=CARTESIAN_POINT('Ctrl Pts',(-20.5265422578919,41.2948564979879,122.399798532575)) ;
#87606=CARTESIAN_POINT('Ctrl Pts',(-20.6848531440753,41.3048287251607,122.608586988607)) ;
#87607=CARTESIAN_POINT('Ctrl Pts',(-20.8041778753836,41.3147373415997,122.840061396327)) ;
#87608=CARTESIAN_POINT('Ctrl Pts',(-20.8825078353512,41.3247905469834,123.092342498857)) ;
#87609=CARTESIAN_POINT('Ctrl Pts',(-20.9153911019207,41.3346556807437,123.349517175633)) ;
#87610=CARTESIAN_POINT('Ctrl Pts',(-20.8994532016943,41.34799473837,123.699671410169)) ;
#87611=CARTESIAN_POINT('Ctrl Pts',(-20.7662682588357,41.3645639257032,124.119498420051)) ;
#87612=CARTESIAN_POINT('Ctrl Pts',(-20.4969289351474,41.3812090655542,124.470369460942)) ;
#87613=CARTESIAN_POINT('Ctrl Pts',(-20.2201112015402,41.3944813680276,124.682651973969)) ;
#87614=CARTESIAN_POINT('Ctrl Pts',(-19.9875982884763,41.4044623314752,124.803972762843)) ;
#87615=CARTESIAN_POINT('Ctrl Pts',(-19.738528944689,41.4144041635445,124.882935891262)) ;
#87616=CARTESIAN_POINT('Ctrl Pts',(-19.3916330563447,41.42772373276,124.929305565793)) ;
#87617=CARTESIAN_POINT('Ctrl Pts',(-18.9557211738586,41.4442538876927,124.873625074331)) ;
#87618=CARTESIAN_POINT('Ctrl Pts',(-18.4827898293542,41.4642756131848,124.629964635199)) ;
#87619=CARTESIAN_POINT('Ctrl Pts',(-18.1247913754587,41.4840870097916,124.243659355812)) ;
#87620=CARTESIAN_POINT('Ctrl Pts',(-17.9175945300158,41.5040722585005,123.754695417451)) ;
#87621=CARTESIAN_POINT('Ctrl Pts',(-17.8901702572938,41.5239663211364,123.226570828249)) ;
#87622=CARTESIAN_POINT('Ctrl Pts',(-18.0441233573117,41.54389800031,122.719693569398)) ;
#87623=CARTESIAN_POINT('Ctrl Pts',(-18.3626064665209,41.563862054782,122.295289089254)) ;
#87624=CARTESIAN_POINT('Ctrl Pts',(-18.8047488016914,41.5837429565449,122.005904879941)) ;
#87625=CARTESIAN_POINT('Ctrl Pts',(-19.320432669292,41.6036816181533,121.883949466073)) ;
#87626=CARTESIAN_POINT('Ctrl Pts',(-19.845694207807,41.6235781434086,121.945081447372)) ;
#87627=CARTESIAN_POINT('Ctrl Pts',(-20.3189427672172,41.6434731818629,122.181005425179)) ;
#87628=CARTESIAN_POINT('Ctrl Pts',(-20.6844409401465,41.663437005169,122.565598444425)) ;
#87629=CARTESIAN_POINT('Ctrl Pts',(-20.8961948389639,41.6833111292981,123.049559754929)) ;
#87630=CARTESIAN_POINT('Ctrl Pts',(-20.930750337764,41.7032862050253,123.5793623284)) ;
#87631=CARTESIAN_POINT('Ctrl Pts',(-20.7818779747331,41.7232397743819,124.088362609543)) ;
#87632=CARTESIAN_POINT('Ctrl Pts',(-20.4708653827436,41.7430776845698,124.514126207426)) ;
#87633=CARTESIAN_POINT('Ctrl Pts',(-20.0305044149458,41.7630535131407,124.810712363069)) ;
#87634=CARTESIAN_POINT('Ctrl Pts',(-19.5167523633582,41.782971557851,124.938278605792)) ;
#87635=CARTESIAN_POINT('Ctrl Pts',(-18.9912886178478,41.8028418036386,124.884326486846)) ;
#87636=CARTESIAN_POINT('Ctrl Pts',(-18.5120647055615,41.8228908067382,124.651624297318)) ;
#87637=CARTESIAN_POINT('Ctrl Pts',(-18.1453880278503,41.842670047979,124.274702004828)) ;
#87638=CARTESIAN_POINT('Ctrl Pts',(-17.9259851440591,41.8627001116879,123.789780611659)) ;
#87639=CARTESIAN_POINT('Ctrl Pts',(-17.8863697134436,41.8825823965899,123.262746959437)) ;
#87640=CARTESIAN_POINT('Ctrl Pts',(-18.0275326386484,41.9024646974829,122.753560552606)) ;
#87641=CARTESIAN_POINT('Ctrl Pts',(-18.3357088896958,41.9224478071012,122.320980688982)) ;
#87642=CARTESIAN_POINT('Ctrl Pts',(-18.7710306130654,41.9423382024791,122.02096992026)) ;
#87643=CARTESIAN_POINT('Ctrl Pts',(-19.2824613005974,41.9622349925134,121.886735352838)) ;
#87644=CARTESIAN_POINT('Ctrl Pts',(-19.8096884308124,41.982152046455,121.934563073507)) ;
#87645=CARTESIAN_POINT('Ctrl Pts',(-20.2909909356095,42.0021555946585,122.16058890975)) ;
#87646=CARTESIAN_POINT('Ctrl Pts',(-20.6644231854792,42.0220938883111,122.53654694601)) ;
#87647=CARTESIAN_POINT('Ctrl Pts',(-20.8870221312374,42.041915375744,123.014039318309)) ;
#87648=CARTESIAN_POINT('Ctrl Pts',(-20.9342135131919,42.0618937687349,123.542870872687)) ;
#87649=CARTESIAN_POINT('Ctrl Pts',(-20.7983116521925,42.0817921503486,124.05406099751)) ;
#87650=CARTESIAN_POINT('Ctrl Pts',(-20.5470876259133,42.0983750810785,124.416078628644)) ;
#87651=CARTESIAN_POINT('Ctrl Pts',(-20.2810340791425,42.1116493166673,124.641785333089)) ;
#87652=CARTESIAN_POINT('Ctrl Pts',(-20.0530711216127,42.1216957341235,124.774894284612)) ;
#87653=CARTESIAN_POINT('Ctrl Pts',(-19.8104700418555,42.1315409593428,124.864850290018)) ;
#87654=CARTESIAN_POINT('Ctrl Pts',(-19.4658985569829,42.1448759303822,124.928521275722)) ;
#87655=CARTESIAN_POINT('Ctrl Pts',(-19.0264447066916,42.1614587871748,124.893669283051)) ;
#87656=CARTESIAN_POINT('Ctrl Pts',(-18.6239261419113,42.1781017895242,124.710472536037)) ;
#87657=CARTESIAN_POINT('Ctrl Pts',(-18.3550087789404,42.1913455205559,124.489421557899)) ;
#87658=CARTESIAN_POINT('Ctrl Pts',(-18.1831612885463,42.2013999152305,124.288789628079)) ;
#87659=CARTESIAN_POINT('Ctrl Pts',(-18.0512749568523,42.2112409766191,124.066279127092)) ;
#87660=CARTESIAN_POINT('Ctrl Pts',(-17.9577303156056,42.2213072009756,123.818889092396)) ;
#87661=CARTESIAN_POINT('Ctrl Pts',(-17.9095286836072,42.2311878138952,123.563707583519)) ;
#87662=CARTESIAN_POINT('Ctrl Pts',(-17.9058337757334,42.2411811070548,123.301162738247)) ;
#87663=CARTESIAN_POINT('Ctrl Pts',(-17.9475195177784,42.2511321152785,123.042958068114)) ;
#87664=CARTESIAN_POINT('Ctrl Pts',(-18.0344126776209,42.2611806296404,122.793630948039)) ;
#87665=CARTESIAN_POINT('Ctrl Pts',(-18.1603920215042,42.2710221357031,122.56773601956)) ;
#87666=CARTESIAN_POINT('Ctrl Pts',(-18.3255845008848,42.2810077883328,122.363897258987)) ;
#87667=CARTESIAN_POINT('Ctrl Pts',(-18.5227313519484,42.2909467971777,122.192513006054)) ;
#87668=CARTESIAN_POINT('Ctrl Pts',(-18.7489176532003,42.3009877224707,122.056676120919)) ;
#87669=CARTESIAN_POINT('Ctrl Pts',(-18.9915477533087,42.3108780442256,121.96343274295)) ;
#87670=CARTESIAN_POINT('Ctrl Pts',(-19.2492897392915,42.320874017559,121.912831427002)) ;
#87671=CARTESIAN_POINT('Ctrl Pts',(-19.510238542724,42.3308054171411,121.90776329539)) ;
#87672=CARTESIAN_POINT('Ctrl Pts',(-19.7700878324599,42.3408109576181,121.948013744856)) ;
#87673=CARTESIAN_POINT('Ctrl Pts',(-20.0195067969403,42.3508439415494,122.033453514433)) ;
#87674=CARTESIAN_POINT('Ctrl Pts',(-20.2464693982846,42.3606995723763,122.158262805078)) ;
#87675=CARTESIAN_POINT('Ctrl Pts',(-20.4514198298294,42.3706989745694,122.322645616245)) ;
#87676=CARTESIAN_POINT('Ctrl Pts',(-20.6231827987995,42.3805934439305,122.517917638285)) ;
#87677=CARTESIAN_POINT('Ctrl Pts',(-20.7606195436203,42.3906565580947,122.743793366782)) ;
#87678=CARTESIAN_POINT('Ctrl Pts',(-20.8549120164977,42.4004962038111,122.984609559958)) ;
#87679=CARTESIAN_POINT('Ctrl Pts',(-20.9074321966083,42.4105593713669,123.243754099235)) ;
#87680=CARTESIAN_POINT('Ctrl Pts',(-20.9138270218801,42.4204536271617,123.503714919927)) ;
#87681=CARTESIAN_POINT('Ctrl Pts',(-20.8755128410189,42.4303954056214,123.762117252756)) ;
#87682=CARTESIAN_POINT('Ctrl Pts',(-20.7924756140901,42.4403980984516,124.011553585451)) ;
#87683=CARTESIAN_POINT('Ctrl Pts',(-20.6666672130897,42.4504321204054,124.243274149404)) ;
#87684=CARTESIAN_POINT('Ctrl Pts',(-20.5058796969663,42.4602799114944,124.446064360107)) ;
#87685=CARTESIAN_POINT('Ctrl Pts',(-20.3101026092512,42.4702614360435,124.62060077918)) ;
#87686=CARTESIAN_POINT('Ctrl Pts',(-20.0876687178098,42.4802106595344,124.758029297087)) ;
#87687=CARTESIAN_POINT('Ctrl Pts',(-19.8436792195384,42.490208315751,124.855531589647)) ;
#87688=CARTESIAN_POINT('Ctrl Pts',(-19.5853068270162,42.500248528806,124.908912389975)) ;
#87689=CARTESIAN_POINT('Ctrl Pts',(-19.3271481560831,42.5100765760823,124.917023207503)) ;
#87690=CARTESIAN_POINT('Ctrl Pts',(-19.065587620381,42.5201309231147,124.879749670527)) ;
#87691=CARTESIAN_POINT('Ctrl Pts',(-18.8174156782774,42.5300720594432,124.798125360101)) ;
#87692=CARTESIAN_POINT('Ctrl Pts',(-18.5876622498009,42.5399762925229,124.675821006536)) ;
#87693=CARTESIAN_POINT('Ctrl Pts',(-18.3798098223478,42.5500229893665,124.513062959193)) ;
#87694=CARTESIAN_POINT('Ctrl Pts',(-18.205809991047,42.5599185406468,124.319751471792)) ;
#87695=CARTESIAN_POINT('Ctrl Pts',(-18.0657424005529,42.5699806184863,124.095520805029)) ;
#87696=CARTESIAN_POINT('Ctrl Pts',(-17.9687323982393,42.5798233275824,123.855713961264)) ;
#87697=CARTESIAN_POINT('Ctrl Pts',(-17.9134293922222,42.5898140598208,123.599092869816)) ;
#87698=CARTESIAN_POINT('Ctrl Pts',(-17.9036266135817,42.5997420850496,123.338364905447)) ;
#87699=CARTESIAN_POINT('Ctrl Pts',(-17.9390160350888,42.6097302317001,123.078277461847)) ;
#87700=CARTESIAN_POINT('Ctrl Pts',(-18.0197861525379,42.6197652495401,122.827237976155)) ;
#87701=CARTESIAN_POINT('Ctrl Pts',(-18.140582591483,42.6296300466453,122.597876275323)) ;
#87702=CARTESIAN_POINT('Ctrl Pts',(-18.3003156640756,42.6395907790014,122.390498248251)) ;
#87703=CARTESIAN_POINT('Ctrl Pts',(-18.4953259743341,42.6496242413984,122.213054154998)) ;
#87704=CARTESIAN_POINT('Ctrl Pts',(-18.7147012146566,42.6595097756098,122.073852925735)) ;
#87705=CARTESIAN_POINT('Ctrl Pts',(-18.9592157983849,42.6695746162898,121.973094770652)) ;
#87706=CARTESIAN_POINT('Ctrl Pts',(-19.211976927808,42.6794227480187,121.917420334612)) ;
#87707=CARTESIAN_POINT('Ctrl Pts',(-19.4752162394926,42.6894502450088,121.905599515675)) ;
#87708=CARTESIAN_POINT('Ctrl Pts',(-19.7364643783176,42.6994786970539,121.940363154748)) ;
#87709=CARTESIAN_POINT('Ctrl Pts',(-19.983240895575,42.709323963618,122.018027966902)) ;
#87710=CARTESIAN_POINT('Ctrl Pts',(-20.2165165477863,42.7193146365589,122.138509322655)) ;
#87711=CARTESIAN_POINT('Ctrl Pts',(-20.42595149829,42.7293525186474,122.298877797518)) ;
#87712=CARTESIAN_POINT('Ctrl Pts',(-20.6012619502332,42.739196889087,122.489133616188)) ;
#87713=CARTESIAN_POINT('Ctrl Pts',(-20.7432777778674,42.7491817164824,122.709727782596)) ;
#87714=CARTESIAN_POINT('Ctrl Pts',(-20.8445084625415,42.7591211618877,122.950553007713)) ;
#87715=CARTESIAN_POINT('Ctrl Pts',(-20.902884175201,42.7691611661736,123.207827740318)) ;
#87716=CARTESIAN_POINT('Ctrl Pts',(-20.9156867364475,42.7790482753592,123.467365079687)) ;
#87717=CARTESIAN_POINT('Ctrl Pts',(-20.8831915581267,42.7890483352617,123.728098704159)) ;
#87718=CARTESIAN_POINT('Ctrl Pts',(-20.8067445599132,42.7989657511764,123.977299323762)) ;
#87719=CARTESIAN_POINT('Ctrl Pts',(-20.686612406926,42.8090125659172,124.212363180922)) ;
#87720=CARTESIAN_POINT('Ctrl Pts',(-20.5303690658562,42.8188880431139,124.419630089936)) ;
#87721=CARTESIAN_POINT('Ctrl Pts',(-20.337202917031,42.8289441388351,124.599902985176)) ;
#87722=CARTESIAN_POINT('Ctrl Pts',(-20.1192329290402,42.8388373008502,124.741697871364)) ;
#87723=CARTESIAN_POINT('Ctrl Pts',(-19.8759728300273,42.8488995368728,124.845270931614)) ;
#87724=CARTESIAN_POINT('Ctrl Pts',(-19.6239615863206,42.8587440025017,124.903774649878)) ;
#87725=CARTESIAN_POINT('Ctrl Pts',(-19.3626527477167,42.8687040952058,124.91873716026)) ;
#87726=CARTESIAN_POINT('Ctrl Pts',(-19.1007442432168,42.8787423841869,124.887345479684)) ;
#87727=CARTESIAN_POINT('Ctrl Pts',(-18.852219395114,42.8886157072931,124.812672988231)) ;
#87728=CARTESIAN_POINT('Ctrl Pts',(-18.6158652448163,42.8986888913782,124.693587821864)) ;
#87729=CARTESIAN_POINT('Ctrl Pts',(-18.408809846254,42.9085094036661,124.539447907291)) ;
#87730=CARTESIAN_POINT('Ctrl Pts',(-18.2269164681603,42.9185873997819,124.347038540938)) ;
#87731=CARTESIAN_POINT('Ctrl Pts',(-18.0843140642102,42.9284414747652,124.130813462835)) ;
#87732=CARTESIAN_POINT('Ctrl Pts',(-17.9790106190544,42.9385053563489,123.888269164773)) ;
#87733=CARTESIAN_POINT('Ctrl Pts',(-17.9185491680014,42.9483887823227,123.635632007947)) ;
#87734=CARTESIAN_POINT('Ctrl Pts',(-17.9022737750403,42.9583893862437,123.373377146627)) ;
#87735=CARTESIAN_POINT('Ctrl Pts',(-17.9313895259165,42.9683091705816,123.114278441424)) ;
#87736=CARTESIAN_POINT('Ctrl Pts',(-18.0060320164047,42.9783565209384,122.861060709944)) ;
#87737=CARTESIAN_POINT('Ctrl Pts',(-18.1212870190588,42.9882338631727,122.628427841327)) ;
#87738=CARTESIAN_POINT('Ctrl Pts',(-18.2781351229889,42.9983037442474,122.415360927794)) ;
#87739=CARTESIAN_POINT('Ctrl Pts',(-18.4649150055318,43.008133449449,122.2368543242)) ;
#87740=CARTESIAN_POINT('Ctrl Pts',(-18.6847596765535,43.0182001106154,122.089792158768)) ;
#87741=CARTESIAN_POINT('Ctrl Pts',(-18.9226931773935,43.0280903324827,121.985125306975)) ;
#87742=CARTESIAN_POINT('Ctrl Pts',(-19.1776048761138,43.0380825085929,121.922176627254)) ;
#87743=CARTESIAN_POINT('Ctrl Pts',(-19.4388303799402,43.0480453387055,121.904745061404)) ;
#87744=CARTESIAN_POINT('Ctrl Pts',(-19.697682792419,43.0579495511058,121.932114404861)) ;
#87745=CARTESIAN_POINT('Ctrl Pts',(-19.951683312586,43.0680102651937,122.005359612903)) ;
#87746=CARTESIAN_POINT('Ctrl Pts',(-20.1841105631504,43.0778497681765,122.118753970002)) ;
#87747=CARTESIAN_POINT('Ctrl Pts',(-20.3982269814349,43.0879159067429,122.274016136349)) ;
#87748=CARTESIAN_POINT('Ctrl Pts',(-20.5787646114016,43.0977984212289,122.460756397599)) ;
#87749=CARTESIAN_POINT('Ctrl Pts',(-20.7261333194938,43.1077907205845,122.678042925821)) ;
#87750=CARTESIAN_POINT('Ctrl Pts',(-20.833206366185,43.1177437875379,122.916721805344)) ;
#87751=CARTESIAN_POINT('Ctrl Pts',(-20.897614117175,43.1277784957431,123.172416207021)) ;
#87752=CARTESIAN_POINT('Ctrl Pts',(-20.9165610195701,43.1376667166473,123.43159275742)) ;
#87753=CARTESIAN_POINT('Ctrl Pts',(-20.8903677843384,43.1476611396777,123.692911928234)) ;
#87754=CARTESIAN_POINT('Ctrl Pts',(-20.8194444690435,43.1576064791239,123.944458675462)) ;
#87755=CARTESIAN_POINT('Ctrl Pts',(-20.7063781227187,43.1675538237352,124.180161559428)) ;
#87756=CARTESIAN_POINT('Ctrl Pts',(-20.5523346077461,43.1776017191462,124.394608128497)) ;
#87757=CARTESIAN_POINT('Ctrl Pts',(-20.3673072274807,43.1874493646256,124.575539263631)) ;
#87758=CARTESIAN_POINT('Ctrl Pts',(-20.1516760965307,43.1974110785396,124.723955111939)) ;
#87759=CARTESIAN_POINT('Ctrl Pts',(-19.9117864879595,43.2074397028305,124.833114513842)) ;
#87760=CARTESIAN_POINT('Ctrl Pts',(-19.6596450451628,43.2173500634872,124.898260239512)) ;
#87761=CARTESIAN_POINT('Ctrl Pts',(-19.3994169455173,43.2272847620605,124.919374953537)) ;
#87762=CARTESIAN_POINT('Ctrl Pts',(-19.1367199893783,43.2373265869147,124.894463864514)) ;
#87763=CARTESIAN_POINT('Ctrl Pts',(-18.886225085537,43.2472111606591,124.825627198555)) ;
#87764=CARTESIAN_POINT('Ctrl Pts',(-18.6486227140851,43.2572130100223,124.713331619215)) ;
#87765=CARTESIAN_POINT('Ctrl Pts',(-18.4357298701924,43.2671323115963,124.562855492148)) ;
#87766=CARTESIAN_POINT('Ctrl Pts',(-18.2499252216547,43.2771764199416,124.375414816484)) ;
#87767=CARTESIAN_POINT('Ctrl Pts',(-18.1017967666107,43.2870608433839,124.162024125329)) ;
#87768=CARTESIAN_POINT('Ctrl Pts',(-17.9909876140739,43.2970772052933,123.923254596581)) ;
#87769=CARTESIAN_POINT('Ctrl Pts',(-17.923859840719,43.3071138607987,123.668202194077)) ;
#87770=CARTESIAN_POINT('Ctrl Pts',(-17.9017809512743,43.316943990988,123.410789908408)) ;
#87771=CARTESIAN_POINT('Ctrl Pts',(-17.9252094807461,43.3270200440779,123.14709156434)) ;
#87772=CARTESIAN_POINT('Ctrl Pts',(-17.9924299188192,43.3368722732637,122.897006470178)) ;
#87773=CARTESIAN_POINT('Ctrl Pts',(-18.1042679823455,43.346945481063,122.657125718903)) ;
#87774=CARTESIAN_POINT('Ctrl Pts',(-18.2526600247285,43.3567869924144,122.445286955059)) ;
#87775=CARTESIAN_POINT('Ctrl Pts',(-18.4370833480714,43.3667479304519,122.259535607649)) ;
#87776=CARTESIAN_POINT('Ctrl Pts',(-18.6529137116503,43.3767857923769,122.107894632329)) ;
#87777=CARTESIAN_POINT('Ctrl Pts',(-18.8877318802292,43.386659978374,121.997399835187)) ;
#87778=CARTESIAN_POINT('Ctrl Pts',(-19.1430767424442,43.3967301379519,121.928047356041)) ;
#87779=CARTESIAN_POINT('Ctrl Pts',(-19.4003939023348,43.4065618853777,121.904482946936)) ;
#87780=CARTESIAN_POINT('Ctrl Pts',(-19.6632619536359,43.416597965449,121.925714449018)) ;
#87781=CARTESIAN_POINT('Ctrl Pts',(-19.9178244791952,43.4266150123015,121.992789588399)) ;
#87782=CARTESIAN_POINT('Ctrl Pts',(-20.1538536760543,43.4364972704681,122.101114447307)) ;
#87783=CARTESIAN_POINT('Ctrl Pts',(-20.3699131764678,43.4464849532645,122.250085365114)) ;
#87784=CARTESIAN_POINT('Ctrl Pts',(-20.5562534234135,43.4564316099812,122.433448480984)) ;
#87785=CARTESIAN_POINT('Ctrl Pts',(-20.7093464656126,43.4664886680613,122.648845014339)) ;
#87786=CARTESIAN_POINT('Ctrl Pts',(-20.8203630654668,43.4763068476108,122.881767028925)) ;
#87787=CARTESIAN_POINT('Ctrl Pts',(-20.8914610512173,43.4863427820498,123.135729585425)) ;
#87788=CARTESIAN_POINT('Ctrl Pts',(-20.9166029199042,43.4963674364788,123.397974203455)) ;
#87789=CARTESIAN_POINT('Ctrl Pts',(-20.8967578932332,43.5062194560583,123.656117782256)) ;
#87790=CARTESIAN_POINT('Ctrl Pts',(-20.831881508292,43.5162103697732,123.910494310723)) ;
#87791=CARTESIAN_POINT('Ctrl Pts',(-20.7247399963963,43.5261283586128,124.148122891889)) ;
#87792=CARTESIAN_POINT('Ctrl Pts',(-20.5764179652717,43.5361564693436,124.365922998669)) ;
#87793=CARTESIAN_POINT('Ctrl Pts',(-20.3952122093275,43.546041667252,124.552066450949)) ;
#87794=CARTESIAN_POINT('Ctrl Pts',(-20.1825938294097,43.55603094252,124.706038954203)) ;
#87795=CARTESIAN_POINT('Ctrl Pts',(-19.9449996926765,43.5660724006895,124.820834858962)) ;
#87796=CARTESIAN_POINT('Ctrl Pts',(-19.6965069343808,43.5759038644778,124.89159240592)) ;
#87797=CARTESIAN_POINT('Ctrl Pts',(-19.4350698137697,43.5859087967817,124.919173839307)) ;
#87798=CARTESIAN_POINT('Ctrl Pts',(-19.1732351295058,43.5958951606764,124.900827612683)) ;
#87799=CARTESIAN_POINT('Ctrl Pts',(-18.9175770787377,43.6059247895623,124.836838031948)) ;
#87800=CARTESIAN_POINT('Ctrl Pts',(-18.6804371598066,43.6158000116707,124.731369996855)) ;
#87801=CARTESIAN_POINT('Ctrl Pts',(-18.4623477415022,43.6258012240678,124.584774106996)) ;
#87802=CARTESIAN_POINT('Ctrl Pts',(-18.2745444168899,43.6357098033033,124.404343207406)) ;
#87803=CARTESIAN_POINT('Ctrl Pts',(-18.1187722259552,43.6457646558593,124.190964881095)) ;
#87804=CARTESIAN_POINT('Ctrl Pts',(-18.004380821327,43.6556232381341,123.958462580893)) ;
#87805=CARTESIAN_POINT('Ctrl Pts',(-17.9304301319305,43.6656913675768,123.704467954817)) ;
#87806=CARTESIAN_POINT('Ctrl Pts',(-17.9023257120292,43.6755468392659,123.446983659363)) ;
#87807=CARTESIAN_POINT('Ctrl Pts',(-17.9188088681527,43.6855416876521,123.18485588981)) ;
#87808=CARTESIAN_POINT('Ctrl Pts',(-17.9813360998204,43.6955729844366,122.928761468334)) ;
#87809=CARTESIAN_POINT('Ctrl Pts',(-18.0852611565216,43.7054395206467,122.691208548975)) ;
#87810=CARTESIAN_POINT('Ctrl Pts',(-18.2302389701534,43.7154269436075,122.472461402679)) ;
#87811=CARTESIAN_POINT('Ctrl Pts',(-18.4101746479847,43.7253718826273,122.282878179321)) ;
#87812=CARTESIAN_POINT('Ctrl Pts',(-18.6224381752842,43.7354167684873,122.125988815331)) ;
#87813=CARTESIAN_POINT('Ctrl Pts',(-18.8545304610227,43.7452853035735,122.010266829846)) ;
#87814=CARTESIAN_POINT('Ctrl Pts',(-19.1054170228572,43.7552511715802,121.935180988231)) ;
#87815=CARTESIAN_POINT('Ctrl Pts',(-19.3670753403128,43.7652738190327,121.904915997745)) ;
#87816=CARTESIAN_POINT('Ctrl Pts',(-19.6273895696262,43.7751974580403,121.920314786866)) ;
#87817=CARTESIAN_POINT('Ctrl Pts',(-19.8817360875412,43.785140183046,121.980191368914)) ;
#87818=CARTESIAN_POINT('Ctrl Pts',(-20.1241540955357,43.7951857890979,122.084667591629)) ;
#87819=CARTESIAN_POINT('Ctrl Pts',(-20.3408919295591,43.805047211619,122.226772581987)) ;
#87820=CARTESIAN_POINT('Ctrl Pts',(-20.5324564346371,43.8150407800682,122.406363357882)) ;
#87821=CARTESIAN_POINT('Ctrl Pts',(-20.6890092975618,43.8249662508235,122.615035530979)) ;
#87822=CARTESIAN_POINT('Ctrl Pts',(-20.8081450016785,43.8349939247794,122.850047539463)) ;
#87823=CARTESIAN_POINT('Ctrl Pts',(-20.8838536120231,43.8448811028211,123.098633773252)) ;
#87824=CARTESIAN_POINT('Ctrl Pts',(-20.9158727010176,43.8549094821892,123.360180929265)) ;
#87825=CARTESIAN_POINT('Ctrl Pts',(-20.9023154130468,43.8648037249107,123.61987110098)) ;
#87826=CARTESIAN_POINT('Ctrl Pts',(-20.8237526627658,43.8781566415616,123.961832644244)) ;
#87827=CARTESIAN_POINT('Ctrl Pts',(-20.659605419344,43.8913591593083,124.272026060151)) ;
#87828=CARTESIAN_POINT('Ctrl Pts',(-20.4209894341323,43.9047150645893,124.529371523142)) ;
#87829=CARTESIAN_POINT('Ctrl Pts',(-20.2138465893309,43.9146117132271,124.686685290461)) ;
#87830=CARTESIAN_POINT('Ctrl Pts',(-19.9790841361338,43.9246598512796,124.807515218539)) ;
#87831=CARTESIAN_POINT('Ctrl Pts',(-19.7308190710791,43.9345508114574,124.884524562432)) ;
#87832=CARTESIAN_POINT('Ctrl Pts',(-19.4703839376697,43.9445436473341,124.918248825918)) ;
#87833=CARTESIAN_POINT('Ctrl Pts',(-19.2068845324014,43.9545827423357,124.905579235426)) ;
#87834=CARTESIAN_POINT('Ctrl Pts',(-18.9545857300593,43.9644200981869,124.849099649171)) ;
#87835=CARTESIAN_POINT('Ctrl Pts',(-18.6296690897415,43.9778130461176,124.713956490856)) ;
#87836=CARTESIAN_POINT('Ctrl Pts',(-18.3520981743961,43.9909797225445,124.500694921199)) ;
#87837=CARTESIAN_POINT('Ctrl Pts',(-18.1378620138643,44.0043645039513,124.221797775786)) ;
#87838=CARTESIAN_POINT('Ctrl Pts',(-18.0179672616378,44.0142262865952,123.991995123024)) ;
#87839=CARTESIAN_POINT('Ctrl Pts',(-17.9383259095293,44.0242254345482,123.741642443432)) ;
#87840=CARTESIAN_POINT('Ctrl Pts',(-17.9034476011342,44.0341282271653,123.483699776961)) ;
#87841=CARTESIAN_POINT('Ctrl Pts',(-17.9141092543276,44.0441778070562,123.219886940427)) ;
#87842=CARTESIAN_POINT('Ctrl Pts',(-17.987359893705,44.0573648808657,122.881047522662)) ;
#87843=CARTESIAN_POINT('Ctrl Pts',(-18.1910325351083,44.0741176708369,122.485294726917)) ;
#87844=CARTESIAN_POINT('Ctrl Pts',(-18.5127079665964,44.0906063229316,122.187409946864)) ;
#87845=CARTESIAN_POINT('Ctrl Pts',(-18.8227881728284,44.103963149115,122.02310778574)) ;
#87846=CARTESIAN_POINT('Ctrl Pts',(-19.0702563997621,44.1138595339929,121.942965399191)) ;
#87847=CARTESIAN_POINT('Ctrl Pts',(-19.3306048043616,44.1238660485134,121.906491121348)) ;
#87848=CARTESIAN_POINT('Ctrl Pts',(-19.6771635039031,44.1370561720298,121.917876124668)) ;
#87849=CARTESIAN_POINT('Ctrl Pts',(-20.1033013954012,44.1538227331793,122.047686667172)) ;
#87850=CARTESIAN_POINT('Ctrl Pts',(-20.5238929989773,44.1736072218874,122.363542810504)) ;
#87851=CARTESIAN_POINT('Ctrl Pts',(-20.815011621917,44.1935526694839,122.806412748844)) ;
#87852=CARTESIAN_POINT('Ctrl Pts',(-20.9368621718498,44.2134643316398,123.321424916447)) ;
#87853=CARTESIAN_POINT('Ctrl Pts',(-20.8768657552607,44.2333565236587,123.846793390736)) ;
#87854=CARTESIAN_POINT('Ctrl Pts',(-20.6387805843268,44.2533976542133,124.323200523711)) ;
#87855=CARTESIAN_POINT('Ctrl Pts',(-20.2567572002547,44.2732159888289,124.686031568202)) ;
#87856=CARTESIAN_POINT('Ctrl Pts',(-19.7707167595738,44.2931885540485,124.899018477373)) ;
#87857=CARTESIAN_POINT('Ctrl Pts',(-19.243012073421,44.3130777702201,124.933377526462)) ;
#87858=CARTESIAN_POINT('Ctrl Pts',(-18.7322499924567,44.3331013445428,124.784342715249)) ;
#87859=CARTESIAN_POINT('Ctrl Pts',(-18.3074523247711,44.352898507631,124.473689351128)) ;
#87860=CARTESIAN_POINT('Ctrl Pts',(-18.0107208479656,44.3728640014548,124.033892370887)) ;
#87861=CARTESIAN_POINT('Ctrl Pts',(-17.8825301084476,44.3928177091962,123.519135613177)) ;
#87862=CARTESIAN_POINT('Ctrl Pts',(-17.9375131053142,44.4127250859228,122.993014954846)) ;
#87863=CARTESIAN_POINT('Ctrl Pts',(-18.1669119070672,44.4325772974714,122.517754743088)) ;
#87864=CARTESIAN_POINT('Ctrl Pts',(-18.5491999521954,44.4526496844171,122.145668046979)) ;
#87865=CARTESIAN_POINT('Ctrl Pts',(-19.0301389700753,44.4724875540574,121.9295612266)) ;
#87866=CARTESIAN_POINT('Ctrl Pts',(-19.556112431027,44.4923382086105,121.888236492257)) ;
#87867=CARTESIAN_POINT('Ctrl Pts',(-20.0695268056747,44.512390142951,122.031046366895)) ;
#87868=CARTESIAN_POINT('Ctrl Pts',(-20.4987446170897,44.532223330517,122.337261350157)) ;
#87869=CARTESIAN_POINT('Ctrl Pts',(-20.7998380093603,44.5521525427477,122.772809047979)) ;
#87870=CARTESIAN_POINT('Ctrl Pts',(-20.9346380609838,44.5720375079621,123.284047944812)) ;
#87871=CARTESIAN_POINT('Ctrl Pts',(-20.8856425940297,44.5921112491067,123.815212598448)) ;
#87872=CARTESIAN_POINT('Ctrl Pts',(-20.6614851629729,44.6119044308871,124.291227274791)) ;
#87873=CARTESIAN_POINT('Ctrl Pts',(-20.2863772074548,44.6318671388898,124.666405427892)) ;
#87874=CARTESIAN_POINT('Ctrl Pts',(-19.8046798286043,44.6518500906322,124.8901432235)) ;
#87875=CARTESIAN_POINT('Ctrl Pts',(-19.2801648941078,44.6716607104044,124.936716143029)) ;
#87876=CARTESIAN_POINT('Ctrl Pts',(-18.7667918531497,44.6916444264373,124.800971420717)) ;
#87877=CARTESIAN_POINT('Ctrl Pts',(-18.332633623527,44.7115258903346,124.499523849295)) ;
#87878=CARTESIAN_POINT('Ctrl Pts',(-18.0261041134591,44.731481220179,124.066823654643)) ;
#87879=CARTESIAN_POINT('Ctrl Pts',(-17.8857718639008,44.7513566809845,123.557460531844)) ;
#87880=CARTESIAN_POINT('Ctrl Pts',(-17.9275871464799,44.771341001036,123.028016369146)) ;
#87881=CARTESIAN_POINT('Ctrl Pts',(-18.1472823916272,44.7912690338256,122.54594681577)) ;
#87882=CARTESIAN_POINT('Ctrl Pts',(-18.4563072638141,44.8078777957654,122.230852995871)) ;
#87883=CARTESIAN_POINT('Ctrl Pts',(-18.7544344166136,44.8210654344555,122.054104346629)) ;
#87884=CARTESIAN_POINT('Ctrl Pts',(-18.9997577413404,44.8310518688156,121.960933276629)) ;
#87885=CARTESIAN_POINT('Ctrl Pts',(-19.2582000487417,44.841061242775,121.911919172374)) ;
#87886=CARTESIAN_POINT('Ctrl Pts',(-19.6074259157018,44.8543512763403,121.90718231146)) ;
#87887=CARTESIAN_POINT('Ctrl Pts',(-20.0350744145889,44.8709452640027,122.015110092288)) ;
#87888=CARTESIAN_POINT('Ctrl Pts',(-20.4010334172279,44.8875775192782,122.263044894367)) ;
#87889=CARTESIAN_POINT('Ctrl Pts',(-20.6289076195677,44.9008199029461,122.52606867887)) ;
#87890=CARTESIAN_POINT('Ctrl Pts',(-20.7634193394176,44.9107341111735,122.749205301052)) ;
#87891=CARTESIAN_POINT('Ctrl Pts',(-20.8581992855926,44.9207907504452,122.995881649194)) ;
#87892=CARTESIAN_POINT('Ctrl Pts',(-20.9079626866539,44.9306365568653,123.249811042525)) ;
#87893=CARTESIAN_POINT('Ctrl Pts',(-20.9134321153544,44.9406815564985,123.513714183674)) ;
#87894=CARTESIAN_POINT('Ctrl Pts',(-20.8594529735354,44.9539625788713,123.85851431483)) ;
#87895=CARTESIAN_POINT('Ctrl Pts',(-20.7185138341195,44.9671600253959,124.179729076087)) ;
#87896=CARTESIAN_POINT('Ctrl Pts',(-20.4978542341181,44.9805743232029,124.454653630732)) ;
#87897=CARTESIAN_POINT('Ctrl Pts',(-20.3035482186063,44.9904133886056,124.625258093541)) ;
#87898=CARTESIAN_POINT('Ctrl Pts',(-20.0797292255048,45.0003965948833,124.762068121514)) ;
#87899=CARTESIAN_POINT('Ctrl Pts',(-19.8362653995539,45.0103478297961,124.857563683997)) ;
#87900=CARTESIAN_POINT('Ctrl Pts',(-19.5787021577369,45.0203488294977,124.90990497468)) ;
#87901=CARTESIAN_POINT('Ctrl Pts',(-19.3151704808666,45.0303801752851,124.916336383632)) ;
#87902=CARTESIAN_POINT('Ctrl Pts',(-19.059076565559,45.0402339399901,124.877961736359)) ;
#87903=CARTESIAN_POINT('Ctrl Pts',(-18.8104579041759,45.0502045936584,124.795331193507)) ;
#87904=CARTESIAN_POINT('Ctrl Pts',(-18.5792936637788,45.0602018373156,124.670414452979)) ;
#87905=CARTESIAN_POINT('Ctrl Pts',(-18.372843216216,45.0702352932598,124.506439042019)) ;
#87906=CARTESIAN_POINT('Ctrl Pts',(-18.2007560512662,45.0800907975602,124.312851502277)) ;
#87907=CARTESIAN_POINT('Ctrl Pts',(-18.0626513107753,45.0900902338463,124.08934966355)) ;
#87908=CARTESIAN_POINT('Ctrl Pts',(-17.966160872868,45.0999846933622,123.847847223486)) ;
#87909=CARTESIAN_POINT('Ctrl Pts',(-17.9122601551696,45.1100478128138,123.588997131048)) ;
#87910=CARTESIAN_POINT('Ctrl Pts',(-17.9040157128179,45.1198874472258,123.330510182851)) ;
#87911=CARTESIAN_POINT('Ctrl Pts',(-17.9412701233928,45.1299506547116,123.068734224408)) ;
#87912=CARTESIAN_POINT('Ctrl Pts',(-18.0222577929814,45.1398447620908,122.821630638561)) ;
#87913=CARTESIAN_POINT('Ctrl Pts',(-18.1448705736183,45.1497870942832,122.590953885684)) ;
#87914=CARTESIAN_POINT('Ctrl Pts',(-18.3065622324811,45.1597877205982,122.383723321206)) ;
#87915=CARTESIAN_POINT('Ctrl Pts',(-18.502862990913,45.1698294548801,122.207402005079)) ;
#87916=CARTESIAN_POINT('Ctrl Pts',(-18.7217059912546,45.1796548808292,122.070339801105)) ;
#87917=CARTESIAN_POINT('Ctrl Pts',(-18.966474765151,45.1897117073569,121.970725354272)) ;
#87918=CARTESIAN_POINT('Ctrl Pts',(-19.2216074988033,45.1996391404784,121.916190939513)) ;
#87919=CARTESIAN_POINT('Ctrl Pts',(-19.4828944941186,45.2095891328847,121.906015436364)) ;
#87920=CARTESIAN_POINT('Ctrl Pts',(-19.7446272926651,45.2196443339587,121.942195083293)) ;
#87921=CARTESIAN_POINT('Ctrl Pts',(-19.9904565700812,45.229466608011,122.020960921677)) ;
#87922=CARTESIAN_POINT('Ctrl Pts',(-20.2244926759389,45.2395225019702,122.143638300963)) ;
#87923=CARTESIAN_POINT('Ctrl Pts',(-20.4310152546762,45.2494632238153,122.303624668569)) ;
#87924=CARTESIAN_POINT('Ctrl Pts',(-20.6065787562621,45.2593675679019,122.495779589979)) ;
#87925=CARTESIAN_POINT('Ctrl Pts',(-20.7479598031112,45.2694142352014,122.718723494218)) ;
#87926=CARTESIAN_POINT('Ctrl Pts',(-20.847214873449,45.2793097936513,122.959126759267)) ;
#87927=CARTESIAN_POINT('Ctrl Pts',(-20.9041452558885,45.289371872356,123.217307547921)) ;
#87928=CARTESIAN_POINT('Ctrl Pts',(-20.9152880545128,45.2992145708218,123.475752573775)) ;
#87929=CARTESIAN_POINT('Ctrl Pts',(-20.8815017658848,45.3092053447163,123.736083691839)) ;
#87930=CARTESIAN_POINT('Ctrl Pts',(-20.803464341165,45.3191332139512,123.985045208885)) ;
#87931=CARTESIAN_POINT('Ctrl Pts',(-20.6830597025419,45.329121942921,124.218310172985)) ;
#87932=CARTESIAN_POINT('Ctrl Pts',(-20.5228027489551,45.3391613449048,124.427867674991)) ;
#87933=CARTESIAN_POINT('Ctrl Pts',(-20.3327730605954,45.3490015126416,124.603267061586)) ;
#87934=CARTESIAN_POINT('Ctrl Pts',(-20.1108060666027,45.3590497230161,124.746272176201)) ;
#87935=CARTESIAN_POINT('Ctrl Pts',(-19.8696532867426,45.3689968933038,124.847160076547)) ;
#87936=CARTESIAN_POINT('Ctrl Pts',(-19.6157459454995,45.3789077415589,124.90519559881)) ;
#87937=CARTESIAN_POINT('Ctrl Pts',(-19.3518125734357,45.3889640692367,124.918205064877)) ;
#87938=CARTESIAN_POINT('Ctrl Pts',(-19.0949419766038,45.3988144820052,124.886084607511)) ;
#87939=CARTESIAN_POINT('Ctrl Pts',(-18.8429458077784,45.4088413678389,124.809102515911)) ;
#87940=CARTESIAN_POINT('Ctrl Pts',(-18.6084007715185,45.4188699834697,124.688897924885)) ;
#87941=CARTESIAN_POINT('Ctrl Pts',(-18.4018578835291,45.4287152068472,124.533108889477)) ;
#87942=CARTESIAN_POINT('Ctrl Pts',(-18.2223677576914,45.4387058889488,124.341493091567)) ;
#87943=CARTESIAN_POINT('Ctrl Pts',(-18.0786949591788,45.4487437775813,124.120270887316)) ;
#87944=CARTESIAN_POINT('Ctrl Pts',(-17.9771820255855,45.4585881126844,123.882309246234)) ;
#87945=CARTESIAN_POINT('Ctrl Pts',(-17.9171992662685,45.4685730748819,123.62689961788)) ;
#87946=CARTESIAN_POINT('Ctrl Pts',(-17.9024172623288,45.4785120164153,123.366094931073)) ;
#87947=CARTESIAN_POINT('Ctrl Pts',(-17.9335377045302,45.4885539013867,123.104071689988)) ;
#87948=CARTESIAN_POINT('Ctrl Pts',(-18.0083583615695,45.498440449295,122.855243316233)) ;
#87949=CARTESIAN_POINT('Ctrl Pts',(-18.1261441567159,45.508434374795,122.620545045069)) ;
#87950=CARTESIAN_POINT('Ctrl Pts',(-18.2819302055561,45.5183704659215,122.410950315548)) ;
#87951=CARTESIAN_POINT('Ctrl Pts',(-18.4735027254418,45.5283997349014,122.229995789476)) ;
#87952=CARTESIAN_POINT('Ctrl Pts',(-18.690241481066,45.5382821174607,122.086859617476)) ;
#87953=CARTESIAN_POINT('Ctrl Pts',(-18.9325349471609,45.5483346345486,121.981703543276)) ;
#87954=CARTESIAN_POINT('Ctrl Pts',(-19.185413729496,45.5582287553725,121.921034104185)) ;
#87955=CARTESIAN_POINT('Ctrl Pts',(-19.4493049697019,45.5682907347929,121.904866941073)) ;
#87956=CARTESIAN_POINT('Ctrl Pts',(-19.7063630081236,45.5781352680218,121.934093132553)) ;
#87957=CARTESIAN_POINT('Ctrl Pts',(-19.9576058706028,45.5880953469281,122.007462571973)) ;
#87958=CARTESIAN_POINT('Ctrl Pts',(-20.1938981415272,45.5981336235007,122.124711964626)) ;
#87959=CARTESIAN_POINT('Ctrl Pts',(-20.4030909048024,45.6080070100386,122.278267729606)) ;
#87960=CARTESIAN_POINT('Ctrl Pts',(-20.5859499300167,45.6180799528056,122.469592306891)) ;
#87961=CARTESIAN_POINT('Ctrl Pts',(-20.7294620067179,45.6279013669339,122.684171707813)) ;
#87962=CARTESIAN_POINT('Ctrl Pts',(-20.836469961144,45.6379759970062,122.92628036698)) ;
#87963=CARTESIAN_POINT('Ctrl Pts',(-20.8984204591589,45.6478426343231,123.178089581566)) ;
#87964=CARTESIAN_POINT('Ctrl Pts',(-20.9166539511471,45.6578661796949,123.440853736035)) ;
#87965=CARTESIAN_POINT('Ctrl Pts',(-20.8883451902421,45.6678919312121,123.702810647261)) ;
#87966=CARTESIAN_POINT('Ctrl Pts',(-20.8166655858108,45.6777455182215,123.951620064222)) ;
#87967=CARTESIAN_POINT('Ctrl Pts',(-20.7020665615135,45.6877224784494,124.187438612339)) ;
#87968=CARTESIAN_POINT('Ctrl Pts',(-20.5472320226334,45.6977436214779,124.400440473039)) ;
#87969=CARTESIAN_POINT('Ctrl Pts',(-20.3607129644231,45.7076262274978,124.581203675269)) ;
#87970=CARTESIAN_POINT('Ctrl Pts',(-20.1416041543845,45.7176946981305,124.729442692636)) ;
#87971=CARTESIAN_POINT('Ctrl Pts',(-19.9058440233542,45.7275247813142,124.835139992)) ;
#87972=CARTESIAN_POINT('Ctrl Pts',(-19.6494558792354,45.7375913409946,124.900127141566)) ;
#87973=CARTESIAN_POINT('Ctrl Pts',(-19.3902123872049,45.7474815908238,124.919112847795)) ;
#87974=CARTESIAN_POINT('Ctrl Pts',(-19.1289348372093,45.7574737565726,124.893103063459)) ;
#87975=CARTESIAN_POINT('Ctrl Pts',(-18.8769434953996,45.7674366001687,124.822088336448)) ;
#87976=CARTESIAN_POINT('Ctrl Pts',(-18.6421852615433,45.7773407689965,124.709652708434)) ;
#87977=CARTESIAN_POINT('Ctrl Pts',(-18.4273528974957,45.7874016438908,124.555606852268)) ;
#87978=CARTESIAN_POINT('Ctrl Pts',(-18.2462968796542,45.7972405472202,124.370967398921)) ;
#87979=CARTESIAN_POINT('Ctrl Pts',(-18.0964786782735,45.8073089235941,124.152936536302)) ;
#87980=CARTESIAN_POINT('Ctrl Pts',(-17.9888851621427,45.8171895402267,123.916582846629)) ;
#87981=CARTESIAN_POINT('Ctrl Pts',(-17.9227453188288,45.8271807004557,123.662532284139)) ;
#87982=CARTESIAN_POINT('Ctrl Pts',(-17.9017535244661,45.8371337738878,123.401780145108)) ;
#87983=CARTESIAN_POINT('Ctrl Pts',(-17.9266404178476,45.8471696095005,123.139247618234)) ;
#87984=CARTESIAN_POINT('Ctrl Pts',(-17.9955552265189,45.8570597362306,122.888631027566)) ;
#87985=CARTESIAN_POINT('Ctrl Pts',(-18.1076934818933,45.8670519179999,122.651211136144)) ;
#87986=CARTESIAN_POINT('Ctrl Pts',(-18.2587304245374,45.8769978579744,122.437900289644)) ;
#87987=CARTESIAN_POINT('Ctrl Pts',(-18.4441704878577,45.8869450417339,122.253645296691)) ;
#87988=CARTESIAN_POINT('Ctrl Pts',(-18.6611101574099,45.8969929800242,122.103131587065)) ;
#87989=CARTESIAN_POINT('Ctrl Pts',(-18.8960272898149,45.9068406148377,121.994572618097)) ;
#87990=CARTESIAN_POINT('Ctrl Pts',(-19.148898873225,45.9168023285357,121.926896838604)) ;
#87991=CARTESIAN_POINT('Ctrl Pts',(-19.4114894160667,45.9268309643569,121.904333417555)) ;
#87992=CARTESIAN_POINT('Ctrl Pts',(-19.6708912056313,45.9367412791087,121.92734461787)) ;
#87993=CARTESIAN_POINT('Ctrl Pts',(-19.9231784918885,45.9466761497713,121.994557839022)) ;
#87994=CARTESIAN_POINT('Ctrl Pts',(-20.1623713001247,45.9567173321731,122.10595274913)) ;
#87995=CARTESIAN_POINT('Ctrl Pts',(-20.3754171966407,45.9666043036378,122.254712550326)) ;
#87996=CARTESIAN_POINT('Ctrl Pts',(-20.5616853384859,45.9766037359004,122.440014625736)) ;
#87997=CARTESIAN_POINT('Ctrl Pts',(-20.7119304588546,45.986523801157,122.65309125952)) ;
#87998=CARTESIAN_POINT('Ctrl Pts',(-20.8242304858689,45.9965606537412,122.891731631287)) ;
#87999=CARTESIAN_POINT('Ctrl Pts',(-20.8925312466949,46.0064733130812,123.143117767075)) ;
#88000=CARTESIAN_POINT('Ctrl Pts',(-20.9169022735991,46.0164645249961,123.404558617935)) ;
#88001=CARTESIAN_POINT('Ctrl Pts',(-20.8948119575861,46.0265061663992,123.667495012575)) ;
#88002=CARTESIAN_POINT('Ctrl Pts',(-20.8294454785966,46.0363349606062,123.917414465479)) ;
#88003=CARTESIAN_POINT('Ctrl Pts',(-20.7191022663443,46.0464113717275,124.158067817818)) ;
#88004=CARTESIAN_POINT('Ctrl Pts',(-20.5720475565284,46.05626350477,124.371223090758)) ;
#88005=CARTESIAN_POINT('Ctrl Pts',(-20.3863654461432,46.0663367391113,124.559830827429)) ;
#88006=CARTESIAN_POINT('Ctrl Pts',(-20.1756244871386,46.0761782404379,124.709777652691)) ;
#88007=CARTESIAN_POINT('Ctrl Pts',(-19.9396627498854,46.0861391920327,124.823081201135)) ;
#88008=CARTESIAN_POINT('Ctrl Pts',(-19.6855248863959,46.0961770097533,124.893729687363)) ;
#88009=CARTESIAN_POINT('Ctrl Pts',(-19.427262518452,46.1060513590104,124.919247547046)) ;
#88010=CARTESIAN_POINT('Ctrl Pts',(-19.1634478041723,46.1161209097526,124.899133803632)) ;
#88011=CARTESIAN_POINT('Ctrl Pts',(-18.9130319171502,46.1259549292612,124.835182189416)) ;
#88012=CARTESIAN_POINT('Ctrl Pts',(-18.6724817634697,46.1359890838408,124.727205773932)) ;
#88013=CARTESIAN_POINT('Ctrl Pts',(-18.4550722737311,46.1460050096632,124.57881549919)) ;
#88014=CARTESIAN_POINT('Ctrl Pts',(-18.2689263313037,46.1558872648575,124.397725200321)) ;
#88015=CARTESIAN_POINT('Ctrl Pts',(-18.1151695920916,46.1658760713684,124.185010592068)) ;
#88016=CARTESIAN_POINT('Ctrl Pts',(-18.0009343743277,46.1758246386311,123.949804922474)) ;
#88017=CARTESIAN_POINT('Ctrl Pts',(-17.9287986502812,46.1858794439331,123.695642276881)) ;
#88018=CARTESIAN_POINT('Ctrl Pts',(-17.9021457183122,46.1956982271967,123.438981604419)) ;
#88019=CARTESIAN_POINT('Ctrl Pts',(-17.920160334372,46.2057339995573,123.175874359375)) ;
#88020=CARTESIAN_POINT('Ctrl Pts',(-17.984249977082,46.2157586985859,122.920340925666)) ;
#88021=CARTESIAN_POINT('Ctrl Pts',(-18.0893591005861,46.225610701845,122.683731790801)) ;
#88022=CARTESIAN_POINT('Ctrl Pts',(-18.2356413391738,46.2356016362422,122.465745544367)) ;
#88023=CARTESIAN_POINT('Ctrl Pts',(-18.4161423749505,46.2455195586733,122.277688444646)) ;
#88024=CARTESIAN_POINT('Ctrl Pts',(-18.6288192425981,46.2555479143556,122.122101309996)) ;
#88025=CARTESIAN_POINT('Ctrl Pts',(-18.8618561314838,46.2654321988662,122.007348465011)) ;
#88026=CARTESIAN_POINT('Ctrl Pts',(-19.1138378721338,46.2754248827741,121.933438370644)) ;
#88027=CARTESIAN_POINT('Ctrl Pts',(-19.3758193880109,46.2854536197818,121.904757212364)) ;
#88028=CARTESIAN_POINT('Ctrl Pts',(-19.6350724012937,46.2953390164107,121.921411675567)) ;
#88029=CARTESIAN_POINT('Ctrl Pts',(-19.8901659266548,46.3053269018246,121.983092596544)) ;
#88030=CARTESIAN_POINT('Ctrl Pts',(-20.1298859961201,46.3152776044852,122.087654097686)) ;
#88031=CARTESIAN_POINT('Ctrl Pts',(-20.3496387002322,46.3253179225826,122.233636338155)) ;
#88032=CARTESIAN_POINT('Ctrl Pts',(-20.5377696612843,46.3351924879158,122.412406684327)) ;
#88033=CARTESIAN_POINT('Ctrl Pts',(-20.6941818778816,46.3451921479769,122.623513973067)) ;
#88034=CARTESIAN_POINT('Ctrl Pts',(-20.8107624841862,46.3551011431446,122.856409152193)) ;
#88035=CARTESIAN_POINT('Ctrl Pts',(-20.8861223158461,46.3651558843079,123.109617925359)) ;
#88036=CARTESIAN_POINT('Ctrl Pts',(-20.9160894530664,46.3750144962217,123.366999052458)) ;
#88037=CARTESIAN_POINT('Ctrl Pts',(-20.90075393306,46.385082618501,123.631095083211)) ;
#88038=CARTESIAN_POINT('Ctrl Pts',(-20.8410490247791,46.3949380892042,123.883133457476)) ;
#88039=CARTESIAN_POINT('Ctrl Pts',(-20.7377739074065,46.4049329486976,124.124622613945)) ;
#88040=CARTESIAN_POINT('Ctrl Pts',(-20.5931317991477,46.4149642020395,124.345013634199)) ;
#88041=CARTESIAN_POINT('Ctrl Pts',(-20.4156811920431,46.4248309009126,124.534077171764)) ;
#88042=CARTESIAN_POINT('Ctrl Pts',(-20.2058603225502,46.4348177166638,124.691672146936)) ;
#88043=CARTESIAN_POINT('Ctrl Pts',(-19.9727878453625,46.4447649218593,124.810106319578)) ;
#88044=CARTESIAN_POINT('Ctrl Pts',(-19.7203014995016,46.4548079099855,124.886878521839)) ;
#88045=CARTESIAN_POINT('Ctrl Pts',(-19.462892547754,46.464675264607,124.918244909157)) ;
#88046=CARTESIAN_POINT('Ctrl Pts',(-19.2013450743715,46.4746411579051,124.905008550705)) ;
#88047=CARTESIAN_POINT('Ctrl Pts',(-18.9446202495613,46.4846649352812,124.845948246086)) ;
#88048=CARTESIAN_POINT('Ctrl Pts',(-18.7044304082566,46.4945904832129,124.744281867912)) ;
#88049=CARTESIAN_POINT('Ctrl Pts',(-18.4848534110883,46.5045309596339,124.60274474947)) ;
#88050=CARTESIAN_POINT('Ctrl Pts',(-18.2913765899753,46.5145771692968,124.423144114639)) ;
#88051=CARTESIAN_POINT('Ctrl Pts',(-18.1347125364933,46.5244384259586,124.216689383634)) ;
#88052=CARTESIAN_POINT('Ctrl Pts',(-18.0143126829843,46.5344320542339,123.983335039586)) ;
#88053=CARTESIAN_POINT('Ctrl Pts',(-17.9366394008495,46.5443574515441,123.734298668841)) ;
#88054=CARTESIAN_POINT('Ctrl Pts',(-17.9030455996264,46.5543853594543,123.472960192196)) ;
#88055=CARTESIAN_POINT('Ctrl Pts',(-17.9149012642186,46.5642716751235,123.213390481439)) ;
#88056=CARTESIAN_POINT('Ctrl Pts',(-17.972325349276,46.5743032700273,122.956144198347)) ;
#88057=CARTESIAN_POINT('Ctrl Pts',(-18.0718482092479,46.584185512979,122.716230515682)) ;
#88058=CARTESIAN_POINT('Ctrl Pts',(-18.2138880944537,46.5942449840088,122.493315287928)) ;
#88059=CARTESIAN_POINT('Ctrl Pts',(-18.3891039122629,46.604111428672,122.302179808622)) ;
#88060=CARTESIAN_POINT('Ctrl Pts',(-18.596403594826,46.6140775531207,122.142134294108)) ;
#88061=CARTESIAN_POINT('Ctrl Pts',(-18.8300357306055,46.6241077965118,122.020104455616)) ;
#88062=CARTESIAN_POINT('Ctrl Pts',(-19.0777840409719,46.6340008314649,121.941221742418)) ;
#88063=CARTESIAN_POINT('Ctrl Pts',(-19.3395213808909,46.6440517457017,121.905936560177)) ;
#88064=CARTESIAN_POINT('Ctrl Pts',(-19.5992144386022,46.6539415719263,121.916434213114)) ;
#88065=CARTESIAN_POINT('Ctrl Pts',(-19.9417614873954,46.6672763869732,121.990497581648)) ;
#88066=CARTESIAN_POINT('Ctrl Pts',(-20.2554096954557,46.6805534781447,122.152105027392)) ;
#88067=CARTESIAN_POINT('Ctrl Pts',(-20.5136667534488,46.693801766743,122.385643139726)) ;
#88068=CARTESIAN_POINT('Ctrl Pts',(-20.6757363842069,46.7038566082371,122.594281387087)) ;
#88069=CARTESIAN_POINT('Ctrl Pts',(-20.7967988624566,46.7136875975446,122.822559708019)) ;
#88070=CARTESIAN_POINT('Ctrl Pts',(-20.8785312557402,46.7237641618679,123.074384834974)) ;
#88071=CARTESIAN_POINT('Ctrl Pts',(-20.9144702982914,46.7336134870018,123.33073485832)) ;
#88072=CARTESIAN_POINT('Ctrl Pts',(-20.9029684187357,46.7469614866391,123.681333495441)) ;
#88073=CARTESIAN_POINT('Ctrl Pts',(-20.7745139330427,46.7635462461757,124.102969724517)) ;
#88074=CARTESIAN_POINT('Ctrl Pts',(-20.5110315388571,46.7801147975237,124.4557847313)) ;
#88075=CARTESIAN_POINT('Ctrl Pts',(-20.23514044175,46.7934746223427,124.672959741583)) ;
#88076=CARTESIAN_POINT('Ctrl Pts',(-20.0058449666823,46.8033800311734,124.796184304861)) ;
#88077=CARTESIAN_POINT('Ctrl Pts',(-19.7574240387125,46.8133400577574,124.878527441293)) ;
#88078=CARTESIAN_POINT('Ctrl Pts',(-19.4127438329402,46.8265976419427,124.929510558515)) ;
#88079=CARTESIAN_POINT('Ctrl Pts',(-18.9730785233433,46.8432488534374,124.87894995727)) ;
#88080=CARTESIAN_POINT('Ctrl Pts',(-18.4995437565153,46.8631670675477,124.642323373345)) ;
#88081=CARTESIAN_POINT('Ctrl Pts',(-18.1350267198472,46.8830448307685,124.259795228635)) ;
#88082=CARTESIAN_POINT('Ctrl Pts',(-17.9219959153182,46.9030574985557,123.772520415574)) ;
#88083=CARTESIAN_POINT('Ctrl Pts',(-17.8878670522062,46.9228700212223,123.246943798671)) ;
#88084=CARTESIAN_POINT('Ctrl Pts',(-18.035546506357,46.9428533212222,122.736872230293)) ;
#88085=CARTESIAN_POINT('Ctrl Pts',(-18.3474461325361,46.9627475983235,122.309804698334)) ;
#88086=CARTESIAN_POINT('Ctrl Pts',(-18.7866677876835,46.9826803600813,122.013601770197)) ;
#88087=CARTESIAN_POINT('Ctrl Pts',(-19.3015657425341,47.002646365846,121.885203552185)) ;
#88088=CARTESIAN_POINT('Ctrl Pts',(-19.8271303436553,47.0225248980109,121.939603120483)) ;
#88089=CARTESIAN_POINT('Ctrl Pts',(-20.3041868868379,47.0424645646712,122.170298147785)) ;
#88090=CARTESIAN_POINT('Ctrl Pts',(-20.6732403950815,47.0623594393166,122.549057326393)) ;
#88091=CARTESIAN_POINT('Ctrl Pts',(-20.8914282381446,47.0822665786099,123.030940138027)) ;
#88092=CARTESIAN_POINT('Ctrl Pts',(-20.9330126326835,47.1021771266884,123.558665033763)) ;
#88093=CARTESIAN_POINT('Ctrl Pts',(-20.7897985089648,47.1222457120455,124.072348596256)) ;
#88094=CARTESIAN_POINT('Ctrl Pts',(-20.4845832960142,47.1420275093603,124.500664842063)) ;
#88095=CARTESIAN_POINT('Ctrl Pts',(-20.0473415775769,47.1620350563049,124.802948543256)) ;
#88096=CARTESIAN_POINT('Ctrl Pts',(-19.5376373388019,47.1818567946077,124.936737621714)) ;
#88097=CARTESIAN_POINT('Ctrl Pts',(-19.0088143994453,47.2018368145119,124.889159509882)) ;
#88098=CARTESIAN_POINT('Ctrl Pts',(-18.5296831814101,47.2217542657741,124.664016484713)) ;
#88099=CARTESIAN_POINT('Ctrl Pts',(-18.156054658413,47.2416291869468,124.290549692997)) ;
#88100=CARTESIAN_POINT('Ctrl Pts',(-17.9309560929439,47.2616535554976,123.808318679437)) ;
#88101=CARTESIAN_POINT('Ctrl Pts',(-17.8844429064027,47.2815202398711,123.282262426708)) ;
#88102=CARTESIAN_POINT('Ctrl Pts',(-18.0199062073946,47.3014640617173,122.769851703785)) ;
#88103=CARTESIAN_POINT('Ctrl Pts',(-18.321723185349,47.3213714309688,122.335270498965)) ;
#88104=CARTESIAN_POINT('Ctrl Pts',(-18.7524373240201,47.3412461287155,122.029471467672)) ;
#88105=CARTESIAN_POINT('Ctrl Pts',(-19.2643995478987,47.3612280712373,121.888115658735)) ;
#88106=CARTESIAN_POINT('Ctrl Pts',(-19.7916438055128,47.3811307381481,121.930221264192)) ;
#88107=CARTESIAN_POINT('Ctrl Pts',(-20.2724952367668,47.4009860956868,122.147830932133)) ;
#88108=CARTESIAN_POINT('Ctrl Pts',(-20.6536636578321,47.4210501344028,122.52065673183)) ;
#88109=CARTESIAN_POINT('Ctrl Pts',(-20.8822481029672,47.4409053141279,122.996516067802)) ;
#88110=CARTESIAN_POINT('Ctrl Pts',(-20.935436165233,47.4608854187923,123.524678358585)) ;
#88111=CARTESIAN_POINT('Ctrl Pts',(-20.8068403946321,47.4806945239621,124.035381850163)) ;
#88112=CARTESIAN_POINT('Ctrl Pts',(-20.5095795524021,47.5006871443028,124.475622450521)) ;
#88113=CARTESIAN_POINT('Ctrl Pts',(-20.1539694207839,47.5172266268069,124.734264236863)) ;
#88114=CARTESIAN_POINT('Ctrl Pts',(-19.8262823346885,47.5305909448711,124.860472249389)) ;
#88115=CARTESIAN_POINT('Ctrl Pts',(-19.485405542771,47.5438085473726,124.927559945783)) ;
#88116=CARTESIAN_POINT('Ctrl Pts',(-19.0437703200357,47.5604661416504,124.898016262381)) ;
#88117=CARTESIAN_POINT('Ctrl Pts',(-18.5604499932118,47.5803318436921,124.685212590745)) ;
#88118=CARTESIAN_POINT('Ctrl Pts',(-18.2406362283115,47.5969615703822,124.380257695188)) ;
#88119=CARTESIAN_POINT('Ctrl Pts',(-18.0589404833083,47.61025068552,124.081950760843)) ;
#88120=CARTESIAN_POINT('Ctrl Pts',(-17.9633474747988,47.6202150324971,123.838187618009)) ;
#88121=CARTESIAN_POINT('Ctrl Pts',(-17.9115445460179,47.6301434004986,123.582486569596)) ;
#88122=CARTESIAN_POINT('Ctrl Pts',(-17.9020103793018,47.6434268335873,123.233497874318)) ;
#88123=CARTESIAN_POINT('Ctrl Pts',(-18.005095080809,47.6600789113277,122.803114333347)) ;
#88124=CARTESIAN_POINT('Ctrl Pts',(-18.247209882945,47.6766302806285,122.435837759358)) ;
#88125=CARTESIAN_POINT('Ctrl Pts',(-18.50783847541,47.6899177087775,122.203427580766)) ;
#88126=CARTESIAN_POINT('Ctrl Pts',(-18.7324805385707,47.6999622484776,122.064856373526)) ;
#88127=CARTESIAN_POINT('Ctrl Pts',(-18.9727568592771,47.7098050903014,121.969045673601)) ;
#88128=CARTESIAN_POINT('Ctrl Pts',(-19.2294948681427,47.7197893745484,121.915068774287)) ;
#88129=CARTESIAN_POINT('Ctrl Pts',(-19.4908350255121,47.7297390199475,121.906573088993)) ;
#88130=CARTESIAN_POINT('Ctrl Pts',(-19.7510324518848,47.7397387816359,121.943450958025)) ;
#88131=CARTESIAN_POINT('Ctrl Pts',(-20.001511154546,47.7497701275948,122.025612884837)) ;
#88132=CARTESIAN_POINT('Ctrl Pts',(-20.2300186287295,47.7596250820719,122.147499644092)) ;
#88133=CARTESIAN_POINT('Ctrl Pts',(-20.4366754769559,47.7695976200724,122.308615609026)) ;
#88134=CARTESIAN_POINT('Ctrl Pts',(-20.612644360831,47.7795926138074,122.503667729469)) ;
#88135=CARTESIAN_POINT('Ctrl Pts',(-20.7523101013191,47.7896266726015,122.727299317315)) ;
#88136=CARTESIAN_POINT('Ctrl Pts',(-20.8496668786128,47.7994820154245,122.967319880366)) ;
#88137=CARTESIAN_POINT('Ctrl Pts',(-20.904992548046,47.8094814947701,123.224157421193)) ;
#88138=CARTESIAN_POINT('Ctrl Pts',(-20.9150779626639,47.8193759435254,123.484026654786)) ;
#88139=CARTESIAN_POINT('Ctrl Pts',(-20.879224101965,47.8294390629599,123.745986877431)) ;
#88140=CARTESIAN_POINT('Ctrl Pts',(-20.8004688342771,47.8392787082011,123.992322380341)) ;
#88141=CARTESIAN_POINT('Ctrl Pts',(-20.6777398160996,47.8493418723872,124.226526704695)) ;
#88142=CARTESIAN_POINT('Ctrl Pts',(-20.5187066498922,47.859236142136,124.432268221858)) ;
#88143=CARTESIAN_POINT('Ctrl Pts',(-20.3259668872383,47.8691778681498,124.608589479913)) ;
#88144=CARTESIAN_POINT('Ctrl Pts',(-20.1041808999464,47.8791807568092,124.749765186793)) ;
#88145=CARTESIAN_POINT('Ctrl Pts',(-19.8602299792522,47.8892206056032,124.850187093091)) ;
#88146=CARTESIAN_POINT('Ctrl Pts',(-19.6081642424219,47.8990448210641,124.906094643254)) ;
#88147=CARTESIAN_POINT('Ctrl Pts',(-19.3441702977261,47.9091016645576,124.918019813108)) ;
#88148=CARTESIAN_POINT('Ctrl Pts',(-19.0854703555384,47.9190302739536,124.884016066394)) ;
#88149=CARTESIAN_POINT('Ctrl Pts',(-18.835802023627,47.9289821579915,124.806127703608)) ;
#88150=CARTESIAN_POINT('Ctrl Pts',(-18.6013347301841,47.9390351107991,124.684442693465)) ;
#88151=CARTESIAN_POINT('Ctrl Pts',(-18.3960367832778,47.9488579872653,124.527928911458)) ;
#88152=CARTESIAN_POINT('Ctrl Pts',(-18.2165695066782,47.9589137198354,124.333990312506)) ;
#88153=CARTESIAN_POINT('Ctrl Pts',(-18.0755119524271,47.9688544848231,124.114102984926)) ;
#88154=CARTESIAN_POINT('Ctrl Pts',(-17.97439677815,47.9787588177287,123.874266207495)) ;
#88155=CARTESIAN_POINT('Ctrl Pts',(-17.9157978478123,47.9888054866094,123.616858452994)) ;
#88156=CARTESIAN_POINT('Ctrl Pts',(-17.9027391893822,47.9987010499152,123.357099240434)) ;
#88157=CARTESIAN_POINT('Ctrl Pts',(-17.9355139727328,48.0087631076155,123.094756208375)) ;
#88158=CARTESIAN_POINT('Ctrl Pts',(-18.0115247975341,48.018605885243,122.847487885336)) ;
#88159=CARTESIAN_POINT('Ctrl Pts',(-18.130499270546,48.0285963634949,122.613492148444)) ;
#88160=CARTESIAN_POINT('Ctrl Pts',(-18.2873849531134,48.0385253361384,122.404982545336)) ;
#88161=CARTESIAN_POINT('Ctrl Pts',(-18.4789956662502,48.048516473018,122.225477178445)) ;
#88162=CARTESIAN_POINT('Ctrl Pts',(-18.6997215251481,48.0585385905069,122.081788244482)) ;
#88163=CARTESIAN_POINT('Ctrl Pts',(-18.9390060894404,48.0684391009091,121.979633386977)) ;
#88164=CARTESIAN_POINT('Ctrl Pts',(-19.1945602868354,48.0784280936552,121.9196516612)) ;
#88165=CARTESIAN_POINT('Ctrl Pts',(-19.4560251777434,48.0883933377058,121.905170872972)) ;
#88166=CARTESIAN_POINT('Ctrl Pts',(-19.714544749918,48.098297602219,121.935512588317)) ;
#88167=CARTESIAN_POINT('Ctrl Pts',(-19.9676521572524,48.1083556939172,122.01159018475)) ;
#88168=CARTESIAN_POINT('Ctrl Pts',(-20.1989410280847,48.1182056343456,122.127843264376)) ;
#88169=CARTESIAN_POINT('Ctrl Pts',(-20.4106352779193,48.1282326455192,122.284734900046)) ;
#88170=CARTESIAN_POINT('Ctrl Pts',(-20.5914129661359,48.1382612321312,122.476515291714)) ;
#88171=CARTESIAN_POINT('Ctrl Pts',(-20.7338940826546,48.1481064462439,122.692453451488)) ;
#88172=CARTESIAN_POINT('Ctrl Pts',(-20.8388889355934,48.1580971944235,122.933098046713)) ;
#88173=CARTESIAN_POINT('Ctrl Pts',(-20.9002278538488,48.168134828009,123.189645406397)) ;
#88174=CARTESIAN_POINT('Ctrl Pts',(-20.9162157833847,48.1779801172218,123.447878692139)) ;
#88175=CARTESIAN_POINT('Ctrl Pts',(-20.8873032918651,48.1879615180277,123.708561008633)) ;
#88176=CARTESIAN_POINT('Ctrl Pts',(-20.8137139164343,48.1979137510176,123.959536527466)) ;
#88177=CARTESIAN_POINT('Ctrl Pts',(-20.6974226162219,48.2079125624742,124.195182186014)) ;
#88178=CARTESIAN_POINT('Ctrl Pts',(-20.5409679874558,48.2179516664049,124.40758088976)) ;
#88179=CARTESIAN_POINT('Ctrl Pts',(-20.3544447338278,48.2277766088242,124.58612785741)) ;
#88180=CARTESIAN_POINT('Ctrl Pts',(-20.1350015577314,48.2378312963002,124.733273340073)) ;
#88181=CARTESIAN_POINT('Ctrl Pts',(-19.8958290741237,48.247774098657,124.838493759771)) ;
#88182=CARTESIAN_POINT('Ctrl Pts',(-19.6432087007226,48.2576778945968,124.901118420341)) ;
#88183=CARTESIAN_POINT('Ctrl Pts',(-19.3798197798372,48.2677246739718,124.919026044654)) ;
#88184=CARTESIAN_POINT('Ctrl Pts',(-19.1211868057863,48.2776203322664,124.891570258685)) ;
#88185=CARTESIAN_POINT('Ctrl Pts',(-18.8671159689922,48.287681899517,124.818466322481)) ;
#88186=CARTESIAN_POINT('Ctrl Pts',(-18.6346672337003,48.2975265439543,124.704882074842)) ;
#88187=CARTESIAN_POINT('Ctrl Pts',(-18.4224774448849,48.307486590197,124.551645752143)) ;
#88188=CARTESIAN_POINT('Ctrl Pts',(-18.2390630273348,48.3175248862154,124.362065332604)) ;
#88189=CARTESIAN_POINT('Ctrl Pts',(-18.0933378214402,48.3273982276337,124.147345292635)) ;
#88190=CARTESIAN_POINT('Ctrl Pts',(-17.9850701345174,48.337471331433,123.905844629381)) ;
#88191=CARTESIAN_POINT('Ctrl Pts',(-17.9216618145417,48.3472921465519,123.655621239189)) ;
#88192=CARTESIAN_POINT('Ctrl Pts',(-17.9018739629238,48.3573690116299,123.391601343181)) ;
#88193=CARTESIAN_POINT('Ctrl Pts',(-17.9277813877702,48.3672337512852,123.133631857944)) ;
#88194=CARTESIAN_POINT('Ctrl Pts',(-17.9985353622652,48.3772561545265,122.879946100013)) ;
#88195=CARTESIAN_POINT('Ctrl Pts',(-18.1129061323741,48.387281878815,122.642581869023)) ;
#88196=CARTESIAN_POINT('Ctrl Pts',(-18.2637423254893,48.3971366618363,122.432087433426)) ;
#88197=CARTESIAN_POINT('Ctrl Pts',(-18.4507029295602,48.4071155055596,122.248197667358)) ;
#88198=CARTESIAN_POINT('Ctrl Pts',(-18.6678616263483,48.4171343977962,122.099352690164)) ;
#88199=CARTESIAN_POINT('Ctrl Pts',(-18.9041396211026,48.4270176068372,121.991439850928)) ;
#88200=CARTESIAN_POINT('Ctrl Pts',(-19.1602260657838,48.4370859161774,121.925097919403)) ;
#88201=CARTESIAN_POINT('Ctrl Pts',(-19.4177670696848,48.4469160415101,121.904413532861)) ;
#88202=CARTESIAN_POINT('Ctrl Pts',(-19.6811181172093,48.4569825938871,121.928996874006)) ;
#88203=CARTESIAN_POINT('Ctrl Pts',(-19.9317618895005,48.4668728307808,121.997882966823)) ;
#88204=CARTESIAN_POINT('Ctrl Pts',(-20.1692610222621,48.4768650555748,122.109851831293)) ;
#88205=CARTESIAN_POINT('Ctrl Pts',(-20.3829445510021,48.4868276759257,122.261113657658)) ;
#88206=CARTESIAN_POINT('Ctrl Pts',(-20.5665261218062,48.4967326786889,122.445666071956)) ;
#88207=CARTESIAN_POINT('Ctrl Pts',(-20.7173958030492,48.506790441087,122.662655601088)) ;
#88208=CARTESIAN_POINT('Ctrl Pts',(-20.8262238273378,48.5166409604658,122.897552034887)) ;
#88209=CARTESIAN_POINT('Ctrl Pts',(-20.8943829996658,48.526672537464,123.152189944527)) ;
#88210=CARTESIAN_POINT('Ctrl Pts',(-20.9167426169127,48.5366822725689,123.414312273892)) ;
#88211=CARTESIAN_POINT('Ctrl Pts',(-20.8937179531658,48.5465918491952,123.673683390135)) ;
#88212=CARTESIAN_POINT('Ctrl Pts',(-20.8265228052753,48.5565192350519,123.925774756106)) ;
#88213=CARTESIAN_POINT('Ctrl Pts',(-20.7150907300863,48.5665641695422,124.165059353475)) ;
#88214=CARTESIAN_POINT('Ctrl Pts',(-20.5663090616085,48.5764501017301,124.378048058078)) ;
#88215=CARTESIAN_POINT('Ctrl Pts',(-20.3811550715041,48.5864434076831,124.564263272707)) ;
#88216=CARTESIAN_POINT('Ctrl Pts',(-20.1674323885774,48.596389045465,124.714704721664)) ;
#88217=CARTESIAN_POINT('Ctrl Pts',(-19.9310127579831,48.6063363138109,124.826259865705)) ;
#88218=CARTESIAN_POINT('Ctrl Pts',(-19.6762062907194,48.616384215948,124.895474138505)) ;
#88219=CARTESIAN_POINT('Ctrl Pts',(-19.4185018206962,48.6262319107882,124.919135372387)) ;
#88220=CARTESIAN_POINT('Ctrl Pts',(-19.157566898572,48.6361934205326,124.898267563706)) ;
#88221=CARTESIAN_POINT('Ctrl Pts',(-18.9025619508575,48.6462228121415,124.831614773843)) ;
#88222=CARTESIAN_POINT('Ctrl Pts',(-18.6658627752509,48.6561303076962,124.723165141493)) ;
#88223=CARTESIAN_POINT('Ctrl Pts',(-18.4504930203598,48.6660756993592,124.575141126783)) ;
#88224=CARTESIAN_POINT('Ctrl Pts',(-18.2628876791554,48.6760776169566,124.391000597497)) ;
#88225=CARTESIAN_POINT('Ctrl Pts',(-18.1099535759632,48.6861176845088,124.176032718824)) ;
#88226=CARTESIAN_POINT('Ctrl Pts',(-17.9985528130765,48.6959419959486,123.943106599342)) ;
#88227=CARTESIAN_POINT('Ctrl Pts',(-17.9273154063796,48.7059982371047,123.688649150822)) ;
#88228=CARTESIAN_POINT('Ctrl Pts',(-17.9019656863292,48.7159291588403,123.428879136997)) ;
#88229=CARTESIAN_POINT('Ctrl Pts',(-17.9215938866681,48.7258723949166,123.168352780034)) ;
#88230=CARTESIAN_POINT('Ctrl Pts',(-17.9861802002328,48.735853678929,122.914090093812)) ;
#88231=CARTESIAN_POINT('Ctrl Pts',(-18.0949989715361,48.7458979805547,122.673647794656)) ;
#88232=CARTESIAN_POINT('Ctrl Pts',(-18.2402534708388,48.7557260617741,122.460043836669)) ;
#88233=CARTESIAN_POINT('Ctrl Pts',(-18.4247849710024,48.7658026646233,122.270203460101)) ;
#88234=CARTESIAN_POINT('Ctrl Pts',(-18.6347065996334,48.7756547437418,122.118569547531)) ;
#88235=CARTESIAN_POINT('Ctrl Pts',(-18.8728105251633,48.7857280020508,122.002995475702)) ;
#88236=CARTESIAN_POINT('Ctrl Pts',(-19.1215857423761,48.7955694614311,121.932239761547)) ;
#88237=CARTESIAN_POINT('Ctrl Pts',(-19.3818649812545,48.8055305568434,121.904458482012)) ;
#88238=CARTESIAN_POINT('Ctrl Pts',(-19.6449795161499,48.8155678412401,121.922944960723)) ;
#88239=CARTESIAN_POINT('Ctrl Pts',(-19.8969273677844,48.8254441799754,121.985379683799)) ;
#88240=CARTESIAN_POINT('Ctrl Pts',(-20.1386336262622,48.8355063061287,122.092521249283)) ;
#88241=CARTESIAN_POINT('Ctrl Pts',(-20.3539244509202,48.8453744801052,122.237144739534)) ;
#88242=CARTESIAN_POINT('Ctrl Pts',(-20.543755011927,48.855380028609,122.419026520356)) ;
#88243=CARTESIAN_POINT('Ctrl Pts',(-20.6987419364052,48.8653626605046,122.630740739498)) ;
#88244=CARTESIAN_POINT('Ctrl Pts',(-20.8150482287937,48.8754066029264,122.867653599729)) ;
#88245=CARTESIAN_POINT('Ctrl Pts',(-20.8872135170498,48.8852347509536,123.115640682786)) ;
#88246=CARTESIAN_POINT('Ctrl Pts',(-20.9165222913364,48.8952246183279,123.376523659417)) ;
#88247=CARTESIAN_POINT('Ctrl Pts',(-20.8993147872527,48.9052683572834,123.639900737698)) ;
#88248=CARTESIAN_POINT('Ctrl Pts',(-20.8385460028974,48.9150901058214,123.890749443944)) ;
#88249=CARTESIAN_POINT('Ctrl Pts',(-20.7334926344583,48.9251250834311,124.132629488794)) ;
#88250=CARTESIAN_POINT('Ctrl Pts',(-20.5875669348054,48.9351499961888,124.351974416172)) ;
#88251=CARTESIAN_POINT('Ctrl Pts',(-20.4093201184437,48.9450019392826,124.539749635484)) ;
#88252=CARTESIAN_POINT('Ctrl Pts',(-20.1985093079883,48.9549929006117,124.696195980077)) ;
#88253=CARTESIAN_POINT('Ctrl Pts',(-19.9654731355136,48.9649107754802,124.812985422573)) ;
#88254=CARTESIAN_POINT('Ctrl Pts',(-19.7129807407904,48.9749392944814,124.888406605347)) ;
#88255=CARTESIAN_POINT('Ctrl Pts',(-19.4549910732823,48.9848229732793,124.918538485184)) ;
#88256=CARTESIAN_POINT('Ctrl Pts',(-19.1927471785049,48.994817916719,124.903825171715)) ;
#88257=CARTESIAN_POINT('Ctrl Pts',(-18.9363271652186,49.0048447705414,124.84316892203)) ;
#88258=CARTESIAN_POINT('Ctrl Pts',(-18.6976274329194,49.0147289348803,124.740719075366)) ;
#88259=CARTESIAN_POINT('Ctrl Pts',(-18.4778974629818,49.0247170329227,124.597194644998)) ;
#88260=CARTESIAN_POINT('Ctrl Pts',(-18.2869925249069,49.0346681393798,124.418428962904)) ;
#88261=CARTESIAN_POINT('Ctrl Pts',(-18.1286921061756,49.0447131905479,124.207206823015)) ;
#88262=CARTESIAN_POINT('Ctrl Pts',(-18.0115110053641,49.0545749509062,123.976053919716)) ;
#88263=CARTESIAN_POINT('Ctrl Pts',(-17.9347018565793,49.0645377677367,123.725760547945)) ;
#88264=CARTESIAN_POINT('Ctrl Pts',(-17.9027372037974,49.0745724490174,123.464015962194)) ;
#88265=CARTESIAN_POINT('Ctrl Pts',(-17.9160561245772,49.0844574787982,123.204553334292)) ;
#88266=CARTESIAN_POINT('Ctrl Pts',(-17.9753271704611,49.0945230721962,122.946810192394)) ;
#88267=CARTESIAN_POINT('Ctrl Pts',(-18.0759231780919,49.1043622405577,122.708574067968)) ;
#88268=CARTESIAN_POINT('Ctrl Pts',(-18.2192006262921,49.1144248382992,122.486356375471)) ;
#88269=CARTESIAN_POINT('Ctrl Pts',(-18.3961652533745,49.1243218507061,122.2957392912)) ;
#88270=CARTESIAN_POINT('Ctrl Pts',(-18.6037154643153,49.1342531725317,122.137521228201)) ;
#88271=CARTESIAN_POINT('Ctrl Pts',(-18.8382964268997,49.1442949352862,122.016665264985)) ;
#88272=CARTESIAN_POINT('Ctrl Pts',(-19.0864079744247,49.1541831341769,121.939390497466)) ;
#88273=CARTESIAN_POINT('Ctrl Pts',(-19.3468353464452,49.1641770727768,121.905608425672)) ;
#88274=CARTESIAN_POINT('Ctrl Pts',(-19.6078151277302,49.1741178938136,121.91751361713)) ;
#88275=CARTESIAN_POINT('Ctrl Pts',(-19.8632816579453,49.1840772761019,121.974327396906)) ;
#88276=CARTESIAN_POINT('Ctrl Pts',(-20.1060322896982,49.1940750357542,122.074891251936)) ;
#88277=CARTESIAN_POINT('Ctrl Pts',(-20.3282620364892,49.2041111719565,122.21690786839)) ;
#88278=CARTESIAN_POINT('Ctrl Pts',(-20.5190808378173,49.2139619694474,122.391836817215)) ;
#88279=CARTESIAN_POINT('Ctrl Pts',(-20.6790012985683,49.2239228345237,122.599055308519)) ;
#88280=CARTESIAN_POINT('Ctrl Pts',(-20.8010708002223,49.2339517021541,122.832645696346)) ;
#88281=CARTESIAN_POINT('Ctrl Pts',(-20.879853818226,49.2438619382905,123.080862806442)) ;
#88282=CARTESIAN_POINT('Ctrl Pts',(-20.9151078932877,49.253796891605,123.339559285952)) ;
#88283=CARTESIAN_POINT('Ctrl Pts',(-20.9045592317714,49.2638378220146,123.603207119489)) ;
#88284=CARTESIAN_POINT('Ctrl Pts',(-20.8494077535675,49.2737257187962,123.857140794924)) ;
#88285=CARTESIAN_POINT('Ctrl Pts',(-20.7504505562724,49.2837151704549,124.100280633098)) ;
#88286=CARTESIAN_POINT('Ctrl Pts',(-20.6110277047872,49.2936742608203,124.321756486501)) ;
#88287=CARTESIAN_POINT('Ctrl Pts',(-20.4368338343713,49.3035715731266,124.514921157602)) ;
#88288=CARTESIAN_POINT('Ctrl Pts',(-20.2284024122809,49.3136279990268,124.677354927092)) ;
#88289=CARTESIAN_POINT('Ctrl Pts',(-19.9992830178138,49.3234980016166,124.798974471006)) ;
#88290=CARTESIAN_POINT('Ctrl Pts',(-19.7493901780766,49.3335019347938,124.880531822233)) ;
#88291=CARTESIAN_POINT('Ctrl Pts',(-19.4894780018953,49.3434891952577,124.917271202357)) ;
#88292=CARTESIAN_POINT('Ctrl Pts',(-19.2261559513639,49.3535162468434,124.908135759446)) ;
#88293=CARTESIAN_POINT('Ctrl Pts',(-18.9718205949569,49.3634073366695,124.854401512994)) ;
#88294=CARTESIAN_POINT('Ctrl Pts',(-18.6475387787366,49.3767050914506,124.724316756299)) ;
#88295=CARTESIAN_POINT('Ctrl Pts',(-18.3663439177842,49.3899031510587,124.514527900887)) ;
#88296=CARTESIAN_POINT('Ctrl Pts',(-18.1484048267078,49.4032998916279,124.238071111464)) ;
#88297=CARTESIAN_POINT('Ctrl Pts',(-18.0253527815644,49.4131708037013,124.009661322498)) ;
#88298=CARTESIAN_POINT('Ctrl Pts',(-17.9421985890326,49.4232443654695,123.758399347314)) ;
#88299=CARTESIAN_POINT('Ctrl Pts',(-17.9045673262481,49.4330657780578,123.502999840485)) ;
#88300=CARTESIAN_POINT('Ctrl Pts',(-17.9117874809025,49.4431397952888,123.238428805641)) ;
#88301=CARTESIAN_POINT('Ctrl Pts',(-17.9808625993538,49.4562985822534,122.899526034126)) ;
#88302=CARTESIAN_POINT('Ctrl Pts',(-18.1386493012278,49.4696646853476,122.58136729471)) ;
#88303=CARTESIAN_POINT('Ctrl Pts',(-18.3706579537025,49.4829786202367,122.319337160576)) ;
#88304=CARTESIAN_POINT('Ctrl Pts',(-18.5739338777232,49.4928786596841,122.157029405636)) ;
#88305=CARTESIAN_POINT('Ctrl Pts',(-18.8036238095851,49.5028430628186,122.031257984843)) ;
#88306=CARTESIAN_POINT('Ctrl Pts',(-19.05335921375,49.5128730299398,121.946955300818)) ;
#88307=CARTESIAN_POINT('Ctrl Pts',(-19.3105895258516,49.5227753065488,121.907692131419)) ;
#88308=CARTESIAN_POINT('Ctrl Pts',(-19.6591707264257,49.536041235718,121.91483615231)) ;
#88309=CARTESIAN_POINT('Ctrl Pts',(-20.0833606626239,49.5526627668244,122.037946979199)) ;
#88310=CARTESIAN_POINT('Ctrl Pts',(-20.5104593674055,49.5725375954691,122.348915166531)) ;
#88311=CARTESIAN_POINT('Ctrl Pts',(-20.7582535736872,49.5892108035709,122.716248365857)) ;
#88312=CARTESIAN_POINT('Ctrl Pts',(-20.8714352247518,49.6024619285522,123.045592382337)) ;
#88313=CARTESIAN_POINT('Ctrl Pts',(-20.9269354813126,49.615704247373,123.389194785708)) ;
#88314=CARTESIAN_POINT('Ctrl Pts',(-20.8811511581855,49.6324374877125,123.831492590155)) ;
#88315=CARTESIAN_POINT('Ctrl Pts',(-20.6511878464973,49.6522666359005,124.305812689138)) ;
#88316=CARTESIAN_POINT('Ctrl Pts',(-20.2723991280832,49.6721913310011,124.675727471051)) ;
#88317=CARTESIAN_POINT('Ctrl Pts',(-19.7899488954886,49.6921145595845,124.894193343067)) ;
#88318=CARTESIAN_POINT('Ctrl Pts',(-19.2619611266706,49.7120416987106,124.935069014905)) ;
#88319=CARTESIAN_POINT('Ctrl Pts',(-18.7527411075181,49.7319181613263,124.794310345686)) ;
#88320=CARTESIAN_POINT('Ctrl Pts',(-18.3198072271694,49.7518953899316,124.486931020539)) ;
#88321=CARTESIAN_POINT('Ctrl Pts',(-18.018710731692,49.7718302479053,124.050908756306)) ;
#88322=CARTESIAN_POINT('Ctrl Pts',(-17.8842375144528,49.7917266968361,123.539519466163)) ;
#88323=CARTESIAN_POINT('Ctrl Pts',(-17.9318221676816,49.8116479809027,123.012164589738)) ;
#88324=CARTESIAN_POINT('Ctrl Pts',(-18.1570615290371,49.8316046305737,122.531918504927)) ;
#88325=CARTESIAN_POINT('Ctrl Pts',(-18.5309830443767,49.8514819236853,122.158801133981)) ;
#88326=CARTESIAN_POINT('Ctrl Pts',(-19.0095255521828,49.8713683959137,121.934252429302)) ;
#88327=CARTESIAN_POINT('Ctrl Pts',(-19.5406391317515,49.8914299618377,121.886868078949)) ;
#88328=CARTESIAN_POINT('Ctrl Pts',(-20.0501878146875,49.9112703693785,122.022537685724)) ;
#88329=CARTESIAN_POINT('Ctrl Pts',(-20.4843856180674,49.9311216933514,122.322319927731)) ;
#88330=CARTESIAN_POINT('Ctrl Pts',(-20.7926218042951,49.9511749633028,122.757047288943)) ;
#88331=CARTESIAN_POINT('Ctrl Pts',(-20.9325314728205,49.9709956206862,123.265078314232)) ;
#88332=CARTESIAN_POINT('Ctrl Pts',(-20.8912422361684,49.9909670420167,123.794102750068)) ;
#88333=CARTESIAN_POINT('Ctrl Pts',(-20.672728228111,50.0108605343804,124.275780483601)) ;
#88334=CARTESIAN_POINT('Ctrl Pts',(-20.3004875803372,50.0308846206214,124.65599343755)) ;
#88335=CARTESIAN_POINT('Ctrl Pts',(-19.8260699488102,50.0506894997343,124.884165170859)) ;
#88336=CARTESIAN_POINT('Ctrl Pts',(-19.2984073272745,50.0706485154322,124.938579634073)) ;
#88337=CARTESIAN_POINT('Ctrl Pts',(-18.7834458131184,50.0906345390612,124.808287005669)) ;
#88338=CARTESIAN_POINT('Ctrl Pts',(-18.3471380862029,50.1104430348217,124.513561025804)) ;
#88339=CARTESIAN_POINT('Ctrl Pts',(-18.034433731144,50.1304256739273,124.08441134622)) ;
#88340=CARTESIAN_POINT('Ctrl Pts',(-17.8877548058213,50.1503071217213,123.576622519046)) ;
#88341=CARTESIAN_POINT('Ctrl Pts',(-17.9228590595857,50.1702635884589,123.047489138174)) ;
#88342=CARTESIAN_POINT('Ctrl Pts',(-18.135325664709,50.1901409854144,122.563692670579)) ;
#88343=CARTESIAN_POINT('Ctrl Pts',(-18.5017404753757,50.2101229315897,122.179326787256)) ;
#88344=CARTESIAN_POINT('Ctrl Pts',(-18.9763311717451,50.2300520306265,121.94386229144)) ;
#88345=CARTESIAN_POINT('Ctrl Pts',(-19.5025542136779,50.2499806538391,121.884425032197)) ;
#88346=CARTESIAN_POINT('Ctrl Pts',(-20.0154098113017,50.2698149779455,122.006618943828)) ;
#88347=CARTESIAN_POINT('Ctrl Pts',(-20.3852796718983,50.2864672653289,122.249530478733)) ;
#88348=CARTESIAN_POINT('Ctrl Pts',(-20.6170613698565,50.2997277663511,122.509825199118)) ;
#88349=CARTESIAN_POINT('Ctrl Pts',(-20.7555282047836,50.3097292435524,122.733215342447)) ;
#88350=CARTESIAN_POINT('Ctrl Pts',(-20.8529948357394,50.3197612644119,122.978175098663)) ;
#88351=CARTESIAN_POINT('Ctrl Pts',(-20.9058575761444,50.3296248081375,123.231923138614)) ;
#88352=CARTESIAN_POINT('Ctrl Pts',(-20.9146380480463,50.3395935218076,123.493747759478)) ;
#88353=CARTESIAN_POINT('Ctrl Pts',(-20.8648603610188,50.3529392692113,123.840886646443)) ;
#88354=CARTESIAN_POINT('Ctrl Pts',(-20.7281950716831,50.366089824284,124.162613928907)) ;
#88355=CARTESIAN_POINT('Ctrl Pts',(-20.5118305427497,50.3794752048338,124.439920066173)) ;
#88356=CARTESIAN_POINT('Ctrl Pts',(-20.3188172284818,50.3893631408267,124.613934022329)) ;
#88357=CARTESIAN_POINT('Ctrl Pts',(-20.0965116250302,50.3993543306393,124.753570663319)) ;
#88358=CARTESIAN_POINT('Ctrl Pts',(-19.8542622927966,50.4093064291776,124.852232186328)) ;
#88359=CARTESIAN_POINT('Ctrl Pts',(-19.5961633789181,50.4193526856281,124.907673196293)) ;
#88360=CARTESIAN_POINT('Ctrl Pts',(-19.3375104748675,50.4292021330222,124.917455726656)) ;
#88361=CARTESIAN_POINT('Ctrl Pts',(-19.0780426601325,50.4391647855174,124.882591527256)) ;
#88362=CARTESIAN_POINT('Ctrl Pts',(-18.8271559377994,50.4491878711595,124.802384290233)) ;
#88363=CARTESIAN_POINT('Ctrl Pts',(-18.5961209801117,50.4591129869164,124.681281420803)) ;
#88364=CARTESIAN_POINT('Ctrl Pts',(-18.3870807334424,50.4691654653163,124.519806842714)) ;
#88365=CARTESIAN_POINT('Ctrl Pts',(-18.2126501072753,50.479016964019,124.32847873655)) ;
#88366=CARTESIAN_POINT('Ctrl Pts',(-18.0718501454337,50.4889887032215,124.107511530402)) ;
#88367=CARTESIAN_POINT('Ctrl Pts',(-17.9713211447881,50.4989839109872,123.864801095388)) ;
#88368=CARTESIAN_POINT('Ctrl Pts',(-17.9145692121074,50.5090179124563,123.607321569366)) ;
#88369=CARTESIAN_POINT('Ctrl Pts',(-17.9031710447773,50.5188732705486,123.348557997671)) ;
#88370=CARTESIAN_POINT('Ctrl Pts',(-17.9370086645265,50.5288727461419,123.088017414384)) ;
#88371=CARTESIAN_POINT('Ctrl Pts',(-18.0144915110239,50.538767194637,122.839763225874)) ;
#88372=CARTESIAN_POINT('Ctrl Pts',(-18.1359636490848,50.5488303188647,122.604915926376)) ;
#88373=CARTESIAN_POINT('Ctrl Pts',(-18.2926316435237,50.5586699451933,122.399152962944)) ;
#88374=CARTESIAN_POINT('Ctrl Pts',(-18.486678321847,50.5687331802363,122.219538927624)) ;
#88375=CARTESIAN_POINT('Ctrl Pts',(-18.7053988201739,50.5786271854703,122.078904883828)) ;
#88376=CARTESIAN_POINT('Ctrl Pts',(-18.9460659097001,50.5885698986861,121.977250669726)) ;
#88377=CARTESIAN_POINT('Ctrl Pts',(-19.2023861460661,50.5985756384843,121.918495735838)) ;
#88378=CARTESIAN_POINT('Ctrl Pts',(-19.4653940518091,50.6085965406307,121.9054168295)) ;
#88379=CARTESIAN_POINT('Ctrl Pts',(-19.7233358092848,50.6184873106796,121.937482828107)) ;
#88380=CARTESIAN_POINT('Ctrl Pts',(-19.9744185614306,50.6284787214593,122.014246082198)) ;
#88381=CARTESIAN_POINT('Ctrl Pts',(-20.2073144805598,50.6384270671238,122.133004263277)) ;
#88382=CARTESIAN_POINT('Ctrl Pts',(-20.4163335012571,50.648371925185,122.289918302436)) ;
#88383=CARTESIAN_POINT('Ctrl Pts',(-20.5965902441456,50.6584267605779,122.483081634732)) ;
#88384=CARTESIAN_POINT('Ctrl Pts',(-20.7376425347096,50.6682491326794,122.69928261909)) ;
#88385=CARTESIAN_POINT('Ctrl Pts',(-20.8418429067607,50.6783050001231,122.942107997445)) ;
#88386=CARTESIAN_POINT('Ctrl Pts',(-20.9011591134657,50.688245729981,123.196526972203)) ;
#88387=CARTESIAN_POINT('Ctrl Pts',(-20.9161606255222,50.6981500685321,123.456374885143)) ;
#88388=CARTESIAN_POINT('Ctrl Pts',(-20.8852161971234,50.7081967499607,123.718548743211)) ;
#88389=CARTESIAN_POINT('Ctrl Pts',(-20.8105731784495,50.7180922574299,123.967693866746)) ;
#88390=CARTESIAN_POINT('Ctrl Pts',(-20.6918696445542,50.7281545259285,124.203934788214)) ;
#88391=CARTESIAN_POINT('Ctrl Pts',(-20.5374931111289,50.7379965161991,124.411487122097)) ;
#88392=CARTESIAN_POINT('Ctrl Pts',(-20.3469886042085,50.7479899330801,124.592192301977)) ;
#88393=CARTESIAN_POINT('Ctrl Pts',(-20.129467915059,50.7579144209322,124.736132155614)) ;
#88394=CARTESIAN_POINT('Ctrl Pts',(-19.8886030526091,50.7679140548407,124.841138181418)) ;
#88395=CARTESIAN_POINT('Ctrl Pts',(-19.6334526076263,50.7779001650975,124.902666745097)) ;
#88396=CARTESIAN_POINT('Ctrl Pts',(-19.370234794874,50.7879361162846,124.9187595243)) ;
#88397=CARTESIAN_POINT('Ctrl Pts',(-19.1128081761444,50.7977927546194,124.889819939285)) ;
#88398=CARTESIAN_POINT('Ctrl Pts',(-18.8606967834269,50.8077917146974,124.815928138923)) ;
#88399=CARTESIAN_POINT('Ctrl Pts',(-18.6274830798784,50.8176869450112,124.700806449973)) ;
#88400=CARTESIAN_POINT('Ctrl Pts',(-18.4143788196718,50.8277474574798,124.544393204072)) ;
#88401=CARTESIAN_POINT('Ctrl Pts',(-18.2353627908807,50.837596749026,124.357426939128)) ;
#88402=CARTESIAN_POINT('Ctrl Pts',(-18.0883925533693,50.8476239349582,124.138724931857)) ;
#88403=CARTESIAN_POINT('Ctrl Pts',(-17.9822394761601,50.8576524714175,123.897495737677)) ;
#88404=CARTESIAN_POINT('Ctrl Pts',(-17.9202588837812,50.8674977113825,123.646321073152)) ;
#88405=CARTESIAN_POINT('Ctrl Pts',(-17.9018714931078,50.8774884063057,123.384414305504)) ;
#88406=CARTESIAN_POINT('Ctrl Pts',(-17.9299486548859,50.8875262270643,123.122130520275)) ;
#88407=CARTESIAN_POINT('Ctrl Pts',(-18.0013103641566,50.8973708208412,122.873455872908)) ;
#88408=CARTESIAN_POINT('Ctrl Pts',(-18.1158568183376,50.9073548162173,122.637438180659)) ;
#88409=CARTESIAN_POINT('Ctrl Pts',(-18.2691496553917,50.9173038647787,122.425625938668)) ;
#88410=CARTESIAN_POINT('Ctrl Pts',(-18.4576995104374,50.9273063037532,122.242469851909)) ;
#88411=CARTESIAN_POINT('Ctrl Pts',(-18.675790127976,50.9373275450496,122.094857283506)) ;
#88412=CARTESIAN_POINT('Ctrl Pts',(-18.9129857115445,50.9472202234891,121.988448302435)) ;
#88413=CARTESIAN_POINT('Ctrl Pts',(-19.1674288630117,50.9572102774367,121.923807401294)) ;
#88414=CARTESIAN_POINT('Ctrl Pts',(-19.42840760001,50.9671686385852,121.904576356759)) ;
#88415=CARTESIAN_POINT('Ctrl Pts',(-19.6873151025459,50.97706826547,121.930161648276)) ;
#88416=CARTESIAN_POINT('Ctrl Pts',(-19.9415317404535,50.9871161622734,122.001441737826)) ;
#88417=CARTESIAN_POINT('Ctrl Pts',(-20.1760473918664,50.9970115199094,122.11388903272)) ;
#88418=CARTESIAN_POINT('Ctrl Pts',(-20.3909934475873,51.0070731723661,122.267820853643)) ;
#88419=CARTESIAN_POINT('Ctrl Pts',(-20.5720124432176,51.016917776638,122.452660571482)) ;
#88420=CARTESIAN_POINT('Ctrl Pts',(-20.7206679475832,51.026877898336,122.668085454437)) ;
#88421=CARTESIAN_POINT('Ctrl Pts',(-20.8300463265181,51.0369159326985,122.908118283207)) ;
#88422=CARTESIAN_POINT('Ctrl Pts',(-20.8954797450795,51.046790245285,123.159253141407)) ;
#88423=CARTESIAN_POINT('Ctrl Pts',(-20.9167078074931,51.0568597260677,123.422979437591)) ;
#88424=CARTESIAN_POINT('Ctrl Pts',(-20.8925366127019,51.0666940620848,123.68030532245)) ;
#88425=CARTESIAN_POINT('Ctrl Pts',(-20.8233738618489,51.076727019813,123.934719313341)) ;
#88426=CARTESIAN_POINT('Ctrl Pts',(-20.7105654023123,51.0867474183882,124.172661102908)) ;
#88427=CARTESIAN_POINT('Ctrl Pts',(-20.5610356799522,51.0966129921594,124.384475866047)) ;
#88428=CARTESIAN_POINT('Ctrl Pts',(-20.3732440668846,51.1066818668155,124.570842766502)) ;
#88429=CARTESIAN_POINT('Ctrl Pts',(-20.1607562670967,51.116527297721,124.718478795522)) ;
#88430=CARTESIAN_POINT('Ctrl Pts',(-19.9230357260641,51.1265069225917,124.829213605734)) ;
#88431=CARTESIAN_POINT('Ctrl Pts',(-19.6685786829973,51.1365256055058,124.896772999361)) ;
#88432=CARTESIAN_POINT('Ctrl Pts',(-19.4098095174621,51.1464088706896,124.919373434)) ;
#88433=CARTESIAN_POINT('Ctrl Pts',(-19.1462888986317,51.156477164781,124.896167375007)) ;
#88434=CARTESIAN_POINT('Ctrl Pts',(-18.8966808735186,51.1663072949663,124.829451529774)) ;
#88435=CARTESIAN_POINT('Ctrl Pts',(-18.6567504696124,51.1763738431815,124.718134366409)) ;
#88436=CARTESIAN_POINT('Ctrl Pts',(-18.4436238223543,51.1862640918701,124.569323332905)) ;
#88437=CARTESIAN_POINT('Ctrl Pts',(-18.2573048544974,51.1962562736461,124.384316168399)) ;
#88438=CARTESIAN_POINT('Ctrl Pts',(-18.1065797448196,51.2062190542739,124.170249228209)) ;
#88439=CARTESIAN_POINT('Ctrl Pts',(-17.9953654455778,51.2161234589477,123.934908116965)) ;
#88440=CARTESIAN_POINT('Ctrl Pts',(-17.925826600637,51.2261834534267,123.679876469333)) ;
#88441=CARTESIAN_POINT('Ctrl Pts',(-17.9019091868143,51.2360320753965,123.422152612981)) ;
#88442=CARTESIAN_POINT('Ctrl Pts',(-17.9229023529744,51.2460625148083,123.15941586086)) ;
#88443=CARTESIAN_POINT('Ctrl Pts',(-17.9895839704234,51.2560722304431,122.904933300777)) ;
#88444=CARTESIAN_POINT('Ctrl Pts',(-18.0981009034146,51.2659829831357,122.668199754966)) ;
#88445=CARTESIAN_POINT('Ctrl Pts',(-18.2458319639415,51.2759122560821,122.453101902059)) ;
#88446=CARTESIAN_POINT('Ctrl Pts',(-18.4308984169478,51.2859549474748,122.264969338689)) ;
#88447=CARTESIAN_POINT('Ctrl Pts',(-18.6424005039535,51.2958414806923,122.114056148567)) ;
#88448=CARTESIAN_POINT('Ctrl Pts',(-18.8792033416488,51.3058346256243,122.000563484601)) ;
#88449=CARTESIAN_POINT('Ctrl Pts',(-19.1309552845419,51.3157803064608,121.930339339444)) ;
#88450=CARTESIAN_POINT('Ctrl Pts',(-19.3910775718894,51.3257275636094,121.904356869132)) ;
#88451=CARTESIAN_POINT('Ctrl Pts',(-19.6543533589848,51.3357754674813,121.924427076619)) ;
#88452=CARTESIAN_POINT('Ctrl Pts',(-19.9051120288232,51.3456231665793,121.988392795178)) ;
#88453=CARTESIAN_POINT('Ctrl Pts',(-20.144008897239,51.355584657558,122.095399647996)) ;
#88454=CARTESIAN_POINT('Ctrl Pts',(-20.3619945141337,51.3656141199719,122.24356719647)) ;
#88455=CARTESIAN_POINT('Ctrl Pts',(-20.5487308944332,51.3755213510718,122.424986082512)) ;
#88456=CARTESIAN_POINT('Ctrl Pts',(-20.7021540436023,51.3854677297493,122.636582411564)) ;
#88457=CARTESIAN_POINT('Ctrl Pts',(-20.8172786899295,51.3954724985581,122.872977021104)) ;
#88458=CARTESIAN_POINT('Ctrl Pts',(-20.889429832364,51.4054936195783,123.126239425325)) ;
#88459=CARTESIAN_POINT('Ctrl Pts',(-20.9164566681768,51.4153844854309,123.384761481474)) ;
#88460=CARTESIAN_POINT('Ctrl Pts',(-20.8983887932973,51.4253752941902,123.646672004827)) ;
#88461=CARTESIAN_POINT('Ctrl Pts',(-20.835318400747,51.4353259523705,123.900458111221)) ;
#88462=CARTESIAN_POINT('Ctrl Pts',(-20.7296282507546,51.4452621620126,124.139202828454)) ;
#88463=CARTESIAN_POINT('Ctrl Pts',(-20.5836546019347,51.4552453287375,124.357227797165)) ;
#88464=CARTESIAN_POINT('Ctrl Pts',(-20.4006303942084,51.4652891259478,124.547361584233)) ;
#88465=CARTESIAN_POINT('Ctrl Pts',(-20.192254850081,51.4751173421161,124.700025669877)) ;
#88466=CARTESIAN_POINT('Ctrl Pts',(-19.9548227665226,51.4851939095853,124.81714527759)) ;
#88467=CARTESIAN_POINT('Ctrl Pts',(-19.7062541409025,51.4950459952747,124.889764801909)) ;
#88468=CARTESIAN_POINT('Ctrl Pts',(-19.4431990726262,51.5051192626801,124.918970553885)) ;
#88469=CARTESIAN_POINT('Ctrl Pts',(-19.1850914917787,51.5149606791037,124.902372431121)) ;
#88470=CARTESIAN_POINT('Ctrl Pts',(-18.9305244646705,51.5249219372464,124.841424401148)) ;
#88471=CARTESIAN_POINT('Ctrl Pts',(-18.6887877930121,51.5349586136784,124.735942523709)) ;
#88472=CARTESIAN_POINT('Ctrl Pts',(-18.4722292764915,51.5448372215422,124.592733444186)) ;
#88473=CARTESIAN_POINT('Ctrl Pts',(-18.2803671864941,51.554897450181,124.410900084706)) ;
#88474=CARTESIAN_POINT('Ctrl Pts',(-18.1259134655434,51.5647644343418,124.202585813997)) ;
#88475=CARTESIAN_POINT('Ctrl Pts',(-18.0079247984675,51.5747700005945,123.96764851309)) ;
#88476=CARTESIAN_POINT('Ctrl Pts',(-17.9327258735387,51.5847537890091,123.716244471843)) ;
#88477=CARTESIAN_POINT('Ctrl Pts',(-17.9024259130523,51.5947996458117,123.454016015245)) ;
#88478=CARTESIAN_POINT('Ctrl Pts',(-17.917439480721,51.6046255230277,123.196237952779)) ;
#88479=CARTESIAN_POINT('Ctrl Pts',(-17.9771454730441,51.614615998869,122.940577894991)) ;
#88480=CARTESIAN_POINT('Ctrl Pts',(-18.0815215144472,51.6246595747678,122.698158310666)) ;
#88481=CARTESIAN_POINT('Ctrl Pts',(-18.2227516785276,51.6344813670658,122.482120314041)) ;
#88482=CARTESIAN_POINT('Ctrl Pts',(-18.40270986864,51.6445163326917,122.289358503398)) ;
#88483=CARTESIAN_POINT('Ctrl Pts',(-18.6136393360001,51.6545412496248,122.13151278075)) ;
#88484=CARTESIAN_POINT('Ctrl Pts',(-18.8444580637235,51.6643931880009,122.014234397312)) ;
#88485=CARTESIAN_POINT('Ctrl Pts',(-19.0954754548516,51.6743841640256,121.9373786769)) ;
#88486=CARTESIAN_POINT('Ctrl Pts',(-19.3541618616858,51.6843019848293,121.905328500858)) ;
#88487=CARTESIAN_POINT('Ctrl Pts',(-19.617334158459,51.6943307053939,121.918784864329)) ;
#88488=CARTESIAN_POINT('Ctrl Pts',(-19.8705294306841,51.7042136320031,121.976713058442)) ;
#88489=CARTESIAN_POINT('Ctrl Pts',(-20.1128710137296,51.7142179171226,122.078557970596)) ;
#88490=CARTESIAN_POINT('Ctrl Pts',(-20.3334390737872,51.7242015983304,122.220706430317)) ;
#88491=CARTESIAN_POINT('Ctrl Pts',(-20.526827334217,51.7342425970603,122.400195572372)) ;
#88492=CARTESIAN_POINT('Ctrl Pts',(-20.6831082514724,51.7440750419275,122.60596620502)) ;
#88493=CARTESIAN_POINT('Ctrl Pts',(-20.8039234261917,51.7540700403578,122.839180993671)) ;
#88494=CARTESIAN_POINT('Ctrl Pts',(-20.8821642141018,51.7641015891074,123.090935669259)) ;
#88495=CARTESIAN_POINT('Ctrl Pts',(-20.915271599229,51.7739669674129,123.348051007155)) ;
#88496=CARTESIAN_POINT('Ctrl Pts',(-20.9038525681082,51.7839288148732,123.609596824492)) ;
#88497=CARTESIAN_POINT('Ctrl Pts',(-20.8463633745007,51.7939637556874,123.866947061797)) ;
#88498=CARTESIAN_POINT('Ctrl Pts',(-20.7469611887257,51.8038487167046,124.106982513468)) ;
#88499=CARTESIAN_POINT('Ctrl Pts',(-20.6048348390858,51.8139143256234,124.330017808425)) ;
#88500=CARTESIAN_POINT('Ctrl Pts',(-20.4302962655908,51.8237535006651,124.520838097593)) ;
#88501=CARTESIAN_POINT('Ctrl Pts',(-20.2209018146829,51.833816056165,124.682277389154)) ;
#88502=CARTESIAN_POINT('Ctrl Pts',(-19.9903358407335,51.843713230858,124.802662438006)) ;
#88503=CARTESIAN_POINT('Ctrl Pts',(-19.7418135968401,51.8536439457813,124.882280836008)) ;
#88504=CARTESIAN_POINT('Ctrl Pts',(-19.4802517626863,51.8636879738589,124.917639362177)) ;
#88505=CARTESIAN_POINT('Ctrl Pts',(-19.2206361067492,51.8735741757122,124.907413635339)) ;
#88506=CARTESIAN_POINT('Ctrl Pts',(-18.9639533078119,51.8835673421791,124.852066742979)) ;
#88507=CARTESIAN_POINT('Ctrl Pts',(-18.7220007871068,51.8935068131662,124.753573074232)) ;
#88508=CARTESIAN_POINT('Ctrl Pts',(-18.4991343218233,51.9035233275204,124.613563016952)) ;
#88509=CARTESIAN_POINT('Ctrl Pts',(-18.3054534957154,51.9134533539972,124.438628708333)) ;
#88510=CARTESIAN_POINT('Ctrl Pts',(-18.1432387360808,51.9235058895067,124.230157322887)) ;
#88511=CARTESIAN_POINT('Ctrl Pts',(-18.02207359166,51.9333522927264,124.001515921378)) ;
#88512=CARTESIAN_POINT('Ctrl Pts',(-17.9407164669733,51.9433143355804,123.752702026381)) ;
#88513=CARTESIAN_POINT('Ctrl Pts',(-17.9038854280585,51.9533428863711,123.491731120395)) ;
#88514=CARTESIAN_POINT('Ctrl Pts',(-17.912731672611,51.9632532120887,123.231460267867)) ;
#88515=CARTESIAN_POINT('Ctrl Pts',(-17.966105221735,51.9731881239183,122.975886847945)) ;
#88516=CARTESIAN_POINT('Ctrl Pts',(-18.0642983867156,51.9832291306864,122.730978652853)) ;
#88517=CARTESIAN_POINT('Ctrl Pts',(-18.2012613019034,51.9931167635186,122.510155194213)) ;
#88518=CARTESIAN_POINT('Ctrl Pts',(-18.3759219646091,52.0031071946166,122.314162879866)) ;
#88519=CARTESIAN_POINT('Ctrl Pts',(-18.5813424888858,52.0130626311739,122.152141812982)) ;
#88520=CARTESIAN_POINT('Ctrl Pts',(-18.8104988520299,52.0229735792732,122.028393562061)) ;
#88521=CARTESIAN_POINT('Ctrl Pts',(-19.0601248152919,52.0329856553709,121.945174289692)) ;
#88522=CARTESIAN_POINT('Ctrl Pts',(-19.3208342889526,52.0430129774459,121.907035972771)) ;
#88523=CARTESIAN_POINT('Ctrl Pts',(-19.5798702658014,52.0528717524,121.913965038983)) ;
#88524=CARTESIAN_POINT('Ctrl Pts',(-19.9254189752122,52.0662979452124,121.984776021455)) ;
#88525=CARTESIAN_POINT('Ctrl Pts',(-20.2369069489131,52.0793819609939,122.139699278538)) ;
#88526=CARTESIAN_POINT('Ctrl Pts',(-20.5025007000134,52.0928554097491,122.373739586692)) ;
#88527=CARTESIAN_POINT('Ctrl Pts',(-20.663502478955,52.1026883675549,122.575893701772)) ;
#88528=CARTESIAN_POINT('Ctrl Pts',(-20.7895447714591,52.1126516410056,122.80536324698)) ;
#88529=CARTESIAN_POINT('Ctrl Pts',(-20.8739174433946,52.1226887148236,123.055264793137)) ;
#88530=CARTESIAN_POINT('Ctrl Pts',(-20.913466812998,52.1325637178352,123.311769299998)) ;
#88531=CARTESIAN_POINT('Ctrl Pts',(-20.907759863983,52.1426313974614,123.576238886036)) ;
#88532=CARTESIAN_POINT('Ctrl Pts',(-20.8575136474615,52.1524722476791,123.829949405008)) ;
#88533=CARTESIAN_POINT('Ctrl Pts',(-20.7314604670083,52.1658084461551,124.156927153833)) ;
#88534=CARTESIAN_POINT('Ctrl Pts',(-20.5246587062285,52.1790259699695,124.440942087782)) ;
#88535=CARTESIAN_POINT('Ctrl Pts',(-20.2524006445835,52.1923608964608,124.661535277277)) ;
#88536=CARTESIAN_POINT('Ctrl Pts',(-20.0229908221438,52.2023439970554,124.788885516254)) ;
#88537=CARTESIAN_POINT('Ctrl Pts',(-19.7733578676333,52.212388772955,124.874606471109)) ;
#88538=CARTESIAN_POINT('Ctrl Pts',(-19.5185625305117,52.2222066961409,124.91526712013)) ;
#88539=CARTESIAN_POINT('Ctrl Pts',(-19.2545108614186,52.2322560100963,124.911509845062)) ;
#88540=CARTESIAN_POINT('Ctrl Pts',(-18.9112692834644,52.2455597507188,124.845226243308)) ;
#88541=CARTESIAN_POINT('Ctrl Pts',(-18.5163692561841,52.2620499461955,124.6549048869)) ;
#88542=CARTESIAN_POINT('Ctrl Pts',(-18.2061367720864,52.2787691111201,124.336934261931)) ;
#88543=CARTESIAN_POINT('Ctrl Pts',(-18.0368883651409,52.2919301047903,124.035235554106)) ;
#88544=CARTESIAN_POINT('Ctrl Pts',(-17.9492083451138,52.3019263268955,123.78763251036)) ;
#88545=CARTESIAN_POINT('Ctrl Pts',(-17.9063157112242,52.3119501664292,123.527728946304)) ;
#88546=CARTESIAN_POINT('Ctrl Pts',(-17.9093488352234,52.3251434884225,123.181008469196)) ;
#88547=CARTESIAN_POINT('Ctrl Pts',(-18.0271239216375,52.3418026601998,122.754229453944)) ;
#88548=CARTESIAN_POINT('Ctrl Pts',(-18.3339431995994,52.3617128356855,122.323055504623)) ;
#88549=CARTESIAN_POINT('Ctrl Pts',(-18.7684450300349,52.3816028235299,122.021837292416)) ;
#88550=CARTESIAN_POINT('Ctrl Pts',(-19.2825994094008,52.4016082715447,121.886694009092)) ;
#88551=CARTESIAN_POINT('Ctrl Pts',(-19.8078170341868,52.421444665572,121.934185674863)) ;
#88552=CARTESIAN_POINT('Ctrl Pts',(-20.289256959109,52.4414524594687,122.159679285256)) ;
#88553=CARTESIAN_POINT('Ctrl Pts',(-20.6617455226346,52.4612790957627,122.532558034168)) ;
#88554=CARTESIAN_POINT('Ctrl Pts',(-20.8871676648136,52.4812580387165,123.013320567925)) ;
#88555=CARTESIAN_POINT('Ctrl Pts',(-20.9339425757462,52.5011898405856,123.540934620001)) ;
#88556=CARTESIAN_POINT('Ctrl Pts',(-20.8002546271562,52.5210141410831,124.050758632293)) ;
#88557=CARTESIAN_POINT('Ctrl Pts',(-20.495952731629,52.5411101424229,124.489450915891)) ;
#88558=CARTESIAN_POINT('Ctrl Pts',(-20.0674306833606,52.5608685585269,124.793545669361)) ;
#88559=CARTESIAN_POINT('Ctrl Pts',(-19.5529252626636,52.580962251411,124.935529369241)) ;
#88560=CARTESIAN_POINT('Ctrl Pts',(-19.2053368719646,52.5940732173177,124.907896808842)) ;
#88561=CARTESIAN_POINT('Ctrl Pts',(-19.0351230767564,52.6007865921055,124.864328531831)) ;
#88562=CARTESIAN_POINT('',(-20.0093941796458,13.5522956097346,122.037202589381)) ;
#88563=CARTESIAN_POINT('Ctrl Pts',(-20.8811762570041,12.5498512937297,123.700066866625)) ;
#88564=CARTESIAN_POINT('Ctrl Pts',(-20.8692620836651,12.5522145745311,123.760777799691)) ;
#88565=CARTESIAN_POINT('Ctrl Pts',(-20.8316080708744,12.5579111037291,123.905360901057)) ;
#88566=CARTESIAN_POINT('Ctrl Pts',(-20.7388385515527,12.5668945320791,124.122491967746)) ;
#88567=CARTESIAN_POINT('Ctrl Pts',(-20.5941950356551,12.5769520351743,124.343654958997)) ;
#88568=CARTESIAN_POINT('Ctrl Pts',(-20.4178326753157,12.5867736915449,124.532143914003)) ;
#88569=CARTESIAN_POINT('Ctrl Pts',(-20.2068320884318,12.59682975421,124.691210472913)) ;
#88570=CARTESIAN_POINT('Ctrl Pts',(-19.9738765529842,12.6067704189132,124.809442393321)) ;
#88571=CARTESIAN_POINT('Ctrl Pts',(-19.7250875546676,12.6166748228617,124.885930317569)) ;
#88572=CARTESIAN_POINT('Ctrl Pts',(-19.4630957051046,12.6267213078553,124.918354057249)) ;
#88573=CARTESIAN_POINT('Ctrl Pts',(-19.2033273420661,12.636617535667,124.905216890975)) ;
#88574=CARTESIAN_POINT('Ctrl Pts',(-18.9456557927353,12.6466771192305,124.846275394572)) ;
#88575=CARTESIAN_POINT('Ctrl Pts',(-18.7071089141504,12.6565291288993,124.74562108305)) ;
#88576=CARTESIAN_POINT('Ctrl Pts',(-18.4867674844916,12.6664916603389,124.604252671323)) ;
#88577=CARTESIAN_POINT('Ctrl Pts',(-18.2932471898541,12.6765232085783,124.425230066221)) ;
#88578=CARTESIAN_POINT('Ctrl Pts',(-18.1357855764971,12.6864146197913,124.218414587344)) ;
#88579=CARTESIAN_POINT('Ctrl Pts',(-18.0146947587827,12.6964308734993,123.984694568915)) ;
#88580=CARTESIAN_POINT('Ctrl Pts',(-17.9364655443542,12.706460976344,123.732995067848)) ;
#88581=CARTESIAN_POINT('Ctrl Pts',(-17.9032103304628,12.7163174252977,123.476104767026)) ;
#88582=CARTESIAN_POINT('Ctrl Pts',(-17.9149031126223,12.72631643607,123.213643474476)) ;
#88583=CARTESIAN_POINT('Ctrl Pts',(-17.9711347927928,12.736211652988,122.959716591098)) ;
#88584=CARTESIAN_POINT('Ctrl Pts',(-18.0722621730133,12.7462721683453,122.715478970838)) ;
#88585=CARTESIAN_POINT('Ctrl Pts',(-18.2111849666589,12.7561214617324,122.497067612659)) ;
#88586=CARTESIAN_POINT('Ctrl Pts',(-18.3885653163835,12.7661486374124,122.30221638746)) ;
#88587=CARTESIAN_POINT('Ctrl Pts',(-18.5975514154094,12.7761772130396,122.141639073802)) ;
#88588=CARTESIAN_POINT('Ctrl Pts',(-18.8267178958733,12.7860223065854,122.021590045095)) ;
#88589=CARTESIAN_POINT('Ctrl Pts',(-19.0767118104658,12.7960135480172,121.94132806078)) ;
#88590=CARTESIAN_POINT('Ctrl Pts',(-19.3380817266942,12.8060493291605,121.906076455516)) ;
#88591=CARTESIAN_POINT('Ctrl Pts',(-19.596780887396,12.8159015348902,121.916202048577)) ;
#88592=CARTESIAN_POINT('Ctrl Pts',(-19.8527792150898,12.8258636290072,121.970959750396)) ;
#88593=CARTESIAN_POINT('Ctrl Pts',(-20.0967365608284,12.8358861898343,122.070232238452)) ;
#88594=CARTESIAN_POINT('Ctrl Pts',(-20.3178000252107,12.8458139614859,122.208825541157)) ;
#88595=CARTESIAN_POINT('Ctrl Pts',(-20.5136248486434,12.8558563456107,122.38570732732)) ;
#88596=CARTESIAN_POINT('Ctrl Pts',(-20.6733958132101,12.8657455696813,122.590690688902)) ;
#88597=CARTESIAN_POINT('Ctrl Pts',(-20.7968031363708,12.8757348178486,122.822371490678)) ;
#88598=CARTESIAN_POINT('Ctrl Pts',(-20.8776695418149,12.8856933948906,123.071257865387)) ;
#88599=CARTESIAN_POINT('Ctrl Pts',(-20.9145160925794,12.8955929639819,123.328801889037)) ;
#88600=CARTESIAN_POINT('Ctrl Pts',(-20.9058665992661,12.9056408760659,123.592681474373)) ;
#88601=CARTESIAN_POINT('Ctrl Pts',(-20.8525411197741,12.9155362303731,123.847236588034)) ;
#88602=CARTESIAN_POINT('Ctrl Pts',(-20.7542629977426,12.9255978808643,124.092671346512)) ;
#88603=CARTESIAN_POINT('Ctrl Pts',(-20.6178824497922,12.9354424963268,124.312521389387)) ;
#88604=CARTESIAN_POINT('Ctrl Pts',(-20.4440872979319,12.9454025752282,124.508228135365)) ;
#88605=CARTESIAN_POINT('Ctrl Pts',(-20.2370284211193,12.9554407695865,124.671653791003)) ;
#88606=CARTESIAN_POINT('Ctrl Pts',(-20.008735431722,12.9653144849861,124.795042874335)) ;
#88607=CARTESIAN_POINT('Ctrl Pts',(-19.7576063109488,12.9753861945204,124.878511544747)) ;
#88608=CARTESIAN_POINT('Ctrl Pts',(-19.5019831838198,12.9852186349729,124.916346652394)) ;
#88609=CARTESIAN_POINT('Ctrl Pts',(-19.2384448043294,12.9952504558983,124.909813965164)) ;
#88610=CARTESIAN_POINT('Ctrl Pts',(-18.9804789488314,13.0052708257839,124.856943439991)) ;
#88611=CARTESIAN_POINT('Ctrl Pts',(-18.7391020985709,13.0151375969176,124.762195065093)) ;
#88612=CARTESIAN_POINT('Ctrl Pts',(-18.5133119731303,13.025208368107,124.624195283185)) ;
#88613=CARTESIAN_POINT('Ctrl Pts',(-18.3193460395093,13.0350515286286,124.453039947988)) ;
#88614=CARTESIAN_POINT('Ctrl Pts',(-18.1551409871327,13.045031761815,124.248545739038)) ;
#88615=CARTESIAN_POINT('Ctrl Pts',(-18.0288968334375,13.0550502818502,124.01751953666)) ;
#88616=CARTESIAN_POINT('Ctrl Pts',(-17.9452843626105,13.0649335902339,123.771589310434)) ;
#88617=CARTESIAN_POINT('Ctrl Pts',(-17.9050279627347,13.0750018744047,123.510130021932)) ;
#88618=CARTESIAN_POINT('Ctrl Pts',(-17.9103427016909,13.0848320010723,123.251814495464)) ;
#88619=CARTESIAN_POINT('Ctrl Pts',(-17.9612809092981,13.0948985732789,122.992269532793)) ;
#88620=CARTESIAN_POINT('Ctrl Pts',(-18.0550171292814,13.1047887295196,122.749822905915)) ;
#88621=CARTESIAN_POINT('Ctrl Pts',(-18.1903054658587,13.114781257096,122.524782428398)) ;
#88622=CARTESIAN_POINT('Ctrl Pts',(-18.3622584156365,13.1247427469703,122.327401305476)) ;
#88623=CARTESIAN_POINT('Ctrl Pts',(-18.5644359884156,13.1346519688575,122.163265725879)) ;
#88624=CARTESIAN_POINT('Ctrl Pts',(-18.7952652342093,13.1447005486678,122.035044644749)) ;
#88625=CARTESIAN_POINT('Ctrl Pts',(-19.0407361930169,13.1545835231379,121.950173803814)) ;
#88626=CARTESIAN_POINT('Ctrl Pts',(-19.3000068336127,13.1645784342806,121.908192940554)) ;
#88627=CARTESIAN_POINT('Ctrl Pts',(-19.5633186687248,13.1745988208542,121.912239958628)) ;
#88628=CARTESIAN_POINT('Ctrl Pts',(-19.8190763964686,13.1845089247113,121.961246286646)) ;
#88629=CARTESIAN_POINT('Ctrl Pts',(-20.0631402215822,13.1944366369212,122.053450497386)) ;
#88630=CARTESIAN_POINT('Ctrl Pts',(-20.2899638294564,13.2044797466884,122.188360062557)) ;
#88631=CARTESIAN_POINT('Ctrl Pts',(-20.4869257177344,13.214366167144,122.35780741445)) ;
#88632=CARTESIAN_POINT('Ctrl Pts',(-20.6535775719235,13.2243593447496,122.560745126669)) ;
#88633=CARTESIAN_POINT('Ctrl Pts',(-20.781768758078,13.2343050076535,122.788511159415)) ;
#88634=CARTESIAN_POINT('Ctrl Pts',(-20.8689866491185,13.2442523038587,123.034949721076)) ;
#88635=CARTESIAN_POINT('Ctrl Pts',(-20.9122331010744,13.2543000694366,123.295421612396)) ;
#88636=CARTESIAN_POINT('Ctrl Pts',(-20.9098535935215,13.2641482826542,123.554208720169)) ;
#88637=CARTESIAN_POINT('Ctrl Pts',(-20.862891829645,13.2741078554483,123.811687555265)) ;
#88638=CARTESIAN_POINT('Ctrl Pts',(-20.7708019573289,13.2841444764808,124.058831482253)) ;
#88639=CARTESIAN_POINT('Ctrl Pts',(-20.6396072016662,13.2940249912912,124.282931024446)) ;
#88640=CARTESIAN_POINT('Ctrl Pts',(-20.4686846093292,13.3040776425982,124.484308739774)) ;
#88641=CARTESIAN_POINT('Ctrl Pts',(-20.2685764087636,13.3139730408782,124.650446241866)) ;
#88642=CARTESIAN_POINT('Ctrl Pts',(-20.0392572485433,13.3240231625843,124.781393384691)) ;
#88643=CARTESIAN_POINT('Ctrl Pts',(-19.7947435724965,13.3339074421262,124.869123479395)) ;
#88644=CARTESIAN_POINT('Ctrl Pts',(-19.5359835923959,13.3439022234181,124.914032922456)) ;
#88645=CARTESIAN_POINT('Ctrl Pts',(-19.2745480154649,13.3538500686049,124.913233748315)) ;
#88646=CARTESIAN_POINT('Ctrl Pts',(-19.0174771736584,13.3637870319923,124.867483970433)) ;
#88647=CARTESIAN_POINT('Ctrl Pts',(-18.770953528208,13.3737699967295,124.777666914607)) ;
#88648=CARTESIAN_POINT('Ctrl Pts',(-18.5426825818329,13.3838138481452,124.645222231553)) ;
#88649=CARTESIAN_POINT('Ctrl Pts',(-18.3447626868737,13.3936420494799,124.479227338155)) ;
#88650=CARTESIAN_POINT('Ctrl Pts',(-18.174439114941,13.403718622078,124.276543144147)) ;
#88651=CARTESIAN_POINT('Ctrl Pts',(-18.0446799079283,13.4135707020855,124.052439270463)) ;
#88652=CARTESIAN_POINT('Ctrl Pts',(-17.9536328215657,13.4236439870896,123.803921128187)) ;
#88653=CARTESIAN_POINT('Ctrl Pts',(-17.908245672822,13.4334853388001,123.549293611183)) ;
#88654=CARTESIAN_POINT('Ctrl Pts',(-17.9067874767793,13.4434468381966,123.287535568875)) ;
#88655=CARTESIAN_POINT('Ctrl Pts',(-17.9515894545495,13.4534826143266,123.027629899913)) ;
#88656=CARTESIAN_POINT('Ctrl Pts',(-18.0392686443259,13.4633710409642,122.783013986504)) ;
#88657=CARTESIAN_POINT('Ctrl Pts',(-18.1693153244225,13.4733863630391,122.554183172307)) ;
#88658=CARTESIAN_POINT('Ctrl Pts',(-18.3378376719635,13.4834167119393,122.35150318048)) ;
#88659=CARTESIAN_POINT('Ctrl Pts',(-18.5349010784944,13.493260087546,122.183945153477)) ;
#88660=CARTESIAN_POINT('Ctrl Pts',(-18.761992836842,13.5032895244431,122.050165209368)) ;
#88661=CARTESIAN_POINT('Ctrl Pts',(-19.0091803607605,13.513321402376,121.958500067657)) ;
#88662=CARTESIAN_POINT('Ctrl Pts',(-19.2631820189547,13.5231510254815,121.911588708017)) ;
#88663=CARTESIAN_POINT('Ctrl Pts',(-19.5256857167379,13.5331404966346,121.908671418978)) ;
#88664=CARTESIAN_POINT('Ctrl Pts',(-19.7794742643537,13.5429325945739,121.95117720022)) ;
#88665=CARTESIAN_POINT('Ctrl Pts',(-19.9360895547681,13.5492395742091,122.005136428262)) ;
#88666=CARTESIAN_POINT('Ctrl Pts',(-20.0093941796458,13.5522956097346,122.037202589381)) ;
#88667=CARTESIAN_POINT('Ctrl Pts',(-19.3053878987309,13.6947924674762,122.201356690921)) ;
#88668=CARTESIAN_POINT('Ctrl Pts',(-19.356349637348,13.6822848109803,122.171875951815)) ;
#88669=CARTESIAN_POINT('Ctrl Pts',(-19.4101184737497,13.6698676303486,122.14590971193)) ;
#88670=CARTESIAN_POINT('Ctrl Pts',(-19.5160286269017,13.6467016771096,122.104119584246)) ;
#88671=CARTESIAN_POINT('Ctrl Pts',(-19.5746444702855,13.6345804393052,122.08517512299)) ;
#88672=CARTESIAN_POINT('Ctrl Pts',(-19.7010870355378,13.6094612987591,122.056219247648)) ;
#88673=CARTESIAN_POINT('Ctrl Pts',(-19.7611384259661,13.5978109265327,122.046461245458)) ;
#88674=CARTESIAN_POINT('Ctrl Pts',(-19.8838264753735,13.5747381235504,122.035109517786)) ;
#88675=CARTESIAN_POINT('Ctrl Pts',(-19.9460097293868,13.5635055402564,122.033994044163)) ;
#88676=CARTESIAN_POINT('Ctrl Pts',(-20.0093941796457,13.5522956097346,122.037202589381)) ;
#88677=CARTESIAN_POINT('Ctrl Pts',(-20.8283360085486,11.7999200508426,122.926058340311)) ;
#88678=CARTESIAN_POINT('Ctrl Pts',(-20.8845464538574,11.8065469016607,123.090182099353)) ;
#88679=CARTESIAN_POINT('Ctrl Pts',(-20.9394674069342,11.8197775281417,123.437524293028)) ;
#88680=CARTESIAN_POINT('Ctrl Pts',(-20.8387914871724,11.8397531494004,123.958813977782)) ;
#88681=CARTESIAN_POINT('Ctrl Pts',(-20.5666784354472,11.8596704843023,124.412866308854)) ;
#88682=CARTESIAN_POINT('Ctrl Pts',(-20.1575619136445,11.8795437610183,124.747046208683)) ;
#88683=CARTESIAN_POINT('Ctrl Pts',(-19.6551371496748,11.8995682511823,124.92249916066)) ;
#88684=CARTESIAN_POINT('Ctrl Pts',(-19.1270451744641,11.919436092333,124.915907267661)) ;
#88685=CARTESIAN_POINT('Ctrl Pts',(-18.6308008607008,11.9393817432125,124.729592278927)) ;
#88686=CARTESIAN_POINT('Ctrl Pts',(-18.2288280457431,11.9592871438295,124.385624086374)) ;
#88687=CARTESIAN_POINT('Ctrl Pts',(-17.9678591535732,11.9791613716459,123.926365470291)) ;
#88688=CARTESIAN_POINT('Ctrl Pts',(-17.8787398474485,11.9991471625235,123.402691583813)) ;
#88689=CARTESIAN_POINT('Ctrl Pts',(-17.9735233382965,12.0190414051832,122.882536434516)) ;
#88690=CARTESIAN_POINT('Ctrl Pts',(-18.2387585289407,12.0389201212553,122.425519450945)) ;
#88691=CARTESIAN_POINT('Ctrl Pts',(-18.6476197278655,12.0589595710999,122.084275218605)) ;
#88692=CARTESIAN_POINT('Ctrl Pts',(-19.1441777499651,12.0788227326378,121.904537351317)) ;
#88693=CARTESIAN_POINT('Ctrl Pts',(-19.6750288445506,12.098802100652,121.904738156225)) ;
#88694=CARTESIAN_POINT('Ctrl Pts',(-20.1701856143784,12.1186126811748,122.084100255283)) ;
#88695=CARTESIAN_POINT('Ctrl Pts',(-20.5782317220315,12.1385936094604,122.423828694064)) ;
#88696=CARTESIAN_POINT('Ctrl Pts',(-20.8444525967082,12.1584862813298,122.880697423595)) ;
#88697=CARTESIAN_POINT('Ctrl Pts',(-20.9398398136422,12.1784126116169,123.401645628938)) ;
#88698=CARTESIAN_POINT('Ctrl Pts',(-20.851062860932,12.1983831657092,123.924943760388)) ;
#88699=CARTESIAN_POINT('Ctrl Pts',(-20.6345502730467,12.2149150047968,124.307289073383)) ;
#88700=CARTESIAN_POINT('Ctrl Pts',(-20.3891153931417,12.2282547436244,124.557618291671)) ;
#88701=CARTESIAN_POINT('Ctrl Pts',(-20.1744356948872,12.238286985843,124.71063155409)) ;
#88702=CARTESIAN_POINT('Ctrl Pts',(-19.9407461181023,12.2481446864865,124.82243808738)) ;
#88703=CARTESIAN_POINT('Ctrl Pts',(-19.6879479903912,12.2581365511257,124.893369098924)) ;
#88704=CARTESIAN_POINT('Ctrl Pts',(-19.4284766803744,12.2680591008858,124.919096784819)) ;
#88705=CARTESIAN_POINT('Ctrl Pts',(-19.0804161519456,12.2813368743793,124.893600455121)) ;
#88706=CARTESIAN_POINT('Ctrl Pts',(-18.7455915471493,12.2946842133199,124.776633305253)) ;
#88707=CARTESIAN_POINT('Ctrl Pts',(-18.4584578761078,12.3078914451131,124.581565716411)) ;
#88708=CARTESIAN_POINT('Ctrl Pts',(-18.2699644759195,12.3178785612028,124.39900581103)) ;
#88709=CARTESIAN_POINT('Ctrl Pts',(-18.1163990348321,12.3278294667826,124.187285865335)) ;
#88710=CARTESIAN_POINT('Ctrl Pts',(-18.0010402192528,12.33788456879,123.949600254045)) ;
#88711=CARTESIAN_POINT('Ctrl Pts',(-17.9299289800127,12.3477062421111,123.701455973458)) ;
#88712=CARTESIAN_POINT('Ctrl Pts',(-17.9019096964941,12.357764713186,123.438645136577)) ;
#88713=CARTESIAN_POINT('Ctrl Pts',(-17.9200603909808,12.3676893243625,123.178453886709)) ;
#88714=CARTESIAN_POINT('Ctrl Pts',(-18.0035385415921,12.3809666632629,122.839641054544)) ;
#88715=CARTESIAN_POINT('Ctrl Pts',(-18.1740845283454,12.3942655425005,122.530112925337)) ;
#88716=CARTESIAN_POINT('Ctrl Pts',(-18.4148347268114,12.4075044146712,122.278925757333)) ;
#88717=CARTESIAN_POINT('Ctrl Pts',(-18.626729428275,12.4175110328078,122.123187062121)) ;
#88718=CARTESIAN_POINT('Ctrl Pts',(-18.8632335737039,12.4275419778693,122.006787551109)) ;
#88719=CARTESIAN_POINT('Ctrl Pts',(-19.1118364896857,12.4373981512211,121.934037501767)) ;
#88720=CARTESIAN_POINT('Ctrl Pts',(-19.3729328187221,12.447397422184,121.904821743981)) ;
#88721=CARTESIAN_POINT('Ctrl Pts',(-19.6324990778504,12.4572918739413,121.920913539679)) ;
#88722=CARTESIAN_POINT('Ctrl Pts',(-19.8895297331301,12.4673551897507,121.982929816623)) ;
#88723=CARTESIAN_POINT('Ctrl Pts',(-20.1266869407979,12.4771940464903,122.086036295395)) ;
#88724=CARTESIAN_POINT('Ctrl Pts',(-20.3474074551281,12.4872601683079,122.231757371538)) ;
#88725=CARTESIAN_POINT('Ctrl Pts',(-20.5359559653956,12.4971433960322,122.410425895404)) ;
#88726=CARTESIAN_POINT('Ctrl Pts',(-20.6927050538892,12.5071328573109,122.620969850052)) ;
#88727=CARTESIAN_POINT('Ctrl Pts',(-20.810144830431,12.5170965677374,122.855005173606)) ;
#88728=CARTESIAN_POINT('Ctrl Pts',(-20.8856671720647,12.5270915704683,123.106592117066)) ;
#88729=CARTESIAN_POINT('Ctrl Pts',(-20.916070552576,12.5371279014786,123.36856478643)) ;
#88730=CARTESIAN_POINT('Ctrl Pts',(-20.9012433064245,12.5469741308209,123.62690469604)) ;
#88731=CARTESIAN_POINT('Ctrl Pts',(-20.8414337010136,12.5569596290961,123.882363589347)) ;
#88732=CARTESIAN_POINT('Ctrl Pts',(-20.7388385515527,12.5668945320791,124.122491967746)) ;
#88733=CARTESIAN_POINT('Ctrl Pts',(-20.5941950356551,12.5769520351743,124.343654958997)) ;
#88734=CARTESIAN_POINT('Ctrl Pts',(-20.4178326753157,12.5867736915449,124.532143914003)) ;
#88735=CARTESIAN_POINT('Ctrl Pts',(-20.2068320884318,12.59682975421,124.691210472913)) ;
#88736=CARTESIAN_POINT('Ctrl Pts',(-19.9738765529842,12.6067704189132,124.809442393321)) ;
#88737=CARTESIAN_POINT('Ctrl Pts',(-19.7250875546676,12.6166748228617,124.885930317569)) ;
#88738=CARTESIAN_POINT('Ctrl Pts',(-19.4630957051046,12.6267213078553,124.918354057249)) ;
#88739=CARTESIAN_POINT('Ctrl Pts',(-19.2033273420661,12.636617535667,124.905216890975)) ;
#88740=CARTESIAN_POINT('Ctrl Pts',(-18.9456557927353,12.6466771192305,124.846275394572)) ;
#88741=CARTESIAN_POINT('Ctrl Pts',(-18.7071089141504,12.6565291288993,124.74562108305)) ;
#88742=CARTESIAN_POINT('Ctrl Pts',(-18.4867674844916,12.6664916603389,124.604252671323)) ;
#88743=CARTESIAN_POINT('Ctrl Pts',(-18.2932471898541,12.6765232085783,124.425230066221)) ;
#88744=CARTESIAN_POINT('Ctrl Pts',(-18.1357855764971,12.6864146197913,124.218414587344)) ;
#88745=CARTESIAN_POINT('Ctrl Pts',(-18.0146947587827,12.6964308734993,123.984694568915)) ;
#88746=CARTESIAN_POINT('Ctrl Pts',(-17.9364655443542,12.706460976344,123.732995067848)) ;
#88747=CARTESIAN_POINT('Ctrl Pts',(-17.9032103304628,12.7163174252977,123.476104767026)) ;
#88748=CARTESIAN_POINT('Ctrl Pts',(-17.9149031126223,12.72631643607,123.213643474476)) ;
#88749=CARTESIAN_POINT('Ctrl Pts',(-17.9711347927928,12.736211652988,122.959716591098)) ;
#88750=CARTESIAN_POINT('Ctrl Pts',(-18.0722621730133,12.7462721683453,122.715478970838)) ;
#88751=CARTESIAN_POINT('Ctrl Pts',(-18.2111849666589,12.7561214617324,122.497067612659)) ;
#88752=CARTESIAN_POINT('Ctrl Pts',(-18.3885653163835,12.7661486374124,122.30221638746)) ;
#88753=CARTESIAN_POINT('Ctrl Pts',(-18.5975514154094,12.7761772130396,122.141639073802)) ;
#88754=CARTESIAN_POINT('Ctrl Pts',(-18.8267178958733,12.7860223065854,122.021590045095)) ;
#88755=CARTESIAN_POINT('Ctrl Pts',(-19.0767118104658,12.7960135480172,121.94132806078)) ;
#88756=CARTESIAN_POINT('Ctrl Pts',(-19.3380817266942,12.8060493291605,121.906076455516)) ;
#88757=CARTESIAN_POINT('Ctrl Pts',(-19.596780887396,12.8159015348902,121.916202048577)) ;
#88758=CARTESIAN_POINT('Ctrl Pts',(-19.8527792150898,12.8258636290072,121.970959750396)) ;
#88759=CARTESIAN_POINT('Ctrl Pts',(-20.0967365608284,12.8358861898343,122.070232238452)) ;
#88760=CARTESIAN_POINT('Ctrl Pts',(-20.3178000252107,12.8458139614859,122.208825541157)) ;
#88761=CARTESIAN_POINT('Ctrl Pts',(-20.5136248486434,12.8558563456107,122.38570732732)) ;
#88762=CARTESIAN_POINT('Ctrl Pts',(-20.67339581321,12.8657455696813,122.590690688902)) ;
#88763=CARTESIAN_POINT('Ctrl Pts',(-20.7968031363708,12.8757348178486,122.822371490678)) ;
#88764=CARTESIAN_POINT('Ctrl Pts',(-20.8776695418149,12.8856933948906,123.071257865387)) ;
#88765=CARTESIAN_POINT('Ctrl Pts',(-20.9145160925794,12.8955929639819,123.328801889037)) ;
#88766=CARTESIAN_POINT('Ctrl Pts',(-20.9058665992661,12.9056408760659,123.592681474373)) ;
#88767=CARTESIAN_POINT('Ctrl Pts',(-20.8525411197741,12.9155362303731,123.847236588034)) ;
#88768=CARTESIAN_POINT('Ctrl Pts',(-20.7542629977425,12.9255978808643,124.092671346512)) ;
#88769=CARTESIAN_POINT('Ctrl Pts',(-20.6178824497922,12.9354424963268,124.312521389387)) ;
#88770=CARTESIAN_POINT('Ctrl Pts',(-20.4440872979319,12.9454025752282,124.508228135365)) ;
#88771=CARTESIAN_POINT('Ctrl Pts',(-20.2370284211193,12.9554407695865,124.671653791003)) ;
#88772=CARTESIAN_POINT('Ctrl Pts',(-20.008735431722,12.9653144849861,124.795042874335)) ;
#88773=CARTESIAN_POINT('Ctrl Pts',(-19.7576063109488,12.9753861945204,124.878511544747)) ;
#88774=CARTESIAN_POINT('Ctrl Pts',(-19.5019831838198,12.9852186349729,124.916346652394)) ;
#88775=CARTESIAN_POINT('Ctrl Pts',(-19.2384448043294,12.9952504558983,124.909813965164)) ;
#88776=CARTESIAN_POINT('Ctrl Pts',(-18.9804789488314,13.0052708257839,124.856943439991)) ;
#88777=CARTESIAN_POINT('Ctrl Pts',(-18.7391020985709,13.0151375969176,124.762195065093)) ;
#88778=CARTESIAN_POINT('Ctrl Pts',(-18.5133119731303,13.025208368107,124.624195283185)) ;
#88779=CARTESIAN_POINT('Ctrl Pts',(-18.3193460395093,13.0350515286286,124.453039947988)) ;
#88780=CARTESIAN_POINT('Ctrl Pts',(-18.1551409871327,13.045031761815,124.248545739038)) ;
#88781=CARTESIAN_POINT('Ctrl Pts',(-18.0288968334375,13.0550502818502,124.01751953666)) ;
#88782=CARTESIAN_POINT('Ctrl Pts',(-17.9452843626105,13.0649335902339,123.771589310434)) ;
#88783=CARTESIAN_POINT('Ctrl Pts',(-17.9050279627347,13.0750018744047,123.510130021932)) ;
#88784=CARTESIAN_POINT('Ctrl Pts',(-17.9103427016909,13.0848320010723,123.251814495464)) ;
#88785=CARTESIAN_POINT('Ctrl Pts',(-17.9612809092981,13.0948985732789,122.992269532793)) ;
#88786=CARTESIAN_POINT('Ctrl Pts',(-18.0550171292814,13.1047887295196,122.749822905915)) ;
#88787=CARTESIAN_POINT('Ctrl Pts',(-18.1903054658587,13.114781257096,122.524782428398)) ;
#88788=CARTESIAN_POINT('Ctrl Pts',(-18.3622584156365,13.1247427469703,122.327401305476)) ;
#88789=CARTESIAN_POINT('Ctrl Pts',(-18.5644359884156,13.1346519688575,122.163265725879)) ;
#88790=CARTESIAN_POINT('Ctrl Pts',(-18.7952652342093,13.1447005486678,122.035044644749)) ;
#88791=CARTESIAN_POINT('Ctrl Pts',(-19.0407361930169,13.1545835231379,121.950173803814)) ;
#88792=CARTESIAN_POINT('Ctrl Pts',(-19.3000068336127,13.1645784342806,121.908192940554)) ;
#88793=CARTESIAN_POINT('Ctrl Pts',(-19.5633186687248,13.1745988208542,121.912239958628)) ;
#88794=CARTESIAN_POINT('Ctrl Pts',(-19.8190763964686,13.1845089247113,121.961246286646)) ;
#88795=CARTESIAN_POINT('Ctrl Pts',(-20.0631402215822,13.1944366369212,122.053450497386)) ;
#88796=CARTESIAN_POINT('Ctrl Pts',(-20.2899638294564,13.2044797466884,122.188360062557)) ;
#88797=CARTESIAN_POINT('Ctrl Pts',(-20.4869257177344,13.214366167144,122.35780741445)) ;
#88798=CARTESIAN_POINT('Ctrl Pts',(-20.6535775719235,13.2243593447496,122.560745126669)) ;
#88799=CARTESIAN_POINT('Ctrl Pts',(-20.781768758078,13.2343050076535,122.788511159415)) ;
#88800=CARTESIAN_POINT('Ctrl Pts',(-20.8689866491185,13.2442523038587,123.034949721076)) ;
#88801=CARTESIAN_POINT('Ctrl Pts',(-20.9122331010744,13.2543000694366,123.295421612396)) ;
#88802=CARTESIAN_POINT('Ctrl Pts',(-20.9098535935215,13.2641482826542,123.554208720169)) ;
#88803=CARTESIAN_POINT('Ctrl Pts',(-20.862891829645,13.2741078554483,123.811687555265)) ;
#88804=CARTESIAN_POINT('Ctrl Pts',(-20.7708019573289,13.2841444764808,124.058831482253)) ;
#88805=CARTESIAN_POINT('Ctrl Pts',(-20.6396072016662,13.2940249912912,124.282931024446)) ;
#88806=CARTESIAN_POINT('Ctrl Pts',(-20.4686846093292,13.3040776425982,124.484308739774)) ;
#88807=CARTESIAN_POINT('Ctrl Pts',(-20.2685764087636,13.3139730408782,124.650446241866)) ;
#88808=CARTESIAN_POINT('Ctrl Pts',(-20.0392572485433,13.3240231625843,124.781393384691)) ;
#88809=CARTESIAN_POINT('Ctrl Pts',(-19.7947435724965,13.3339074421262,124.869123479395)) ;
#88810=CARTESIAN_POINT('Ctrl Pts',(-19.5359835923959,13.3439022234181,124.914032922456)) ;
#88811=CARTESIAN_POINT('Ctrl Pts',(-19.2745480154649,13.3538500686049,124.913233748315)) ;
#88812=CARTESIAN_POINT('Ctrl Pts',(-19.0174771736584,13.3637870319923,124.867483970433)) ;
#88813=CARTESIAN_POINT('Ctrl Pts',(-18.770953528208,13.3737699967295,124.777666914607)) ;
#88814=CARTESIAN_POINT('Ctrl Pts',(-18.5426825818329,13.3838138481452,124.645222231553)) ;
#88815=CARTESIAN_POINT('Ctrl Pts',(-18.3447626868737,13.3936420494799,124.479227338155)) ;
#88816=CARTESIAN_POINT('Ctrl Pts',(-18.174439114941,13.403718622078,124.276543144147)) ;
#88817=CARTESIAN_POINT('Ctrl Pts',(-18.0446799079283,13.4135707020855,124.052439270463)) ;
#88818=CARTESIAN_POINT('Ctrl Pts',(-17.9536328215657,13.4236439870896,123.803921128187)) ;
#88819=CARTESIAN_POINT('Ctrl Pts',(-17.908245672822,13.4334853388001,123.549293611183)) ;
#88820=CARTESIAN_POINT('Ctrl Pts',(-17.9067874767793,13.4434468381966,123.287535568875)) ;
#88821=CARTESIAN_POINT('Ctrl Pts',(-17.9515894545495,13.4534826143266,123.027629899913)) ;
#88822=CARTESIAN_POINT('Ctrl Pts',(-18.0392686443259,13.4633710409642,122.783013986504)) ;
#88823=CARTESIAN_POINT('Ctrl Pts',(-18.1693153244225,13.4733863630391,122.554183172307)) ;
#88824=CARTESIAN_POINT('Ctrl Pts',(-18.3378376719635,13.4834167119393,122.35150318048)) ;
#88825=CARTESIAN_POINT('Ctrl Pts',(-18.5349010784944,13.493260087546,122.183945153477)) ;
#88826=CARTESIAN_POINT('Ctrl Pts',(-18.761992836842,13.5032895244431,122.050165209368)) ;
#88827=CARTESIAN_POINT('Ctrl Pts',(-19.0091803607605,13.513321402376,121.958500067657)) ;
#88828=CARTESIAN_POINT('Ctrl Pts',(-19.2631820189547,13.5231510254815,121.911588708017)) ;
#88829=CARTESIAN_POINT('Ctrl Pts',(-19.5256857167379,13.5331404966346,121.908671418978)) ;
#88830=CARTESIAN_POINT('Ctrl Pts',(-19.7859990638554,13.543184345397,121.952270006427)) ;
#88831=CARTESIAN_POINT('Ctrl Pts',(-20.0294662569613,13.5530060509287,122.037953136693)) ;
#88832=CARTESIAN_POINT('Ctrl Pts',(-20.2595578583272,13.5630410907565,122.166795368885)) ;
#88833=CARTESIAN_POINT('Ctrl Pts',(-20.4631193550347,13.573065797648,122.334030527681)) ;
#88834=CARTESIAN_POINT('Ctrl Pts',(-20.6320196881759,13.5829185019887,122.530273988873)) ;
#88835=CARTESIAN_POINT('Ctrl Pts',(-20.7664821078402,13.5929066241964,122.755672189208)) ;
#88836=CARTESIAN_POINT('Ctrl Pts',(-20.8592301070909,13.6028350943037,122.999547591303)) ;
#88837=CARTESIAN_POINT('Ctrl Pts',(-20.9089521249442,13.6128240714709,123.257308236829)) ;
#88838=CARTESIAN_POINT('Ctrl Pts',(-20.9127323662985,13.6228618787506,123.521057016566)) ;
#88839=CARTESIAN_POINT('Ctrl Pts',(-20.8718783998989,13.6327081796139,123.776564736996)) ;
#88840=CARTESIAN_POINT('Ctrl Pts',(-20.7862945910431,13.6427339229932,124.025746367502)) ;
#88841=CARTESIAN_POINT('Ctrl Pts',(-20.6580767870656,13.6527647894322,124.256070820692)) ;
#88842=CARTESIAN_POINT('Ctrl Pts',(-20.4954356848382,13.662602148231,124.457000727745)) ;
#88843=CARTESIAN_POINT('Ctrl Pts',(-20.2977665459096,13.6725941091647,124.629841734287)) ;
#88844=CARTESIAN_POINT('Ctrl Pts',(-20.0718975262772,13.6826264717213,124.765837185899)) ;
#88845=CARTESIAN_POINT('Ctrl Pts',(-19.8300805604924,13.6924916322957,124.859254064222)) ;
#88846=CARTESIAN_POINT('Ctrl Pts',(-19.5733470333744,13.7024535368734,124.910489003739)) ;
#88847=CARTESIAN_POINT('Ctrl Pts',(-19.3097110945833,13.7124884669491,124.915979322584)) ;
#88848=CARTESIAN_POINT('Ctrl Pts',(-19.052903569064,13.7223734138028,124.876639088694)) ;
#88849=CARTESIAN_POINT('Ctrl Pts',(-18.802425491904,13.7324390901142,124.791752081939)) ;
#88850=CARTESIAN_POINT('Ctrl Pts',(-18.5755121673576,13.7422780097491,124.667718382011)) ;
#88851=CARTESIAN_POINT('Ctrl Pts',(-18.3688230223248,13.7523415194835,124.502800514481)) ;
#88852=CARTESIAN_POINT('Ctrl Pts',(-18.1969779972077,13.7622351326453,124.307654410282)) ;
#88853=CARTESIAN_POINT('Ctrl Pts',(-18.0603814063974,13.7721791394587,124.084921230377)) ;
#88854=CARTESIAN_POINT('Ctrl Pts',(-17.9638424346081,13.782180093813,123.840436569305)) ;
#88855=CARTESIAN_POINT('Ctrl Pts',(-17.9114952956979,13.7922188515053,123.581898288947)) ;
#88856=CARTESIAN_POINT('Ctrl Pts',(-17.9044097597817,13.8020430356753,123.323804444879)) ;
#88857=CARTESIAN_POINT('Ctrl Pts',(-17.942755586416,13.8121011012747,123.062308840123)) ;
#88858=CARTESIAN_POINT('Ctrl Pts',(-18.0252033616295,13.8220311480494,122.814707785698)) ;
#88859=CARTESIAN_POINT('Ctrl Pts',(-18.1490450109907,13.8319825903865,122.58437299172)) ;
#88860=CARTESIAN_POINT('Ctrl Pts',(-18.312830616674,13.8420293875658,122.377301209051)) ;
#88861=CARTESIAN_POINT('Ctrl Pts',(-18.5060204476613,13.8518773282459,122.20510405819)) ;
#88862=CARTESIAN_POINT('Ctrl Pts',(-18.7282785603277,13.8618389595885,122.066811224224)) ;
#88863=CARTESIAN_POINT('Ctrl Pts',(-18.9729559764164,13.8718676189644,121.968851551182)) ;
#88864=CARTESIAN_POINT('Ctrl Pts',(-19.2278374256175,13.8817779218526,121.915423966121)) ;
#88865=CARTESIAN_POINT('Ctrl Pts',(-19.4887668418426,13.8917128164148,121.906358743324)) ;
#88866=CARTESIAN_POINT('Ctrl Pts',(-19.7500201068666,13.9017539150817,121.943366287556)) ;
#88867=CARTESIAN_POINT('Ctrl Pts',(-19.997114009859,13.9116411975861,122.023756349265)) ;
#88868=CARTESIAN_POINT('Ctrl Pts',(-20.229100640813,13.9216329380966,122.146710775795)) ;
#88869=CARTESIAN_POINT('Ctrl Pts',(-20.435328819661,13.931583487332,122.307501482509)) ;
#88870=CARTESIAN_POINT('Ctrl Pts',(-20.610513668173,13.9415191649668,122.501085313789)) ;
#88871=CARTESIAN_POINT('Ctrl Pts',(-20.7503773911135,13.9515045827596,122.723134407814)) ;
#88872=CARTESIAN_POINT('Ctrl Pts',(-20.8496809192691,13.9615333756301,122.967254089343)) ;
#88873=CARTESIAN_POINT('Ctrl Pts',(-20.9045337829199,13.9714128868581,123.221012810142)) ;
#88874=CARTESIAN_POINT('Ctrl Pts',(-20.9152110491903,13.981406423531,123.483425425094)) ;
#88875=CARTESIAN_POINT('Ctrl Pts',(-20.8794859206276,13.9914386917948,123.744619970286)) ;
#88876=CARTESIAN_POINT('Ctrl Pts',(-20.8008196116492,14.0013026538007,123.991638075795)) ;
#88877=CARTESIAN_POINT('Ctrl Pts',(-20.6780078275285,14.0113727151456,124.226013909898)) ;
#88878=CARTESIAN_POINT('Ctrl Pts',(-20.5199890005443,14.0212150794943,124.43079250126)) ;
#88879=CARTESIAN_POINT('Ctrl Pts',(-20.3271803845075,14.0311757519968,124.607819487763)) ;
#88880=CARTESIAN_POINT('Ctrl Pts',(-20.1045706887236,14.0412138230646,124.749326629548)) ;
#88881=CARTESIAN_POINT('Ctrl Pts',(-19.8649107838462,14.051087438025,124.848860391817)) ;
#88882=CARTESIAN_POINT('Ctrl Pts',(-19.6065853682649,14.0611596726063,124.906317466992)) ;
#88883=CARTESIAN_POINT('Ctrl Pts',(-19.3486353561911,14.0709836910551,124.91805722916)) ;
#88884=CARTESIAN_POINT('Ctrl Pts',(-19.0863513066081,14.0810486120311,124.884370279709)) ;
#88885=CARTESIAN_POINT('Ctrl Pts',(-18.7548552994364,14.0942589103259,124.781024489845)) ;
#88886=CARTESIAN_POINT('Ctrl Pts',(-18.4555139703643,14.1075743570578,124.592476583949)) ;
#88887=CARTESIAN_POINT('Ctrl Pts',(-18.2182215362896,14.1208646023251,124.336059674344)) ;
#88888=CARTESIAN_POINT('Ctrl Pts',(-18.0753754053462,14.1309153519322,124.113963002068)) ;
#88889=CARTESIAN_POINT('Ctrl Pts',(-17.9751742641188,14.1407279589144,123.876319735043)) ;
#88890=CARTESIAN_POINT('Ctrl Pts',(-17.9159189092107,14.1507990569087,123.618416063707)) ;
#88891=CARTESIAN_POINT('Ctrl Pts',(-17.9028526558769,14.1606886296836,123.35883798821)) ;
#88892=CARTESIAN_POINT('Ctrl Pts',(-17.9449956703198,14.1739587364869,123.012660958945)) ;
#88893=CARTESIAN_POINT('Ctrl Pts',(-18.110043879932,14.1905754234094,122.603035428979)) ;
#88894=CARTESIAN_POINT('Ctrl Pts',(-18.4039594470265,14.2071494667256,122.274938448092)) ;
#88895=CARTESIAN_POINT('Ctrl Pts',(-18.6963137378166,14.2204460341574,122.08351795448)) ;
#88896=CARTESIAN_POINT('Ctrl Pts',(-18.9385848307681,14.2304760977348,121.979689993019)) ;
#88897=CARTESIAN_POINT('Ctrl Pts',(-19.1916875088085,14.240369989584,121.920298097705)) ;
#88898=CARTESIAN_POINT('Ctrl Pts',(-19.5394066171243,14.2536227453696,121.899565963118)) ;
#88899=CARTESIAN_POINT('Ctrl Pts',(-19.9747350131759,14.270350850362,121.989580778364)) ;
#88900=CARTESIAN_POINT('Ctrl Pts',(-20.4235622970495,14.2901816868405,122.266085506153)) ;
#88901=CARTESIAN_POINT('Ctrl Pts',(-20.7535383605483,14.3101070787307,122.680152104981)) ;
#88902=CARTESIAN_POINT('Ctrl Pts',(-20.9224097639681,14.3300322920827,123.182173590077)) ;
#88903=CARTESIAN_POINT('Ctrl Pts',(-20.909967365172,14.3499573055678,123.711540173755)) ;
#88904=CARTESIAN_POINT('Ctrl Pts',(-20.7187416801209,14.3698337772678,124.204034514213)) ;
#88905=CARTESIAN_POINT('Ctrl Pts',(-20.3693357021894,14.3898130951767,124.603894071184)) ;
#88906=CARTESIAN_POINT('Ctrl Pts',(-19.9052962266747,14.4097460987527,124.85959923876)) ;
#88907=CARTESIAN_POINT('Ctrl Pts',(-19.3830046122281,14.4296413687804,124.941993474064)) ;
#88908=CARTESIAN_POINT('Ctrl Pts',(-18.863111653506,14.4495627066862,124.841603993362)) ;
#88909=CARTESIAN_POINT('Ctrl Pts',(-18.4079099213766,14.4695203299524,124.569231338478)) ;
#88910=CARTESIAN_POINT('Ctrl Pts',(-18.0742589102781,14.4894001619096,124.159636622647)) ;
#88911=CARTESIAN_POINT('Ctrl Pts',(-17.8989537036202,14.5092820132065,123.661028976949)) ;
#88912=CARTESIAN_POINT('Ctrl Pts',(-17.9053799742444,14.5293530303103,123.127680005003)) ;
#88913=CARTESIAN_POINT('Ctrl Pts',(-18.090928041147,14.5491602540634,122.634917461125)) ;
#88914=CARTESIAN_POINT('Ctrl Pts',(-18.4354593545979,14.5691413896322,122.230840604619)) ;
#88915=CARTESIAN_POINT('Ctrl Pts',(-18.8964698224689,14.5890688829714,121.970192630458)) ;
#88916=CARTESIAN_POINT('Ctrl Pts',(-19.4158400705055,14.6088895443292,121.881168125595)) ;
#88917=CARTESIAN_POINT('Ctrl Pts',(-19.9411622969537,14.628986733551,121.976797339529)) ;
#88918=CARTESIAN_POINT('Ctrl Pts',(-20.3952297063123,14.6487504125593,122.241401014461)) ;
#88919=CARTESIAN_POINT('Ctrl Pts',(-20.7369043382646,14.6688076912324,122.650295252524)) ;
#88920=CARTESIAN_POINT('Ctrl Pts',(-20.9160056364455,14.6886031149798,123.145152863214)) ;
#88921=CARTESIAN_POINT('Ctrl Pts',(-20.9171281004685,14.7085667597074,123.675691935841)) ;
#88922=CARTESIAN_POINT('Ctrl Pts',(-20.7357205067967,14.7285502509815,124.174887049982)) ;
#88923=CARTESIAN_POINT('Ctrl Pts',(-20.398657784175,14.7483577461308,124.579349028364)) ;
#88924=CARTESIAN_POINT('Ctrl Pts',(-19.9402292141674,14.7683403368509,124.847300212365)) ;
#88925=CARTESIAN_POINT('Ctrl Pts',(-19.4202472432439,14.7882229908422,124.942207693304)) ;
#88926=CARTESIAN_POINT('Ctrl Pts',(-18.8972710117422,14.8081812357052,124.854072619313)) ;
#88927=CARTESIAN_POINT('Ctrl Pts',(-18.4373523571738,14.8280568227468,124.59403836842)) ;
#88928=CARTESIAN_POINT('Ctrl Pts',(-18.0917464518894,14.8480377108821,124.190871761856)) ;
#88929=CARTESIAN_POINT('Ctrl Pts',(-17.9052470733622,14.8679728519931,123.694860655022)) ;
#88930=CARTESIAN_POINT('Ctrl Pts',(-17.8988327545552,14.8878848700041,123.165719308424)) ;
#88931=CARTESIAN_POINT('Ctrl Pts',(-18.0726432682034,14.9077730882477,122.666502021473)) ;
#88932=CARTESIAN_POINT('Ctrl Pts',(-18.3508412756587,14.9243713920946,122.324182529583)) ;
#88933=CARTESIAN_POINT('Ctrl Pts',(-18.6332517724376,14.9376439819974,122.119434069299)) ;
#88934=CARTESIAN_POINT('Ctrl Pts',(-18.8696162522265,14.9476513969483,122.004144120758)) ;
#88935=CARTESIAN_POINT('Ctrl Pts',(-19.122481344444,14.9576587436809,121.931865885675)) ;
#88936=CARTESIAN_POINT('Ctrl Pts',(-19.4692168268051,14.9709251034825,121.895493051636)) ;
#88937=CARTESIAN_POINT('Ctrl Pts',(-19.9027943031777,14.9874397611055,121.963407923393)) ;
#88938=CARTESIAN_POINT('Ctrl Pts',(-20.289623579524,15.0040371943481,122.175392008362)) ;
#88939=CARTESIAN_POINT('Ctrl Pts',(-20.5428597744861,15.0173851914931,122.41816948796)) ;
#88940=CARTESIAN_POINT('Ctrl Pts',(-20.6967684183011,15.0272809458447,122.627784026657)) ;
#88941=CARTESIAN_POINT('Ctrl Pts',(-20.81329530157,15.0372688997761,122.862950598469)) ;
#88942=CARTESIAN_POINT('Ctrl Pts',(-20.8871174069244,15.0472261234808,123.114018836122)) ;
#88943=CARTESIAN_POINT('Ctrl Pts',(-20.9163251075997,15.0572616700375,123.376101669285)) ;
#88944=CARTESIAN_POINT('Ctrl Pts',(-20.9000253490332,15.0671487813136,123.635429990405)) ;
#88945=CARTESIAN_POINT('Ctrl Pts',(-20.8387149445651,15.0771401864144,123.890722088326)) ;
#88946=CARTESIAN_POINT('Ctrl Pts',(-20.7344102203298,15.0870858076292,124.130366678656)) ;
#88947=CARTESIAN_POINT('Ctrl Pts',(-20.5904612859192,15.0970350558975,124.348645357239)) ;
#88948=CARTESIAN_POINT('Ctrl Pts',(-20.4088366867784,15.1070815510661,124.540239084563)) ;
#88949=CARTESIAN_POINT('Ctrl Pts',(-20.2009583169496,15.1169328938577,124.694555578007)) ;
#88950=CARTESIAN_POINT('Ctrl Pts',(-19.966949092894,15.126904673985,124.812422819299)) ;
#88951=CARTESIAN_POINT('Ctrl Pts',(-19.7153621269984,15.1368998739627,124.888039277954)) ;
#88952=CARTESIAN_POINT('Ctrl Pts',(-19.4534809990243,15.1469338656587,124.918615290549)) ;
#88953=CARTESIAN_POINT('Ctrl Pts',(-19.1948823108826,15.1567892706313,124.903936975073)) ;
#88954=CARTESIAN_POINT('Ctrl Pts',(-18.9390660225398,15.166788568477,124.844078851224)) ;
#88955=CARTESIAN_POINT('Ctrl Pts',(-18.6998538262199,15.1766836810822,124.742011656425)) ;
#88956=CARTESIAN_POINT('Ctrl Pts',(-18.4784349324494,15.1867443266172,124.59760214482)) ;
#88957=CARTESIAN_POINT('Ctrl Pts',(-18.289374519982,15.1965932036064,124.420815614991)) ;
#88958=CARTESIAN_POINT('Ctrl Pts',(-18.1305264432099,15.2066219147,124.210528253693)) ;
#88959=CARTESIAN_POINT('Ctrl Pts',(-18.0112304288892,15.2166513159561,123.975504636893)) ;
#88960=CARTESIAN_POINT('Ctrl Pts',(-17.9354501387818,15.2264915077521,123.728262940677)) ;
#88961=CARTESIAN_POINT('Ctrl Pts',(-17.9027451697684,15.2364949369451,123.467452153963)) ;
#88962=CARTESIAN_POINT('Ctrl Pts',(-17.9158870952322,15.2464804494113,123.205327859872)) ;
#88963=CARTESIAN_POINT('Ctrl Pts',(-17.9749122216437,15.2565215457953,122.94817162508)) ;
#88964=CARTESIAN_POINT('Ctrl Pts',(-18.075352673942,15.2663647417463,122.709774454952)) ;
#88965=CARTESIAN_POINT('Ctrl Pts',(-18.2172239193815,15.2763510528007,122.489051700623)) ;
#88966=CARTESIAN_POINT('Ctrl Pts',(-18.3942788891156,15.2862857380584,122.297122889139)) ;
#88967=CARTESIAN_POINT('Ctrl Pts',(-18.6046088256348,15.2963432992754,122.137133343391)) ;
#88968=CARTESIAN_POINT('Ctrl Pts',(-18.8338906873732,15.306164940884,122.018552182692)) ;
#88969=CARTESIAN_POINT('Ctrl Pts',(-19.0859639637451,15.316221004475,121.939290081059)) ;
#88970=CARTESIAN_POINT('Ctrl Pts',(-19.3450573076827,15.3261616802368,121.905856443279)) ;
#88971=CARTESIAN_POINT('Ctrl Pts',(-19.6050966128801,15.3360660390251,121.917057614141)) ;
#88972=CARTESIAN_POINT('Ctrl Pts',(-19.8628314894455,15.3461126936009,121.974204391667)) ;
#88973=CARTESIAN_POINT('Ctrl Pts',(-20.1032054022461,15.3560082882438,122.073524957395)) ;
#88974=CARTESIAN_POINT('Ctrl Pts',(-20.3263274818967,15.3660702349007,122.215360141734)) ;
#88975=CARTESIAN_POINT('Ctrl Pts',(-20.5173806023937,15.3759198588328,122.390011089637)) ;
#88976=CARTESIAN_POINT('Ctrl Pts',(-20.6776940933443,15.3858830978627,122.596996909064)) ;
#88977=CARTESIAN_POINT('Ctrl Pts',(-20.8000760560513,15.3959076726385,122.830296872806)) ;
#88978=CARTESIAN_POINT('Ctrl Pts',(-20.8793976462342,15.4058262353262,123.078576451367)) ;
#88979=CARTESIAN_POINT('Ctrl Pts',(-20.9151255754094,15.4158184220502,123.338734291713)) ;
#88980=CARTESIAN_POINT('Ctrl Pts',(-20.9046224904582,15.4258532206344,123.602218432797)) ;
#88981=CARTESIAN_POINT('Ctrl Pts',(-20.8499613006373,15.4357084113081,123.855389436239)) ;
#88982=CARTESIAN_POINT('Ctrl Pts',(-20.7510911952532,15.4457077594611,124.098804793932)) ;
#88983=CARTESIAN_POINT('Ctrl Pts',(-20.6131053102038,15.4556028851362,124.319258702986)) ;
#88984=CARTESIAN_POINT('Ctrl Pts',(-20.4360576038621,15.4656634280843,124.51555709839)) ;
#88985=CARTESIAN_POINT('Ctrl Pts',(-20.2320397835465,15.4755127023512,124.674867184459)) ;
#88986=CARTESIAN_POINT('Ctrl Pts',(-19.9996679689736,15.4855399269211,124.799102630686)) ;
#88987=CARTESIAN_POINT('Ctrl Pts',(-19.7489910633449,15.4955683261089,124.880464971312)) ;
#88988=CARTESIAN_POINT('Ctrl Pts',(-19.4928458279102,15.5054140765224,124.916870140584)) ;
#88989=CARTESIAN_POINT('Ctrl Pts',(-19.2304605256444,15.5154028669231,124.908855957832)) ;
#88990=CARTESIAN_POINT('Ctrl Pts',(-18.9721684140402,15.5254477953228,124.854455310312)) ;
#88991=CARTESIAN_POINT('Ctrl Pts',(-18.7323714755152,15.5352722801118,124.7587411508)) ;
#88992=CARTESIAN_POINT('Ctrl Pts',(-18.5074627778425,15.545329677653,124.619968276734)) ;
#88993=CARTESIAN_POINT('Ctrl Pts',(-18.3128405903418,15.5552557692392,124.446263039187)) ;
#88994=CARTESIAN_POINT('Ctrl Pts',(-18.150350868832,15.5652105543838,124.241248427742)) ;
#88995=CARTESIAN_POINT('Ctrl Pts',(-18.0251521487945,15.5752479240414,124.009084692641)) ;
#88996=CARTESIAN_POINT('Ctrl Pts',(-17.9432016162711,15.585136734163,123.762469410516)) ;
#88997=CARTESIAN_POINT('Ctrl Pts',(-17.9044670409744,15.5951260932141,123.502838762861)) ;
#88998=CARTESIAN_POINT('Ctrl Pts',(-17.9115749765126,15.6050846406702,123.24124293323)) ;
#88999=CARTESIAN_POINT('Ctrl Pts',(-17.9630623576573,15.6149842172212,122.986221570105)) ;
#89000=CARTESIAN_POINT('Ctrl Pts',(-18.0595417871603,15.6250321290519,122.740459685975)) ;
#89001=CARTESIAN_POINT('Ctrl Pts',(-18.1949986414737,15.6349274769125,122.518438659765)) ;
#89002=CARTESIAN_POINT('Ctrl Pts',(-18.3697629356532,15.6449891534437,122.320059129432)) ;
#89003=CARTESIAN_POINT('Ctrl Pts',(-18.5718644577124,15.6548336711928,122.158541982419)) ;
#89004=CARTESIAN_POINT('Ctrl Pts',(-18.8011526189207,15.6647941149076,122.032301199326)) ;
#89005=CARTESIAN_POINT('Ctrl Pts',(-19.0509357609831,15.6748309477258,121.947606476504)) ;
#89006=CARTESIAN_POINT('Ctrl Pts',(-19.3074921480599,15.6847097444726,121.907773626489)) ;
#89007=CARTESIAN_POINT('Ctrl Pts',(-19.5717593834283,15.694769060601,121.913104494787)) ;
#89008=CARTESIAN_POINT('Ctrl Pts',(-19.8262605890557,15.7046395073542,121.963283380412)) ;
#89009=CARTESIAN_POINT('Ctrl Pts',(-20.0714198955884,15.7146321456122,122.057380334014)) ;
#89010=CARTESIAN_POINT('Ctrl Pts',(-20.2971021415107,15.7246641611601,122.193630102715)) ;
#89011=CARTESIAN_POINT('Ctrl Pts',(-20.4928065396954,15.7345300174667,122.363722707075)) ;
#89012=CARTESIAN_POINT('Ctrl Pts',(-20.659353254304,15.7445993069358,122.569307538849)) ;
#89013=CARTESIAN_POINT('Ctrl Pts',(-20.7848456281026,15.7544428644871,122.795525024093)) ;
#89014=CARTESIAN_POINT('Ctrl Pts',(-20.8711257023825,15.764422991275,123.043184928911)) ;
#89015=CARTESIAN_POINT('Ctrl Pts',(-20.9127559215498,15.7744415398749,123.303142599032)) ;
#89016=CARTESIAN_POINT('Ctrl Pts',(-20.9092242705699,15.7843248403981,123.562873547571)) ;
#89017=CARTESIAN_POINT('Ctrl Pts',(-20.8596396741269,15.7943931274462,123.822725252708)) ;
#89018=CARTESIAN_POINT('Ctrl Pts',(-20.7681651750302,15.8042232504649,124.064360555124)) ;
#89019=CARTESIAN_POINT('Ctrl Pts',(-20.6332871001612,15.8142898343902,124.291882100143)) ;
#89020=CARTESIAN_POINT('Ctrl Pts',(-20.4638049151612,15.8241799474047,124.48896825144)) ;
#89021=CARTESIAN_POINT('Ctrl Pts',(-20.2609877478758,15.8341726361673,124.655734358688)) ;
#89022=CARTESIAN_POINT('Ctrl Pts',(-20.0329028474693,15.8441335245231,124.784198130911)) ;
#89023=CARTESIAN_POINT('Ctrl Pts',(-19.7872175767508,15.8540514694031,124.871145968037)) ;
#89024=CARTESIAN_POINT('Ctrl Pts',(-19.5278485703835,15.8640592224993,124.914811107078)) ;
#89025=CARTESIAN_POINT('Ctrl Pts',(-19.2642689030462,15.8740903164583,124.91223920911)) ;
#89026=CARTESIAN_POINT('Ctrl Pts',(-19.0097316360131,15.8839382844863,124.865387875955)) ;
#89027=CARTESIAN_POINT('Ctrl Pts',(-18.761882854262,15.8940002406122,124.773318370912)) ;
#89028=CARTESIAN_POINT('Ctrl Pts',(-18.5376157807696,15.9038974522133,124.641576258663)) ;
#89029=CARTESIAN_POINT('Ctrl Pts',(-18.3384056514573,15.9138286188779,124.472982338498)) ;
#89030=CARTESIAN_POINT('Ctrl Pts',(-18.1698491513015,15.9238708030821,124.269933564785)) ;
#89031=CARTESIAN_POINT('Ctrl Pts',(-18.0409623377378,15.9337574713353,124.044330723478)) ;
#89032=CARTESIAN_POINT('Ctrl Pts',(-17.9518555076836,15.9437505833135,123.79731633989)) ;
#89033=CARTESIAN_POINT('Ctrl Pts',(-17.9072992563308,15.9536962609293,123.539779663906)) ;
#89034=CARTESIAN_POINT('Ctrl Pts',(-17.9076038590327,15.9636435639143,123.278362513842)) ;
#89035=CARTESIAN_POINT('Ctrl Pts',(-17.954039484633,15.9736912876611,123.018441119269)) ;
#89036=CARTESIAN_POINT('Ctrl Pts',(-18.0429092629221,15.9835396614236,122.77537631077)) ;
#89037=CARTESIAN_POINT('Ctrl Pts',(-18.1733362386872,15.9934986338693,122.548480377477)) ;
#89038=CARTESIAN_POINT('Ctrl Pts',(-18.3428858266523,16.0035374957505,122.346380568049)) ;
#89039=CARTESIAN_POINT('Ctrl Pts',(-18.5414869910732,16.0134160999223,122.179156901752)) ;
#89040=CARTESIAN_POINT('Ctrl Pts',(-18.7699271953843,16.0234676411256,122.046612208989)) ;
#89041=CARTESIAN_POINT('Ctrl Pts',(-19.0141072069317,16.0333630391059,121.957051725276)) ;
#89042=CARTESIAN_POINT('Ctrl Pts',(-19.2740547380586,16.0434142716512,121.910401805192)) ;
#89043=CARTESIAN_POINT('Ctrl Pts',(-19.5338803406111,16.0533004622755,121.909579455401)) ;
#89044=CARTESIAN_POINT('Ctrl Pts',(-19.7926868268136,16.0632930015913,121.953875934243)) ;
#89045=CARTESIAN_POINT('Ctrl Pts',(-20.0387894173471,16.073241447486,122.04213980991)) ;
#89046=CARTESIAN_POINT('Ctrl Pts',(-20.265712566684,16.0831782500179,122.171300244256)) ;
#89047=CARTESIAN_POINT('Ctrl Pts',(-20.4679516213838,16.0931612574692,122.338455368566)) ;
#89048=CARTESIAN_POINT('Ctrl Pts',(-20.6387206153012,16.103205098884,122.539669360996)) ;
#89049=CARTESIAN_POINT('Ctrl Pts',(-20.7696595815421,16.1130332975079,122.762338547933)) ;
#89050=CARTESIAN_POINT('Ctrl Pts',(-20.8623125592493,16.1231098909501,123.010343765831)) ;
#89051=CARTESIAN_POINT('Ctrl Pts',(-20.9095729442255,16.1329618902917,123.264952690282)) ;
#89052=CARTESIAN_POINT('Ctrl Pts',(-20.9121762627497,16.1430354771156,123.529617389355)) ;
#89053=CARTESIAN_POINT('Ctrl Pts',(-20.869730533684,16.152875702213,123.784725112839)) ;
#89054=CARTESIAN_POINT('Ctrl Pts',(-20.7834213237411,16.1628414062417,124.031959888329)) ;
#89055=CARTESIAN_POINT('Ctrl Pts',(-20.6543616553613,16.1728680395483,124.261695407877)) ;
#89056=CARTESIAN_POINT('Ctrl Pts',(-20.4893937694131,16.1827823352601,124.463343826805)) ;
#89057=CARTESIAN_POINT('Ctrl Pts',(-20.2907385375805,16.1927706239526,124.634927879414)) ;
#89058=CARTESIAN_POINT('Ctrl Pts',(-20.063944204818,16.2028093571109,124.769667401044)) ;
#89059=CARTESIAN_POINT('Ctrl Pts',(-19.8221495313365,16.2126526889385,124.861577146822)) ;
#89060=CARTESIAN_POINT('Ctrl Pts',(-19.5634230879079,16.2226804148181,124.911613949581)) ;
#89061=CARTESIAN_POINT('Ctrl Pts',(-19.2997995110888,16.2327127512066,124.915252649983)) ;
#89062=CARTESIAN_POINT('Ctrl Pts',(-19.0447508850932,16.2425422515072,124.87443461805)) ;
#89063=CARTESIAN_POINT('Ctrl Pts',(-18.7964127409365,16.252531755424,124.789315485236)) ;
#89064=CARTESIAN_POINT('Ctrl Pts',(-18.5657100501157,16.2625755959364,124.661096709419)) ;
#89065=CARTESIAN_POINT('Ctrl Pts',(-18.3649684583117,16.2723973017045,124.498860195946)) ;
#89066=CARTESIAN_POINT('Ctrl Pts',(-18.1912776614032,16.2824323488368,124.30043121603)) ;
#89067=CARTESIAN_POINT('Ctrl Pts',(-18.0554378922695,16.2924570262737,124.074705597496)) ;
#89068=CARTESIAN_POINT('Ctrl Pts',(-17.9619696621494,16.3023098411282,123.833243322249)) ;
#89069=CARTESIAN_POINT('Ctrl Pts',(-17.9107123152974,16.3122975507357,123.575850309162)) ;
#89070=CARTESIAN_POINT('Ctrl Pts',(-17.9049458569947,16.3222275607298,123.314954275145)) ;
#89071=CARTESIAN_POINT('Ctrl Pts',(-17.9444047205986,16.332217315949,123.055411337041)) ;
#89072=CARTESIAN_POINT('Ctrl Pts',(-18.0289611024086,16.3422439246319,122.805854001657)) ;
#89073=CARTESIAN_POINT('Ctrl Pts',(-18.1535398915879,16.3521278646537,122.577945287591)) ;
#89074=CARTESIAN_POINT('Ctrl Pts',(-18.3170581793031,16.3621170921922,122.372577155451)) ;
#89075=CARTESIAN_POINT('Ctrl Pts',(-18.5151613636324,16.3721599627159,122.198204531201)) ;
#89076=CARTESIAN_POINT('Ctrl Pts',(-18.7355937159182,16.3819923494713,122.06340510794)) ;
#89077=CARTESIAN_POINT('Ctrl Pts',(-18.9797379454661,16.3919856426429,121.966674506609)) ;
#89078=CARTESIAN_POINT('Ctrl Pts',(-19.2380933202206,16.4020176482913,121.914136786792)) ;
#89079=CARTESIAN_POINT('Ctrl Pts',(-19.4972319162803,16.4118829042603,121.907050750478)) ;
#89080=CARTESIAN_POINT('Ctrl Pts',(-19.7563049005742,16.4218447841678,121.944708800064)) ;
#89081=CARTESIAN_POINT('Ctrl Pts',(-20.0065704728934,16.4318797175297,122.027782317763)) ;
#89082=CARTESIAN_POINT('Ctrl Pts',(-20.235395236987,16.441764675909,122.150815185132)) ;
#89083=CARTESIAN_POINT('Ctrl Pts',(-20.4430095418267,16.4518303028317,122.314647056948)) ;
#89084=CARTESIAN_POINT('Ctrl Pts',(-20.6153156253427,16.461669408496,122.507485556433)) ;
#89085=CARTESIAN_POINT('Ctrl Pts',(-20.7548759132793,16.4717322235013,122.732057555602)) ;
#89086=CARTESIAN_POINT('Ctrl Pts',(-20.8514951454901,16.48162842955,122.973534637153)) ;
#89087=CARTESIAN_POINT('Ctrl Pts',(-20.9056579365925,16.4915692525753,123.229061857975)) ;
#89088=CARTESIAN_POINT('Ctrl Pts',(-20.9147539350784,16.501573835554,123.491844043348)) ;
#89089=CARTESIAN_POINT('Ctrl Pts',(-20.8777116944424,16.5115947299987,123.752558207369)) ;
#89090=CARTESIAN_POINT('Ctrl Pts',(-20.7973193962089,16.5214866505881,123.9997713371)) ;
#89091=CARTESIAN_POINT('Ctrl Pts',(-20.6743097948123,16.5314800829335,124.231787262463)) ;
#89092=CARTESIAN_POINT('Ctrl Pts',(-20.5135843010475,16.5414256878334,124.437884102592)) ;
#89093=CARTESIAN_POINT('Ctrl Pts',(-20.3198274952116,16.5513729613149,124.613376926942)) ;
#89094=CARTESIAN_POINT('Ctrl Pts',(-20.0961655477988,16.5614208757913,124.753706244345)) ;
#89095=CARTESIAN_POINT('Ctrl Pts',(-19.8564832755268,16.5712685161386,124.851295914385)) ;
#89096=CARTESIAN_POINT('Ctrl Pts',(-19.6007546274818,16.5812302315152,124.907216087891)) ;
#89097=CARTESIAN_POINT('Ctrl Pts',(-19.3374019357033,16.591258855088,124.917623305779)) ;
#89098=CARTESIAN_POINT('Ctrl Pts',(-19.0793392609636,16.6011692171544,124.882650735253)) ;
#89099=CARTESIAN_POINT('Ctrl Pts',(-18.8304294039593,16.6111039108068,124.803856446845)) ;
#89100=CARTESIAN_POINT('Ctrl Pts',(-18.596627686363,16.6211457539347,124.681515843378)) ;
#89101=CARTESIAN_POINT('Ctrl Pts',(-18.3907224983714,16.6310302595051,124.523120625139)) ;
#89102=CARTESIAN_POINT('Ctrl Pts',(-18.213179611499,16.6410323632903,124.329353348425)) ;
#89103=CARTESIAN_POINT('Ctrl Pts',(-18.0729347335421,16.6509507147053,124.109605240172)) ;
#89104=CARTESIAN_POINT('Ctrl Pts',(-17.9717684511152,16.6609983707262,123.865757550208)) ;
#89105=CARTESIAN_POINT('Ctrl Pts',(-17.9151801485084,16.6708695637544,123.612544609832)) ;
#89106=CARTESIAN_POINT('Ctrl Pts',(-17.9031486210089,16.6809352768979,123.348363900477)) ;
#89107=CARTESIAN_POINT('Ctrl Pts',(-17.9361680628292,16.6907877374706,123.091490849331)) ;
#89108=CARTESIAN_POINT('Ctrl Pts',(-18.041350571431,16.7042162001931,122.754758769299)) ;
#89109=CARTESIAN_POINT('Ctrl Pts',(-18.2267930848674,16.7172971477102,122.460500377085)) ;
#89110=CARTESIAN_POINT('Ctrl Pts',(-18.4863600281543,16.7307716459448,122.219764136354)) ;
#89111=CARTESIAN_POINT('Ctrl Pts',(-18.7036600720593,16.7406037495542,122.079903461464)) ;
#89112=CARTESIAN_POINT('Ctrl Pts',(-18.9447043729808,16.7505696526809,121.977589420528)) ;
#89113=CARTESIAN_POINT('Ctrl Pts',(-19.2015822289623,16.7605970619911,121.918702174221)) ;
#89114=CARTESIAN_POINT('Ctrl Pts',(-19.4616612966653,16.7705080933577,121.90540119112)) ;
#89115=CARTESIAN_POINT('Ctrl Pts',(-19.8072674417979,16.7837524009787,121.947145247852)) ;
#89116=CARTESIAN_POINT('Ctrl Pts',(-20.2188607320283,16.8004528836499,122.113061781685)) ;
#89117=CARTESIAN_POINT('Ctrl Pts',(-20.5455735820307,16.8169597128057,122.405977428994)) ;
#89118=CARTESIAN_POINT('Ctrl Pts',(-20.7373318770542,16.8302703410433,122.698474315006)) ;
#89119=CARTESIAN_POINT('Ctrl Pts',(-20.8410538416381,16.8402629045834,122.939759731386)) ;
#89120=CARTESIAN_POINT('Ctrl Pts',(-20.9012068159582,16.8502929875849,123.196350988495)) ;
#89121=CARTESIAN_POINT('Ctrl Pts',(-20.9212193192341,16.8634665915827,123.542025913649)) ;
#89122=CARTESIAN_POINT('Ctrl Pts',(-20.832303368653,16.8801042968141,123.975028581527)) ;
#89123=CARTESIAN_POINT('Ctrl Pts',(-20.5559527242748,16.8999860593815,124.425665773585)) ;
#89124=CARTESIAN_POINT('Ctrl Pts',(-20.2087278908941,16.916682411598,124.701769095248)) ;
#89125=CARTESIAN_POINT('Ctrl Pts',(-19.8917137009118,16.9298394393871,124.83996615317)) ;
#89126=CARTESIAN_POINT('Ctrl Pts',(-19.5501593226237,16.9432167940307,124.923024211938)) ;
#89127=CARTESIAN_POINT('Ctrl Pts',(-19.1108610444918,16.9597476282895,124.912764903616)) ;
#89128=CARTESIAN_POINT('Ctrl Pts',(-18.6161741406845,16.9797123180326,124.720936570403)) ;
#89129=CARTESIAN_POINT('Ctrl Pts',(-18.2178875673859,16.9996288114562,124.372240740112)) ;
#89130=CARTESIAN_POINT('Ctrl Pts',(-17.9619000053034,17.0195185308058,123.909658769635)) ;
#89131=CARTESIAN_POINT('Ctrl Pts',(-17.8790923718899,17.0395252604536,123.384478022634)) ;
#89132=CARTESIAN_POINT('Ctrl Pts',(-17.9792607793457,17.0593633141005,122.866706624068)) ;
#89133=CARTESIAN_POINT('Ctrl Pts',(-18.251654980879,17.0793566523141,122.410555995914)) ;
#89134=CARTESIAN_POINT('Ctrl Pts',(-18.6614413308425,17.0992394517207,122.076728435462)) ;
#89135=CARTESIAN_POINT('Ctrl Pts',(-19.1602498824996,17.1191316326394,121.901928665033)) ;
#89136=CARTESIAN_POINT('Ctrl Pts',(-19.6893506726758,17.1390338111345,121.906954280708)) ;
#89137=CARTESIAN_POINT('Ctrl Pts',(-20.1877372859541,17.1590711223382,122.094250728715)) ;
#89138=CARTESIAN_POINT('Ctrl Pts',(-20.5885147516778,17.1788835638791,122.436171529998)) ;
#89139=CARTESIAN_POINT('Ctrl Pts',(-20.8514859106502,17.198948804614,122.899836288904)) ;
#89140=CARTESIAN_POINT('Ctrl Pts',(-20.9395751047835,17.2187060094698,123.417764524091)) ;
#89141=CARTESIAN_POINT('Ctrl Pts',(-20.8451902721094,17.2387392821155,123.941511312625)) ;
#89142=CARTESIAN_POINT('Ctrl Pts',(-20.5803738327966,17.2585521905694,124.396949460866)) ;
#89143=CARTESIAN_POINT('Ctrl Pts',(-20.1731152784338,17.2785483366968,124.738041234505)) ;
#89144=CARTESIAN_POINT('Ctrl Pts',(-19.6769118272769,17.2984100899193,124.918872799759)) ;
#89145=CARTESIAN_POINT('Ctrl Pts',(-19.1436416860639,17.3184786070474,124.919193987262)) ;
#89146=CARTESIAN_POINT('Ctrl Pts',(-18.648109623505,17.3383094800442,124.739265310968)) ;
#89147=CARTESIAN_POINT('Ctrl Pts',(-18.2411319113203,17.3582313908609,124.40073894506)) ;
#89148=CARTESIAN_POINT('Ctrl Pts',(-17.9740323769222,17.3781608342962,123.94322080473)) ;
#89149=CARTESIAN_POINT('Ctrl Pts',(-17.8790250602224,17.3980705044126,123.422734778079)) ;
#89150=CARTESIAN_POINT('Ctrl Pts',(-17.9662662127267,17.4179438616755,122.901724773555)) ;
#89151=CARTESIAN_POINT('Ctrl Pts',(-18.2276294818176,17.4379353962934,122.439190238654)) ;
#89152=CARTESIAN_POINT('Ctrl Pts',(-18.6285734387837,17.4578010137041,122.095521594485)) ;
#89153=CARTESIAN_POINT('Ctrl Pts',(-19.1253152085356,17.4777819435324,121.907762643509)) ;
#89154=CARTESIAN_POINT('Ctrl Pts',(-19.6552200286643,17.4977204056155,121.901390129916)) ;
#89155=CARTESIAN_POINT('Ctrl Pts',(-20.1546489410619,17.5176125988372,122.075060293898)) ;
#89156=CARTESIAN_POINT('Ctrl Pts',(-20.5661552710587,17.5375833138726,122.410136115304)) ;
#89157=CARTESIAN_POINT('Ctrl Pts',(-20.837318013256,17.5573929855387,122.861593772204)) ;
#89158=CARTESIAN_POINT('Ctrl Pts',(-20.9394053743083,17.5773862022299,123.382882566089)) ;
#89159=CARTESIAN_POINT('Ctrl Pts',(-20.8584272459729,17.5972371144262,123.904456907226)) ;
#89160=CARTESIAN_POINT('Ctrl Pts',(-20.6013722647494,17.6173117207453,124.371835879059)) ;
#89161=CARTESIAN_POINT('Ctrl Pts',(-20.2709413387604,17.6338283526286,124.661087804809)) ;
#89162=CARTESIAN_POINT('Ctrl Pts',(-19.9567456572262,17.6471670603227,124.816311506479)) ;
#89163=CARTESIAN_POINT('Ctrl Pts',(-19.7085634180374,17.657009434631,124.889285728244)) ;
#89164=CARTESIAN_POINT('Ctrl Pts',(-19.4460346302332,17.6670644546137,124.918920394545)) ;
#89165=CARTESIAN_POINT('Ctrl Pts',(-19.0989340056819,17.6802966112713,124.897325675655)) ;
#89166=CARTESIAN_POINT('Ctrl Pts',(-18.6800921880835,17.6969115786164,124.757498322391)) ;
#89167=CARTESIAN_POINT('Ctrl Pts',(-18.3346383771164,17.7135061656276,124.483309875907)) ;
#89168=CARTESIAN_POINT('Ctrl Pts',(-18.1268953740658,17.726739733983,124.204383339548)) ;
#89169=CARTESIAN_POINT('Ctrl Pts',(-18.0083495823601,17.7367833517917,123.968592623646)) ;
#89170=CARTESIAN_POINT('Ctrl Pts',(-17.9336310060421,17.7466702760265,123.71972753629)) ;
#89171=CARTESIAN_POINT('Ctrl Pts',(-17.9024800444537,17.7566609304733,123.459055825321)) ;
#89172=CARTESIAN_POINT('Ctrl Pts',(-17.91707504202,17.7666226889273,123.197677226246)) ;
#89173=CARTESIAN_POINT('Ctrl Pts',(-17.9967448142101,17.7799625539945,122.856223951778)) ;
#89174=CARTESIAN_POINT('Ctrl Pts',(-18.1639793074523,17.7932713369078,122.544584740488)) ;
#89175=CARTESIAN_POINT('Ctrl Pts',(-18.4009261605596,17.8064670943519,122.291390427509)) ;
#89176=CARTESIAN_POINT('Ctrl Pts',(-18.6098409160699,17.8164289780284,122.133625520298)) ;
#89177=CARTESIAN_POINT('Ctrl Pts',(-18.8450658298774,17.826472087543,122.013949993326)) ;
#89178=CARTESIAN_POINT('Ctrl Pts',(-19.092621766734,17.8363243375422,121.938100172443)) ;
#89179=CARTESIAN_POINT('Ctrl Pts',(-19.3525817752957,17.8462958744927,121.905367673207)) ;
#89180=CARTESIAN_POINT('Ctrl Pts',(-19.6149678521797,17.8562911399702,121.918326097359)) ;
#89181=CARTESIAN_POINT('Ctrl Pts',(-19.8719764054818,17.8663251128439,121.977174194731)) ;
#89182=CARTESIAN_POINT('Ctrl Pts',(-20.1107443124788,17.8761805276062,122.07756701248)) ;
#89183=CARTESIAN_POINT('Ctrl Pts',(-20.3317665609879,17.886179805115,122.219601552815)) ;
#89184=CARTESIAN_POINT('Ctrl Pts',(-20.5230159036683,17.896074989278,122.39585448978)) ;
#89185=CARTESIAN_POINT('Ctrl Pts',(-20.6833174072794,17.9061353689188,122.60604307054)) ;
#89186=CARTESIAN_POINT('Ctrl Pts',(-20.8023179831757,17.9159852379269,122.835939812967)) ;
#89187=CARTESIAN_POINT('Ctrl Pts',(-20.8815806037002,17.9260167991348,123.08734301173)) ;
#89188=CARTESIAN_POINT('Ctrl Pts',(-20.9153942834191,17.9360272480171,123.348249186297)) ;
#89189=CARTESIAN_POINT('Ctrl Pts',(-20.9038056440646,17.9459339874341,123.608321329956)) ;
#89190=CARTESIAN_POINT('Ctrl Pts',(-20.8475549821368,17.9558720035025,123.863336913945)) ;
#89191=CARTESIAN_POINT('Ctrl Pts',(-20.7473491124227,17.9658772499537,124.106450718163)) ;
#89192=CARTESIAN_POINT('Ctrl Pts',(-20.6056897092289,17.97591131101,124.328835897672)) ;
#89193=CARTESIAN_POINT('Ctrl Pts',(-20.4312337067048,17.9857563920681,124.519908095883)) ;
#89194=CARTESIAN_POINT('Ctrl Pts',(-20.2236664013566,17.9957421980216,124.680396433313)) ;
#89195=CARTESIAN_POINT('Ctrl Pts',(-19.992579689612,18.0056770185758,124.801991034309)) ;
#89196=CARTESIAN_POINT('Ctrl Pts',(-19.7408295621782,18.015734543708,124.882346278087)) ;
#89197=CARTESIAN_POINT('Ctrl Pts',(-19.4850812770158,18.0255561943594,124.917339204616)) ;
#89198=CARTESIAN_POINT('Ctrl Pts',(-19.2210175734843,18.0356122578641,124.907651917327)) ;
#89199=CARTESIAN_POINT('Ctrl Pts',(-18.9656796380445,18.045552924928,124.85243013731)) ;
#89200=CARTESIAN_POINT('Ctrl Pts',(-18.7243886052584,18.055457318594,124.754831562349)) ;
#89201=CARTESIAN_POINT('Ctrl Pts',(-18.5006574893832,18.065503842357,124.61470975614)) ;
#89202=CARTESIAN_POINT('Ctrl Pts',(-18.307369291185,18.0753999253734,124.440656203214)) ;
#89203=CARTESIAN_POINT('Ctrl Pts',(-18.1445872821212,18.0854666246034,124.232186912263)) ;
#89204=CARTESIAN_POINT('Ctrl Pts',(-18.0231672453592,18.0952902350045,124.004324151478)) ;
#89205=CARTESIAN_POINT('Ctrl Pts',(-17.9408459619243,18.105346095182,123.753251808151)) ;
#89206=CARTESIAN_POINT('Ctrl Pts',(-17.9041508391774,18.1152792414869,123.494778928388)) ;
#89207=CARTESIAN_POINT('Ctrl Pts',(-17.9123669611964,18.1252244972575,123.233587463902)) ;
#89208=CARTESIAN_POINT('Ctrl Pts',(-17.965820602866,18.135207795696,122.976706518041)) ;
#89209=CARTESIAN_POINT('Ctrl Pts',(-18.063904304486,18.1452449758426,122.731876350353)) ;
#89210=CARTESIAN_POINT('Ctrl Pts',(-18.2001593676184,18.1550995285521,122.511623169625)) ;
#89211=CARTESIAN_POINT('Ctrl Pts',(-18.3748041349657,18.1650990469994,122.315340175389)) ;
#89212=CARTESIAN_POINT('Ctrl Pts',(-18.5786232758408,18.1749941294615,122.153792991792)) ;
#89213=CARTESIAN_POINT('Ctrl Pts',(-18.8111647901301,18.1850546749676,122.028081402506)) ;
#89214=CARTESIAN_POINT('Ctrl Pts',(-19.0567404030301,18.1949039822156,121.94625334283)) ;
#89215=CARTESIAN_POINT('Ctrl Pts',(-19.3172903973273,18.204931072303,121.906964506293)) ;
#89216=CARTESIAN_POINT('Ctrl Pts',(-19.5807510422382,18.2149599764399,121.914213939927)) ;
#89217=CARTESIAN_POINT('Ctrl Pts',(-19.8342692925352,18.2248038415392,121.965616328592)) ;
#89218=CARTESIAN_POINT('Ctrl Pts',(-20.0789732695833,18.2347996682476,122.061118208397)) ;
#89219=CARTESIAN_POINT('Ctrl Pts',(-20.3037898720174,18.2448248848966,122.198476327115)) ;
#89220=CARTESIAN_POINT('Ctrl Pts',(-20.4989049499709,18.2547147170542,122.37016702887)) ;
#89221=CARTESIAN_POINT('Ctrl Pts',(-20.6631753421901,18.2647055731389,122.574966335763)) ;
#89222=CARTESIAN_POINT('Ctrl Pts',(-20.788773377905,18.2746506677318,122.804154170433)) ;
#89223=CARTESIAN_POINT('Ctrl Pts',(-20.8731939482788,18.2846025714999,123.051690442556)) ;
#89224=CARTESIAN_POINT('Ctrl Pts',(-20.9134619567521,18.2946389709693,123.312337432225)) ;
#89225=CARTESIAN_POINT('Ctrl Pts',(-20.9081339354844,18.304528041058,123.572166354225)) ;
#89226=CARTESIAN_POINT('Ctrl Pts',(-20.8577276976876,18.3145173304289,123.829783197126)) ;
#89227=CARTESIAN_POINT('Ctrl Pts',(-20.7634652567705,18.3244758966386,124.073909818492)) ;
#89228=CARTESIAN_POINT('Ctrl Pts',(-20.6295842577516,18.3343754678554,124.296985254271)) ;
#89229=CARTESIAN_POINT('Ctrl Pts',(-20.4564060477001,18.3444233822697,124.496275231277)) ;
#89230=CARTESIAN_POINT('Ctrl Pts',(-20.2544457726215,18.3543187251302,124.660147079943)) ;
#89231=CARTESIAN_POINT('Ctrl Pts',(-20.0233589167788,18.3643804190777,124.788582887775)) ;
#89232=CARTESIAN_POINT('Ctrl Pts',(-19.7788516309637,18.3742248721618,124.873135508736)) ;
#89233=CARTESIAN_POINT('Ctrl Pts',(-19.5205311753707,18.3841855571203,124.915333903471)) ;
#89234=CARTESIAN_POINT('Ctrl Pts',(-19.2568158507944,18.3942214896288,124.91156959599)) ;
#89235=CARTESIAN_POINT('Ctrl Pts',(-19.0015267672572,18.4041101053169,124.863056912793)) ;
#89236=CARTESIAN_POINT('Ctrl Pts',(-18.7552413200576,18.4141245144593,124.770264913515)) ;
#89237=CARTESIAN_POINT('Ctrl Pts',(-18.5287491933341,18.4241583234171,124.635287434208)) ;
#89238=CARTESIAN_POINT('Ctrl Pts',(-18.3326736838035,18.4339887776733,124.467040337069)) ;
#89239=CARTESIAN_POINT('Ctrl Pts',(-18.1646552309895,18.4440664452515,124.262399712302)) ;
#89240=CARTESIAN_POINT('Ctrl Pts',(-18.0374628156085,18.4539183133737,124.036835965427)) ;
#89241=CARTESIAN_POINT('Ctrl Pts',(-17.9492624861745,18.4639913509391,123.787301761498)) ;
#89242=CARTESIAN_POINT('Ctrl Pts',(-17.9067521481246,18.47383390429,123.532143869047)) ;
#89243=CARTESIAN_POINT('Ctrl Pts',(-17.9083434021815,18.4838142997834,123.269885593791)) ;
#89244=CARTESIAN_POINT('Ctrl Pts',(-17.9561323187471,18.4938327777612,123.010990190508)) ;
#89245=CARTESIAN_POINT('Ctrl Pts',(-18.0463999219275,18.5037160920673,122.767424084949)) ;
#89246=CARTESIAN_POINT('Ctrl Pts',(-18.1801054394556,18.513784394606,122.53915993018)) ;
#89247=CARTESIAN_POINT('Ctrl Pts',(-18.3471840847822,18.5236144418794,122.342083268111)) ;
#89248=CARTESIAN_POINT('Ctrl Pts',(-18.5504477114517,18.5336813132949,122.172834206145)) ;
#89249=CARTESIAN_POINT('Ctrl Pts',(-18.7760961055222,18.543570352094,122.043850044035)) ;
#89250=CARTESIAN_POINT('Ctrl Pts',(-19.0231397001699,18.5535670502281,121.954587201367)) ;
#89251=CARTESIAN_POINT('Ctrl Pts',(-19.2808470530102,18.5635194759401,121.909875533707)) ;
#89252=CARTESIAN_POINT('Ctrl Pts',(-19.5420744376569,18.573460778173,121.910226123319)) ;
#89253=CARTESIAN_POINT('Ctrl Pts',(-19.8004561957054,18.5834440172569,121.955853427861)) ;
#89254=CARTESIAN_POINT('Ctrl Pts',(-20.048172080969,18.5934828188255,122.046518326737)) ;
#89255=CARTESIAN_POINT('Ctrl Pts',(-20.2723410125305,18.6033309249472,122.17589057555)) ;
#89256=CARTESIAN_POINT('Ctrl Pts',(-20.4750350377161,18.6133911205225,122.345583287443)) ;
#89257=CARTESIAN_POINT('Ctrl Pts',(-20.6422769769176,18.6232888038339,122.544802617581)) ;
#89258=CARTESIAN_POINT('Ctrl Pts',(-20.7735588255307,18.6332198442079,122.770350862156)) ;
#89259=CARTESIAN_POINT('Ctrl Pts',(-20.8644257386545,18.6432620618645,123.018108220622)) ;
#89260=CARTESIAN_POINT('Ctrl Pts',(-20.9103608198524,18.6531487225985,123.2738391975)) ;
#89261=CARTESIAN_POINT('Ctrl Pts',(-20.9116439914806,18.663141831201,123.536431039595)) ;
#89262=CARTESIAN_POINT('Ctrl Pts',(-20.8674236850463,18.6730875298392,123.794025919388)) ;
#89263=CARTESIAN_POINT('Ctrl Pts',(-20.7796339406571,18.6830347521103,124.040260003737)) ;
#89264=CARTESIAN_POINT('Ctrl Pts',(-20.648865853499,18.6930827776904,124.269647102596)) ;
#89265=CARTESIAN_POINT('Ctrl Pts',(-20.4837880164837,18.7029300248333,124.468930982032)) ;
#89266=CARTESIAN_POINT('Ctrl Pts',(-20.2848353076597,18.712893201924,124.639124066068)) ;
#89267=CARTESIAN_POINT('Ctrl Pts',(-20.057643225627,18.7229229229575,124.772734603442)) ;
#89268=CARTESIAN_POINT('Ctrl Pts',(-19.8138733025437,18.7328273904903,124.864024891333)) ;
#89269=CARTESIAN_POINT('Ctrl Pts',(-19.5549244555012,18.7428518763201,124.91225661059)) ;
#89270=CARTESIAN_POINT('Ctrl Pts',(-19.2946394655604,18.752755711444,124.914979535986)) ;
#89271=CARTESIAN_POINT('Ctrl Pts',(-19.0340712151648,18.762806902154,124.871903053952)) ;
#89272=CARTESIAN_POINT('Ctrl Pts',(-18.7890046631621,18.7726913448123,124.785719653912)) ;
#89273=CARTESIAN_POINT('Ctrl Pts',(-18.5599429927726,18.7826843526642,124.657344067074)) ;
#89274=CARTESIAN_POINT('Ctrl Pts',(-18.3575852293697,18.7926326723805,124.491794444498)) ;
#89275=CARTESIAN_POINT('Ctrl Pts',(-18.1869857767214,18.8025695110899,124.294126119609)) ;
#89276=CARTESIAN_POINT('Ctrl Pts',(-18.0523654033191,18.8125525000095,124.068917991237)) ;
#89277=CARTESIAN_POINT('Ctrl Pts',(-17.9588008233373,18.8225963793736,123.822148861517)) ;
#89278=CARTESIAN_POINT('Ctrl Pts',(-17.9099472787027,18.832424444732,123.568497660891)) ;
#89279=CARTESIAN_POINT('Ctrl Pts',(-17.9056636523394,18.8425015332869,123.303776150982)) ;
#89280=CARTESIAN_POINT('Ctrl Pts',(-17.9463206545568,18.8523516854432,123.048068626949)) ;
#89281=CARTESIAN_POINT('Ctrl Pts',(-18.0325884242925,18.8624321658956,122.797675319086)) ;
#89282=CARTESIAN_POINT('Ctrl Pts',(-18.1574960786457,18.8722466636644,122.571957568326)) ;
#89283=CARTESIAN_POINT('Ctrl Pts',(-18.3234918042426,18.8823149596845,122.366002659658)) ;
#89284=CARTESIAN_POINT('Ctrl Pts',(-18.5195168321674,18.8922137921673,122.194898302409)) ;
#89285=CARTESIAN_POINT('Ctrl Pts',(-18.7455899254507,18.9022666721818,122.058322027411)) ;
#89286=CARTESIAN_POINT('Ctrl Pts',(-18.9874685791596,18.912136487678,121.96454261231)) ;
#89287=CARTESIAN_POINT('Ctrl Pts',(-19.247074514884,18.9222091687608,121.913098195303)) ;
#89288=CARTESIAN_POINT('Ctrl Pts',(-19.5054282253465,18.9320416473318,121.907540984529)) ;
#89289=CARTESIAN_POINT('Ctrl Pts',(-19.7660476083419,18.9420722813179,121.946964015993)) ;
#89290=CARTESIAN_POINT('Ctrl Pts',(-20.015663124333,18.952103838537,122.031786628564)) ;
#89291=CARTESIAN_POINT('Ctrl Pts',(-20.242340733487,18.9619335474087,122.155620704585)) ;
#89292=CARTESIAN_POINT('Ctrl Pts',(-20.4478596794803,18.9719229962108,122.318956902595)) ;
#89293=CARTESIAN_POINT('Ctrl Pts',(-20.6223353947974,18.9819668486108,122.517002479713)) ;
#89294=CARTESIAN_POINT('Ctrl Pts',(-20.7571909721581,18.9917885619429,122.737075061606)) ;
#89295=CARTESIAN_POINT('Ctrl Pts',(-20.8544420213186,19.0018235669316,122.982196100149)) ;
#89296=CARTESIAN_POINT('Ctrl Pts',(-20.9068867752531,19.0118484053792,123.24037432519)) ;
#89297=CARTESIAN_POINT('Ctrl Pts',(-20.9141429657687,19.0217006183344,123.499179168148)) ;
#89298=CARTESIAN_POINT('Ctrl Pts',(-20.8762673910892,19.0316905745282,123.758937854536)) ;
#89299=CARTESIAN_POINT('Ctrl Pts',(-20.7943862514496,19.0416186848114,124.00666549439)) ;
#89300=CARTESIAN_POINT('Ctrl Pts',(-20.6703510230735,19.051607284891,124.238008956621)) ;
#89301=CARTESIAN_POINT('Ctrl Pts',(-20.5071291776537,19.0616338768185,124.444859269663)) ;
#89302=CARTESIAN_POINT('Ctrl Pts',(-20.3134350002054,19.0715190048827,124.617949216475)) ;
#89303=CARTESIAN_POINT('Ctrl Pts',(-20.0905630047009,19.0815101223562,124.756761630848)) ;
#89304=CARTESIAN_POINT('Ctrl Pts',(-19.8455702342905,19.091550738208,124.854732580101)) ;
#89305=CARTESIAN_POINT('Ctrl Pts',(-19.5927186533089,19.1013837290617,124.907978535889)) ;
#89306=CARTESIAN_POINT('Ctrl Pts',(-19.3302830880624,19.111376860512,124.917403980521)) ;
#89307=CARTESIAN_POINT('Ctrl Pts',(-19.0692443271857,19.1214089089474,124.880431822587)) ;
#89308=CARTESIAN_POINT('Ctrl Pts',(-18.8226828953735,19.1312741554898,124.800366929372)) ;
#89309=CARTESIAN_POINT('Ctrl Pts',(-18.5911601979227,19.1412360303166,124.678161518773)) ;
#89310=CARTESIAN_POINT('Ctrl Pts',(-18.3831390570505,19.1512709934279,124.516107567008)) ;
#89311=CARTESIAN_POINT('Ctrl Pts',(-18.2086970669107,19.1611558378903,124.323580061315)) ;
#89312=CARTESIAN_POINT('Ctrl Pts',(-18.0679004045374,19.171221890731,124.099692955036)) ;
#89313=CARTESIAN_POINT('Ctrl Pts',(-17.9700782692514,19.18105940664,123.860343413881)) ;
#89314=CARTESIAN_POINT('Ctrl Pts',(-17.9137587529611,19.1911281547489,123.601857544703)) ;
#89315=CARTESIAN_POINT('Ctrl Pts',(-17.9034670306657,19.2010086717799,123.342371871998)) ;
#89316=CARTESIAN_POINT('Ctrl Pts',(-17.9382401306853,19.2109998587144,123.08216562488)) ;
#89317=CARTESIAN_POINT('Ctrl Pts',(-18.017346517817,19.2209529249893,122.83281725219)) ;
#89318=CARTESIAN_POINT('Ctrl Pts',(-18.1396020443988,19.2309887625219,122.599158531839)) ;
#89319=CARTESIAN_POINT('Ctrl Pts',(-18.2981172600277,19.2408788887333,122.393170709056)) ;
#89320=CARTESIAN_POINT('Ctrl Pts',(-18.4916634610177,19.2508710706413,122.215735660309)) ;
#89321=CARTESIAN_POINT('Ctrl Pts',(-18.7121126054784,19.2608170105799,122.075322038536)) ;
#89322=CARTESIAN_POINT('Ctrl Pts',(-18.9534330921312,19.270764194344,121.974810909958)) ;
#89323=CARTESIAN_POINT('Ctrl Pts',(-19.2111660245585,19.2808121326514,121.917443070718)) ;
#89324=CARTESIAN_POINT('Ctrl Pts',(-19.46968806927,19.2906597673917,121.905712436638)) ;
#89325=CARTESIAN_POINT('Ctrl Pts',(-19.7293828802566,19.3006214813655,121.938618525281)) ;
#89326=CARTESIAN_POINT('Ctrl Pts',(-19.9810273924312,19.3106501161564,122.01696448955)) ;
#89327=CARTESIAN_POINT('Ctrl Pts',(-20.2124964374937,19.3205604347535,122.136300351223)) ;
#89328=CARTESIAN_POINT('Ctrl Pts',(-20.4206742458988,19.330495291065,122.293871266416)) ;
#89329=CARTESIAN_POINT('Ctrl Pts',(-20.6000312207341,19.3405365270257,122.487400631673)) ;
#89330=CARTESIAN_POINT('Ctrl Pts',(-20.7410617512557,19.3504232986057,122.705636493677)) ;
#89331=CARTESIAN_POINT('Ctrl Pts',(-20.8434829085783,19.3604234773119,122.947608430064)) ;
#89332=CARTESIAN_POINT('Ctrl Pts',(-20.9020842657226,19.3703407555215,123.201594819178)) ;
#89333=CARTESIAN_POINT('Ctrl Pts',(-20.9157885273105,19.3803880019352,123.465233400112)) ;
#89334=CARTESIAN_POINT('Ctrl Pts',(-20.8843312394049,19.3902618909165,123.722835831488)) ;
#89335=CARTESIAN_POINT('Ctrl Pts',(-20.8073413256974,19.400323908497,123.975764420132)) ;
#89336=CARTESIAN_POINT('Ctrl Pts',(-20.6898211294301,19.4101949702313,124.207038033062)) ;
#89337=CARTESIAN_POINT('Ctrl Pts',(-20.5325845494946,19.4201890335916,124.417401603479)) ;
#89338=CARTESIAN_POINT('Ctrl Pts',(-20.3400856995338,19.430221191625,124.59752229965)) ;
#89339=CARTESIAN_POINT('Ctrl Pts',(-20.1232221891283,19.4400850678652,124.739562342653)) ;
#89340=CARTESIAN_POINT('Ctrl Pts',(-19.8800650899672,19.4501555825034,124.843936496975)) ;
#89341=CARTESIAN_POINT('Ctrl Pts',(-19.6283151955898,19.4599962194444,124.903158307787)) ;
#89342=CARTESIAN_POINT('Ctrl Pts',(-19.3668809125715,19.4699633482846,124.91881772904)) ;
#89343=CARTESIAN_POINT('Ctrl Pts',(-19.1054682843621,19.4799773214091,124.888425374719)) ;
#89344=CARTESIAN_POINT('Ctrl Pts',(-18.7709161948087,19.4932620552724,124.788603773578)) ;
#89345=CARTESIAN_POINT('Ctrl Pts',(-18.4713172138264,19.5064873199872,124.604876555852)) ;
#89346=CARTESIAN_POINT('Ctrl Pts',(-18.2302531727005,19.519797842542,124.351369013514)) ;
#89347=CARTESIAN_POINT('Ctrl Pts',(-18.0847512811712,19.5298264874442,124.131644354945)) ;
#89348=CARTESIAN_POINT('Ctrl Pts',(-17.9809400631191,19.5397075197981,123.89362910154)) ;
#89349=CARTESIAN_POINT('Ctrl Pts',(-17.9188886192552,19.5496884924782,123.638788056693)) ;
#89350=CARTESIAN_POINT('Ctrl Pts',(-17.902254691945,19.5596696200642,123.377037428699)) ;
#89351=CARTESIAN_POINT('Ctrl Pts',(-17.9400916999754,19.5729128103256,123.031015386685)) ;
#89352=CARTESIAN_POINT('Ctrl Pts',(-18.1006952198866,19.5895808056864,122.618253916938)) ;
#89353=CARTESIAN_POINT('Ctrl Pts',(-18.3897868588537,19.6061013056984,122.287674714517)) ;
#89354=CARTESIAN_POINT('Ctrl Pts',(-18.6800761568763,19.6194143220144,122.092482801336)) ;
#89355=CARTESIAN_POINT('Ctrl Pts',(-18.9182029603172,19.6293308802474,121.986519910248)) ;
#89356=CARTESIAN_POINT('Ctrl Pts',(-19.1738678812539,19.6393585485503,121.922922940547)) ;
#89357=CARTESIAN_POINT('Ctrl Pts',(-19.5194780323658,19.652539138295,121.898097021449)) ;
#89358=CARTESIAN_POINT('Ctrl Pts',(-19.9563288314783,19.6692872774143,121.982471851941)) ;
#89359=CARTESIAN_POINT('Ctrl Pts',(-20.4082007931077,19.6890820199249,122.252403503244)) ;
#89360=CARTESIAN_POINT('Ctrl Pts',(-20.7451774511471,19.7091264127337,122.664799510157)) ;
#89361=CARTESIAN_POINT('Ctrl Pts',(-20.9190665009058,19.7289655950324,123.162745067453)) ;
#89362=CARTESIAN_POINT('Ctrl Pts',(-20.9138754834601,19.7488909187253,123.692173591397)) ;
#89363=CARTESIAN_POINT('Ctrl Pts',(-20.7282061366091,19.7688145567768,124.188186165143)) ;
#89364=CARTESIAN_POINT('Ctrl Pts',(-20.384618994923,19.7887394302423,124.591086031158)) ;
#89365=CARTESIAN_POINT('Ctrl Pts',(-19.9254980781481,19.8086180373213,124.852590538209)) ;
#89366=CARTESIAN_POINT('Ctrl Pts',(-19.4021944235472,19.8285954801532,124.942415684017)) ;
#89367=CARTESIAN_POINT('Ctrl Pts',(-18.8808504945977,19.8485273282379,124.848110950266)) ;
#89368=CARTESIAN_POINT('Ctrl Pts',(-18.4236327836799,19.8684225965805,124.582537401173)) ;
#89369=CARTESIAN_POINT('Ctrl Pts',(-18.0835396042065,19.8883450949926,124.176670177314)) ;
#89370=CARTESIAN_POINT('Ctrl Pts',(-17.9021501379471,19.9083045768686,123.678122009356)) ;
#89371=CARTESIAN_POINT('Ctrl Pts',(-17.9016826808945,19.928182329328,123.14988706624)) ;
#89372=CARTESIAN_POINT('Ctrl Pts',(-18.0801848929392,19.9480641200625,122.652414260717)) ;
#89373=CARTESIAN_POINT('Ctrl Pts',(-18.4216899540666,19.9681374589135,122.242615414334)) ;
#89374=CARTESIAN_POINT('Ctrl Pts',(-18.8764503196767,19.9879419261493,121.977339845321)) ;
#89375=CARTESIAN_POINT('Ctrl Pts',(-19.398725666126,20.0079252665571,121.881194515216)) ;
#89376=CARTESIAN_POINT('Ctrl Pts',(-19.9205991086772,20.0278402311551,121.96959503457)) ;
#89377=CARTESIAN_POINT('Ctrl Pts',(-20.3807214883969,20.0477087658715,122.228929102253)) ;
#89378=CARTESIAN_POINT('Ctrl Pts',(-20.7270865861408,20.0677611500832,122.633789392997)) ;
#89379=CARTESIAN_POINT('Ctrl Pts',(-20.9126916804623,20.0875351138724,123.125708607321)) ;
#89380=CARTESIAN_POINT('Ctrl Pts',(-20.9197926939565,20.1075894928938,123.658461280195)) ;
#89381=CARTESIAN_POINT('Ctrl Pts',(-20.7466018541178,20.127386230467,124.1554690317)) ;
#89382=CARTESIAN_POINT('Ctrl Pts',(-20.4126503321151,20.1473540428185,124.567785296605)) ;
#89383=CARTESIAN_POINT('Ctrl Pts',(-19.9576268829892,20.1673130188835,124.840673205932)) ;
#89384=CARTESIAN_POINT('Ctrl Pts',(-19.4386508322908,20.1872079371609,124.94188751217)) ;
#89385=CARTESIAN_POINT('Ctrl Pts',(-18.9161782831837,20.2071042496112,124.860571732585)) ;
#89386=CARTESIAN_POINT('Ctrl Pts',(-18.4521872012561,20.2270121829853,124.606170401089)) ;
#89387=CARTESIAN_POINT('Ctrl Pts',(-18.1022237455605,20.2469620732738,124.207890683089)) ;
#89388=CARTESIAN_POINT('Ctrl Pts',(-17.9093454009066,20.2668393037751,123.715999312751)) ;
#89389=CARTESIAN_POINT('Ctrl Pts',(-17.8955608540406,20.2868219726461,123.185097942073)) ;
#89390=CARTESIAN_POINT('Ctrl Pts',(-18.0637245954641,20.3067548592265,122.682641570739)) ;
#89391=CARTESIAN_POINT('Ctrl Pts',(-18.3925761888793,20.3266676052444,122.268015072213)) ;
#89392=CARTESIAN_POINT('Ctrl Pts',(-18.7672875195584,20.3432373265862,122.036639218976)) ;
#89393=CARTESIAN_POINT('Ctrl Pts',(-19.1020112523894,20.3565373378912,121.93602784581)) ;
#89394=CARTESIAN_POINT('Ctrl Pts',(-19.4482933884682,20.3698075256411,121.894667854607)) ;
#89395=CARTESIAN_POINT('Ctrl Pts',(-19.8857616860693,20.3864349080065,121.957330261882)) ;
#89396=CARTESIAN_POINT('Ctrl Pts',(-20.2753843629908,20.4030571977517,122.165611719854)) ;
#89397=CARTESIAN_POINT('Ctrl Pts',(-20.5295904307739,20.4163024121462,122.403368996714)) ;
#89398=CARTESIAN_POINT('Ctrl Pts',(-20.6866680641732,20.4262143771069,122.61117509767)) ;
#89399=CARTESIAN_POINT('Ctrl Pts',(-20.806737474672,20.4362730002714,122.846628519742)) ;
#89400=CARTESIAN_POINT('Ctrl Pts',(-20.8828053848385,20.4461131143872,123.093815056759)) ;
#89401=CARTESIAN_POINT('Ctrl Pts',(-20.9157850235484,20.4561788993448,123.356230024175)) ;
#89402=CARTESIAN_POINT('Ctrl Pts',(-20.9028213821857,20.4660622171327,123.615663268066)) ;
#89403=CARTESIAN_POINT('Ctrl Pts',(-20.8449589694743,20.4760516549913,123.871692434311)) ;
#89404=CARTESIAN_POINT('Ctrl Pts',(-20.74368006627,20.486015369044,124.113161475895)) ;
#89405=CARTESIAN_POINT('Ctrl Pts',(-20.6017961937113,20.4960103807032,124.334224144279)) ;
#89406=CARTESIAN_POINT('Ctrl Pts',(-20.4226668968658,20.5060466723975,124.527786878245)) ;
#89407=CARTESIAN_POINT('Ctrl Pts',(-20.2168574908497,20.5158930500909,124.684641027028)) ;
#89408=CARTESIAN_POINT('Ctrl Pts',(-19.9839816914647,20.5258779942416,124.805469402538)) ;
#89409=CARTESIAN_POINT('Ctrl Pts',(-19.7348364121739,20.5358149653716,124.883819573151)) ;
#89410=CARTESIAN_POINT('Ctrl Pts',(-19.4729804417369,20.5458647500033,124.917956892684)) ;
#89411=CARTESIAN_POINT('Ctrl Pts',(-19.2143536333705,20.5557152120808,124.906538794214)) ;
#89412=CARTESIAN_POINT('Ctrl Pts',(-18.9584230841274,20.5656872256012,124.850373618486)) ;
#89413=CARTESIAN_POINT('Ctrl Pts',(-18.7155134690777,20.5756823727206,124.75033150436)) ;
#89414=CARTESIAN_POINT('Ctrl Pts',(-18.4930284866175,20.5857163424567,124.608850714625)) ;
#89415=CARTESIAN_POINT('Ctrl Pts',(-18.301639069362,20.5955718881273,124.43432218421)) ;
#89416=CARTESIAN_POINT('Ctrl Pts',(-18.1409105781554,20.6055706451405,124.22651165924)) ;
#89417=CARTESIAN_POINT('Ctrl Pts',(-18.0196900933075,20.6154677803777,123.996357848347)) ;
#89418=CARTESIAN_POINT('Ctrl Pts',(-17.9389969296105,20.6255208762173,123.744826815494)) ;
#89419=CARTESIAN_POINT('Ctrl Pts',(-17.9037758541384,20.6354043849479,123.487479681158)) ;
#89420=CARTESIAN_POINT('Ctrl Pts',(-17.9132711224096,20.645399257594,123.225004546721)) ;
#89421=CARTESIAN_POINT('Ctrl Pts',(-17.9687399657228,20.6554192192297,122.96758422729)) ;
#89422=CARTESIAN_POINT('Ctrl Pts',(-18.0667172219578,20.6653245830296,122.726428828135)) ;
#89423=CARTESIAN_POINT('Ctrl Pts',(-18.2051112656729,20.6752651706371,122.504892851635)) ;
#89424=CARTESIAN_POINT('Ctrl Pts',(-18.3808832318701,20.6852679887378,122.309400454705)) ;
#89425=CARTESIAN_POINT('Ctrl Pts',(-18.5888185798447,20.6953027004619,122.147247116949)) ;
#89426=CARTESIAN_POINT('Ctrl Pts',(-18.8171665168026,20.7051476071992,122.025597143536)) ;
#89427=CARTESIAN_POINT('Ctrl Pts',(-19.0664811329135,20.7151334597682,121.943845159401)) ;
#89428=CARTESIAN_POINT('Ctrl Pts',(-19.3249386776779,20.7250682681813,121.906617308344)) ;
#89429=CARTESIAN_POINT('Ctrl Pts',(-19.5890636684313,20.7351257952623,121.915166166779)) ;
#89430=CARTESIAN_POINT('Ctrl Pts',(-19.8417720817048,20.7449474502594,121.967799082809)) ;
#89431=CARTESIAN_POINT('Ctrl Pts',(-20.0873597067846,20.7550034944324,122.065317687553)) ;
#89432=CARTESIAN_POINT('Ctrl Pts',(-20.3094854721539,20.7649442344776,122.202825084637)) ;
#89433=CARTESIAN_POINT('Ctrl Pts',(-20.5041808420828,20.7748483555505,122.375555985901)) ;
#89434=CARTESIAN_POINT('Ctrl Pts',(-20.6681287825517,20.7848958967047,122.582504505087)) ;
#89435=CARTESIAN_POINT('Ctrl Pts',(-20.7919881814226,20.7947946483051,122.811292280779)) ;
#89436=CARTESIAN_POINT('Ctrl Pts',(-20.8755740195429,20.8048431272709,123.061746962003)) ;
#89437=CARTESIAN_POINT('Ctrl Pts',(-20.9138090117843,20.8147306243546,123.318779270284)) ;
#89438=CARTESIAN_POINT('Ctrl Pts',(-20.9072479453517,20.8247237146527,123.581282226704)) ;
#89439=CARTESIAN_POINT('Ctrl Pts',(-20.8553241322653,20.834675884713,123.837624769112)) ;
#89440=CARTESIAN_POINT('Ctrl Pts',(-20.7601574063262,20.8446143046275,124.080820832448)) ;
#89441=CARTESIAN_POINT('Ctrl Pts',(-20.6237998714096,20.8545994347131,124.305038244249)) ;
#89442=CARTESIAN_POINT('Ctrl Pts',(-20.4494221518513,20.8646361241272,124.502900480269)) ;
#89443=CARTESIAN_POINT('Ctrl Pts',(-20.2473013388322,20.8744908081197,124.664842526609)) ;
#89444=CARTESIAN_POINT('Ctrl Pts',(-20.0170290666669,20.8844902921675,124.7913425284)) ;
#89445=CARTESIAN_POINT('Ctrl Pts',(-19.7708926225284,20.8943853809444,124.875346148885)) ;
#89446=CARTESIAN_POINT('Ctrl Pts',(-19.5096857275806,20.9044459355906,124.915966548158)) ;
#89447=CARTESIAN_POINT('Ctrl Pts',(-19.2508869429393,20.9142951999635,124.910873014686)) ;
#89448=CARTESIAN_POINT('Ctrl Pts',(-18.9922127135504,20.9243224524113,124.860678227348)) ;
#89449=CARTESIAN_POINT('Ctrl Pts',(-18.7463889477668,20.9343507499815,124.765668763576)) ;
#89450=CARTESIAN_POINT('Ctrl Pts',(-18.5246560820803,20.9441968789875,124.632331993503)) ;
#89451=CARTESIAN_POINT('Ctrl Pts',(-18.3260748632208,20.9541907843496,124.460462272426)) ;
#89452=CARTESIAN_POINT('Ctrl Pts',(-18.1602131738219,20.9642148820326,124.255803821438)) ;
#89453=CARTESIAN_POINT('Ctrl Pts',(-18.0338336778558,20.9741047098866,124.028700863845)) ;
#89454=CARTESIAN_POINT('Ctrl Pts',(-17.9475715523185,20.9840966913171,123.780706945075)) ;
#89455=CARTESIAN_POINT('Ctrl Pts',(-17.9059277190108,20.9940436960829,123.522648076826)) ;
#89456=CARTESIAN_POINT('Ctrl Pts',(-17.9092446774268,21.0039933474727,123.26119173999)) ;
#89457=CARTESIAN_POINT('Ctrl Pts',(-17.9585439446535,21.0140303504501,123.002085877506)) ;
#89458=CARTESIAN_POINT('Ctrl Pts',(-18.0505382977171,21.0239192588851,122.759033267901)) ;
#89459=CARTESIAN_POINT('Ctrl Pts',(-18.1842691504711,21.0339085913626,122.533148901569)) ;
#89460=CARTESIAN_POINT('Ctrl Pts',(-18.3548109388882,21.0438671467997,122.334658060956)) ;
#89461=CARTESIAN_POINT('Ctrl Pts',(-18.5556391649582,21.0537667180002,122.16926520889)) ;
#89462=CARTESIAN_POINT('Ctrl Pts',(-18.7855363124599,21.0638146432522,122.039439979611)) ;
#89463=CARTESIAN_POINT('Ctrl Pts',(-19.030698238794,21.0737099427782,121.952623471748)) ;
#89464=CARTESIAN_POINT('Ctrl Pts',(-19.291450065471,21.0837717992262,121.908950298832)) ;
#89465=CARTESIAN_POINT('Ctrl Pts',(-19.5501399989178,21.0936156456428,121.91111408291)) ;
#89466=CARTESIAN_POINT('Ctrl Pts',(-19.807740031436,21.1035785947709,121.957838664783)) ;
#89467=CARTESIAN_POINT('Ctrl Pts',(-20.0549347555783,21.1136126311989,122.049642784503)) ;
#89468=CARTESIAN_POINT('Ctrl Pts',(-20.2792391844421,21.1235000581569,122.180784673848)) ;
#89469=CARTESIAN_POINT('Ctrl Pts',(-20.4802501125778,21.1335144924933,122.350672310585)) ;
#89470=CARTESIAN_POINT('Ctrl Pts',(-20.6485231786559,21.1435494371282,122.553690979311)) ;
#89471=CARTESIAN_POINT('Ctrl Pts',(-20.776994667693,21.1533817871592,122.777909498819)) ;
#89472=CARTESIAN_POINT('Ctrl Pts',(-20.8667919124949,21.1634572262764,123.026935129347)) ;
#89473=CARTESIAN_POINT('Ctrl Pts',(-20.911151449371,21.173309691511,123.282075921991)) ;
#89474=CARTESIAN_POINT('Ctrl Pts',(-20.9107346702923,21.1833825690879,123.546735142883)) ;
#89475=CARTESIAN_POINT('Ctrl Pts',(-20.8653838187256,21.1932251652804,123.801404395061)) ;
#89476=CARTESIAN_POINT('Ctrl Pts',(-20.776098005712,21.2032055493957,124.048000989328)) ;
#89477=CARTESIAN_POINT('Ctrl Pts',(-20.6444053880161,21.2132240300445,124.275965170634)) ;
#89478=CARTESIAN_POINT('Ctrl Pts',(-20.4778156031857,21.2231073450449,124.47526543333)) ;
#89479=CARTESIAN_POINT('Ctrl Pts',(-20.2754160656576,21.2331756421353,124.645605897759)) ;
#89480=CARTESIAN_POINT('Ctrl Pts',(-20.0520068570127,21.2430057105076,124.775388910782)) ;
#89481=CARTESIAN_POINT('Ctrl Pts',(-19.8038192003743,21.253072502976,124.866829885988)) ;
#89482=CARTESIAN_POINT('Ctrl Pts',(-19.5479997475856,21.2629618364645,124.912863623908)) ;
#89483=CARTESIAN_POINT('Ctrl Pts',(-19.2852043849924,21.2729639678806,124.914202847899)) ;
#89484=CARTESIAN_POINT('Ctrl Pts',(-19.0280750006297,21.2828878375016,124.870388521691)) ;
#89485=CARTESIAN_POINT('Ctrl Pts',(-18.77960570535,21.2929313530188,124.781491000549)) ;
#89486=CARTESIAN_POINT('Ctrl Pts',(-18.5538025555048,21.3028135659071,124.653119146439)) ;
#89487=CARTESIAN_POINT('Ctrl Pts',(-18.3500349006823,21.3128816431265,124.484434278303)) ;
#89488=CARTESIAN_POINT('Ctrl Pts',(-18.1823229673718,21.3227201478607,124.28760693878)) ;
#89489=CARTESIAN_POINT('Ctrl Pts',(-18.0480641582105,21.3327829162901,124.059823359472)) ;
#89490=CARTESIAN_POINT('Ctrl Pts',(-17.9571706997418,21.3426799095728,123.816123607726)) ;
#89491=CARTESIAN_POINT('Ctrl Pts',(-17.9089560570351,21.3526111372076,123.559639960323)) ;
#89492=CARTESIAN_POINT('Ctrl Pts',(-17.9062641201702,21.3626532958498,123.295759494904)) ;
#89493=CARTESIAN_POINT('Ctrl Pts',(-17.9485807750656,21.3725400053808,123.039404443611)) ;
#89494=CARTESIAN_POINT('Ctrl Pts',(-18.0352662045675,21.3825329778094,122.791531975748)) ;
#89495=CARTESIAN_POINT('Ctrl Pts',(-18.1631733074527,21.392479172346,122.56359572005)) ;
#89496=CARTESIAN_POINT('Ctrl Pts',(-18.3282744150043,21.4024245471975,122.360963544721)) ;
#89497=CARTESIAN_POINT('Ctrl Pts',(-18.5284565572223,21.4124794665574,122.188538399723)) ;
#89498=CARTESIAN_POINT('Ctrl Pts',(-18.7500672200615,21.4223009860009,122.056167239099)) ;
#89499=CARTESIAN_POINT('Ctrl Pts',(-18.9971032250605,21.4323667547678,121.961729368594)) ;
#89500=CARTESIAN_POINT('Ctrl Pts',(-19.252665844166,21.4422686764229,121.912504687733)) ;
#89501=CARTESIAN_POINT('Ctrl Pts',(-19.516526510854,21.4523117352439,121.908111222315)) ;
#89502=CARTESIAN_POINT('Ctrl Pts',(-19.7735943063744,21.4622177292866,121.949174521215)) ;
#89503=CARTESIAN_POINT('Ctrl Pts',(-20.0206585177756,21.4721555023684,122.033793699405)) ;
#89504=CARTESIAN_POINT('Ctrl Pts',(-20.2514967965682,21.4821958661007,122.161575037695)) ;
#89505=CARTESIAN_POINT('Ctrl Pts',(-20.4536528904977,21.4920832098242,122.324826619752)) ;
#89506=CARTESIAN_POINT('Ctrl Pts',(-20.6265093028174,21.5020754403929,122.522468692439)) ;
#89507=CARTESIAN_POINT('Ctrl Pts',(-20.7617843910413,21.5120239681765,122.746204499775)) ;
#89508=CARTESIAN_POINT('Ctrl Pts',(-20.8563752029685,21.5219607518998,122.989574942634)) ;
#89509=CARTESIAN_POINT('Ctrl Pts',(-20.9078459005937,21.5319437526968,123.246853300404)) ;
#89510=CARTESIAN_POINT('Ctrl Pts',(-20.9134112422956,21.5419876395375,123.510706398789)) ;
#89511=CARTESIAN_POINT('Ctrl Pts',(-20.8745423295287,21.5518156631121,123.766077419227)) ;
#89512=CARTESIAN_POINT('Ctrl Pts',(-20.7899649656379,21.5618929113257,124.016964720075)) ;
#89513=CARTESIAN_POINT('Ctrl Pts',(-20.6660716447633,21.571742466631,124.244301696396)) ;
#89514=CARTESIAN_POINT('Ctrl Pts',(-20.5009218271621,21.5818251748287,124.451413147156)) ;
#89515=CARTESIAN_POINT('Ctrl Pts',(-20.3077024679785,21.5916377677552,124.622265315751)) ;
#89516=CARTESIAN_POINT('Ctrl Pts',(-20.082372609264,21.6017049600131,124.76077174282)) ;
#89517=CARTESIAN_POINT('Ctrl Pts',(-19.8403774418101,21.6116037894757,124.856379349723)) ;
#89518=CARTESIAN_POINT('Ctrl Pts',(-19.5816048957035,21.6216577806659,124.909420890267)) ;
#89519=CARTESIAN_POINT('Ctrl Pts',(-19.3222374612088,21.6315295054491,124.916826891635)) ;
#89520=CARTESIAN_POINT('Ctrl Pts',(-19.0604462619463,21.6415999475793,124.878403745685)) ;
#89521=CARTESIAN_POINT('Ctrl Pts',(-18.8151200955136,21.6514330260096,124.797161576374)) ;
#89522=CARTESIAN_POINT('Ctrl Pts',(-18.5827353405762,21.661463499511,124.672775000186)) ;
#89523=CARTESIAN_POINT('Ctrl Pts',(-18.3759109672851,21.6714950988097,124.509291299171)) ;
#89524=CARTESIAN_POINT('Ctrl Pts',(-18.2037611889679,21.6813247998478,124.316724488468)) ;
#89525=CARTESIAN_POINT('Ctrl Pts',(-18.0647714451557,21.6913142379043,124.094017139833)) ;
#89526=CARTESIAN_POINT('Ctrl Pts',(-17.9666536761754,21.7013581411204,123.848992514289)) ;
#89527=CARTESIAN_POINT('Ctrl Pts',(-17.9132395630017,21.7111796619339,123.596478590155)) ;
#89528=CARTESIAN_POINT('Ctrl Pts',(-17.9036603191974,21.721215386181,123.332930237762)) ;
#89529=CARTESIAN_POINT('Ctrl Pts',(-17.9406169716176,21.7312375401135,123.072144554952)) ;
#89530=CARTESIAN_POINT('Ctrl Pts',(-18.0205753951748,21.7410997718708,122.825638668101)) ;
#89531=CARTESIAN_POINT('Ctrl Pts',(-18.1426765255731,21.7510588423287,122.5941443993)) ;
#89532=CARTESIAN_POINT('Ctrl Pts',(-18.3046553200881,21.7610940147049,122.386052860544)) ;
#89533=CARTESIAN_POINT('Ctrl Pts',(-18.4970548092859,21.7709743998631,122.211659235178)) ;
#89534=CARTESIAN_POINT('Ctrl Pts',(-18.7206332905695,21.7810311144571,122.070794791818)) ;
#89535=CARTESIAN_POINT('Ctrl Pts',(-18.9610017685015,21.7909103830291,121.972655816629)) ;
#89536=CARTESIAN_POINT('Ctrl Pts',(-19.2174642405481,21.8009013405148,121.916435631599)) ;
#89537=CARTESIAN_POINT('Ctrl Pts',(-19.4811229674523,21.81094199915,121.906127926293)) ;
#89538=CARTESIAN_POINT('Ctrl Pts',(-19.7372102471354,21.820774978858,121.940589760359)) ;
#89539=CARTESIAN_POINT('Ctrl Pts',(-19.987662151828,21.8307681121077,122.019553890229)) ;
#89540=CARTESIAN_POINT('Ctrl Pts',(-20.221266587985,21.8408001644911,122.141771264833)) ;
#89541=CARTESIAN_POINT('Ctrl Pts',(-20.4268046448549,21.8506653934424,122.299749040127)) ;
#89542=CARTESIAN_POINT('Ctrl Pts',(-20.6040649592092,21.8606273346856,122.492404487236)) ;
#89543=CARTESIAN_POINT('Ctrl Pts',(-20.7458436231991,21.8706620497224,122.714735308757)) ;
#89544=CARTESIAN_POINT('Ctrl Pts',(-20.8457694698757,21.8805478200664,122.954570602703)) ;
#89545=CARTESIAN_POINT('Ctrl Pts',(-20.903532112246,21.8906104174552,123.212586648096)) ;
#89546=CARTESIAN_POINT('Ctrl Pts',(-20.9154805876386,21.9004608292904,123.471189998348)) ;
#89547=CARTESIAN_POINT('Ctrl Pts',(-20.882426858183,21.9104879985763,123.73260477288)) ;
#89548=CARTESIAN_POINT('Ctrl Pts',(-20.8038186859197,21.9205154792905,123.984131914222)) ;
#89549=CARTESIAN_POINT('Ctrl Pts',(-20.6854109255077,21.9303585318698,124.214093694813)) ;
#89550=CARTESIAN_POINT('Ctrl Pts',(-20.5270023291853,21.9403524353084,124.423570385325)) ;
#89551=CARTESIAN_POINT('Ctrl Pts',(-20.3336537691034,21.9503795580848,124.602604087814)) ;
#89552=CARTESIAN_POINT('Ctrl Pts',(-20.1153478377517,21.9602702629769,124.743677527019)) ;
#89553=CARTESIAN_POINT('Ctrl Pts',(-19.8735692667385,21.9702622898272,124.846083256019)) ;
#89554=CARTESIAN_POINT('Ctrl Pts',(-19.6188372985755,21.9802082713157,124.904607587831)) ;
#89555=CARTESIAN_POINT('Ctrl Pts',(-19.3577931878943,21.9901554439376,124.918542373026)) ;
#89556=CARTESIAN_POINT('Ctrl Pts',(-19.0957252140819,22.0002033852638,124.886329581241)) ;
#89557=CARTESIAN_POINT('Ctrl Pts',(-18.8481898209292,22.0100510190716,124.810847917876)) ;
#89558=CARTESIAN_POINT('Ctrl Pts',(-18.6144904935636,22.0200127337566,124.692911935522)) ;
#89559=CARTESIAN_POINT('Ctrl Pts',(-18.4035879139127,22.0300413666351,124.534852114603)) ;
#89560=CARTESIAN_POINT('Ctrl Pts',(-18.2254150484394,22.0399516921703,124.344920009527)) ;
#89561=CARTESIAN_POINT('Ctrl Pts',(-18.0819977432726,22.049886522642,124.126756044865)) ;
#89562=CARTESIAN_POINT('Ctrl Pts',(-17.9777399583878,22.059927855024,123.884350623129)) ;
#89563=CARTESIAN_POINT('Ctrl Pts',(-17.9179599830939,22.0698207284628,123.631344850412)) ;
#89564=CARTESIAN_POINT('Ctrl Pts',(-17.9022371535386,22.0797898942807,123.369827155738)) ;
#89565=CARTESIAN_POINT('Ctrl Pts',(-17.9327716986324,22.0898186279972,123.108078060828)) ;
#89566=CARTESIAN_POINT('Ctrl Pts',(-18.0314269334723,22.1030111467684,122.775654275456)) ;
#89567=CARTESIAN_POINT('Ctrl Pts',(-18.2167874151558,22.1163710148111,122.472935258562)) ;
#89568=CARTESIAN_POINT('Ctrl Pts',(-18.4689775945887,22.1295963519599,122.233681798304)) ;
#89569=CARTESIAN_POINT('Ctrl Pts',(-18.6872947818254,22.1395775778005,122.088312201797)) ;
#89570=CARTESIAN_POINT('Ctrl Pts',(-18.9290513962181,22.1496131447834,121.982956255966)) ;
#89571=CARTESIAN_POINT('Ctrl Pts',(-19.1809335406282,22.1594762227455,121.921719585)) ;
#89572=CARTESIAN_POINT('Ctrl Pts',(-19.4449971797,22.1695465215466,121.904746363636)) ;
#89573=CARTESIAN_POINT('Ctrl Pts',(-19.7020801434068,22.1793888201144,121.933241045844)) ;
#89574=CARTESIAN_POINT('Ctrl Pts',(-19.9535498675344,22.1893495182842,122.005881902579)) ;
#89575=CARTESIAN_POINT('Ctrl Pts',(-20.1901770423832,22.1993875524637,122.122446448014)) ;
#89576=CARTESIAN_POINT('Ctrl Pts',(-20.3998103087612,22.2092612893102,122.275407092462)) ;
#89577=CARTESIAN_POINT('Ctrl Pts',(-20.5832357329711,22.2193330732354,122.466165386452)) ;
#89578=CARTESIAN_POINT('Ctrl Pts',(-20.7274078859713,22.2291651944366,122.680609736101)) ;
#89579=CARTESIAN_POINT('Ctrl Pts',(-20.8349279101504,22.239198218462,122.921333612289)) ;
#89580=CARTESIAN_POINT('Ctrl Pts',(-20.8982607406429,22.2492140986587,123.176824810715)) ;
#89581=CARTESIAN_POINT('Ctrl Pts',(-20.9165125593692,22.2590976177529,123.43591069118)) ;
#89582=CARTESIAN_POINT('Ctrl Pts',(-20.8895476418826,22.2690880301166,123.697042256073)) ;
#89583=CARTESIAN_POINT('Ctrl Pts',(-20.794199097017,22.28235119332,124.032313731486)) ;
#89584=CARTESIAN_POINT('Ctrl Pts',(-20.6136506128505,22.2956287635712,124.335485744995)) ;
#89585=CARTESIAN_POINT('Ctrl Pts',(-20.3624307998912,22.3089590660778,124.579675665852)) ;
#89586=CARTESIAN_POINT('Ctrl Pts',(-20.1474734503822,22.3188577478942,124.726159691664)) ;
#89587=CARTESIAN_POINT('Ctrl Pts',(-19.9083044716856,22.3288472629417,124.8343602261)) ;
#89588=CARTESIAN_POINT('Ctrl Pts',(-19.6550143972876,22.3387953147168,124.89911320866)) ;
#89589=CARTESIAN_POINT('Ctrl Pts',(-19.3945571768419,22.3487367179953,124.919216158149)) ;
#89590=CARTESIAN_POINT('Ctrl Pts',(-19.0469801715719,22.3620233827762,124.885646801854)) ;
#89591=CARTESIAN_POINT('Ctrl Pts',(-18.6334919756593,22.378633804431,124.731055814575)) ;
#89592=CARTESIAN_POINT('Ctrl Pts',(-18.2305162797271,22.3985450666818,124.387992218144)) ;
#89593=CARTESIAN_POINT('Ctrl Pts',(-17.9681847100688,22.4184891958467,123.927340765981)) ;
#89594=CARTESIAN_POINT('Ctrl Pts',(-17.8789700282879,22.4384123584518,123.405435456902)) ;
#89595=CARTESIAN_POINT('Ctrl Pts',(-17.9722068017202,22.4583024808584,122.88499296031)) ;
#89596=CARTESIAN_POINT('Ctrl Pts',(-18.2392469664603,22.4783074344585,122.425313505132)) ;
#89597=CARTESIAN_POINT('Ctrl Pts',(-18.6435932599694,22.4981456914741,122.086755742294)) ;
#89598=CARTESIAN_POINT('Ctrl Pts',(-19.1427570950757,22.5181399922607,121.904630400796)) ;
#89599=CARTESIAN_POINT('Ctrl Pts',(-19.6712866823868,22.5380252343051,121.904256042346)) ;
#89600=CARTESIAN_POINT('Ctrl Pts',(-20.1684531083155,22.557900180781,122.082765057008)) ;
#89601=CARTESIAN_POINT('Ctrl Pts',(-20.5778666143493,22.5779332507221,122.423256582873)) ;
#89602=CARTESIAN_POINT('Ctrl Pts',(-20.8439539041053,22.5978217576225,122.879952432642)) ;
#89603=CARTESIAN_POINT('Ctrl Pts',(-20.9398901568453,22.6176766174038,123.398949134001)) ;
#89604=CARTESIAN_POINT('Ctrl Pts',(-20.8512776370932,22.6377274511915,123.92432167666)) ;
#89605=CARTESIAN_POINT('Ctrl Pts',(-20.5928105483306,22.6574933930808,124.381851942389)) ;
#89606=CARTESIAN_POINT('Ctrl Pts',(-20.1896636816174,22.6775061245401,124.728595251841)) ;
#89607=CARTESIAN_POINT('Ctrl Pts',(-19.6948416932879,22.6973989594837,124.915260290639)) ;
#89608=CARTESIAN_POINT('Ctrl Pts',(-19.1659292643134,22.7173059828232,124.922744509421)) ;
#89609=CARTESIAN_POINT('Ctrl Pts',(-18.6655675605648,22.7372212477239,124.749699013636)) ;
#89610=CARTESIAN_POINT('Ctrl Pts',(-18.2524453398778,22.7572529398836,124.413924653691)) ;
#89611=CARTESIAN_POINT('Ctrl Pts',(-17.9812029359813,22.7770959864566,123.961563010291)) ;
#89612=CARTESIAN_POINT('Ctrl Pts',(-17.8790677895418,22.7970125343564,123.442240253503)) ;
#89613=CARTESIAN_POINT('Ctrl Pts',(-17.9604555657489,22.8169447773477,122.918716094646)) ;
#89614=CARTESIAN_POINT('Ctrl Pts',(-18.2149597212616,22.836848612157,122.454982006216)) ;
#89615=CARTESIAN_POINT('Ctrl Pts',(-18.6119455544731,22.8567490123445,122.105477724641)) ;
#89616=CARTESIAN_POINT('Ctrl Pts',(-19.1055301645696,22.8766986887238,121.911730698857)) ;
#89617=CARTESIAN_POINT('Ctrl Pts',(-19.6351375624815,22.8966312129442,121.898173547559)) ;
#89618=CARTESIAN_POINT('Ctrl Pts',(-20.1374387737837,22.9165512219304,122.065632357375)) ;
#89619=CARTESIAN_POINT('Ctrl Pts',(-20.5530897144561,22.9365081281066,122.395063821693)) ;
#89620=CARTESIAN_POINT('Ctrl Pts',(-20.8308724977881,22.9563939676081,122.844830062582)) ;
#89621=CARTESIAN_POINT('Ctrl Pts',(-20.9388539512202,22.9763651397439,123.364411422884)) ;
#89622=CARTESIAN_POINT('Ctrl Pts',(-20.8643389626638,22.9961793367283,123.885825621413)) ;
#89623=CARTESIAN_POINT('Ctrl Pts',(-20.6149971103256,23.0161605226965,124.354606393768)) ;
#89624=CARTESIAN_POINT('Ctrl Pts',(-20.2875827610197,23.0327360280858,124.64946647421)) ;
#89625=CARTESIAN_POINT('Ctrl Pts',(-19.9761963329815,23.0460454759494,124.808750590775)) ;
#89626=CARTESIAN_POINT('Ctrl Pts',(-19.6403478940357,23.059413173726,124.911784399414)) ;
#89627=CARTESIAN_POINT('Ctrl Pts',(-19.2023596389031,23.0759037453919,124.927929061235)) ;
#89628=CARTESIAN_POINT('Ctrl Pts',(-18.6980186540393,23.0958240177247,124.767071885537)) ;
#89629=CARTESIAN_POINT('Ctrl Pts',(-18.3484072158521,23.1124410534457,124.497150544743)) ;
#89630=CARTESIAN_POINT('Ctrl Pts',(-18.1364154882604,23.1257319037268,124.219541419118)) ;
#89631=CARTESIAN_POINT('Ctrl Pts',(-18.0158927766921,23.1357009488813,123.986966551078)) ;
#89632=CARTESIAN_POINT('Ctrl Pts',(-17.937590459842,23.1456043395148,123.738742873997)) ;
#89633=CARTESIAN_POINT('Ctrl Pts',(-17.9031973751966,23.1556621256276,123.476711455943)) ;
#89634=CARTESIAN_POINT('Ctrl Pts',(-17.9143593563858,23.1655141622773,123.218025990263)) ;
#89635=CARTESIAN_POINT('Ctrl Pts',(-17.9896268659552,23.1788792864205,122.874973437508)) ;
#89636=CARTESIAN_POINT('Ctrl Pts',(-18.151401302181,23.1921053493835,122.562854577334)) ;
#89637=CARTESIAN_POINT('Ctrl Pts',(-18.3866165742264,23.2054089976658,122.304238650459)) ;
#89638=CARTESIAN_POINT('Ctrl Pts',(-18.5942744744476,23.2154005288288,122.143499851417)) ;
#89639=CARTESIAN_POINT('Ctrl Pts',(-18.8279217544426,23.2254399766281,122.02101181735)) ;
#89640=CARTESIAN_POINT('Ctrl Pts',(-19.0743059149406,23.235283752142,121.942132253362)) ;
#89641=CARTESIAN_POINT('Ctrl Pts',(-19.3342082548891,23.2452693935296,121.906215557607)) ;
#89642=CARTESIAN_POINT('Ctrl Pts',(-19.595203409344,23.2552061778914,121.915784532965)) ;
#89643=CARTESIAN_POINT('Ctrl Pts',(-19.8533817478491,23.2652560123588,121.971267328799)) ;
#89644=CARTESIAN_POINT('Ctrl Pts',(-20.0932669657549,23.2751064618619,122.068597590794)) ;
#89645=CARTESIAN_POINT('Ctrl Pts',(-20.3156335651349,23.285078475844,122.207190765456)) ;
#89646=CARTESIAN_POINT('Ctrl Pts',(-20.5110432440586,23.2950736336911,122.382771699199)) ;
#89647=CARTESIAN_POINT('Ctrl Pts',(-20.6733357401702,23.3051075600548,122.590562603099)) ;
#89648=CARTESIAN_POINT('Ctrl Pts',(-20.7952641776477,23.3149632684872,122.81909160789)) ;
#89649=CARTESIAN_POINT('Ctrl Pts',(-20.8771604366914,23.3249614178259,123.068699179642)) ;
#89650=CARTESIAN_POINT('Ctrl Pts',(-20.9143466504709,23.3348608209994,123.326212352676)) ;
#89651=CARTESIAN_POINT('Ctrl Pts',(-20.9061903378289,23.3449120178879,123.590193277281)) ;
#89652=CARTESIAN_POINT('Ctrl Pts',(-20.8532554613795,23.3547943417008,123.844458307403)) ;
#89653=CARTESIAN_POINT('Ctrl Pts',(-20.7564386685029,23.3647892373574,124.088610236154)) ;
#89654=CARTESIAN_POINT('Ctrl Pts',(-20.6179988147476,23.3748103367399,124.312644230857)) ;
#89655=CARTESIAN_POINT('Ctrl Pts',(-20.4449168413211,23.384717604602,124.507129660358)) ;
#89656=CARTESIAN_POINT('Ctrl Pts',(-20.240390604112,23.3946559484272,124.669516991948)) ;
#89657=CARTESIAN_POINT('Ctrl Pts',(-20.0093102113973,23.4046593677277,124.794907442227)) ;
#89658=CARTESIAN_POINT('Ctrl Pts',(-19.7590948886003,23.4146939184348,124.878100956568)) ;
#89659=CARTESIAN_POINT('Ctrl Pts',(-19.5031986835257,23.4245388680404,124.916298887153)) ;
#89660=CARTESIAN_POINT('Ctrl Pts',(-19.240901379397,23.4345247101533,124.909881080696)) ;
#89661=CARTESIAN_POINT('Ctrl Pts',(-18.9848919832439,23.4444595175224,124.858447576063)) ;
#89662=CARTESIAN_POINT('Ctrl Pts',(-18.7388649759424,23.4545170592357,124.761980421742)) ;
#89663=CARTESIAN_POINT('Ctrl Pts',(-18.5183526283299,23.4643386567478,124.627795609594)) ;
#89664=CARTESIAN_POINT('Ctrl Pts',(-18.3195736794291,23.4743949162283,124.453691135326)) ;
#89665=CARTESIAN_POINT('Ctrl Pts',(-18.1562934925279,23.4843348525287,124.249783586925)) ;
#89666=CARTESIAN_POINT('Ctrl Pts',(-18.0306337931109,23.4942419732731,124.021771235105)) ;
#89667=CARTESIAN_POINT('Ctrl Pts',(-17.9454129427096,23.5042848791984,123.771998892176)) ;
#89668=CARTESIAN_POINT('Ctrl Pts',(-17.9053473190908,23.5141926602976,123.514723390938)) ;
#89669=CARTESIAN_POINT('Ctrl Pts',(-17.9101532963783,23.5242030293,123.251696708579)) ;
#89670=CARTESIAN_POINT('Ctrl Pts',(-17.961184062847,23.5342338678688,122.993085702516)) ;
#89671=CARTESIAN_POINT('Ctrl Pts',(-18.0542237398046,23.5440867075085,122.751450868495)) ;
#89672=CARTESIAN_POINT('Ctrl Pts',(-18.1892126976711,23.5540747086735,122.526373711805)) ;
#89673=CARTESIAN_POINT('Ctrl Pts',(-18.3602268731788,23.5640035276526,122.329304006708)) ;
#89674=CARTESIAN_POINT('Ctrl Pts',(-18.5637893871461,23.5739912303749,122.163599331592)) ;
#89675=CARTESIAN_POINT('Ctrl Pts',(-18.7943337470643,23.5840272301776,122.035538227318)) ;
#89676=CARTESIAN_POINT('Ctrl Pts',(-19.0390033894445,23.593882099979,121.95058970854)) ;
#89677=CARTESIAN_POINT('Ctrl Pts',(-19.2983352169612,23.6038815304026,121.908467679911)) ;
#89678=CARTESIAN_POINT('Ctrl Pts',(-19.5583918752554,23.6137766478679,121.911699650908)) ;
#89679=CARTESIAN_POINT('Ctrl Pts',(-19.8181268029097,23.6238371413848,121.960855606037)) ;
#89680=CARTESIAN_POINT('Ctrl Pts',(-20.0602942162802,23.633686621586,122.052288166794)) ;
#89681=CARTESIAN_POINT('Ctrl Pts',(-20.2872341468449,23.6437130718498,122.186156421621)) ;
#89682=CARTESIAN_POINT('Ctrl Pts',(-20.4871135693957,23.6537443623279,122.358035384557)) ;
#89683=CARTESIAN_POINT('Ctrl Pts',(-20.6513848025357,23.6635857499797,122.55778850806)) ;
#89684=CARTESIAN_POINT('Ctrl Pts',(-20.7809994490433,23.6735891508709,122.786461903559)) ;
#89685=CARTESIAN_POINT('Ctrl Pts',(-20.8686943861811,23.6835735336621,123.033800795154)) ;
#89686=CARTESIAN_POINT('Ctrl Pts',(-20.9120896033788,23.6936126236755,123.2939975435)) ;
#89687=CARTESIAN_POINT('Ctrl Pts',(-20.9100555677439,23.7034584325847,123.552746650312)) ;
#89688=CARTESIAN_POINT('Ctrl Pts',(-20.8629995601481,23.7134428554037,123.810834394173)) ;
#89689=CARTESIAN_POINT('Ctrl Pts',(-20.7723339495502,23.7233824806449,124.055836429127)) ;
#89690=CARTESIAN_POINT('Ctrl Pts',(-20.6391535588763,23.7334221701635,124.283563391533)) ;
#89691=CARTESIAN_POINT('Ctrl Pts',(-20.4711070029557,23.7433103585821,124.481782915492)) ;
#89692=CARTESIAN_POINT('Ctrl Pts',(-20.2694803443746,23.7532998845842,124.649877833456)) ;
#89693=CARTESIAN_POINT('Ctrl Pts',(-20.042335267145,23.7632583859393,124.7798313255)) ;
#89694=CARTESIAN_POINT('Ctrl Pts',(-19.7977296828341,23.773157979943,124.868459892283)) ;
#89695=CARTESIAN_POINT('Ctrl Pts',(-19.5376387109747,23.7832058680643,124.913842306988)) ;
#89696=CARTESIAN_POINT('Ctrl Pts',(-19.2775559394141,23.7931012933098,124.913585868621)) ;
#89697=CARTESIAN_POINT('Ctrl Pts',(-19.0172389437925,23.8031626840104,124.867462659727)) ;
#89698=CARTESIAN_POINT('Ctrl Pts',(-18.774152370709,23.8130082676971,124.778813564933)) ;
#89699=CARTESIAN_POINT('Ctrl Pts',(-18.5470679864683,23.8229712410063,124.648540906934)) ;
#89700=CARTESIAN_POINT('Ctrl Pts',(-18.3449854684297,23.8329969078321,124.479471088792)) ;
#89701=CARTESIAN_POINT('Ctrl Pts',(-18.1771183031737,23.8429113856984,124.280226434427)) ;
#89702=CARTESIAN_POINT('Ctrl Pts',(-18.0449530498413,23.8528999003734,124.053415180834)) ;
#89703=CARTESIAN_POINT('Ctrl Pts',(-17.9542174865925,23.8629440112888,123.805578221622)) ;
#89704=CARTESIAN_POINT('Ctrl Pts',(-17.9082598864059,23.8727721488834,123.551388438519)) ;
#89705=CARTESIAN_POINT('Ctrl Pts',(-17.9069862290974,23.8828487169423,123.286644032258)) ;
#89706=CARTESIAN_POINT('Ctrl Pts',(-17.9505929400621,23.8927008788465,123.031379907163)) ;
#89707=CARTESIAN_POINT('Ctrl Pts',(-18.0395746759122,23.9027738408033,122.782125620061)) ;
#89708=CARTESIAN_POINT('Ctrl Pts',(-18.1675552431538,23.9126164028062,122.557328161597)) ;
#89709=CARTESIAN_POINT('Ctrl Pts',(-18.3342353084014,23.9225968393,122.35484385985)) ;
#89710=CARTESIAN_POINT('Ctrl Pts',(-18.5346335209383,23.9326151446244,122.184110750498)) ;
#89711=CARTESIAN_POINT('Ctrl Pts',(-18.7583418735152,23.9424991085438,122.052074633009)) ;
#89712=CARTESIAN_POINT('Ctrl Pts',(-19.0060227711856,23.9525649852824,121.959294062984)) ;
#89713=CARTESIAN_POINT('Ctrl Pts',(-19.2602154899171,23.9624040861433,121.911839822886)) ;
#89714=CARTESIAN_POINT('Ctrl Pts',(-19.5238406827779,23.972437169009,121.90852668778)) ;
#89715=CARTESIAN_POINT('Ctrl Pts',(-19.7836670395102,23.9824588542845,121.951641266166)) ;
#89716=CARTESIAN_POINT('Ctrl Pts',(-20.0283217952903,23.992325549383,122.037454405699)) ;
#89717=CARTESIAN_POINT('Ctrl Pts',(-20.256860421925,24.0022854391175,122.165053725248)) ;
#89718=CARTESIAN_POINT('Ctrl Pts',(-20.4610242017121,24.012320426943,122.331938946934)) ;
#89719=CARTESIAN_POINT('Ctrl Pts',(-20.6309297767146,24.0222071310173,122.528544653014)) ;
#89720=CARTESIAN_POINT('Ctrl Pts',(-20.7664224941324,24.0322722752502,122.755656874661)) ;
#89721=CARTESIAN_POINT('Ctrl Pts',(-20.858590344017,24.0421115659788,122.997281659938)) ;
#89722=CARTESIAN_POINT('Ctrl Pts',(-20.9088537868088,24.0521741234172,123.256862342196)) ;
#89723=CARTESIAN_POINT('Ctrl Pts',(-20.9129308819633,24.0620711746693,123.516929777868)) ;
#89724=CARTESIAN_POINT('Ctrl Pts',(-20.8725108015801,24.0720023814176,123.77475646931)) ;
#89725=CARTESIAN_POINT('Ctrl Pts',(-20.7867177695425,24.0820445656364,124.024315773816)) ;
#89726=CARTESIAN_POINT('Ctrl Pts',(-20.661034087862,24.0919311937473,124.251717624557)) ;
#89727=CARTESIAN_POINT('Ctrl Pts',(-20.4963706306924,24.1019244662797,124.456275571947)) ;
#89728=CARTESIAN_POINT('Ctrl Pts',(-20.2995736659004,24.1118695418212,124.628245533589)) ;
#89729=CARTESIAN_POINT('Ctrl Pts',(-20.0760604743478,24.1218190925494,124.763934584824)) ;
#89730=CARTESIAN_POINT('Ctrl Pts',(-19.8301158593886,24.1318584273974,124.859366095419)) ;
#89731=CARTESIAN_POINT('Ctrl Pts',(-19.5752990612999,24.1417445663413,124.910102290642)) ;
#89732=CARTESIAN_POINT('Ctrl Pts',(-19.3126616551709,24.151742679315,124.916221608112)) ;
#89733=CARTESIAN_POINT('Ctrl Pts',(-19.0549019437606,24.1616624416675,124.877102085613)) ;
#89734=CARTESIAN_POINT('Ctrl Pts',(-18.8048861129423,24.1717018372801,124.792908728752)) ;
#89735=CARTESIAN_POINT('Ctrl Pts',(-18.5763150218767,24.1816110230684,124.668144211837)) ;
#89736=CARTESIAN_POINT('Ctrl Pts',(-18.3718886839389,24.1915462072259,124.50573368631)) ;
#89737=CARTESIAN_POINT('Ctrl Pts',(-18.1971228535137,24.2015872646118,124.308047316945)) ;
#89738=CARTESIAN_POINT('Ctrl Pts',(-18.0612783306157,24.2114744226451,124.086547050275)) ;
#89739=CARTESIAN_POINT('Ctrl Pts',(-17.9645493227509,24.221466702321,123.842445202394)) ;
#89740=CARTESIAN_POINT('Ctrl Pts',(-17.9119696693637,24.2314152193661,123.586335183678)) ;
#89741=CARTESIAN_POINT('Ctrl Pts',(-17.9042989976674,24.2413519969365,123.325341447214)) ;
#89742=CARTESIAN_POINT('Ctrl Pts',(-17.9419176299516,24.2513350330834,123.06567537359)) ;
#89743=CARTESIAN_POINT('Ctrl Pts',(-18.0249900888699,24.2613787846771,122.815181470846)) ;
#89744=CARTESIAN_POINT('Ctrl Pts',(-18.1471098273281,24.2712073138897,122.587547692865)) ;
#89745=CARTESIAN_POINT('Ctrl Pts',(-18.3107425634225,24.2812826747984,122.379462252064)) ;
#89746=CARTESIAN_POINT('Ctrl Pts',(-18.5037560854593,24.2911392736856,122.206642338797)) ;
#89747=CARTESIAN_POINT('Ctrl Pts',(-18.7282169843324,24.3012022677035,122.066922869341)) ;
#89748=CARTESIAN_POINT('Ctrl Pts',(-18.9691137819942,24.311080201993,121.970094344382)) ;
#89749=CARTESIAN_POINT('Ctrl Pts',(-19.2261436370484,24.321080849551,121.915522158594)) ;
#89750=CARTESIAN_POINT('Ctrl Pts',(-19.4866572465794,24.3309986959891,121.906283510334)) ;
#89751=CARTESIAN_POINT('Ctrl Pts',(-19.7481874126353,24.3410498129947,121.942965407598)) ;
#89752=CARTESIAN_POINT('Ctrl Pts',(-19.995044655726,24.3509205483053,122.022786909086)) ;
#89753=CARTESIAN_POINT('Ctrl Pts',(-20.2288798534327,24.3609912555483,122.146628302463)) ;
#89754=CARTESIAN_POINT('Ctrl Pts',(-20.4328576975085,24.3708242630002,122.305301061164)) ;
#89755=CARTESIAN_POINT('Ctrl Pts',(-20.6102013492879,24.3808547553025,122.500299127757)) ;
#89756=CARTESIAN_POINT('Ctrl Pts',(-20.7503713756113,24.3908863503759,122.723582642861)) ;
#89757=CARTESIAN_POINT('Ctrl Pts',(-20.8481322685785,24.4007160495141,122.962664906748)) ;
#89758=CARTESIAN_POINT('Ctrl Pts',(-20.9045567151015,24.4107054993957,123.219049565126)) ;
#89759=CARTESIAN_POINT('Ctrl Pts',(-20.9149976124652,24.4207493572114,123.482781782384)) ;
#89760=CARTESIAN_POINT('Ctrl Pts',(-20.8808031916903,24.4305710478016,123.738611883266)) ;
#89761=CARTESIAN_POINT('Ctrl Pts',(-20.8016222714478,24.440606138342,123.990150687533)) ;
#89762=CARTESIAN_POINT('Ctrl Pts',(-20.6794652177334,24.4506306573247,124.223569827565)) ;
#89763=CARTESIAN_POINT('Ctrl Pts',(-20.5216485278088,24.4604905027349,124.429046599541)) ;
#89764=CARTESIAN_POINT('Ctrl Pts',(-20.3290856748974,24.4704502790506,124.60632034406)) ;
#89765=CARTESIAN_POINT('Ctrl Pts',(-20.1069640189552,24.4804784763652,124.748123595379)) ;
#89766=CARTESIAN_POINT('Ctrl Pts',(-19.8666180274097,24.4903860186555,124.848283735091)) ;
#89767=CARTESIAN_POINT('Ctrl Pts',(-19.6093832914182,24.5004186692194,124.905987754454)) ;
#89768=CARTESIAN_POINT('Ctrl Pts',(-19.3499154760575,24.510302625646,124.918048718704)) ;
#89769=CARTESIAN_POINT('Ctrl Pts',(-19.0894596086663,24.5202923270079,124.885168267668)) ;
#89770=CARTESIAN_POINT('Ctrl Pts',(-18.8375518685682,24.5303333222839,124.806629416254)) ;
#89771=CARTESIAN_POINT('Ctrl Pts',(-18.607775073596,24.5401662115523,124.688434190657)) ;
#89772=CARTESIAN_POINT('Ctrl Pts',(-18.3982021069512,24.5501593699197,124.530191196066)) ;
#89773=CARTESIAN_POINT('Ctrl Pts',(-18.2189836852721,24.5601914122718,124.336829304906)) ;
#89774=CARTESIAN_POINT('Ctrl Pts',(-18.0781826899015,24.5700566562302,124.119164288488)) ;
#89775=CARTESIAN_POINT('Ctrl Pts',(-17.9756353809418,24.5800185474762,123.878288988731)) ;
#89776=CARTESIAN_POINT('Ctrl Pts',(-17.9164583703033,24.5900534474947,123.621321390185)) ;
#89777=CARTESIAN_POINT('Ctrl Pts',(-17.9025709875067,24.5999385279093,123.361889607157)) ;
#89778=CARTESIAN_POINT('Ctrl Pts',(-17.9345306575501,24.6100037000341,123.0993606842)) ;
#89779=CARTESIAN_POINT('Ctrl Pts',(-18.009793838017,24.6198509347576,122.851745183802)) ;
#89780=CARTESIAN_POINT('Ctrl Pts',(-18.1285188816227,24.6298817460754,122.616416570995)) ;
#89781=CARTESIAN_POINT('Ctrl Pts',(-18.2864282941797,24.6398913619889,122.406008126817)) ;
#89782=CARTESIAN_POINT('Ctrl Pts',(-18.4763620674248,24.6498021413926,122.227839272266)) ;
#89783=CARTESIAN_POINT('Ctrl Pts',(-18.6944258490363,24.6597314071816,122.084521998851)) ;
#89784=CARTESIAN_POINT('Ctrl Pts',(-18.9368657879906,24.6697741004942,121.980279706775)) ;
#89785=CARTESIAN_POINT('Ctrl Pts',(-19.1897153085028,24.679660633189,121.92048694765)) ;
#89786=CARTESIAN_POINT('Ctrl Pts',(-19.4518476983688,24.6896537782922,121.904901247144)) ;
#89787=CARTESIAN_POINT('Ctrl Pts',(-19.7114689211226,24.6995994589663,121.935024786244)) ;
#89788=CARTESIAN_POINT('Ctrl Pts',(-19.9621203216531,24.709546716593,122.009272431099)) ;
#89789=CARTESIAN_POINT('Ctrl Pts',(-20.1982874731001,24.7195946187145,122.127349372162)) ;
#89790=CARTESIAN_POINT('Ctrl Pts',(-20.4062771468984,24.7294423243362,122.281336350192)) ;
#89791=CARTESIAN_POINT('Ctrl Pts',(-20.5870191315301,24.7394037909703,122.470689270979)) ;
#89792=CARTESIAN_POINT('Ctrl Pts',(-20.7328443334499,24.7494333442385,122.690250749449)) ;
#89793=CARTESIAN_POINT('Ctrl Pts',(-20.8371756815299,24.7593402362659,122.928777696645)) ;
#89794=CARTESIAN_POINT('Ctrl Pts',(-20.8992448149416,24.7692878803789,123.182694125672)) ;
#89795=CARTESIAN_POINT('Ctrl Pts',(-20.9165397755815,24.7792879234078,123.444949438803)) ;
#89796=CARTESIAN_POINT('Ctrl Pts',(-20.8874649816599,24.7893266894018,123.707130191398)) ;
#89797=CARTESIAN_POINT('Ctrl Pts',(-20.8154023193973,24.7991517514241,123.955080646736)) ;
#89798=CARTESIAN_POINT('Ctrl Pts',(-20.6991263352566,24.8092062987504,124.192325406435)) ;
#89799=CARTESIAN_POINT('Ctrl Pts',(-20.5447671392046,24.8191495421996,124.403167472963)) ;
#89800=CARTESIAN_POINT('Ctrl Pts',(-20.3574869860895,24.8290517138075,124.58383784483)) ;
#89801=CARTESIAN_POINT('Ctrl Pts',(-20.1383185841272,24.8391045494177,124.731315017245)) ;
#89802=CARTESIAN_POINT('Ctrl Pts',(-19.901213310372,24.8489776071032,124.836683877999)) ;
#89803=CARTESIAN_POINT('Ctrl Pts',(-19.646468082972,24.8589728686289,124.900684701347)) ;
#89804=CARTESIAN_POINT('Ctrl Pts',(-19.3836496123046,24.8689982380494,124.919067997293)) ;
#89805=CARTESIAN_POINT('Ctrl Pts',(-19.1251299071319,24.878888070576,124.892249885578)) ;
#89806=CARTESIAN_POINT('Ctrl Pts',(-18.7890091715742,24.8921860413854,124.796799294934)) ;
#89807=CARTESIAN_POINT('Ctrl Pts',(-18.4874128569439,24.9053844364946,124.617566260999)) ;
#89808=CARTESIAN_POINT('Ctrl Pts',(-18.2417575404836,24.918779878774,124.365456812483)) ;
#89809=CARTESIAN_POINT('Ctrl Pts',(-18.0954573193109,24.928655717013,124.151048711038)) ;
#89810=CARTESIAN_POINT('Ctrl Pts',(-17.9865203150819,24.9387171196107,123.910175250881)) ;
#89811=CARTESIAN_POINT('Ctrl Pts',(-17.9222460999715,24.9485821765459,123.658987057165)) ;
#89812=CARTESIAN_POINT('Ctrl Pts',(-17.9018079283208,24.9585942724947,123.396707820689)) ;
#89813=CARTESIAN_POINT('Ctrl Pts',(-17.9355686586318,24.9718715816401,123.049393446101)) ;
#89814=CARTESIAN_POINT('Ctrl Pts',(-18.0899475407356,24.9884706071474,122.636126991343)) ;
#89815=CARTESIAN_POINT('Ctrl Pts',(-18.3760314708444,25.0050696551804,122.300327989926)) ;
#89816=CARTESIAN_POINT('Ctrl Pts',(-18.6623187112641,25.0183130672114,122.102384463216)) ;
#89817=CARTESIAN_POINT('Ctrl Pts',(-18.9019733035102,25.0283504948998,121.992225850964)) ;
#89818=CARTESIAN_POINT('Ctrl Pts',(-19.1537567559459,25.0382547968554,121.926273908146)) ;
#89819=CARTESIAN_POINT('Ctrl Pts',(-19.5011724762164,25.0515216368306,121.896923152544)) ;
#89820=CARTESIAN_POINT('Ctrl Pts',(-19.9361209211562,25.0681478349205,121.974892242463)) ;
#89821=CARTESIAN_POINT('Ctrl Pts',(-20.3941483506745,25.0880669503039,122.240432926128)) ;
#89822=CARTESIAN_POINT('Ctrl Pts',(-20.6778013141646,25.1046733734382,122.578575786354)) ;
#89823=CARTESIAN_POINT('Ctrl Pts',(-20.8254198064288,25.1179695939339,122.895276836921)) ;
#89824=CARTESIAN_POINT('Ctrl Pts',(-20.9163896664301,25.1312384262753,123.231970672834)) ;
#89825=CARTESIAN_POINT('Ctrl Pts',(-20.9167689419944,25.1479296743084,123.675492638632)) ;
#89826=CARTESIAN_POINT('Ctrl Pts',(-20.7380584204792,25.1677394059812,124.170815449789)) ;
#89827=CARTESIAN_POINT('Ctrl Pts',(-20.3990544179289,25.1877170133098,124.579453442232)) ;
#89828=CARTESIAN_POINT('Ctrl Pts',(-19.9416756734989,25.2076433223676,124.846325842365)) ;
#89829=CARTESIAN_POINT('Ctrl Pts',(-19.4236779184025,25.2274601825323,124.942437107342)) ;
#89830=CARTESIAN_POINT('Ctrl Pts',(-18.8970108487145,25.2475599981263,124.854014090052)) ;
#89831=CARTESIAN_POINT('Ctrl Pts',(-18.4395915110761,25.2673169620089,124.595686505518)) ;
#89832=CARTESIAN_POINT('Ctrl Pts',(-18.0924071157132,25.2873538880783,124.192105333411)) ;
#89833=CARTESIAN_POINT('Ctrl Pts',(-17.9060265000467,25.3072234704598,123.697842908581)) ;
#89834=CARTESIAN_POINT('Ctrl Pts',(-17.8981566895004,25.327128042213,123.168973851605)) ;
#89835=CARTESIAN_POINT('Ctrl Pts',(-18.0717642136479,25.3470806444115,122.667793933237)) ;
#89836=CARTESIAN_POINT('Ctrl Pts',(-18.4052645219479,25.3669901353818,122.257095727428)) ;
#89837=CARTESIAN_POINT('Ctrl Pts',(-18.8570067132281,25.3868415040812,121.984255857802)) ;
#89838=CARTESIAN_POINT('Ctrl Pts',(-19.3806239056403,25.4069217002172,121.881586989434)) ;
#89839=CARTESIAN_POINT('Ctrl Pts',(-19.9007576230194,25.4267226437926,121.962652492736)) ;
#89840=CARTESIAN_POINT('Ctrl Pts',(-20.3666506513675,25.4467066203021,122.217535832542)) ;
#89841=CARTESIAN_POINT('Ctrl Pts',(-20.7158407306792,25.4666225832777,122.615352102572)) ;
#89842=CARTESIAN_POINT('Ctrl Pts',(-20.9092753913654,25.4864930180996,123.10688621769)) ;
#89843=CARTESIAN_POINT('Ctrl Pts',(-20.9225933282135,25.5065433033327,123.63946964645)) ;
#89844=CARTESIAN_POINT('Ctrl Pts',(-20.7563011574428,25.526317272092,124.138248789555)) ;
#89845=CARTESIAN_POINT('Ctrl Pts',(-20.4256737839772,25.5463737302116,124.55612392467)) ;
#89846=CARTESIAN_POINT('Ctrl Pts',(-19.9778044990182,25.5661686132026,124.832472781124)) ;
#89847=CARTESIAN_POINT('Ctrl Pts',(-19.4586089000129,25.5861352685049,124.941740459474)) ;
#89848=CARTESIAN_POINT('Ctrl Pts',(-18.933405433002,25.6060942385814,124.866405585267)) ;
#89849=CARTESIAN_POINT('Ctrl Pts',(-18.4668441914665,25.6259903261715,124.617555781116)) ;
#89850=CARTESIAN_POINT('Ctrl Pts',(-18.1127144201242,25.6458884960831,124.224823959823)) ;
#89851=CARTESIAN_POINT('Ctrl Pts',(-17.9132301741929,25.6657943314502,123.734766837906)) ;
#89852=CARTESIAN_POINT('Ctrl Pts',(-17.8929228695584,25.6857442563881,123.204966867725)) ;
#89853=CARTESIAN_POINT('Ctrl Pts',(-18.0536111401075,25.7056234462985,122.701580140501)) ;
#89854=CARTESIAN_POINT('Ctrl Pts',(-18.377808589848,25.7256047705791,122.281003832198)) ;
#89855=CARTESIAN_POINT('Ctrl Pts',(-18.8251899843192,25.7455345547874,121.99718762822)) ;
#89856=CARTESIAN_POINT('Ctrl Pts',(-19.3420583616094,25.7654545441782,121.883074058097)) ;
#89857=CARTESIAN_POINT('Ctrl Pts',(-19.8655398108464,25.7853097395322,121.95081448643)) ;
#89858=CARTESIAN_POINT('Ctrl Pts',(-20.3385236962934,25.8053557411916,122.195787304325)) ;
#89859=CARTESIAN_POINT('Ctrl Pts',(-20.6359551620709,25.8218554884014,122.518224212841)) ;
#89860=CARTESIAN_POINT('Ctrl Pts',(-20.7997772299296,25.8352440928495,122.829543405343)) ;
#89861=CARTESIAN_POINT('Ctrl Pts',(-20.878806089281,25.8451059211844,123.076370301885)) ;
#89862=CARTESIAN_POINT('Ctrl Pts',(-20.9149660822381,25.855072063942,123.335767898469)) ;
#89863=CARTESIAN_POINT('Ctrl Pts',(-20.901681357157,25.8684338100669,123.686592876107)) ;
#89864=CARTESIAN_POINT('Ctrl Pts',(-20.7738066717889,25.884888139022,124.104963749759)) ;
#89865=CARTESIAN_POINT('Ctrl Pts',(-20.5060796437535,25.9016553840703,124.461005538212)) ;
#89866=CARTESIAN_POINT('Ctrl Pts',(-20.2328324341928,25.9148419493443,124.674328351222)) ;
#89867=CARTESIAN_POINT('Ctrl Pts',(-20.0014412245227,25.9248314080889,124.798165745444)) ;
#89868=CARTESIAN_POINT('Ctrl Pts',(-19.7528536304337,25.93478518057,124.879736163845)) ;
#89869=CARTESIAN_POINT('Ctrl Pts',(-19.4914876961368,25.9448329971027,124.917038232705)) ;
#89870=CARTESIAN_POINT('Ctrl Pts',(-19.2329656958291,25.9546745302252,124.908870993837)) ;
#89871=CARTESIAN_POINT('Ctrl Pts',(-18.9760196741983,25.9646607724449,124.85572458636)) ;
#89872=CARTESIAN_POINT('Ctrl Pts',(-18.7332872577401,25.9745973958698,124.759342505799)) ;
#89873=CARTESIAN_POINT('Ctrl Pts',(-18.5085731788918,25.9846472732528,124.620640269178)) ;
#89874=CARTESIAN_POINT('Ctrl Pts',(-18.3151059732975,25.9944977120304,124.448627307497)) ;
#89875=CARTESIAN_POINT('Ctrl Pts',(-18.1519582512238,26.0044697259991,124.243595958302)) ;
#89876=CARTESIAN_POINT('Ctrl Pts',(-18.0265942662714,26.0144648946252,124.012733796054)) ;
#89877=CARTESIAN_POINT('Ctrl Pts',(-17.94321575523,26.0244987778864,123.762605317723)) ;
#89878=CARTESIAN_POINT('Ctrl Pts',(-17.9048256332287,26.0343546479497,123.506445495096)) ;
#89879=CARTESIAN_POINT('Ctrl Pts',(-17.9111726656182,26.0443521938669,123.243825664362)) ;
#89880=CARTESIAN_POINT('Ctrl Pts',(-17.9624847437566,26.0542603207662,122.988545851874)) ;
#89881=CARTESIAN_POINT('Ctrl Pts',(-18.0578964910856,26.0642706922883,122.743382417585)) ;
#89882=CARTESIAN_POINT('Ctrl Pts',(-18.195192673543,26.0743011350357,122.518384012855)) ;
#89883=CARTESIAN_POINT('Ctrl Pts',(-18.3658649539483,26.084149087589,122.323819765035)) ;
#89884=CARTESIAN_POINT('Ctrl Pts',(-18.5719645952938,26.09421175661,122.158181340976)) ;
#89885=CARTESIAN_POINT('Ctrl Pts',(-18.7999511759967,26.1041061320739,122.033112687758)) ;
#89886=CARTESIAN_POINT('Ctrl Pts',(-19.0470918391407,26.1140479303921,121.948484295276)) ;
#89887=CARTESIAN_POINT('Ctrl Pts',(-19.3067989983835,26.1240504241194,121.907695937297)) ;
#89888=CARTESIAN_POINT('Ctrl Pts',(-19.5704318398782,26.1340852226263,121.913051573615)) ;
#89889=CARTESIAN_POINT('Ctrl Pts',(-19.824351246944,26.1439301066057,121.9627151315)) ;
#89890=CARTESIAN_POINT('Ctrl Pts',(-20.0693695516345,26.1539159634237,122.056561537333)) ;
#89891=CARTESIAN_POINT('Ctrl Pts',(-20.2933941815534,26.1638507775985,122.19072291664)) ;
#89892=CARTESIAN_POINT('Ctrl Pts',(-20.4929379375906,26.1739082773838,122.36397713695)) ;
#89893=CARTESIAN_POINT('Ctrl Pts',(-20.6558144439717,26.1837300358021,122.564237995494)) ;
#89894=CARTESIAN_POINT('Ctrl Pts',(-20.7848455998996,26.1937856935861,122.79482096552)) ;
#89895=CARTESIAN_POINT('Ctrl Pts',(-20.8704620781849,26.2037278757661,123.041679298249)) ;
#89896=CARTESIAN_POINT('Ctrl Pts',(-20.9125411179837,26.2136330844608,123.298550407497)) ;
#89897=CARTESIAN_POINT('Ctrl Pts',(-20.9092518862155,26.2236748754233,123.56241297677)) ;
#89898=CARTESIAN_POINT('Ctrl Pts',(-20.8608770737848,26.2335826498955,123.81825615933)) ;
#89899=CARTESIAN_POINT('Ctrl Pts',(-20.7683065805399,26.2435941501231,124.064531536108)) ;
#89900=CARTESIAN_POINT('Ctrl Pts',(-20.6336276204181,26.2536269105158,124.291186385178)) ;
#89901=CARTESIAN_POINT('Ctrl Pts',(-20.4651029134243,26.2634774796507,124.487687379059)) ;
#89902=CARTESIAN_POINT('Ctrl Pts',(-20.2625522855935,26.2734660891806,124.654609276642)) ;
#89903=CARTESIAN_POINT('Ctrl Pts',(-20.0354400287525,26.2833947452047,124.783063120699)) ;
#89904=CARTESIAN_POINT('Ctrl Pts',(-19.7881531187985,26.2933824913825,124.871070996956)) ;
#89905=CARTESIAN_POINT('Ctrl Pts',(-19.5280420904567,26.3034184803182,124.914573869556)) ;
#89906=CARTESIAN_POINT('Ctrl Pts',(-19.2690516259357,26.3132733501318,124.912723418728)) ;
#89907=CARTESIAN_POINT('Ctrl Pts',(-19.0105800370941,26.3232727913736,124.86560866309)) ;
#89908=CARTESIAN_POINT('Ctrl Pts',(-18.7666075707734,26.3331678655537,124.775514885921)) ;
#89909=CARTESIAN_POINT('Ctrl Pts',(-18.5383077888514,26.3432285213934,124.642249303302)) ;
#89910=CARTESIAN_POINT('Ctrl Pts',(-18.3407235540066,26.353077395589,124.475043878373)) ;
#89911=CARTESIAN_POINT('Ctrl Pts',(-18.1716552019844,26.3631061075523,124.272882308973)) ;
#89912=CARTESIAN_POINT('Ctrl Pts',(-18.040865209082,26.3731355081354,124.044055902173)) ;
#89913=CARTESIAN_POINT('Ctrl Pts',(-17.9529323432651,26.3829757017522,123.800871133778)) ;
#89914=CARTESIAN_POINT('Ctrl Pts',(-17.907349688925,26.3929791243274,123.542000520602)) ;
#89915=CARTESIAN_POINT('Ctrl Pts',(-17.9074933099312,26.4029646614205,123.279546917314)) ;
#89916=CARTESIAN_POINT('Ctrl Pts',(-17.9537071122485,26.4130056659073,123.019784028195)) ;
#89917=CARTESIAN_POINT('Ctrl Pts',(-18.0422247319121,26.4228492048485,122.776701044052)) ;
#89918=CARTESIAN_POINT('Ctrl Pts',(-18.172959280111,26.4328342358393,122.549236855608)) ;
#89919=CARTESIAN_POINT('Ctrl Pts',(-18.3404039267093,26.4427736983613,122.348721052526)) ;
#89920=CARTESIAN_POINT('Ctrl Pts',(-18.5421292540438,26.4528134305851,122.17870944488)) ;
#89921=CARTESIAN_POINT('Ctrl Pts',(-18.7668321702435,26.4627016109023,122.048175439295)) ;
#89922=CARTESIAN_POINT('Ctrl Pts',(-19.0130942013059,26.4726911266048,121.957267850095)) ;
#89923=CARTESIAN_POINT('Ctrl Pts',(-19.270636423452,26.4826496772595,121.910844672131)) ;
#89924=CARTESIAN_POINT('Ctrl Pts',(-19.5307953770956,26.4925490843645,121.909202223713)) ;
#89925=CARTESIAN_POINT('Ctrl Pts',(-19.7910846414141,26.5025976707808,121.953512811704)) ;
#89926=CARTESIAN_POINT('Ctrl Pts',(-20.0360368235489,26.5124904897453,122.040759031323)) ;
#89927=CARTESIAN_POINT('Ctrl Pts',(-20.2660528706653,26.5225616072751,122.171557281645)) ;
#89928=CARTESIAN_POINT('Ctrl Pts',(-20.4649953247139,26.5323773012411,122.335824675937)) ;
#89929=CARTESIAN_POINT('Ctrl Pts',(-20.6368891208767,26.5424436787384,122.536824123293)) ;
#89930=CARTESIAN_POINT('Ctrl Pts',(-20.7690314537872,26.5523426648203,122.760972791709)) ;
#89931=CARTESIAN_POINT('Ctrl Pts',(-20.8617289021231,26.5623968448138,123.008329329804)) ;
#89932=CARTESIAN_POINT('Ctrl Pts',(-20.9094601027412,26.5722676577465,123.263357508459)) ;
#89933=CARTESIAN_POINT('Ctrl Pts',(-20.9122321988059,26.5823415586003,123.528012047214)) ;
#89934=CARTESIAN_POINT('Ctrl Pts',(-20.8703917027367,26.592161713987,123.782723049251)) ;
#89935=CARTESIAN_POINT('Ctrl Pts',(-20.7829899901851,26.6022404209392,124.032674888992)) ;
#89936=CARTESIAN_POINT('Ctrl Pts',(-20.6564493553006,26.612092009478,124.25860286663)) ;
#89937=CARTESIAN_POINT('Ctrl Pts',(-20.4891684822601,26.622165126003,124.463697321808)) ;
#89938=CARTESIAN_POINT('Ctrl Pts',(-20.293323576881,26.6320076430988,124.632686826274)) ;
#89939=CARTESIAN_POINT('Ctrl Pts',(-20.0684805251643,26.6419881046528,124.76769750117)) ;
#89940=CARTESIAN_POINT('Ctrl Pts',(-19.8224939925488,26.6520063546435,124.861502416363)) ;
#89941=CARTESIAN_POINT('Ctrl Pts',(-19.5674893463834,26.6618905148373,124.91103746618)) ;
#89942=CARTESIAN_POINT('Ctrl Pts',(-19.3030567708649,26.6719556618123,124.915566855908)) ;
#89943=CARTESIAN_POINT('Ctrl Pts',(-19.0475793987206,26.6817974854531,124.875168472208)) ;
#89944=CARTESIAN_POINT('Ctrl Pts',(-18.7981276860572,26.6918269579139,124.79009847604)) ;
#89945=CARTESIAN_POINT('Ctrl Pts',(-18.5676426643981,26.701853813176,124.662390118096)) ;
#89946=CARTESIAN_POINT('Ctrl Pts',(-18.3661950342201,26.7116970632865,124.500120225689)) ;
#89947=CARTESIAN_POINT('Ctrl Pts',(-18.1921722448789,26.7217455028697,124.301522698417)) ;
#89948=CARTESIAN_POINT('Ctrl Pts',(-18.0569733160775,26.7316949971176,124.077726969622)) ;
#89949=CARTESIAN_POINT('Ctrl Pts',(-17.9623479206744,26.7416028528436,123.835146450497)) ;
#89950=CARTESIAN_POINT('Ctrl Pts',(-17.9107817759331,26.7516623294935,123.57590066682)) ;
#89951=CARTESIAN_POINT('Ctrl Pts',(-17.9047865023787,26.7615031389022,123.317331030199)) ;
#89952=CARTESIAN_POINT('Ctrl Pts',(-17.9443188755689,26.771565289203,123.055908426171)) ;
#89953=CARTESIAN_POINT('Ctrl Pts',(-18.0275281430875,26.7814624503255,122.809476370172)) ;
#89954=CARTESIAN_POINT('Ctrl Pts',(-18.1519197086005,26.7913936247296,122.580053321706)) ;
#89955=CARTESIAN_POINT('Ctrl Pts',(-18.3162992678989,26.8014358284546,122.373607725889)) ;
#89956=CARTESIAN_POINT('Ctrl Pts',(-18.5108502149347,26.8113224108851,122.201394321902)) ;
#89957=CARTESIAN_POINT('Ctrl Pts',(-18.7344911406208,26.8213158466334,122.063754577682)) ;
#89958=CARTESIAN_POINT('Ctrl Pts',(-18.9774833859817,26.8312603149915,121.96757970157)) ;
#89959=CARTESIAN_POINT('Ctrl Pts',(-19.2335820350933,26.8412121312371,121.91453316318)) ;
#89960=CARTESIAN_POINT('Ctrl Pts',(-19.4972322377189,26.8512495673516,121.906934424089)) ;
#89961=CARTESIAN_POINT('Ctrl Pts',(-19.754305398308,26.8611345265279,121.944403815041)) ;
#89962=CARTESIAN_POINT('Ctrl Pts',(-20.0038371906887,26.8711326447399,122.026561032475)) ;
#89963=CARTESIAN_POINT('Ctrl Pts',(-20.2336644999362,26.8810535772519,122.149706995992)) ;
#89964=CARTESIAN_POINT('Ctrl Pts',(-20.4411151613036,26.8910948774739,122.312763749208)) ;
#89965=CARTESIAN_POINT('Ctrl Pts',(-20.6146912031061,26.9010017958639,122.506803957199)) ;
#89966=CARTESIAN_POINT('Ctrl Pts',(-20.7529734778652,26.910937587573,122.728283521879)) ;
#89967=CARTESIAN_POINT('Ctrl Pts',(-20.8514823737436,26.9209784821509,122.973063068783)) ;
#89968=CARTESIAN_POINT('Ctrl Pts',(-20.9053481968387,26.9308656838647,123.227257943129)) ;
#89969=CARTESIAN_POINT('Ctrl Pts',(-20.9147883410893,26.9408579516263,123.489656489309)) ;
#89970=CARTESIAN_POINT('Ctrl Pts',(-20.8786067103794,26.9508064726481,123.74859249786)) ;
#89971=CARTESIAN_POINT('Ctrl Pts',(-20.7984720557952,26.9607432462258,123.997098137103)) ;
#89972=CARTESIAN_POINT('Ctrl Pts',(-20.676104628499,26.9707262943668,124.229192313943)) ;
#89973=CARTESIAN_POINT('Ctrl Pts',(-20.5139774785616,26.9807700019769,124.437430943901)) ;
#89974=CARTESIAN_POINT('Ctrl Pts',(-20.3227007873807,26.9905986951302,124.61104899263)) ;
#89975=CARTESIAN_POINT('Ctrl Pts',(-20.0988745919875,27.0006734442596,124.75238354413)) ;
#89976=CARTESIAN_POINT('Ctrl Pts',(-19.8589158285045,27.0105387700552,124.850593645606)) ;
#89977=CARTESIAN_POINT('Ctrl Pts',(-19.6017027315997,27.0205609444121,124.907173107382)) ;
#89978=CARTESIAN_POINT('Ctrl Pts',(-19.3384167298905,27.030586997619,124.917590734457)) ;
#89979=CARTESIAN_POINT('Ctrl Pts',(-19.0817902884042,27.0404406944653,124.883165473566)) ;
#89980=CARTESIAN_POINT('Ctrl Pts',(-18.8321269948554,27.0504000992183,124.804605397786)) ;
#89981=CARTESIAN_POINT('Ctrl Pts',(-18.5982965329107,27.0604383449232,124.682527849518)) ;
#89982=CARTESIAN_POINT('Ctrl Pts',(-18.3923088563404,27.0703125290852,124.524671749467)) ;
#89983=CARTESIAN_POINT('Ctrl Pts',(-18.213440473293,27.0803823122231,124.329704461917)) ;
#89984=CARTESIAN_POINT('Ctrl Pts',(-18.074335807759,27.0902155672439,124.111906520483)) ;
#89985=CARTESIAN_POINT('Ctrl Pts',(-17.9724962914812,27.1002459933756,123.868794804679)) ;
#89986=CARTESIAN_POINT('Ctrl Pts',(-17.9151518381184,27.1102776055626,123.61147237248)) ;
#89987=CARTESIAN_POINT('Ctrl Pts',(-17.9030590057314,27.1201073024172,123.353458137196)) ;
#89988=CARTESIAN_POINT('Ctrl Pts',(-17.9357095844985,27.1300967443197,123.092976875081)) ;
#89989=CARTESIAN_POINT('Ctrl Pts',(-18.0141505189305,27.1401406363354,122.840961680301)) ;
#89990=CARTESIAN_POINT('Ctrl Pts',(-18.1320070501894,27.1499621981046,122.611342543819)) ;
#89991=CARTESIAN_POINT('Ctrl Pts',(-18.2908176421164,27.1599977697288,122.400792255072)) ;
#89992=CARTESIAN_POINT('Ctrl Pts',(-18.4841896216697,27.1700270440106,122.221709205105)) ;
#89993=CARTESIAN_POINT('Ctrl Pts',(-18.7010325739723,27.1798608811293,122.08111845669)) ;
#89994=CARTESIAN_POINT('Ctrl Pts',(-18.9441365822861,27.1899132772174,121.97778844473)) ;
#89995=CARTESIAN_POINT('Ctrl Pts',(-19.1986307271689,27.1998500441679,121.919247113411)) ;
#89996=CARTESIAN_POINT('Ctrl Pts',(-19.4593067664465,27.2097842791472,121.905113637741)) ;
#89997=CARTESIAN_POINT('Ctrl Pts',(-19.7207933748905,27.219808042474,121.936899749053)) ;
#89998=CARTESIAN_POINT('Ctrl Pts',(-19.9693907811413,27.2296943838587,122.012371578883)) ;
#89999=CARTESIAN_POINT('Ctrl Pts',(-20.2037993675098,27.2396834326256,122.130541837784)) ;
#90000=CARTESIAN_POINT('Ctrl Pts',(-20.4148911017479,27.249724653323,122.288871926613)) ;
#90001=CARTESIAN_POINT('Ctrl Pts',(-20.5918449134471,27.2595572935009,122.477157471636)) ;
#90002=CARTESIAN_POINT('Ctrl Pts',(-20.7363711758217,27.2695512228089,122.696442446085)) ;
#90003=CARTESIAN_POINT('Ctrl Pts',(-20.8404837011343,27.2795804304894,122.938566164147)) ;
#90004=CARTESIAN_POINT('Ctrl Pts',(-20.9004632009322,27.2894562421935,123.191081286783)) ;
#90005=CARTESIAN_POINT('Ctrl Pts',(-20.9161620820543,27.2994554691649,123.453345856358)) ;
#90006=CARTESIAN_POINT('Ctrl Pts',(-20.8865937388302,27.3093649503206,123.712111167712)) ;
#90007=CARTESIAN_POINT('Ctrl Pts',(-20.8114565304405,27.3194181806215,123.9653601692)) ;
#90008=CARTESIAN_POINT('Ctrl Pts',(-20.695723180066,27.3292887971726,124.197519423031)) ;
#90009=CARTESIAN_POINT('Ctrl Pts',(-20.5395590565441,27.3393104589046,124.409577578881)) ;
#90010=CARTESIAN_POINT('Ctrl Pts',(-20.3484964827814,27.3493332720857,124.590894769313)) ;
#90011=CARTESIAN_POINT('Ctrl Pts',(-20.1325252181775,27.3592004365456,124.734373686293)) ;
#90012=CARTESIAN_POINT('Ctrl Pts',(-19.8921052555751,27.3691938787656,124.840061281651)) ;
#90013=CARTESIAN_POINT('Ctrl Pts',(-19.6358971489778,27.3792255523659,124.902135847813)) ;
#90014=CARTESIAN_POINT('Ctrl Pts',(-19.3771491513025,27.3890919874789,124.918905570282)) ;
#90015=CARTESIAN_POINT('Ctrl Pts',(-19.1162550336676,27.399079438012,124.890574288521)) ;
#90016=CARTESIAN_POINT('Ctrl Pts',(-18.8652095381394,27.4090243678399,124.817799802531)) ;
#90017=CARTESIAN_POINT('Ctrl Pts',(-18.6283777604426,27.4190692628951,124.701277213198)) ;
#90018=CARTESIAN_POINT('Ctrl Pts',(-18.4190826873744,27.4289313245809,124.548398528838)) ;
#90019=CARTESIAN_POINT('Ctrl Pts',(-18.23679990877,27.4389230473678,124.35943784464)) ;
#90020=CARTESIAN_POINT('Ctrl Pts',(-18.0910351330655,27.4488552616077,124.142920914045)) ;
#90021=CARTESIAN_POINT('Ctrl Pts',(-17.9844514742124,27.4587945801734,123.90445397346)) ;
#90022=CARTESIAN_POINT('Ctrl Pts',(-17.9204596210356,27.4688387549493,123.648382078966)) ;
#90023=CARTESIAN_POINT('Ctrl Pts',(-17.902082443692,27.4787093090143,123.389646586281)) ;
#90024=CARTESIAN_POINT('Ctrl Pts',(-17.9284117059881,27.4886742913685,123.129103791897)) ;
#90025=CARTESIAN_POINT('Ctrl Pts',(-18.0004358375775,27.4987049942583,122.875545886623)) ;
#90026=CARTESIAN_POINT('Ctrl Pts',(-18.1134828367361,27.5085973342835,122.641417708606)) ;
#90027=CARTESIAN_POINT('Ctrl Pts',(-18.2678736241984,27.5186505674435,122.427083046342)) ;
#90028=CARTESIAN_POINT('Ctrl Pts',(-18.4538449647151,27.5285318119202,122.245793517395)) ;
#90029=CARTESIAN_POINT('Ctrl Pts',(-18.6715808971833,27.5385649327912,122.097192547089)) ;
#90030=CARTESIAN_POINT('Ctrl Pts',(-18.9081664411668,27.5484461430663,121.990047207349)) ;
#90031=CARTESIAN_POINT('Ctrl Pts',(-19.1642609051452,27.5585082188356,121.924381854683)) ;
#90032=CARTESIAN_POINT('Ctrl Pts',(-19.4225664239136,27.5683652772174,121.904494754885)) ;
#90033=CARTESIAN_POINT('Ctrl Pts',(-19.6839699262157,27.5783598325064,121.929577621368)) ;
#90034=CARTESIAN_POINT('Ctrl Pts',(-19.9354082337427,27.5882857200419,121.999117799901)) ;
#90035=CARTESIAN_POINT('Ctrl Pts',(-20.1732877832902,27.5983107400372,122.112287014641)) ;
#90036=CARTESIAN_POINT('Ctrl Pts',(-20.3852469318587,27.6082081171408,122.263036295737)) ;
#90037=CARTESIAN_POINT('Ctrl Pts',(-20.5699322318413,27.6181983542217,122.44963382705)) ;
#90038=CARTESIAN_POINT('Ctrl Pts',(-20.7196829783269,27.6282349670305,122.666746029416)) ;
#90039=CARTESIAN_POINT('Ctrl Pts',(-20.8278068728803,27.6380848504485,122.901936609501)) ;
#90040=CARTESIAN_POINT('Ctrl Pts',(-20.8949783481644,27.648088467351,123.156067646929)) ;
#90041=CARTESIAN_POINT('Ctrl Pts',(-20.9168353812002,27.6580778791161,123.417709468201)) ;
#90042=CARTESIAN_POINT('Ctrl Pts',(-20.8927038903756,27.6680966404609,123.679858425827)) ;
#90043=CARTESIAN_POINT('Ctrl Pts',(-20.8017637690144,27.681315315842,124.015169943229)) ;
#90044=CARTESIAN_POINT('Ctrl Pts',(-20.624397640746,27.6946256230867,124.321149899939)) ;
#90045=CARTESIAN_POINT('Ctrl Pts',(-20.3779433771167,27.7078632893127,124.566721861766)) ;
#90046=CARTESIAN_POINT('Ctrl Pts',(-20.1646154796001,27.7177829847234,124.716537787326)) ;
#90047=CARTESIAN_POINT('Ctrl Pts',(-19.9252314219541,27.727835851722,124.828242513711)) ;
#90048=CARTESIAN_POINT('Ctrl Pts',(-19.6751407014436,27.7376912600512,124.895632476655)) ;
#90049=CARTESIAN_POINT('Ctrl Pts',(-19.412428193496,27.7477298917278,124.919430792106)) ;
#90050=CARTESIAN_POINT('Ctrl Pts',(-19.0641209038591,27.7610320739948,124.889619359484)) ;
#90051=CARTESIAN_POINT('Ctrl Pts',(-18.6502903905597,27.7775770870777,124.740836279188)) ;
#90052=CARTESIAN_POINT('Ctrl Pts',(-18.3098859245536,27.7942291031539,124.458090863763)) ;
#90053=CARTESIAN_POINT('Ctrl Pts',(-18.1090493187269,27.8074521940591,124.17447204272)) ;
#90054=CARTESIAN_POINT('Ctrl Pts',(-17.9965232918457,27.8174131536185,123.938133979673)) ;
#90055=CARTESIAN_POINT('Ctrl Pts',(-17.9266087730233,27.8274379503696,123.684145144491)) ;
#90056=CARTESIAN_POINT('Ctrl Pts',(-17.8934656932994,27.8406623977654,123.338168391895)) ;
#90057=CARTESIAN_POINT('Ctrl Pts',(-17.9661155358838,27.8572961824645,122.902139051415)) ;
#90058=CARTESIAN_POINT('Ctrl Pts',(-18.2260073081097,27.8771988491894,122.441354547989)) ;
#90059=CARTESIAN_POINT('Ctrl Pts',(-18.6269746119238,27.8970990769713,122.096481259438)) ;
#90060=CARTESIAN_POINT('Ctrl Pts',(-19.1218890723207,27.9170165645028,121.908622605301)) ;
#90061=CARTESIAN_POINT('Ctrl Pts',(-19.6515477387723,27.9369460903197,121.90059571952)) ;
#90062=CARTESIAN_POINT('Ctrl Pts',(-20.1529442502027,27.956908358206,122.07417484712)) ;
#90063=CARTESIAN_POINT('Ctrl Pts',(-20.5634708106491,27.9767985531582,122.407134552226)) ;
#90064=CARTESIAN_POINT('Ctrl Pts',(-20.8369751729256,27.9966887979044,122.859670241796)) ;
#90065=CARTESIAN_POINT('Ctrl Pts',(-20.9394668766951,28.0167631704669,123.383205991598)) ;
#90066=CARTESIAN_POINT('Ctrl Pts',(-20.8584842588624,28.0365485478272,123.902864524186)) ;
#90067=CARTESIAN_POINT('Ctrl Pts',(-20.6042776799615,28.0565104218943,124.368499119697)) ;
#90068=CARTESIAN_POINT('Ctrl Pts',(-20.2051858780569,28.0764903973848,124.718841264619)) ;
#90069=CARTESIAN_POINT('Ctrl Pts',(-19.7150043467851,28.0963028272628,124.911309469325)) ;
#90070=CARTESIAN_POINT('Ctrl Pts',(-19.1842604378428,28.1162829353531,124.925752106115)) ;
#90071=CARTESIAN_POINT('Ctrl Pts',(-18.6824773897549,28.1361773189503,124.758643613806)) ;
#90072=CARTESIAN_POINT('Ctrl Pts',(-18.2670496367191,28.1561042469275,124.430319759425)) ;
#90073=CARTESIAN_POINT('Ctrl Pts',(-17.9883198062167,28.1759991042288,123.980833693048)) ;
#90074=CARTESIAN_POINT('Ctrl Pts',(-17.8794805614305,28.1960382978324,123.459516608282)) ;
#90075=CARTESIAN_POINT('Ctrl Pts',(-17.9544486755063,28.2158782657432,122.937505697659)) ;
#90076=CARTESIAN_POINT('Ctrl Pts',(-18.2027332815713,28.2357930827073,122.470098177361)) ;
#90077=CARTESIAN_POINT('Ctrl Pts',(-18.5964066329864,28.2557353281035,122.115256848635)) ;
#90078=CARTESIAN_POINT('Ctrl Pts',(-19.0856168086369,28.275607376218,121.915866271612)) ;
#90079=CARTESIAN_POINT('Ctrl Pts',(-19.6169218061426,28.2956184411721,121.895642781133)) ;
#90080=CARTESIAN_POINT('Ctrl Pts',(-20.1188292935515,28.3154299654757,122.055652903489)) ;
#90081=CARTESIAN_POINT('Ctrl Pts',(-20.5414244265229,28.3355251774391,122.381920562138)) ;
#90082=CARTESIAN_POINT('Ctrl Pts',(-20.8229842740963,28.3553059013589,122.826156087312)) ;
#90083=CARTESIAN_POINT('Ctrl Pts',(-20.9383586766976,28.3752969770017,123.344606135062)) ;
#90084=CARTESIAN_POINT('Ctrl Pts',(-20.8698588440805,28.3951789160447,123.868727080192)) ;
#90085=CARTESIAN_POINT('Ctrl Pts',(-20.6263861212141,28.415131520548,124.33974290189)) ;
#90086=CARTESIAN_POINT('Ctrl Pts',(-20.2377379988083,28.4350303892786,124.69852394791)) ;
#90087=CARTESIAN_POINT('Ctrl Pts',(-19.7505120225895,28.4549237890882,124.903632562329)) ;
#90088=CARTESIAN_POINT('Ctrl Pts',(-19.2219604499456,28.4748329199282,124.931009679036)) ;
#90089=CARTESIAN_POINT('Ctrl Pts',(-18.7130412720916,28.4948650196918,124.774779736929)) ;
#90090=CARTESIAN_POINT('Ctrl Pts',(-18.3620584933981,28.5113970928613,124.510284590691)) ;
#90091=CARTESIAN_POINT('Ctrl Pts',(-18.1460674126106,28.5247324334672,124.234383966013)) ;
#90092=CARTESIAN_POINT('Ctrl Pts',(-18.0239856925731,28.5345749920069,124.006320082283)) ;
#90093=CARTESIAN_POINT('Ctrl Pts',(-17.9414030192515,28.5446268988568,123.755444503094)) ;
#90094=CARTESIAN_POINT('Ctrl Pts',(-17.8916917870985,28.5578754132477,123.410803822859)) ;
#90095=CARTESIAN_POINT('Ctrl Pts',(-17.9431871506201,28.5744745881955,122.972697293955)) ;
#90096=CARTESIAN_POINT('Ctrl Pts',(-18.1408539621108,28.5910633739905,122.578582469759)) ;
#90097=CARTESIAN_POINT('Ctrl Pts',(-18.3723983221645,28.6043391903325,122.317615113724)) ;
#90098=CARTESIAN_POINT('Ctrl Pts',(-18.577527292145,28.6143130411263,122.154436808147)) ;
#90099=CARTESIAN_POINT('Ctrl Pts',(-18.8092646056395,28.6243420732187,122.028922034954)) ;
#90100=CARTESIAN_POINT('Ctrl Pts',(-19.0557478273817,28.6342321987206,121.946437772454)) ;
#90101=CARTESIAN_POINT('Ctrl Pts',(-19.3153706733146,28.6442246769921,121.907264160908)) ;
#90102=CARTESIAN_POINT('Ctrl Pts',(-19.5768427425273,28.6541758920895,121.913598624698)) ;
#90103=CARTESIAN_POINT('Ctrl Pts',(-19.8356388835886,28.6642243938445,121.9659387871)) ;
#90104=CARTESIAN_POINT('Ctrl Pts',(-20.0765080850792,28.6740657434613,122.060169659542)) ;
#90105=CARTESIAN_POINT('Ctrl Pts',(-20.300843510358,28.6840520344815,122.196258449548)) ;
#90106=CARTESIAN_POINT('Ctrl Pts',(-20.4973109441294,28.6939886462101,122.368330827901)) ;
#90107=CARTESIAN_POINT('Ctrl Pts',(-20.6626341566035,28.7040385215777,122.57425065372)) ;
#90108=CARTESIAN_POINT('Ctrl Pts',(-20.7873624065296,28.7138889801131,122.801100887893)) ;
#90109=CARTESIAN_POINT('Ctrl Pts',(-20.8724691047688,28.7238609170659,123.048913631883)) ;
#90110=CARTESIAN_POINT('Ctrl Pts',(-20.9133208956479,28.733856373998,123.308428140769)) ;
#90111=CARTESIAN_POINT('Ctrl Pts',(-20.9081765057666,28.7438891810511,123.572012092005)) ;
#90112=CARTESIAN_POINT('Ctrl Pts',(-20.8585590805843,28.7537490676411,123.826338311456)) ;
#90113=CARTESIAN_POINT('Ctrl Pts',(-20.764789229398,28.7637381482063,124.071497059533)) ;
#90114=CARTESIAN_POINT('Ctrl Pts',(-20.6306361728563,28.7736696274155,124.295376547867)) ;
#90115=CARTESIAN_POINT('Ctrl Pts',(-20.4590320836787,28.7836554868614,124.493932716745)) ;
#90116=CARTESIAN_POINT('Ctrl Pts',(-20.2542272972785,28.7936936375086,124.660161314307)) ;
#90117=CARTESIAN_POINT('Ctrl Pts',(-20.0282560662824,28.803541728013,124.78635916123)) ;
#90118=CARTESIAN_POINT('Ctrl Pts',(-19.7786454124,28.813602636531,124.873435806326)) ;
#90119=CARTESIAN_POINT('Ctrl Pts',(-19.5219342752848,28.8234974836889,124.914980277803)) ;
#90120=CARTESIAN_POINT('Ctrl Pts',(-19.26072567087,28.833439155734,124.911999560869)) ;
#90121=CARTESIAN_POINT('Ctrl Pts',(-19.0023461124135,28.8434416828595,124.863503088264)) ;
#90122=CARTESIAN_POINT('Ctrl Pts',(-18.7557142855735,28.8534764740469,124.770209950683)) ;
#90123=CARTESIAN_POINT('Ctrl Pts',(-18.5330665031705,28.863321353906,124.638416591467)) ;
#90124=CARTESIAN_POINT('Ctrl Pts',(-18.3335959771311,28.8733072345245,124.467967806184)) ;
#90125=CARTESIAN_POINT('Ctrl Pts',(-18.1674022200289,28.8832419576177,124.266559871745)) ;
#90126=CARTESIAN_POINT('Ctrl Pts',(-18.0373647499672,28.8932997979289,124.036497815317)) ;
#90127=CARTESIAN_POINT('Ctrl Pts',(-17.950911814326,28.9031202853254,123.793301563566)) ;
#90128=CARTESIAN_POINT('Ctrl Pts',(-17.9065295280347,28.9131806866705,123.532709133583)) ;
#90129=CARTESIAN_POINT('Ctrl Pts',(-17.9084022908856,28.9231116522234,123.271710634104)) ;
#90130=CARTESIAN_POINT('Ctrl Pts',(-17.9550199869084,28.9330505145599,123.014749249068)) ;
#90131=CARTESIAN_POINT('Ctrl Pts',(-18.0458283672377,28.9430362454861,122.768516340365)) ;
#90132=CARTESIAN_POINT('Ctrl Pts',(-18.1787394441072,28.9530606309135,122.541096570347)) ;
#90133=CARTESIAN_POINT('Ctrl Pts',(-18.3467919785273,28.9629639152668,122.342338042519)) ;
#90134=CARTESIAN_POINT('Ctrl Pts',(-18.5499731696622,28.9730239198448,122.173252013428)) ;
#90135=CARTESIAN_POINT('Ctrl Pts',(-18.7744434743641,28.9828671889139,122.044654486055)) ;
#90136=CARTESIAN_POINT('Ctrl Pts',(-19.0212126462486,28.9928577545216,121.955119711378)) ;
#90137=CARTESIAN_POINT('Ctrl Pts',(-19.2782134163419,29.0027858863004,121.910108935023)) ;
#90138=CARTESIAN_POINT('Ctrl Pts',(-19.5406963148018,29.0127737733813,121.909949720142)) ;
#90139=CARTESIAN_POINT('Ctrl Pts',(-19.8003636387641,29.02280972295,121.956024596532)) ;
#90140=CARTESIAN_POINT('Ctrl Pts',(-20.0437946869578,29.0326646093288,122.0444605937)) ;
#90141=CARTESIAN_POINT('Ctrl Pts',(-20.2715846639012,29.0426640236767,122.175375625611)) ;
#90142=CARTESIAN_POINT('Ctrl Pts',(-20.4713275194905,29.0525591888672,122.34193965665)) ;
#90143=CARTESIAN_POINT('Ctrl Pts',(-20.6418433631902,29.0626195075592,122.543928922245)) ;
#90144=CARTESIAN_POINT('Ctrl Pts',(-20.7720825546946,29.0724696393352,122.767656038512)) ;
#90145=CARTESIAN_POINT('Ctrl Pts',(-20.8637061447357,29.0825002097855,123.014799627036)) ;
#90146=CARTESIAN_POINT('Ctrl Pts',(-20.9103762630913,29.0925143604583,123.273804452751)) ;
#90147=CARTESIAN_POINT('Ctrl Pts',(-20.9117741336975,29.1024072940037,123.53378141723)) ;
#90148=CARTESIAN_POINT('Ctrl Pts',(-20.867883240844,29.112396807994,123.792574654758)) ;
#90149=CARTESIAN_POINT('Ctrl Pts',(-20.7801810778798,29.1223505786464,124.039048417847)) ;
#90150=CARTESIAN_POINT('Ctrl Pts',(-20.6496213778519,29.132398347307,124.268526107138)) ;
#90151=CARTESIAN_POINT('Ctrl Pts',(-20.4848587379141,29.1422400737468,124.46791155322)) ;
#90152=CARTESIAN_POINT('Ctrl Pts',(-20.2855219341304,29.1522255905695,124.638505213354)) ;
#90153=CARTESIAN_POINT('Ctrl Pts',(-20.0606187506956,29.1621649222651,124.771401656305)) ;
#90154=CARTESIAN_POINT('Ctrl Pts',(-19.8136216179253,29.1722046919626,124.864082795799)) ;
#90155=CARTESIAN_POINT('Ctrl Pts',(-19.558187368143,29.1820928532114,124.911871502229)) ;
#90156=CARTESIAN_POINT('Ctrl Pts',(-19.2957011783519,29.1920824077138,124.915102448404)) ;
#90157=CARTESIAN_POINT('Ctrl Pts',(-19.0374781818425,29.2020408222374,124.872643060304)) ;
#90158=CARTESIAN_POINT('Ctrl Pts',(-18.7917703837319,29.2119407350668,124.787095968834)) ;
#90159=CARTESIAN_POINT('Ctrl Pts',(-18.5613536456222,29.2219874347167,124.65825660223)) ;
#90160=CARTESIAN_POINT('Ctrl Pts',(-18.3596420924881,29.2318872950223,124.493892512925)) ;
#90161=CARTESIAN_POINT('Ctrl Pts',(-18.1869148909575,29.2419386992278,124.294103199834)) ;
#90162=CARTESIAN_POINT('Ctrl Pts',(-18.0536769669931,29.2518197361489,124.071184737114)) ;
#90163=CARTESIAN_POINT('Ctrl Pts',(-17.9597521892141,29.2618195683264,123.825804732125)) ;
#90164=CARTESIAN_POINT('Ctrl Pts',(-17.9100403484687,29.2717375713113,123.569907928987)) ;
#90165=CARTESIAN_POINT('Ctrl Pts',(-17.9055429199268,29.2817888771858,123.305853384214)) ;
#90166=CARTESIAN_POINT('Ctrl Pts',(-17.9459174143974,29.2916587005774,123.049589465829)) ;
#90167=CARTESIAN_POINT('Ctrl Pts',(-18.0318972364498,29.3017328666277,122.799266072468)) ;
#90168=CARTESIAN_POINT('Ctrl Pts',(-18.1565829873438,29.3115529507693,122.573255953319)) ;
#90169=CARTESIAN_POINT('Ctrl Pts',(-18.3226099186623,29.3216316775052,122.36697855623)) ;
#90170=CARTESIAN_POINT('Ctrl Pts',(-18.5174760158988,29.3314832581547,122.196440883835)) ;
#90171=CARTESIAN_POINT('Ctrl Pts',(-18.7437589213341,29.3415563864531,122.059171973647)) ;
#90172=CARTESIAN_POINT('Ctrl Pts',(-18.9848715208291,29.3513988643445,121.965485865843)) ;
#90173=CARTESIAN_POINT('Ctrl Pts',(-19.2419396876553,29.3613794709426,121.913527744618)) ;
#90174=CARTESIAN_POINT('Ctrl Pts',(-19.5051237744955,29.3713971799614,121.907465724619)) ;
#90175=CARTESIAN_POINT('Ctrl Pts',(-19.7620431375332,29.3812833589988,121.946175909808)) ;
#90176=CARTESIAN_POINT('Ctrl Pts',(-20.0125730392579,29.3913409715712,122.030311528781)) ;
#90177=CARTESIAN_POINT('Ctrl Pts',(-20.2405533557099,29.4012173649433,122.154388504609)) ;
#90178=CARTESIAN_POINT('Ctrl Pts',(-20.4463541851592,29.4112123930937,122.317580930784)) ;
#90179=CARTESIAN_POINT('Ctrl Pts',(-20.6208172138511,29.4212331399397,122.514846934847)) ;
#90180=CARTESIAN_POINT('Ctrl Pts',(-20.7570016708868,29.4311352086061,122.736578720449)) ;
#90181=CARTESIAN_POINT('Ctrl Pts',(-20.8538352390123,29.4411259484258,122.980616710616)) ;
#90182=CARTESIAN_POINT('Ctrl Pts',(-20.9064868502557,29.4510891446361,123.23707769916)) ;
#90183=CARTESIAN_POINT('Ctrl Pts',(-20.914410419633,29.4609933289362,123.497253000178)) ;
#90184=CARTESIAN_POINT('Ctrl Pts',(-20.8762358005154,29.4710537893271,123.758827580412)) ;
#90185=CARTESIAN_POINT('Ctrl Pts',(-20.7953305897781,29.4808943351979,124.004481871684)) ;
#90186=CARTESIAN_POINT('Ctrl Pts',(-20.6705730749621,29.4909565559097,124.237592816873)) ;
#90187=CARTESIAN_POINT('Ctrl Pts',(-20.5096749757579,29.5008536989262,124.441955772106)) ;
#90188=CARTESIAN_POINT('Ctrl Pts',(-20.3156640114165,29.5107848753434,124.616506656617)) ;
#90189=CARTESIAN_POINT('Ctrl Pts',(-20.0916629418475,29.520827089122,124.756019382219)) ;
#90190=CARTESIAN_POINT('Ctrl Pts',(-19.8506899321232,29.5307136293248,124.853178323577)) ;
#90191=CARTESIAN_POINT('Ctrl Pts',(-19.5938766834909,29.5407072239302,124.908009663912)) ;
#90192=CARTESIAN_POINT('Ctrl Pts',(-19.332712747215,29.5506510990877,124.917331744836)) ;
#90193=CARTESIAN_POINT('Ctrl Pts',(-19.0734479879124,29.5606116352025,124.881449299093)) ;
#90194=CARTESIAN_POINT('Ctrl Pts',(-18.8233593876915,29.5706082385252,124.800941689882)) ;
#90195=CARTESIAN_POINT('Ctrl Pts',(-18.5904051560722,29.5806413214798,124.677470404879)) ;
#90196=CARTESIAN_POINT('Ctrl Pts',(-18.3859961074744,29.5904924901813,124.518621309858)) ;
#90197=CARTESIAN_POINT('Ctrl Pts',(-18.2097416401463,29.6004549808802,124.325047682833)) ;
#90198=CARTESIAN_POINT('Ctrl Pts',(-18.0691118335263,29.6104834092979,124.102151585275)) ;
#90199=CARTESIAN_POINT('Ctrl Pts',(-17.9704269675126,29.6203937766625,123.861151262509)) ;
#90200=CARTESIAN_POINT('Ctrl Pts',(-17.9142776230811,29.6303286442776,123.606174600459)) ;
#90201=CARTESIAN_POINT('Ctrl Pts',(-17.9033816131702,29.6403697862566,123.342537736076)) ;
#90202=CARTESIAN_POINT('Ctrl Pts',(-17.9377116774726,29.6502569224598,123.084976886491)) ;
#90203=CARTESIAN_POINT('Ctrl Pts',(-18.0166487960382,29.6602492048632,122.834555046718)) ;
#90204=CARTESIAN_POINT('Ctrl Pts',(-18.1374177643865,29.6701977328284,122.60266731771)) ;
#90205=CARTESIAN_POINT('Ctrl Pts',(-18.2961113277449,29.6801344639905,122.395320977446)) ;
#90206=CARTESIAN_POINT('Ctrl Pts',(-18.4891133100422,29.6901176748505,122.217574840443)) ;
#90207=CARTESIAN_POINT('Ctrl Pts',(-18.7115763555757,29.7001607740004,122.075621485712)) ;
#90208=CARTESIAN_POINT('Ctrl Pts',(-18.949992826985,29.7099917382753,121.976031903192)) ;
#90209=CARTESIAN_POINT('Ctrl Pts',(-19.2081671628499,29.7200645906612,121.917784053486)) ;
#90210=CARTESIAN_POINT('Ctrl Pts',(-19.467127300379,29.729928718373,121.905550210389)) ;
#90211=CARTESIAN_POINT('Ctrl Pts',(-19.7284409010787,29.7399509205079,121.938343116302)) ;
#90212=CARTESIAN_POINT('Ctrl Pts',(-19.9800566224885,29.7499781134763,122.016652854863)) ;
#90213=CARTESIAN_POINT('Ctrl Pts',(-20.210400702207,29.7598337074433,122.135017062282)) ;
#90214=CARTESIAN_POINT('Ctrl Pts',(-20.4193129127433,29.7697908793086,122.292588450327)) ;
#90215=CARTESIAN_POINT('Ctrl Pts',(-20.5988052662756,29.779829723307,122.485901523046)) ;
#90216=CARTESIAN_POINT('Ctrl Pts',(-20.740066998357,29.7897037471826,122.703600137925)) ;
#90217=CARTESIAN_POINT('Ctrl Pts',(-20.8433563231969,29.799773573173,122.947193893449)) ;
#90218=CARTESIAN_POINT('Ctrl Pts',(-20.9015323318944,29.8096068170702,123.198990450446)) ;
#90219=CARTESIAN_POINT('Ctrl Pts',(-20.9161199372986,29.8196372448433,123.462166811631)) ;
#90220=CARTESIAN_POINT('Ctrl Pts',(-20.8840222579638,29.8296688615884,123.723840344967)) ;
#90221=CARTESIAN_POINT('Ctrl Pts',(-20.8090522677205,29.8394985385691,123.971017934646)) ;
#90222=CARTESIAN_POINT('Ctrl Pts',(-20.6910925085159,29.8494880554091,124.205545773944)) ;
#90223=CARTESIAN_POINT('Ctrl Pts',(-20.5328239158274,29.8595316675488,124.416758785664)) ;
#90224=CARTESIAN_POINT('Ctrl Pts',(-20.3448871273158,29.8693542738841,124.593710045622)) ;
#90225=CARTESIAN_POINT('Ctrl Pts',(-20.1246838233644,29.8793925037834,124.738944315077)) ;
#90226=CARTESIAN_POINT('Ctrl Pts',(-19.8829956359094,29.8894035385753,124.842903601253)) ;
#90227=CARTESIAN_POINT('Ctrl Pts',(-19.629944134694,29.8993012695424,124.903033941421)) ;
#90228=CARTESIAN_POINT('Ctrl Pts',(-19.3679037961103,29.9092908973929,124.918797744218)) ;
#90229=CARTESIAN_POINT('Ctrl Pts',(-19.1080010949963,29.9192466878389,124.88883390131)) ;
#90230=CARTESIAN_POINT('Ctrl Pts',(-18.857809354991,29.929174086401,124.814884890953)) ;
#90231=CARTESIAN_POINT('Ctrl Pts',(-18.6219992187214,29.9391996815108,124.697407355649)) ;
#90232=CARTESIAN_POINT('Ctrl Pts',(-18.4130181328675,29.9490855321804,124.543075003642)) ;
#90233=CARTESIAN_POINT('Ctrl Pts',(-18.2316836984906,29.9590747120246,124.353257774373)) ;
#90234=CARTESIAN_POINT('Ctrl Pts',(-18.0857681933595,29.9691158991282,124.133401993258)) ;
#90235=CARTESIAN_POINT('Ctrl Pts',(-17.9820470555373,29.9789485426041,123.896746050801)) ;
#90236=CARTESIAN_POINT('Ctrl Pts',(-17.9192601596466,29.9889424923136,123.641732893525)) ;
#90237=CARTESIAN_POINT('Ctrl Pts',(-17.9021985043466,29.9989716150901,123.378728309774)) ;
#90238=CARTESIAN_POINT('Ctrl Pts',(-17.9302095800825,30.0088477460088,123.120696813041)) ;
#90239=CARTESIAN_POINT('Ctrl Pts',(-18.0031833304748,30.0188457810258,122.868329081507)) ;
#90240=CARTESIAN_POINT('Ctrl Pts',(-18.1177424147025,30.0287597107845,122.634304146691)) ;
#90241=CARTESIAN_POINT('Ctrl Pts',(-18.2731207173211,30.0388028985223,122.420990591887)) ;
#90242=CARTESIAN_POINT('Ctrl Pts',(-18.460477880612,30.0487027406627,122.240473905107)) ;
#90243=CARTESIAN_POINT('Ctrl Pts',(-18.6780038327348,30.0586940074707,122.093431755788)) ;
#90244=CARTESIAN_POINT('Ctrl Pts',(-18.9189236827015,30.0687261096027,121.986371546732)) ;
#90245=CARTESIAN_POINT('Ctrl Pts',(-19.170468246111,30.0785929905574,121.92348620404)) ;
#90246=CARTESIAN_POINT('Ctrl Pts',(-19.4323508510835,30.0885847818456,121.904376081853)) ;
#90247=CARTESIAN_POINT('Ctrl Pts',(-19.6945696776365,30.0986168977571,121.931642192667)) ;
#90248=CARTESIAN_POINT('Ctrl Pts',(-19.9440014901615,30.1084832145571,122.002451382793)) ;
#90249=CARTESIAN_POINT('Ctrl Pts',(-20.1803630188248,30.1184706960307,122.116477795654)) ;
#90250=CARTESIAN_POINT('Ctrl Pts',(-20.392566350984,30.1284156204096,122.269087188915)) ;
#90251=CARTESIAN_POINT('Ctrl Pts',(-20.5767324875527,30.1384605063203,122.458162856591)) ;
#90252=CARTESIAN_POINT('Ctrl Pts',(-20.7227801654869,30.1483226100329,122.67228121434)) ;
#90253=CARTESIAN_POINT('Ctrl Pts',(-20.8312983726913,30.1583141738574,122.911353552395)) ;
#90254=CARTESIAN_POINT('Ctrl Pts',(-20.8961724450446,30.1682469819203,123.164186294995)) ;
#90255=CARTESIAN_POINT('Ctrl Pts',(-20.916810994507,30.1781840841566,123.424522266059)) ;
#90256=CARTESIAN_POINT('Ctrl Pts',(-20.8912996042722,30.188236530427,123.687434835979)) ;
#90257=CARTESIAN_POINT('Ctrl Pts',(-20.8223241947769,30.1980826460086,123.936840767883)) ;
#90258=CARTESIAN_POINT('Ctrl Pts',(-20.7091987850365,30.2081306657235,124.17541152145)) ;
#90259=CARTESIAN_POINT('Ctrl Pts',(-20.5576650602483,30.2180726173524,124.388259700238)) ;
#90260=CARTESIAN_POINT('Ctrl Pts',(-20.3719976932811,30.2280113983515,124.57195695698)) ;
#90261=CARTESIAN_POINT('Ctrl Pts',(-20.1552718930415,30.2380374470776,124.721755575099)) ;
#90262=CARTESIAN_POINT('Ctrl Pts',(-19.9192454996909,30.2479243074858,124.830442864662)) ;
#90263=CARTESIAN_POINT('Ctrl Pts',(-19.6643659591417,30.2579555826176,124.897557475444)) ;
#90264=CARTESIAN_POINT('Ctrl Pts',(-19.4055132729224,30.267838559918,124.919346689653)) ;
#90265=CARTESIAN_POINT('Ctrl Pts',(-19.1423742851105,30.2778954133252,124.895462225033)) ;
#90266=CARTESIAN_POINT('Ctrl Pts',(-18.8081585492134,30.2910636544011,124.805348478367)) ;
#90267=CARTESIAN_POINT('Ctrl Pts',(-18.4999606060616,30.3044646836276,124.627109350704)) ;
#90268=CARTESIAN_POINT('Ctrl Pts',(-18.2548402508357,30.3176776003585,124.381034742561)) ;
#90269=CARTESIAN_POINT('Ctrl Pts',(-18.1049154570646,30.3276059948117,124.167570645998)) ;
#90270=CARTESIAN_POINT('Ctrl Pts',(-17.9935223888196,30.3375874949398,123.930052646589)) ;
#90271=CARTESIAN_POINT('Ctrl Pts',(-17.9250251231697,30.3476280382099,123.675258459608)) ;
#90272=CARTESIAN_POINT('Ctrl Pts',(-17.9019089621538,30.357477369993,123.417459308466)) ;
#90273=CARTESIAN_POINT('Ctrl Pts',(-17.9235593814897,30.3674727744647,123.155687344675)) ;
#90274=CARTESIAN_POINT('Ctrl Pts',(-17.9909293206155,30.3774891019133,122.901233828562)) ;
#90275=CARTESIAN_POINT('Ctrl Pts',(-18.1363619700471,30.3907127590798,122.585590307536)) ;
#90276=CARTESIAN_POINT('Ctrl Pts',(-18.3617445260575,30.4040070504692,122.313580619713)) ;
#90277=CARTESIAN_POINT('Ctrl Pts',(-18.6465310373536,30.4172914014007,122.111548083525)) ;
#90278=CARTESIAN_POINT('Ctrl Pts',(-18.8832363601411,30.4272637824625,121.999174549586)) ;
#90279=CARTESIAN_POINT('Ctrl Pts',(-19.1341844428468,30.4371721620881,121.929596295639)) ;
#90280=CARTESIAN_POINT('Ctrl Pts',(-19.3971607833827,30.4472261608362,121.904405542938)) ;
#90281=CARTESIAN_POINT('Ctrl Pts',(-19.6555624151399,30.4570883579525,121.924666180462)) ;
#90282=CARTESIAN_POINT('Ctrl Pts',(-19.9952854684949,30.4704354843266,122.01183022792)) ;
#90283=CARTESIAN_POINT('Ctrl Pts',(-20.3783427936636,30.486972449968,122.227450317524)) ;
#90284=CARTESIAN_POINT('Ctrl Pts',(-20.6669629084573,30.5036070541419,122.562246315872)) ;
#90285=CARTESIAN_POINT('Ctrl Pts',(-20.8186251415275,30.5168968473846,122.876913691283)) ;
#90286=CARTESIAN_POINT('Ctrl Pts',(-20.8898702450345,30.526849478644,123.128536989928)) ;
#90287=CARTESIAN_POINT('Ctrl Pts',(-20.9166526278365,30.5368014459487,123.388718812429)) ;
#90288=CARTESIAN_POINT('Ctrl Pts',(-20.8911983771875,30.5501687044125,123.739033428064)) ;
#90289=CARTESIAN_POINT('Ctrl Pts',(-20.7477475189037,30.5666855163617,124.154053346653)) ;
#90290=CARTESIAN_POINT('Ctrl Pts',(-20.4126988443248,30.586711411368,124.567435413989)) ;
#90291=CARTESIAN_POINT('Ctrl Pts',(-19.9614671654052,30.6065221414982,124.838987072851)) ;
#90292=CARTESIAN_POINT('Ctrl Pts',(-19.4406806653169,30.626499357628,124.942199667842)) ;
#90293=CARTESIAN_POINT('Ctrl Pts',(-18.9173904837054,30.6464262330233,124.86074682562)) ;
#90294=CARTESIAN_POINT('Ctrl Pts',(-18.4548551754709,30.6662476944996,124.608403042469)) ;
#90295=CARTESIAN_POINT('Ctrl Pts',(-18.1021138578036,30.6863220123089,124.208208372338)) ;
#90296=CARTESIAN_POINT('Ctrl Pts',(-17.9097086793361,30.7061699813168,123.716866447982)) ;
#90297=CARTESIAN_POINT('Ctrl Pts',(-17.8953715490996,30.72611701538,123.187016557676)) ;
#90298=CARTESIAN_POINT('Ctrl Pts',(-18.0624519723751,30.7460129663522,122.685261153681)) ;
#90299=CARTESIAN_POINT('Ctrl Pts',(-18.3899873246686,30.7659084459704,122.270164037835)) ;
#90300=CARTESIAN_POINT('Ctrl Pts',(-18.8408813750857,30.7858645569352,121.990764998331)) ;
#90301=CARTESIAN_POINT('Ctrl Pts',(-19.3586318139167,30.8057691049752,121.882458783378)) ;
#90302=CARTESIAN_POINT('Ctrl Pts',(-19.8818185744041,30.8256432292943,121.955925643777)) ;
#90303=CARTESIAN_POINT('Ctrl Pts',(-20.3522474723433,30.8456977592933,122.206355579186)) ;
#90304=CARTESIAN_POINT('Ctrl Pts',(-20.7048311303731,30.8655052730533,122.59744630561)) ;
#90305=CARTESIAN_POINT('Ctrl Pts',(-20.9055172328141,30.885488628821,123.089116826482)) ;
#90306=CARTESIAN_POINT('Ctrl Pts',(-20.9255113800788,30.905406931405,123.618128166974)) ;
#90307=CARTESIAN_POINT('Ctrl Pts',(-20.7655078140649,30.9252751468507,124.121480433858)) ;
#90308=CARTESIAN_POINT('Ctrl Pts',(-20.4398813109932,30.945325463647,124.543131309097)) ;
#90309=CARTESIAN_POINT('Ctrl Pts',(-19.9961416301673,30.9651015255295,124.825243045067)) ;
#90310=CARTESIAN_POINT('Ctrl Pts',(-19.4760428857146,30.9851561312219,124.940890724397)) ;
#90311=CARTESIAN_POINT('Ctrl Pts',(-18.9542245242808,31.0049498203778,124.872803577724)) ;
#90312=CARTESIAN_POINT('Ctrl Pts',(-18.4824553574321,31.0249165119722,124.630033633571)) ;
#90313=CARTESIAN_POINT('Ctrl Pts',(-18.1224338999949,31.0448765577232,124.240259071478)) ;
#90314=CARTESIAN_POINT('Ctrl Pts',(-17.9173964213131,31.0647748178734,123.752794316431)) ;
#90315=CARTESIAN_POINT('Ctrl Pts',(-17.8903757638579,31.0846697334226,123.22473469265)) ;
#90316=CARTESIAN_POINT('Ctrl Pts',(-18.0448284170245,31.1045799138362,122.718600932171)) ;
#90317=CARTESIAN_POINT('Ctrl Pts',(-18.3629565328079,31.1245157129505,122.29484956572)) ;
#90318=CARTESIAN_POINT('Ctrl Pts',(-18.8066023023989,31.1444535746046,122.005048043472)) ;
#90319=CARTESIAN_POINT('Ctrl Pts',(-19.3219837707938,31.1643726212422,121.883821949317)) ;
#90320=CARTESIAN_POINT('Ctrl Pts',(-19.8485586474663,31.1843215192964,121.945761987751)) ;
#90321=CARTESIAN_POINT('Ctrl Pts',(-20.3214530576657,31.2042273467395,122.183047702527)) ;
#90322=CARTESIAN_POINT('Ctrl Pts',(-20.62457405632,31.2208100421048,122.502904725448)) ;
#90323=CARTESIAN_POINT('Ctrl Pts',(-20.7912398187945,31.2340842558284,122.809407390215)) ;
#90324=CARTESIAN_POINT('Ctrl Pts',(-20.8750277230681,31.2441309750277,123.059747682737)) ;
#90325=CARTESIAN_POINT('Ctrl Pts',(-20.9135794146644,31.2539750096734,123.315566077138)) ;
#90326=CARTESIAN_POINT('Ctrl Pts',(-20.9056166911276,31.267309394578,123.665879105346)) ;
#90327=CARTESIAN_POINT('Ctrl Pts',(-20.7817240069621,31.2838966118777,124.089024590941)) ;
#90328=CARTESIAN_POINT('Ctrl Pts',(-20.5204927418564,31.3005298239156,124.44560763796)) ;
#90329=CARTESIAN_POINT('Ctrl Pts',(-20.2482842473179,31.3138122661878,124.664159228814)) ;
#90330=CARTESIAN_POINT('Ctrl Pts',(-20.0203552489676,31.323718154102,124.789870365395)) ;
#90331=CARTESIAN_POINT('Ctrl Pts',(-19.7720861356419,31.3337065722071,124.875118114952)) ;
#90332=CARTESIAN_POINT('Ctrl Pts',(-19.5118369240493,31.3437299994459,124.915827009597)) ;
#90333=CARTESIAN_POINT('Ctrl Pts',(-19.2516219194721,31.3536344305629,124.910938614496)) ;
#90334=CARTESIAN_POINT('Ctrl Pts',(-18.9093544512018,31.3668975831733,124.844874070695)) ;
#90335=CARTESIAN_POINT('Ctrl Pts',(-18.5909341743351,31.3802224810772,124.689988959161)) ;
#90336=CARTESIAN_POINT('Ctrl Pts',(-18.3276472878309,31.3934782246928,124.461818204276)) ;
#90337=CARTESIAN_POINT('Ctrl Pts',(-18.1623509832731,31.4034375981401,124.258944934311)) ;
#90338=CARTESIAN_POINT('Ctrl Pts',(-18.0346692467731,31.4133814220671,124.030912426066)) ;
#90339=CARTESIAN_POINT('Ctrl Pts',(-17.9478499345261,31.4234293662144,123.781565182109)) ;
#90340=CARTESIAN_POINT('Ctrl Pts',(-17.9062405916385,31.4332803374325,123.526042263013)) ;
#90341=CARTESIAN_POINT('Ctrl Pts',(-17.9089961332649,31.4432521548746,123.264037869211)) ;
#90342=CARTESIAN_POINT('Ctrl Pts',(-17.9573713255669,31.4532475771667,123.0058246328)) ;
#90343=CARTESIAN_POINT('Ctrl Pts',(-18.0504365475839,31.4632806422904,122.759146467247)) ;
#90344=CARTESIAN_POINT('Ctrl Pts',(-18.182455819894,31.4731459749556,122.53603494168)) ;
#90345=CARTESIAN_POINT('Ctrl Pts',(-18.3522600986835,31.4831065175532,122.336826203529)) ;
#90346=CARTESIAN_POINT('Ctrl Pts',(-18.555825302581,31.4931402030549,122.169258613365)) ;
#90347=CARTESIAN_POINT('Ctrl Pts',(-18.7818081775691,31.5030250350452,122.04108939127)) ;
#90348=CARTESIAN_POINT('Ctrl Pts',(-19.0310789742768,31.513092461805,121.952582039014)) ;
#90349=CARTESIAN_POINT('Ctrl Pts',(-19.2860425398375,31.5229309509638,121.909432534115)) ;
#90350=CARTESIAN_POINT('Ctrl Pts',(-19.5504588373335,31.532994432154,121.910897207184)) ;
#90351=CARTESIAN_POINT('Ctrl Pts',(-19.806252038689,31.5428885899691,121.957687925717)) ;
#90352=CARTESIAN_POINT('Ctrl Pts',(-20.0513987980626,31.5528304467134,122.047929059202)) ;
#90353=CARTESIAN_POINT('Ctrl Pts',(-20.2786389120805,31.5628329243848,122.180116472421)) ;
#90354=CARTESIAN_POINT('Ctrl Pts',(-20.4798154738035,31.5728677286891,122.350583181619)) ;
#90355=CARTESIAN_POINT('Ctrl Pts',(-20.6455040679005,31.5827126055348,122.549301249805)) ;
#90356=CARTESIAN_POINT('Ctrl Pts',(-20.7764127766709,31.5926984850903,122.776686313643)) ;
#90357=CARTESIAN_POINT('Ctrl Pts',(-20.8656033287989,31.6026332154488,123.022106958682)) ;
#90358=CARTESIAN_POINT('Ctrl Pts',(-20.9111243111444,31.6126910277617,123.282421856098)) ;
#90359=CARTESIAN_POINT('Ctrl Pts',(-20.9112068367647,31.6225116198861,123.540539997943)) ;
#90360=CARTESIAN_POINT('Ctrl Pts',(-20.865687331279,31.6325782054958,123.801079440899)) ;
#90361=CARTESIAN_POINT('Ctrl Pts',(-20.7770317266897,31.6424777860777,124.045722854565)) ;
#90362=CARTESIAN_POINT('Ctrl Pts',(-20.6453936142839,31.6525293857559,124.274672946805)) ;
#90363=CARTESIAN_POINT('Ctrl Pts',(-20.4790792984421,31.6624035721729,124.473913961419)) ;
#90364=CARTESIAN_POINT('Ctrl Pts',(-20.2772197656373,31.6724600480538,124.644405849723)) ;
#90365=CARTESIAN_POINT('Ctrl Pts',(-20.0524976022664,31.6823529793564,124.775234014397)) ;
#90366=CARTESIAN_POINT('Ctrl Pts',(-19.8043940631741,31.692415758069,124.866611670972)) ;
#90367=CARTESIAN_POINT('Ctrl Pts',(-19.5498389701363,31.7022582836502,124.912638260607)) ;
#90368=CARTESIAN_POINT('Ctrl Pts',(-19.287331714963,31.7122490490751,124.914410642322)) ;
#90369=CARTESIAN_POINT('Ctrl Pts',(-19.0300907670381,31.7221771250731,124.870797527224)) ;
#90370=CARTESIAN_POINT('Ctrl Pts',(-18.7826960536114,31.7321650354601,124.783086226261)) ;
#90371=CARTESIAN_POINT('Ctrl Pts',(-18.5534309522588,31.7422009475851,124.652751134591)) ;
#90372=CARTESIAN_POINT('Ctrl Pts',(-18.353644514985,31.7520559604328,124.487929296874)) ;
#90373=CARTESIAN_POINT('Ctrl Pts',(-18.1828179715406,31.762054906349,124.288330075696)) ;
#90374=CARTESIAN_POINT('Ctrl Pts',(-18.0503460097519,31.771951818797,124.064468215422)) ;
#90375=CARTESIAN_POINT('Ctrl Pts',(-17.9573008027146,31.7820056168905,123.817225770989)) ;
#90376=CARTESIAN_POINT('Ctrl Pts',(-17.9093501306192,31.7918865377172,123.562001493347)) ;
#90377=CARTESIAN_POINT('Ctrl Pts',(-17.9059334517401,31.8018910637149,123.299145753374)) ;
#90378=CARTESIAN_POINT('Ctrl Pts',(-17.9482120491376,31.8118750273324,123.040161685246)) ;
#90379=CARTESIAN_POINT('Ctrl Pts',(-18.0355138245975,31.8219146678837,122.791213968382)) ;
#90380=CARTESIAN_POINT('Ctrl Pts',(-18.1619308507885,31.8317586934984,122.565514127231)) ;
#90381=CARTESIAN_POINT('Ctrl Pts',(-18.3274742184349,31.8417496993158,122.361724868883)) ;
#90382=CARTESIAN_POINT('Ctrl Pts',(-18.5272092718872,31.8517874908479,122.189426042634)) ;
#90383=CARTESIAN_POINT('Ctrl Pts',(-18.7492365418585,31.8616318906363,122.05662983357)) ;
#90384=CARTESIAN_POINT('Ctrl Pts',(-18.9941697641335,31.8716166911931,121.962618647792)) ;
#90385=CARTESIAN_POINT('Ctrl Pts',(-19.2505857843533,31.8815562146042,121.912666206365)) ;
#90386=CARTESIAN_POINT('Ctrl Pts',(-19.5143572467387,31.8915959337052,121.908010594915)) ;
#90387=CARTESIAN_POINT('Ctrl Pts',(-19.771053035124,31.9014841056245,121.94848018403)) ;
#90388=CARTESIAN_POINT('Ctrl Pts',(-20.0194783206586,31.9114736680415,122.033298650539)) ;
#90389=CARTESIAN_POINT('Ctrl Pts',(-20.2485944427228,31.9214320402362,122.159742447755)) ;
#90390=CARTESIAN_POINT('Ctrl Pts',(-20.4514867933735,31.9313321144669,122.322607169725)) ;
#90391=CARTESIAN_POINT('Ctrl Pts',(-20.6255075792033,31.9413782108405,122.521118480551)) ;
#90392=CARTESIAN_POINT('Ctrl Pts',(-20.7605689119132,31.9512867948376,122.743753647204)) ;
#90393=CARTESIAN_POINT('Ctrl Pts',(-20.8563432165643,31.9612973734285,122.988771599216)) ;
#90394=CARTESIAN_POINT('Ctrl Pts',(-20.9076937965973,31.9713265315413,123.247285998441)) ;
#90395=CARTESIAN_POINT('Ctrl Pts',(-20.9136494977614,31.9811794133794,123.506125048581)) ;
#90396=CARTESIAN_POINT('Ctrl Pts',(-20.8749431252904,31.9911389745304,123.764982177503)) ;
#90397=CARTESIAN_POINT('Ctrl Pts',(-20.7907719543159,32.0011774091195,124.014974716044)) ;
#90398=CARTESIAN_POINT('Ctrl Pts',(-20.66695264249,32.0110506813466,124.243030789615)) ;
#90399=CARTESIAN_POINT('Ctrl Pts',(-20.5021399302121,32.0211239233402,124.450109642599)) ;
#90400=CARTESIAN_POINT('Ctrl Pts',(-20.3089945095504,32.0309442548732,124.621352168166)) ;
#90401=CARTESIAN_POINT('Ctrl Pts',(-20.0834973590324,32.0410229161,124.760153885266)) ;
#90402=CARTESIAN_POINT('Ctrl Pts',(-19.8427881240408,32.0508745113942,124.855626446842)) ;
#90403=CARTESIAN_POINT('Ctrl Pts',(-19.5836101770202,32.060947646623,124.909232373603)) ;
#90404=CARTESIAN_POINT('Ctrl Pts',(-19.3250477235278,32.0707900821481,124.91680672433)) ;
#90405=CARTESIAN_POINT('Ctrl Pts',(-19.0654135129984,32.0807708512815,124.879716005305)) ;
#90406=CARTESIAN_POINT('Ctrl Pts',(-18.8153951069858,32.0907879525253,124.797342091289)) ;
#90407=CARTESIAN_POINT('Ctrl Pts',(-18.5862068913827,32.1006764001272,124.674829079308)) ;
#90408=CARTESIAN_POINT('Ctrl Pts',(-18.3783323865825,32.110732114308,124.511717380021)) ;
#90409=CARTESIAN_POINT('Ctrl Pts',(-18.20504643639,32.1206073207219,124.318515886017)) ;
#90410=CARTESIAN_POINT('Ctrl Pts',(-18.0657523054065,32.1306023731946,124.095843008576)) ;
#90411=CARTESIAN_POINT('Ctrl Pts',(-17.9673624393521,32.1406242571567,123.851536926118)) ;
#90412=CARTESIAN_POINT('Ctrl Pts',(-17.9132447511668,32.150528229686,123.596960929366)) ;
#90413=CARTESIAN_POINT('Ctrl Pts',(-17.9036966014167,32.1605167263469,123.334645288358)) ;
#90414=CARTESIAN_POINT('Ctrl Pts',(-17.939924691972,32.1704805235949,123.07533896734)) ;
#90415=CARTESIAN_POINT('Ctrl Pts',(-18.0195480393415,32.1803845469029,122.827524176256)) ;
#90416=CARTESIAN_POINT('Ctrl Pts',(-18.1430776002173,32.1904450502245,122.593816083373)) ;
#90417=CARTESIAN_POINT('Ctrl Pts',(-18.3015440658301,32.2002855853644,122.389414603507)) ;
#90418=CARTESIAN_POINT('Ctrl Pts',(-18.4971343102704,32.210347806069,122.211511240556)) ;
#90419=CARTESIAN_POINT('Ctrl Pts',(-18.7171578358292,32.2202449598452,122.072795116102)) ;
#90420=CARTESIAN_POINT('Ctrl Pts',(-18.9584036223106,32.2301760932307,121.973254778566)) ;
#90421=CARTESIAN_POINT('Ctrl Pts',(-19.2161862551315,32.2402184683764,121.916771627792)) ;
#90422=CARTESIAN_POINT('Ctrl Pts',(-19.4757653790532,32.2501044061426,121.905874060276)) ;
#90423=CARTESIAN_POINT('Ctrl Pts',(-19.7361743618916,32.2601002491274,121.940186996512)) ;
#90424=CARTESIAN_POINT('Ctrl Pts',(-19.9853445011283,32.270042227006,122.01880797192)) ;
#90425=CARTESIAN_POINT('Ctrl Pts',(-20.2176224237473,32.280001601487,122.139380240724)) ;
#90426=CARTESIAN_POINT('Ctrl Pts',(-20.4263292540062,32.2899982173208,122.298965348353)) ;
#90427=CARTESIAN_POINT('Ctrl Pts',(-20.6045437074103,32.3000324358943,122.49330330733)) ;
#90428=CARTESIAN_POINT('Ctrl Pts',(-20.7440160089712,32.3098855031049,122.711454247693)) ;
#90429=CARTESIAN_POINT('Ctrl Pts',(-20.8452761241106,32.3198457609825,122.952809541801)) ;
#90430=CARTESIAN_POINT('Ctrl Pts',(-20.9031915155856,32.3298747876881,123.209934123648)) ;
#90431=CARTESIAN_POINT('Ctrl Pts',(-20.9155108381836,32.3397849947225,123.470061362045)) ;
#90432=CARTESIAN_POINT('Ctrl Pts',(-20.8830729146311,32.3497199053701,123.729125220497)) ;
#90433=CARTESIAN_POINT('Ctrl Pts',(-20.8050925575432,32.3597610355494,123.98120077394)) ;
#90434=CARTESIAN_POINT('Ctrl Pts',(-20.6865290803088,32.3696481759193,124.212412477173)) ;
#90435=CARTESIAN_POINT('Ctrl Pts',(-20.5283214706852,32.3796404534553,124.421965720278)) ;
#90436=CARTESIAN_POINT('Ctrl Pts',(-20.3368987653535,32.3895889967236,124.600050795474)) ;
#90437=CARTESIAN_POINT('Ctrl Pts',(-20.1179553075885,32.3995256715408,124.742318590014)) ;
#90438=CARTESIAN_POINT('Ctrl Pts',(-19.8765857645309,32.4095090924772,124.845198491733)) ;
#90439=CARTESIAN_POINT('Ctrl Pts',(-19.6194540624684,32.4195514076664,124.904530262006)) ;
#90440=CARTESIAN_POINT('Ctrl Pts',(-19.3612323588906,32.4293917251056,124.918456384701)) ;
#90441=CARTESIAN_POINT('Ctrl Pts',(-19.0995012622624,32.4394214291631,124.887349726659)) ;
#90442=CARTESIAN_POINT('Ctrl Pts',(-18.8475761386304,32.4494423858856,124.81065894568)) ;
#90443=CARTESIAN_POINT('Ctrl Pts',(-18.6160938856141,32.4593089281892,124.693811732837)) ;
#90444=CARTESIAN_POINT('Ctrl Pts',(-18.4041445829569,32.4693800281344,124.535355939284)) ;
#90445=CARTESIAN_POINT('Ctrl Pts',(-18.2270297897121,32.4792221023119,124.346861724585)) ;
#90446=CARTESIAN_POINT('Ctrl Pts',(-18.0828270949522,32.489182896899,124.128411540511)) ;
#90447=CARTESIAN_POINT('Ctrl Pts',(-17.978420138532,32.4992207697998,123.88617867698)) ;
#90448=CARTESIAN_POINT('Ctrl Pts',(-17.918171831887,32.5090950553439,123.633750736518)) ;
#90449=CARTESIAN_POINT('Ctrl Pts',(-17.9023810135821,32.5191648057578,123.369635645094)) ;
#90450=CARTESIAN_POINT('Ctrl Pts',(-17.9318454096663,32.5289980902925,123.112890613939)) ;
#90451=CARTESIAN_POINT('Ctrl Pts',(-18.0061909068655,32.5390284310925,122.860013828916)) ;
#90452=CARTESIAN_POINT('Ctrl Pts',(-18.1240350153628,32.5490603550921,122.624176778822)) ;
#90453=CARTESIAN_POINT('Ctrl Pts',(-18.2773901023668,32.558888890028,122.416362824848)) ;
#90454=CARTESIAN_POINT('Ctrl Pts',(-18.4671549519202,32.5688826677927,122.234811814169)) ;
#90455=CARTESIAN_POINT('Ctrl Pts',(-18.6865982599419,32.5789103782782,122.088899208413)) ;
#90456=CARTESIAN_POINT('Ctrl Pts',(-18.9245545564035,32.5887987891122,121.984478210373)) ;
#90457=CARTESIAN_POINT('Ctrl Pts',(-19.179155033595,32.5987756396477,121.921970498854)) ;
#90458=CARTESIAN_POINT('Ctrl Pts',(-19.4411893341139,32.6087674361982,121.904567510373)) ;
#90459=CARTESIAN_POINT('Ctrl Pts',(-19.703326580114,32.6188034422919,121.933365758691)) ;
#90460=CARTESIAN_POINT('Ctrl Pts',(-19.9519587960283,32.6286541765547,122.005505794216)) ;
#90461=CARTESIAN_POINT('Ctrl Pts',(-20.1877508005523,32.6386454350829,122.120918680607)) ;
#90462=CARTESIAN_POINT('Ctrl Pts',(-20.3985123625034,32.6485633299861,122.274300781478)) ;
#90463=CARTESIAN_POINT('Ctrl Pts',(-20.5814614274393,32.6585914716491,122.463947516891)) ;
#90464=CARTESIAN_POINT('Ctrl Pts',(-20.7267096138185,32.668476639765,122.679326125919)) ;
#90465=CARTESIAN_POINT('Ctrl Pts',(-20.8340502982722,32.678466003271,122.918892802554)) ;
#90466=CARTESIAN_POINT('Ctrl Pts',(-20.8979545030379,32.6885071382811,123.174908117759)) ;
#90467=CARTESIAN_POINT('Ctrl Pts',(-20.9164761609195,32.6983398064691,123.432631238316)) ;
#90468=CARTESIAN_POINT('Ctrl Pts',(-20.8902807920564,32.7083337094236,123.693949516132)) ;
#90469=CARTESIAN_POINT('Ctrl Pts',(-20.8183191956796,32.7183629945081,123.947496333409)) ;
#90470=CARTESIAN_POINT('Ctrl Pts',(-20.7055639452945,32.72823852295,124.181255541168)) ;
#90471=CARTESIAN_POINT('Ctrl Pts',(-20.5522820009705,32.7382388055661,124.394679958423)) ;
#90472=CARTESIAN_POINT('Ctrl Pts',(-20.366031988061,32.7481508216231,124.57682210646)) ;
#90473=CARTESIAN_POINT('Ctrl Pts',(-20.1482437968875,32.7581928969621,124.725815001188)) ;
#90474=CARTESIAN_POINT('Ctrl Pts',(-19.9112655719754,32.7680927296182,124.8331936985)) ;
#90475=CARTESIAN_POINT('Ctrl Pts',(-19.65704415951,32.7780851301962,124.898959513189)) ;
#90476=CARTESIAN_POINT('Ctrl Pts',(-19.3941345542646,32.7881191519556,124.919203661167)) ;
#90477=CARTESIAN_POINT('Ctrl Pts',(-19.1361107148346,32.7979837627968,124.894256925511)) ;
#90478=CARTESIAN_POINT('Ctrl Pts',(-18.8829224544705,32.807976162258,124.824605397838)) ;
#90479=CARTESIAN_POINT('Ctrl Pts',(-18.6449612635533,32.8180081155909,124.711138853319)) ;
#90480=CARTESIAN_POINT('Ctrl Pts',(-18.4336192368535,32.8278744745325,124.560921747617)) ;
#90481=CARTESIAN_POINT('Ctrl Pts',(-18.2490612673754,32.8378619500183,124.374355254994)) ;
#90482=CARTESIAN_POINT('Ctrl Pts',(-18.1001820205622,32.8478068562068,124.159518606616)) ;
#90483=CARTESIAN_POINT('Ctrl Pts',(-17.9899307415803,32.857851820867,123.919702152225)) ;
#90484=CARTESIAN_POINT('Ctrl Pts',(-17.9239755325999,32.8677136277719,123.669054864759)) ;
#90485=CARTESIAN_POINT('Ctrl Pts',(-17.9017602263012,32.8777063000777,123.407426433999)) ;
#90486=CARTESIAN_POINT('Ctrl Pts',(-17.9251935246742,32.887634971023,123.147548631717)) ;
#90487=CARTESIAN_POINT('Ctrl Pts',(-17.9931352135227,32.8975875132483,122.895003816011)) ;
#90488=CARTESIAN_POINT('Ctrl Pts',(-18.1043312287972,32.9075888692442,122.656829799846)) ;
#90489=CARTESIAN_POINT('Ctrl Pts',(-18.2558767004374,32.9176174815189,122.441233493131)) ;
#90490=CARTESIAN_POINT('Ctrl Pts',(-18.4392492938704,32.9274818160684,122.257982555295)) ;
#90491=CARTESIAN_POINT('Ctrl Pts',(-18.6541333399341,32.937474140145,122.107122522269)) ;
#90492=CARTESIAN_POINT('Ctrl Pts',(-18.8904036310431,32.9474016325109,121.996414241407)) ;
#90493=CARTESIAN_POINT('Ctrl Pts',(-19.144776160248,32.9574289910617,121.927756331862)) ;
#90494=CARTESIAN_POINT('Ctrl Pts',(-19.4035634233285,32.9673154091128,121.904356292453)) ;
#90495=CARTESIAN_POINT('Ctrl Pts',(-19.6662173972518,32.9773471438482,121.926427682475)) ;
#90496=CARTESIAN_POINT('Ctrl Pts',(-19.9173873207107,32.9872287250915,121.992537401162)) ;
#90497=CARTESIAN_POINT('Ctrl Pts',(-20.1575155915266,32.9972907031238,122.103143972169)) ;
#90498=CARTESIAN_POINT('Ctrl Pts',(-20.370483550717,33.0071477814855,122.250663584042)) ;
#90499=CARTESIAN_POINT('Ctrl Pts',(-20.5574852732715,33.0171423545915,122.435031329392)) ;
#90500=CARTESIAN_POINT('Ctrl Pts',(-20.7087098909113,33.0270681508791,122.647604267584)) ;
#90501=CARTESIAN_POINT('Ctrl Pts',(-20.8218893770371,33.0370935180488,122.885487342572)) ;
#90502=CARTESIAN_POINT('Ctrl Pts',(-20.8912556584646,33.0469895977027,123.136134795138)) ;
#90503=CARTESIAN_POINT('Ctrl Pts',(-20.9168234356785,33.0569846774083,123.397550614612)) ;
#90504=CARTESIAN_POINT('Ctrl Pts',(-20.8961029605947,33.0670097652241,123.660183142044)) ;
#90505=CARTESIAN_POINT('Ctrl Pts',(-20.8098991145045,33.0801935875914,123.99574300305)) ;
#90506=CARTESIAN_POINT('Ctrl Pts',(-20.6369446858756,33.0935157057373,124.304678709047)) ;
#90507=CARTESIAN_POINT('Ctrl Pts',(-20.3908204960889,33.1068949153649,124.555834602614)) ;
#90508=CARTESIAN_POINT('Ctrl Pts',(-20.1809494793358,33.1167331526091,124.706837071298)) ;
#90509=CARTESIAN_POINT('Ctrl Pts',(-19.942577781835,33.1268060758678,124.821869252031)) ;
#90510=CARTESIAN_POINT('Ctrl Pts',(-19.693263181732,33.1366627173229,124.892205355517)) ;
#90511=CARTESIAN_POINT('Ctrl Pts',(-19.4322613230798,33.146648092829,124.919218109963)) ;
#90512=CARTESIAN_POINT('Ctrl Pts',(-19.0841401970618,33.1599321242894,124.89401589364)) ;
#90513=CARTESIAN_POINT('Ctrl Pts',(-18.6686887473864,33.1764509161598,124.751538820693)) ;
#90514=CARTESIAN_POINT('Ctrl Pts',(-18.322123263724,33.1932366331664,124.470796884464)) ;
#90515=CARTESIAN_POINT('Ctrl Pts',(-18.1195228019478,33.2063497816754,124.191941939277)) ;
#90516=CARTESIAN_POINT('Ctrl Pts',(-18.0029823657326,33.2163853307556,123.955407109914)) ;
#90517=CARTESIAN_POINT('Ctrl Pts',(-17.9301367991554,33.226401386935,123.70244375215)) ;
#90518=CARTESIAN_POINT('Ctrl Pts',(-17.8928038233433,33.239579422801,123.358205398184)) ;
#90519=CARTESIAN_POINT('Ctrl Pts',(-17.9589484139631,33.2561812999881,122.921862723111)) ;
#90520=CARTESIAN_POINT('Ctrl Pts',(-18.2153509315473,33.276244444604,122.454328572859)) ;
#90521=CARTESIAN_POINT('Ctrl Pts',(-18.610517617413,33.2960453346877,122.106659477122)) ;
#90522=CARTESIAN_POINT('Ctrl Pts',(-19.1034981315604,33.3159884599664,121.912149478104)) ;
#90523=CARTESIAN_POINT('Ctrl Pts',(-19.6321521720369,33.335886505086,121.897927841427)) ;
#90524=CARTESIAN_POINT('Ctrl Pts',(-20.1341123261989,33.3557722647127,122.063632571961)) ;
#90525=CARTESIAN_POINT('Ctrl Pts',(-20.5525339489159,33.3758374398926,122.394216721666)) ;
#90526=CARTESIAN_POINT('Ctrl Pts',(-20.8296056794486,33.3956640829954,122.842560084467)) ;
#90527=CARTESIAN_POINT('Ctrl Pts',(-20.9388743874097,33.4155727924438,123.360152546638)) ;
#90528=CARTESIAN_POINT('Ctrl Pts',(-20.8648847574417,33.4355246294756,123.885402002908)) ;
#90529=CARTESIAN_POINT('Ctrl Pts',(-20.6147318866576,33.4555331041787,124.35462141048)) ;
#90530=CARTESIAN_POINT('Ctrl Pts',(-20.2239322170856,33.4753345629402,124.707141469447)) ;
#90531=CARTESIAN_POINT('Ctrl Pts',(-19.7330000970732,33.4952914511762,124.907967316448)) ;
#90532=CARTESIAN_POINT('Ctrl Pts',(-19.2022616264228,33.5152752885903,124.92803419319)) ;
#90533=CARTESIAN_POINT('Ctrl Pts',(-18.7005637331334,33.5350837278112,124.768198422526)) ;
#90534=CARTESIAN_POINT('Ctrl Pts',(-18.2796383911774,33.5550694371914,124.44444941678)) ;
#90535=CARTESIAN_POINT('Ctrl Pts',(-17.9957682334727,33.5749389602067,123.998878153294)) ;
#90536=CARTESIAN_POINT('Ctrl Pts',(-17.8804168309484,33.5949596993239,123.479617978128)) ;
#90537=CARTESIAN_POINT('Ctrl Pts',(-17.9478193704265,33.6147637643009,122.957391827928)) ;
#90538=CARTESIAN_POINT('Ctrl Pts',(-18.1922075876265,33.6348257280316,122.483648094758)) ;
#90539=CARTESIAN_POINT('Ctrl Pts',(-18.5796761414085,33.6546589083201,122.126063706925)) ;
#90540=CARTESIAN_POINT('Ctrl Pts',(-19.0672471785734,33.6745781056462,121.919993572332)) ;
#90541=CARTESIAN_POINT('Ctrl Pts',(-19.5964794361335,33.6945161307595,121.892984850209)) ;
#90542=CARTESIAN_POINT('Ctrl Pts',(-20.1019033803434,33.7143941768156,122.047027331049)) ;
#90543=CARTESIAN_POINT('Ctrl Pts',(-20.5266212368,33.7343789111036,122.365892503823)) ;
#90544=CARTESIAN_POINT('Ctrl Pts',(-20.8161596894946,33.7542897277821,122.809038474966)) ;
#90545=CARTESIAN_POINT('Ctrl Pts',(-20.9372320691971,33.7742887033008,123.326476372936)) ;
#90546=CARTESIAN_POINT('Ctrl Pts',(-20.8757063920879,33.794093623946,123.849357303765)) ;
#90547=CARTESIAN_POINT('Ctrl Pts',(-20.6381117871144,33.8140775842373,124.324253054695)) ;
#90548=CARTESIAN_POINT('Ctrl Pts',(-20.2542831223755,33.8339637879612,124.68776744017)) ;
#90549=CARTESIAN_POINT('Ctrl Pts',(-19.7682875774795,33.8539129662844,124.899638859617)) ;
#90550=CARTESIAN_POINT('Ctrl Pts',(-19.2403826918121,33.8738147655239,124.932749323291)) ;
#90551=CARTESIAN_POINT('Ctrl Pts',(-18.7331049966278,33.8936933705763,124.784958195481)) ;
#90552=CARTESIAN_POINT('Ctrl Pts',(-18.3035554846274,33.913725730302,124.470321163056)) ;
#90553=CARTESIAN_POINT('Ctrl Pts',(-18.0587986989934,33.9303074562581,124.103799046386)) ;
#90554=CARTESIAN_POINT('Ctrl Pts',(-17.9464440989299,33.943501626556,123.775801865132)) ;
#90555=CARTESIAN_POINT('Ctrl Pts',(-17.891701854277,33.9568138046492,123.430280794334)) ;
#90556=CARTESIAN_POINT('Ctrl Pts',(-17.937495113229,33.9733799842425,122.992341681738)) ;
#90557=CARTESIAN_POINT('Ctrl Pts',(-18.1302774467429,33.9900081791027,122.594720028889)) ;
#90558=CARTESIAN_POINT('Ctrl Pts',(-18.3588197435753,34.0032967608125,122.330608010279)) ;
#90559=CARTESIAN_POINT('Ctrl Pts',(-18.5618595656554,34.0132650089161,122.165129183368)) ;
#90560=CARTESIAN_POINT('Ctrl Pts',(-18.7891847096601,34.0231797651722,122.037806845521)) ;
#90561=CARTESIAN_POINT('Ctrl Pts',(-19.0375192291355,34.0331929158234,121.950759748817)) ;
#90562=CARTESIAN_POINT('Ctrl Pts',(-19.2972286630396,34.0432056230254,121.908570343025)) ;
#90563=CARTESIAN_POINT('Ctrl Pts',(-19.6446460039,34.0564249117167,121.912596021897)) ;
#90564=CARTESIAN_POINT('Ctrl Pts',(-20.0699254705713,34.0730435927147,122.03142792988)) ;
#90565=CARTESIAN_POINT('Ctrl Pts',(-20.4284671618756,34.0896085004882,122.287092857787)) ;
#90566=CARTESIAN_POINT('Ctrl Pts',(-20.6522378081821,34.103006972099,122.558923682417)) ;
#90567=CARTESIAN_POINT('Ctrl Pts',(-20.779673548747,34.112848227586,122.78398886291)) ;
#90568=CARTESIAN_POINT('Ctrl Pts',(-20.8678897526762,34.1228345431742,123.031102300472)) ;
#90569=CARTESIAN_POINT('Ctrl Pts',(-20.9117788511624,34.1327711507606,123.288555336312)) ;
#90570=CARTESIAN_POINT('Ctrl Pts',(-20.9101514532125,34.1428210181289,123.552623293535)) ;
#90571=CARTESIAN_POINT('Ctrl Pts',(-20.863821952132,34.1526715128037,123.807324091934)) ;
#90572=CARTESIAN_POINT('Ctrl Pts',(-20.7735256213535,34.1626433131982,124.053287870522)) ;
#90573=CARTESIAN_POINT('Ctrl Pts',(-20.6415098394546,34.172639280224,124.280439245738)) ;
#90574=CARTESIAN_POINT('Ctrl Pts',(-20.4711254085416,34.1826767396052,124.481765931649)) ;
#90575=CARTESIAN_POINT('Ctrl Pts',(-20.2726263760509,34.1925174405059,124.647547741897)) ;
#90576=CARTESIAN_POINT('Ctrl Pts',(-20.0438538007464,34.2025654617733,124.779381747442)) ;
#90577=CARTESIAN_POINT('Ctrl Pts',(-19.7979948387222,34.212512854856,124.868199817644)) ;
#90578=CARTESIAN_POINT('Ctrl Pts',(-19.5415398597008,34.2224230009024,124.913598266864)) ;
#90579=CARTESIAN_POINT('Ctrl Pts',(-19.2772295562355,34.232481914752,124.913481740672)) ;
#90580=CARTESIAN_POINT('Ctrl Pts',(-19.0224749494035,34.2423226850413,124.868818922004)) ;
#90581=CARTESIAN_POINT('Ctrl Pts',(-18.7738170634932,34.2523855546199,124.778924498811)) ;
#90582=CARTESIAN_POINT('Ctrl Pts',(-18.5484380725391,34.2622798777504,124.649212333765)) ;
#90583=CARTESIAN_POINT('Ctrl Pts',(-18.3476405758638,34.2722216848449,124.482118201079)) ;
#90584=CARTESIAN_POINT('Ctrl Pts',(-18.1777564580938,34.2822241958002,124.281491322928)) ;
#90585=CARTESIAN_POINT('Ctrl Pts',(-18.0452449011872,34.2922589166186,124.053519923631)) ;
#90586=CARTESIAN_POINT('Ctrl Pts',(-17.9556349074693,34.3021040941243,123.810796881849)) ;
#90587=CARTESIAN_POINT('Ctrl Pts',(-17.9083784162444,34.3120888545254,123.552736052031)) ;
#90588=CARTESIAN_POINT('Ctrl Pts',(-17.9065296697451,34.3220277608418,123.291519123483)) ;
#90589=CARTESIAN_POINT('Ctrl Pts',(-17.9505964036269,34.3320699884775,123.031352463089)) ;
#90590=CARTESIAN_POINT('Ctrl Pts',(-18.037624931531,34.3419552000619,122.786560063066)) ;
#90591=CARTESIAN_POINT('Ctrl Pts',(-18.1669823934787,34.3519541302638,122.557890019545)) ;
#90592=CARTESIAN_POINT('Ctrl Pts',(-18.3326161325234,34.3618715531743,122.356617211244)) ;
#90593=CARTESIAN_POINT('Ctrl Pts',(-18.5332582552476,34.371919485253,122.185024436481)) ;
#90594=CARTESIAN_POINT('Ctrl Pts',(-18.7567288565943,34.3817968610624,122.052891702144)) ;
#90595=CARTESIAN_POINT('Ctrl Pts',(-19.0039582074564,34.3918507542303,121.959841830907)) ;
#90596=CARTESIAN_POINT('Ctrl Pts',(-19.2595239194454,34.4017443774836,121.911772148145)) ;
#90597=CARTESIAN_POINT('Ctrl Pts',(-19.5238983005659,34.4118069711066,121.908716657906)) ;
#90598=CARTESIAN_POINT('Ctrl Pts',(-19.7791766052678,34.4216495450957,121.950552116811)) ;
#90599=CARTESIAN_POINT('Ctrl Pts',(-20.0271336820024,34.4316403019786,122.036751836133)) ;
#90600=CARTESIAN_POINT('Ctrl Pts',(-20.254936747224,34.4415683637365,122.163955290834)) ;
#90601=CARTESIAN_POINT('Ctrl Pts',(-20.4586999823896,34.4515563396257,122.329419432095)) ;
#90602=CARTESIAN_POINT('Ctrl Pts',(-20.6311135230344,34.4615920039821,122.528971921844)) ;
#90603=CARTESIAN_POINT('Ctrl Pts',(-20.7641991432005,34.4714479424018,122.751184316972)) ;
#90604=CARTESIAN_POINT('Ctrl Pts',(-20.8583766148853,34.4814434337987,122.996362053338)) ;
#90605=CARTESIAN_POINT('Ctrl Pts',(-20.9082075537525,34.4913532387521,123.251982490847)) ;
#90606=CARTESIAN_POINT('Ctrl Pts',(-20.9133731041675,34.5013654610189,123.515048494353)) ;
#90607=CARTESIAN_POINT('Ctrl Pts',(-20.8722117287927,34.5113933417117,123.775338285339)) ;
#90608=CARTESIAN_POINT('Ctrl Pts',(-20.7883656546394,34.5212497376943,124.020406248148)) ;
#90609=CARTESIAN_POINT('Ctrl Pts',(-20.6615835386418,34.5312745348743,124.251337874107)) ;
#90610=CARTESIAN_POINT('Ctrl Pts',(-20.4960213753757,34.5413054648581,124.456471359235)) ;
#90611=CARTESIAN_POINT('Ctrl Pts',(-20.3013678063014,34.5511500673668,124.626861391942)) ;
#90612=CARTESIAN_POINT('Ctrl Pts',(-20.0771540029309,34.5611409185909,124.763475181664)) ;
#90613=CARTESIAN_POINT('Ctrl Pts',(-19.8312684979688,34.5711787516021,124.858978848205)) ;
#90614=CARTESIAN_POINT('Ctrl Pts',(-19.577597721108,34.5810231400675,124.909794407279)) ;
#90615=CARTESIAN_POINT('Ctrl Pts',(-19.3153254135936,34.5910079444371,124.916395570921)) ;
#90616=CARTESIAN_POINT('Ctrl Pts',(-19.0569804860377,34.6009474639199,124.87763585839)) ;
#90617=CARTESIAN_POINT('Ctrl Pts',(-18.806866607614,34.6109871949213,124.793729916711)) ;
#90618=CARTESIAN_POINT('Ctrl Pts',(-18.5785256075441,34.6208753231676,124.669671687923)) ;
#90619=CARTESIAN_POINT('Ctrl Pts',(-18.3728209709373,34.6308650483761,124.506586268412)) ;
#90620=CARTESIAN_POINT('Ctrl Pts',(-18.1992525056931,34.6408228130776,124.31075898755)) ;
#90621=CARTESIAN_POINT('Ctrl Pts',(-18.0625580666762,34.6507251544896,124.089319343284)) ;
#90622=CARTESIAN_POINT('Ctrl Pts',(-17.9650433992383,34.660769350196,123.844056094203)) ;
#90623=CARTESIAN_POINT('Ctrl Pts',(-17.9122901221407,34.6706767509553,123.589085907757)) ;
#90624=CARTESIAN_POINT('Ctrl Pts',(-17.9040671219944,34.6806873508296,123.326142620746)) ;
#90625=CARTESIAN_POINT('Ctrl Pts',(-17.942203265216,34.6907176467418,123.065322697016)) ;
#90626=CARTESIAN_POINT('Ctrl Pts',(-18.0232493114111,34.7005724263915,122.819373677744)) ;
#90627=CARTESIAN_POINT('Ctrl Pts',(-18.1463519672124,34.710529754609,122.588461269854)) ;
#90628=CARTESIAN_POINT('Ctrl Pts',(-18.309353042108,34.7205687875159,122.381049743484)) ;
#90629=CARTESIAN_POINT('Ctrl Pts',(-18.5023659383517,34.7304418994052,122.207599723295)) ;
#90630=CARTESIAN_POINT('Ctrl Pts',(-18.7269874138073,34.7405151844323,122.06763353317)) ;
#90631=CARTESIAN_POINT('Ctrl Pts',(-18.966311174259,34.7503355041691,121.970921603636)) ;
#90632=CARTESIAN_POINT('Ctrl Pts',(-19.2252615250139,34.7604141695475,121.915607928114)) ;
#90633=CARTESIAN_POINT('Ctrl Pts',(-19.4840428530472,34.7702657600313,121.906215757302)) ;
#90634=CARTESIAN_POINT('Ctrl Pts',(-19.7462130095486,34.7803389103502,121.942457891797)) ;
#90635=CARTESIAN_POINT('Ctrl Pts',(-19.9923964312408,34.7901812903253,122.021867293698)) ;
#90636=CARTESIAN_POINT('Ctrl Pts',(-20.224633402004,34.8001622665683,122.143734711503)) ;
#90637=CARTESIAN_POINT('Ctrl Pts',(-20.4326722972678,34.8101785949236,122.305014175264)) ;
#90638=CARTESIAN_POINT('Ctrl Pts',(-20.6076836467507,34.8200763919147,122.497420427446)) ;
#90639=CARTESIAN_POINT('Ctrl Pts',(-20.7486352078836,34.8300889486468,122.719624524635)) ;
#90640=CARTESIAN_POINT('Ctrl Pts',(-20.8484693509522,34.8401209834933,122.963608083388)) ;
#90641=CARTESIAN_POINT('Ctrl Pts',(-20.9039852822509,34.8499603843087,123.216169118791)) ;
#90642=CARTESIAN_POINT('Ctrl Pts',(-20.915252015336,34.8600261699603,123.480416453755)) ;
#90643=CARTESIAN_POINT('Ctrl Pts',(-20.8809428954112,34.8699166250749,123.738080890662)) ;
#90644=CARTESIAN_POINT('Ctrl Pts',(-20.8021590268459,34.8799087437107,123.988551842107)) ;
#90645=CARTESIAN_POINT('Ctrl Pts',(-20.6812162451853,34.8898715704737,124.220748500845)) ;
#90646=CARTESIAN_POINT('Ctrl Pts',(-20.5232363311893,34.8997758537466,124.427621791333)) ;
#90647=CARTESIAN_POINT('Ctrl Pts',(-20.328602748606,34.9098362876937,124.606497029424)) ;
#90648=CARTESIAN_POINT('Ctrl Pts',(-20.1108581510111,34.9196768403669,124.746063981003)) ;
#90649=CARTESIAN_POINT('Ctrl Pts',(-19.8670007279919,34.9297390603126,124.848234310547)) ;
#90650=CARTESIAN_POINT('Ctrl Pts',(-19.6132374871759,34.9396361995912,124.9052994767)) ;
#90651=CARTESIAN_POINT('Ctrl Pts',(-19.352586866818,34.9495673917262,124.918345206172)) ;
#90652=CARTESIAN_POINT('Ctrl Pts',(-19.0907761598874,34.9596095463713,124.885281266899)) ;
#90653=CARTESIAN_POINT('Ctrl Pts',(-18.8424935087745,34.9694963073906,124.808663455936)) ;
#90654=CARTESIAN_POINT('Ctrl Pts',(-18.6085514013706,34.9794956091078,124.689074670539)) ;
#90655=CARTESIAN_POINT('Ctrl Pts',(-18.4004100503073,34.9894164072746,124.532024155764)) ;
#90656=CARTESIAN_POINT('Ctrl Pts',(-18.220695374879,34.9994504608713,124.339108184459)) ;
#90657=CARTESIAN_POINT('Ctrl Pts',(-18.0786234259347,35.0093735784377,124.120391230864)) ;
#90658=CARTESIAN_POINT('Ctrl Pts',(-17.9753990929057,35.0194297019368,123.877150159267)) ;
#90659=CARTESIAN_POINT('Ctrl Pts',(-17.917104068257,35.0292751435917,123.62506345845)) ;
#90660=CARTESIAN_POINT('Ctrl Pts',(-17.9024452588224,35.0392374447158,123.36369174523)) ;
#90661=CARTESIAN_POINT('Ctrl Pts',(-17.933946461117,35.0492659239909,123.102025569632)) ;
#90662=CARTESIAN_POINT('Ctrl Pts',(-18.0094085575674,35.0591762775006,122.852777323591)) ;
#90663=CARTESIAN_POINT('Ctrl Pts',(-18.1266927602278,35.0691111496778,122.619516835167)) ;
#90664=CARTESIAN_POINT('Ctrl Pts',(-18.2845521812503,35.0791522872635,122.408084929037)) ;
#90665=CARTESIAN_POINT('Ctrl Pts',(-18.4736704054688,35.0890394364781,122.22989810543)) ;
#90666=CARTESIAN_POINT('Ctrl Pts',(-18.6928945527343,35.0990316712291,122.085390254205)) ;
#90667=CARTESIAN_POINT('Ctrl Pts',(-18.932889746988,35.1089803767921,121.9816540539)) ;
#90668=CARTESIAN_POINT('Ctrl Pts',(-19.1868087710443,35.1189164452158,121.92087877605)) ;
#90669=CARTESIAN_POINT('Ctrl Pts',(-19.4487510389459,35.1289021294316,121.904734357307)) ;
#90670=CARTESIAN_POINT('Ctrl Pts',(-19.7108597155161,35.1389425560002,121.934890399688)) ;
#90671=CARTESIAN_POINT('Ctrl Pts',(-19.9588218803458,35.148781669464,122.008182230702)) ;
#90672=CARTESIAN_POINT('Ctrl Pts',(-20.195037968623,35.1588114036398,122.125114451366)) ;
#90673=CARTESIAN_POINT('Ctrl Pts',(-20.4067898564085,35.1688335031457,122.281715086655)) ;
#90674=CARTESIAN_POINT('Ctrl Pts',(-20.5858406931206,35.1787019430391,122.46934344386)) ;
#90675=CARTESIAN_POINT('Ctrl Pts',(-20.7324825930465,35.1887708077248,122.689561854867)) ;
#90676=CARTESIAN_POINT('Ctrl Pts',(-20.8362960938539,35.1986134808234,122.926479912635)) ;
#90677=CARTESIAN_POINT('Ctrl Pts',(-20.899055079425,35.2085741149858,123.180594616481)) ;
#90678=CARTESIAN_POINT('Ctrl Pts',(-20.9163568869125,35.2186120306639,123.44380305098)) ;
#90679=CARTESIAN_POINT('Ctrl Pts',(-20.8886337721967,35.2284863055234,123.701836099716)) ;
#90680=CARTESIAN_POINT('Ctrl Pts',(-20.815106074293,35.2385560558985,123.956001024207)) ;
#90681=CARTESIAN_POINT('Ctrl Pts',(-20.701400325098,35.248389351273,124.188072701268)) ;
#90682=CARTESIAN_POINT('Ctrl Pts',(-20.5466987675831,35.2584196487526,124.401475805769)) ;
#90683=CARTESIAN_POINT('Ctrl Pts',(-20.3567063540923,35.2684517351941,124.584263100217)) ;
#90684=CARTESIAN_POINT('Ctrl Pts',(-20.1426513521819,35.278279663683,124.72875221101)) ;
#90685=CARTESIAN_POINT('Ctrl Pts',(-19.9030046171071,35.2882757047938,124.836324512499)) ;
#90686=CARTESIAN_POINT('Ctrl Pts',(-19.6474276615906,35.298301516895,124.900352262788)) ;
#90687=CARTESIAN_POINT('Ctrl Pts',(-19.3882751938659,35.3081887517898,124.919108279541)) ;
#90688=CARTESIAN_POINT('Ctrl Pts',(-19.1274391236298,35.3181656180008,124.892776277121)) ;
#90689=CARTESIAN_POINT('Ctrl Pts',(-18.8746646646945,35.3281585618726,124.821468377364)) ;
#90690=CARTESIAN_POINT('Ctrl Pts',(-18.6372430900327,35.338196484544,124.706562893995)) ;
#90691=CARTESIAN_POINT('Ctrl Pts',(-18.4271550056594,35.3480449488057,124.555385469111)) ;
#90692=CARTESIAN_POINT('Ctrl Pts',(-18.2435829818069,35.3580368155497,124.367696236912)) ;
#90693=CARTESIAN_POINT('Ctrl Pts',(-18.0963252747795,35.3679545475909,124.152615497661)) ;
#90694=CARTESIAN_POINT('Ctrl Pts',(-17.9874096726993,35.3779827324862,123.912669454081)) ;
#90695=CARTESIAN_POINT('Ctrl Pts',(-17.9226347534564,35.387867890535,123.66109622289)) ;
#90696=CARTESIAN_POINT('Ctrl Pts',(-17.9016765666423,35.3978572510767,123.39941901094)) ;
#90697=CARTESIAN_POINT('Ctrl Pts',(-17.9271558083283,35.4078984080111,123.136781335397)) ;
#90698=CARTESIAN_POINT('Ctrl Pts',(-17.9959687525466,35.4177309914662,122.88772650032)) ;
#90699=CARTESIAN_POINT('Ctrl Pts',(-18.1081319471754,35.4277252114282,122.650247800051)) ;
#90700=CARTESIAN_POINT('Ctrl Pts',(-18.2607849253877,35.4377533132155,122.435427774985)) ;
#90701=CARTESIAN_POINT('Ctrl Pts',(-18.4453853520115,35.4476332578386,122.252848690864)) ;
#90702=CARTESIAN_POINT('Ctrl Pts',(-18.6610214269731,35.4576235843956,122.103123520847)) ;
#90703=CARTESIAN_POINT('Ctrl Pts',(-18.8982196683709,35.4675645160499,121.993647605999)) ;
#90704=CARTESIAN_POINT('Ctrl Pts',(-19.1519136468404,35.4775516345528,121.926344805637)) ;
#90705=CARTESIAN_POINT('Ctrl Pts',(-19.4146479680384,35.48758496745,121.904428438846)) ;
#90706=CARTESIAN_POINT('Ctrl Pts',(-19.6729148068661,35.4974510718947,121.927562236653)) ;
#90707=CARTESIAN_POINT('Ctrl Pts',(-19.9282737618614,35.5075171857751,121.996483449793)) ;
#90708=CARTESIAN_POINT('Ctrl Pts',(-20.1628377208178,35.5173731975435,122.106361679407)) ;
#90709=CARTESIAN_POINT('Ctrl Pts',(-20.3781660934209,35.5273679011748,122.256744946492)) ;
#90710=CARTESIAN_POINT('Ctrl Pts',(-20.5644031071723,35.5373992368997,122.443319308297)) ;
#90711=CARTESIAN_POINT('Ctrl Pts',(-20.7132753997824,35.5472657621033,122.655613795221)) ;
#90712=CARTESIAN_POINT('Ctrl Pts',(-20.824735991116,35.5572531901491,122.893195278124)) ;
#90713=CARTESIAN_POINT('Ctrl Pts',(-20.8931143715501,35.5671981198355,123.145473611636)) ;
#90714=CARTESIAN_POINT('Ctrl Pts',(-20.916731989703,35.5772430379441,123.408359549251)) ;
#90715=CARTESIAN_POINT('Ctrl Pts',(-20.8949804435051,35.587105007558,123.66662867698)) ;
#90716=CARTESIAN_POINT('Ctrl Pts',(-20.8283478671713,35.5970970755792,123.920587710675)) ;
#90717=CARTESIAN_POINT('Ctrl Pts',(-20.719243324381,35.6070280009538,124.157679141684)) ;
#90718=CARTESIAN_POINT('Ctrl Pts',(-20.5707147508326,35.6169786291772,124.372871095378)) ;
#90719=CARTESIAN_POINT('Ctrl Pts',(-20.3862369565019,35.6269788682363,124.560073078809)) ;
#90720=CARTESIAN_POINT('Ctrl Pts',(-20.1712640574126,35.6370073236055,124.712497104667)) ;
#90721=CARTESIAN_POINT('Ctrl Pts',(-19.9370958263856,35.6468733581888,124.823815964018)) ;
#90722=CARTESIAN_POINT('Ctrl Pts',(-19.6841078343026,35.6568656799362,124.894073754451)) ;
#90723=CARTESIAN_POINT('Ctrl Pts',(-19.4242931282444,35.6667979696132,124.919232541197)) ;
#90724=CARTESIAN_POINT('Ctrl Pts',(-19.1622457507477,35.676799614584,124.89901214049)) ;
#90725=CARTESIAN_POINT('Ctrl Pts',(-18.8234350299955,35.690112248,124.811793581749)) ;
#90726=CARTESIAN_POINT('Ctrl Pts',(-18.5168964604078,35.7033439973816,124.639445590766)) ;
#90727=CARTESIAN_POINT('Ctrl Pts',(-18.2664225908945,35.7166672621986,124.394805388771)) ;
#90728=CARTESIAN_POINT('Ctrl Pts',(-18.1147450135693,35.7265429684163,124.184207203932)) ;
#90729=CARTESIAN_POINT('Ctrl Pts',(-18.0003454842561,35.7365325595163,123.947960343234)) ;
#90730=CARTESIAN_POINT('Ctrl Pts',(-17.9289701667244,35.7464596559717,123.697008534527)) ;
#90731=CARTESIAN_POINT('Ctrl Pts',(-17.9019627690378,35.7564848044763,123.434969684401)) ;
#90732=CARTESIAN_POINT('Ctrl Pts',(-17.9204625057985,35.766380458623,123.175558526549)) ;
#90733=CARTESIAN_POINT('Ctrl Pts',(-17.9840399510721,35.7763839930012,122.920505986074)) ;
#90734=CARTESIAN_POINT('Ctrl Pts',(-18.0907912526402,35.7863691314413,122.680759611974)) ;
#90735=CARTESIAN_POINT('Ctrl Pts',(-18.2384845563749,35.7964050560366,122.462276828214)) ;
#90736=CARTESIAN_POINT('Ctrl Pts',(-18.4182832581623,35.8062563314643,122.276022071899)) ;
#90737=CARTESIAN_POINT('Ctrl Pts',(-18.6302545916797,35.8162485926257,122.121024656498)) ;
#90738=CARTESIAN_POINT('Ctrl Pts',(-18.8673155093982,35.8262884766433,122.005244450248)) ;
#90739=CARTESIAN_POINT('Ctrl Pts',(-19.1155599860478,35.8361232511457,121.93323039927)) ;
#90740=CARTESIAN_POINT('Ctrl Pts',(-19.3787662820051,35.846199632166,121.90464170685)) ;
#90741=CARTESIAN_POINT('Ctrl Pts',(-19.6369856027935,35.8560459053166,121.921721200336)) ;
#90742=CARTESIAN_POINT('Ctrl Pts',(-19.9782318745606,35.8694104266019,122.004755386422)) ;
#90743=CARTESIAN_POINT('Ctrl Pts',(-20.2860781894191,35.8826166710363,122.173358222392)) ;
#90744=CARTESIAN_POINT('Ctrl Pts',(-20.5388194305417,35.8958816257135,122.413415383819)) ;
#90745=CARTESIAN_POINT('Ctrl Pts',(-20.6954518663001,35.9059139062652,122.625487616004)) ;
#90746=CARTESIAN_POINT('Ctrl Pts',(-20.8114494728934,35.9158226397831,122.858608403369)) ;
#90747=CARTESIAN_POINT('Ctrl Pts',(-20.8860782708486,35.9257601906506,123.108875396054)) ;
#90748=CARTESIAN_POINT('Ctrl Pts',(-20.9161752733181,35.9357900382445,123.370700554843)) ;
#90749=CARTESIAN_POINT('Ctrl Pts',(-20.8957731929268,35.949025178165,123.717991080168)) ;
#90750=CARTESIAN_POINT('Ctrl Pts',(-20.7562782646861,35.9656936425361,124.138331425498)) ;
#90751=CARTESIAN_POINT('Ctrl Pts',(-20.4290918169683,35.98556465441,124.553143935095)) ;
#90752=CARTESIAN_POINT('Ctrl Pts',(-20.0516669376428,36.002271738793,124.786848654509)) ;
#90753=CARTESIAN_POINT('Ctrl Pts',(-19.7200488034031,36.0154490201036,124.886772678737)) ;
#90754=CARTESIAN_POINT('Ctrl Pts',(-19.3739896601812,36.0287164806177,124.929104605177)) ;
#90755=CARTESIAN_POINT('Ctrl Pts',(-18.9367256618785,36.0453303713049,124.867571649377)) ;
#90756=CARTESIAN_POINT('Ctrl Pts',(-18.4683585867537,36.0652791707323,124.618963683723)) ;
#90757=CARTESIAN_POINT('Ctrl Pts',(-18.1135879764182,36.0852002822632,124.2260271695)) ;
#90758=CARTESIAN_POINT('Ctrl Pts',(-17.9136719684102,36.1050667304361,123.737230065052)) ;
#90759=CARTESIAN_POINT('Ctrl Pts',(-17.8927126209991,36.1250930770532,123.205433374261)) ;
#90760=CARTESIAN_POINT('Ctrl Pts',(-18.0533007215964,36.1449551214427,122.702455916173)) ;
#90761=CARTESIAN_POINT('Ctrl Pts',(-18.3764776353452,36.1649004241238,122.282339628229)) ;
#90762=CARTESIAN_POINT('Ctrl Pts',(-18.8226158877263,36.1847957311827,121.998462474444)) ;
#90763=CARTESIAN_POINT('Ctrl Pts',(-19.3385842783177,36.2046890013503,121.882951679264)) ;
#90764=CARTESIAN_POINT('Ctrl Pts',(-19.8648495105545,36.2246545940308,121.950798037064)) ;
#90765=CARTESIAN_POINT('Ctrl Pts',(-20.334465653922,36.2445299177156,122.192756268591)) ;
#90766=CARTESIAN_POINT('Ctrl Pts',(-20.6955169132806,36.2645049802905,122.582020760569)) ;
#90767=CARTESIAN_POINT('Ctrl Pts',(-20.9010738348726,36.2844573899217,123.070861900805)) ;
#90768=CARTESIAN_POINT('Ctrl Pts',(-20.9283436001929,36.3042934441578,123.597363126459)) ;
#90769=CARTESIAN_POINT('Ctrl Pts',(-20.7737705212242,36.3242713555753,124.10534582472)) ;
#90770=CARTESIAN_POINT('Ctrl Pts',(-20.4556033727974,36.3441894050788,124.528410951894)) ;
#90771=CARTESIAN_POINT('Ctrl Pts',(-20.0139153720363,36.3640575488469,124.818025234808)) ;
#90772=CARTESIAN_POINT('Ctrl Pts',(-19.4952301669597,36.3841084054342,124.939796977761)) ;
#90773=CARTESIAN_POINT('Ctrl Pts',(-18.9729215440468,36.4038888418901,124.878628473693)) ;
#90774=CARTESIAN_POINT('Ctrl Pts',(-18.4967651240595,36.4239188975679,124.640802577976)) ;
#90775=CARTESIAN_POINT('Ctrl Pts',(-18.1335848516454,36.4438000027427,124.25686352696)) ;
#90776=CARTESIAN_POINT('Ctrl Pts',(-17.9219195474901,36.4636804651105,123.77277946085)) ;
#90777=CARTESIAN_POINT('Ctrl Pts',(-17.8881151233781,36.4836656122549,123.242666380459)) ;
#90778=CARTESIAN_POINT('Ctrl Pts',(-18.0366553794252,36.5035561907912,122.73529278596)) ;
#90779=CARTESIAN_POINT('Ctrl Pts',(-18.3487072158258,36.5234502106656,122.308453160384)) ;
#90780=CARTESIAN_POINT('Ctrl Pts',(-18.7881486981132,36.543371655392,122.013243316393)) ;
#90781=CARTESIAN_POINT('Ctrl Pts',(-19.3013483876729,36.5632697934474,121.884892286894)) ;
#90782=CARTESIAN_POINT('Ctrl Pts',(-19.8317595038524,36.5833405486635,121.940839429391)) ;
#90783=CARTESIAN_POINT('Ctrl Pts',(-20.3047244450388,36.6031260987147,122.170976388332)) ;
#90784=CARTESIAN_POINT('Ctrl Pts',(-20.6751961018729,36.6231091735921,122.551414789717)) ;
#90785=CARTESIAN_POINT('Ctrl Pts',(-20.8920876251874,36.643018256238,123.034079238211)) ;
#90786=CARTESIAN_POINT('Ctrl Pts',(-20.9326736949197,36.6628768153608,123.560393777446)) ;
#90787=CARTESIAN_POINT('Ctrl Pts',(-20.7893507745121,36.6829202591995,124.073361851782)) ;
#90788=CARTESIAN_POINT('Ctrl Pts',(-20.5344135959182,36.6994203239287,124.430349947457)) ;
#90789=CARTESIAN_POINT('Ctrl Pts',(-20.2630412458369,36.7128100637776,124.654248532504)) ;
#90790=CARTESIAN_POINT('Ctrl Pts',(-20.0376657911243,36.722666964986,124.781998493706)) ;
#90791=CARTESIAN_POINT('Ctrl Pts',(-19.790451891043,36.7326584908325,124.870339079412)) ;
#90792=CARTESIAN_POINT('Ctrl Pts',(-19.5333205208731,36.7425831712835,124.914226210988)) ;
#90793=CARTESIAN_POINT('Ctrl Pts',(-19.2702961550599,36.7525937613279,124.912889798325)) ;
#90794=CARTESIAN_POINT('Ctrl Pts',(-18.9272992756477,36.7658530220315,124.851022900053)) ;
#90795=CARTESIAN_POINT('Ctrl Pts',(-18.6064416437255,36.7792040971818,124.699737523157)) ;
#90796=CARTESIAN_POINT('Ctrl Pts',(-18.3413179144251,36.7924104064166,124.475682143339)) ;
#90797=CARTESIAN_POINT('Ctrl Pts',(-18.1729500479038,36.8023972400069,124.274423037726)) ;
#90798=CARTESIAN_POINT('Ctrl Pts',(-18.0423739740692,36.812349967503,124.047750299169)) ;
#90799=CARTESIAN_POINT('Ctrl Pts',(-17.952518013425,36.8223980643446,123.799486638763)) ;
#90800=CARTESIAN_POINT('Ctrl Pts',(-17.907757267272,36.8322395212164,123.544740945739)) ;
#90801=CARTESIAN_POINT('Ctrl Pts',(-17.9073502062391,36.8422257881299,123.282355578864)) ;
#90802=CARTESIAN_POINT('Ctrl Pts',(-17.9521694205823,36.8521623890303,123.025063136411)) ;
#90803=CARTESIAN_POINT('Ctrl Pts',(-18.0420963058471,36.8622123318174,122.776771029239)) ;
#90804=CARTESIAN_POINT('Ctrl Pts',(-18.1710052785227,36.8720625315031,122.552279193621)) ;
#90805=CARTESIAN_POINT('Ctrl Pts',(-18.3384408575299,36.8820354364352,122.350698607091)) ;
#90806=CARTESIAN_POINT('Ctrl Pts',(-18.5389463808558,36.8920338109148,122.18084427361)) ;
#90807=CARTESIAN_POINT('Ctrl Pts',(-18.7664541058527,36.9020539847848,122.048279786072)) ;
#90808=CARTESIAN_POINT('Ctrl Pts',(-19.0105222002321,36.9119550287268,121.95809778858)) ;
#90809=CARTESIAN_POINT('Ctrl Pts',(-19.268728383313,36.9219438324511,121.910847088745)) ;
#90810=CARTESIAN_POINT('Ctrl Pts',(-19.5305939085291,36.9319092992829,121.909337770446)) ;
#90811=CARTESIAN_POINT('Ctrl Pts',(-19.7872824216961,36.9418128615559,121.95243202349)) ;
#90812=CARTESIAN_POINT('Ctrl Pts',(-20.0363517848326,36.9518735394339,122.041006819332)) ;
#90813=CARTESIAN_POINT('Ctrl Pts',(-20.2614482794892,36.9617138373834,122.1683698474)) ;
#90814=CARTESIAN_POINT('Ctrl Pts',(-20.4656746860891,36.9717768322928,122.336311677907)) ;
#90815=CARTESIAN_POINT('Ctrl Pts',(-20.6346325844978,36.9816711264399,122.533982970242)) ;
#90816=CARTESIAN_POINT('Ctrl Pts',(-20.7679155889213,36.9916129241368,122.758650934849)) ;
#90817=CARTESIAN_POINT('Ctrl Pts',(-20.8608421966797,37.0016155016659,123.004571300072)) ;
#90818=CARTESIAN_POINT('Ctrl Pts',(-20.9094048501918,37.011649965587,123.26374268831)) ;
#90819=CARTESIAN_POINT('Ctrl Pts',(-20.9125815920894,37.0214961041081,123.522477689503)) ;
#90820=CARTESIAN_POINT('Ctrl Pts',(-20.8707936127288,37.0314772773451,123.781401079755)) ;
#90821=CARTESIAN_POINT('Ctrl Pts',(-20.7848638119868,37.0414295713023,124.028425816195)) ;
#90822=CARTESIAN_POINT('Ctrl Pts',(-20.6570438981956,37.0514283664369,124.258022088148)) ;
#90823=CARTESIAN_POINT('Ctrl Pts',(-20.4902612991329,37.0614674746977,124.462411340172)) ;
#90824=CARTESIAN_POINT('Ctrl Pts',(-20.2951235539568,37.0712924161369,124.631500866346)) ;
#90825=CARTESIAN_POINT('Ctrl Pts',(-20.0686616200432,37.0813471032113,124.767597084672)) ;
#90826=CARTESIAN_POINT('Ctrl Pts',(-19.8245710827869,37.0912899081514,124.860842297865)) ;
#90827=CARTESIAN_POINT('Ctrl Pts',(-19.5691588004271,37.1011936941479,124.910878499083)) ;
#90828=CARTESIAN_POINT('Ctrl Pts',(-19.3052063233042,37.1112405107127,124.915717087351)) ;
#90829=CARTESIAN_POINT('Ctrl Pts',(-19.0482495106725,37.1211360301914,124.875491392646)) ;
#90830=CARTESIAN_POINT('Ctrl Pts',(-18.7981148297119,37.1311981155158,124.789869782215)) ;
#90831=CARTESIAN_POINT('Ctrl Pts',(-18.5715632075335,37.1410408264737,124.664999559399)) ;
#90832=CARTESIAN_POINT('Ctrl Pts',(-18.3667645398744,37.1510315437798,124.500772902301)) ;
#90833=CARTESIAN_POINT('Ctrl Pts',(-18.1946815226206,37.1609596268764,124.304654257152)) ;
#90834=CARTESIAN_POINT('Ctrl Pts',(-18.0580587042926,37.1709475569881,124.080530224495)) ;
#90835=CARTESIAN_POINT('Ctrl Pts',(-17.9623882859192,37.1809833831154,123.834772735687)) ;
#90836=CARTESIAN_POINT('Ctrl Pts',(-17.9113591892937,37.190838720229,123.580846703996)) ;
#90837=CARTESIAN_POINT('Ctrl Pts',(-17.9046918793828,37.2008364550792,123.318229679078)) ;
#90838=CARTESIAN_POINT('Ctrl Pts',(-17.9432929783789,37.2107443590637,123.060725439739)) ;
#90839=CARTESIAN_POINT('Ctrl Pts',(-18.0264609446868,37.2207554336121,122.811128639324)) ;
#90840=CARTESIAN_POINT('Ctrl Pts',(-18.1523845768401,37.2307832891477,122.579637946315)) ;
#90841=CARTESIAN_POINT('Ctrl Pts',(-18.313434602913,37.240640883053,122.376742009224)) ;
#90842=CARTESIAN_POINT('Ctrl Pts',(-18.510241481172,37.2506675698911,122.201537057415)) ;
#90843=CARTESIAN_POINT('Ctrl Pts',(-18.7348729634303,37.2606962390448,122.063695449204)) ;
#90844=CARTESIAN_POINT('Ctrl Pts',(-18.9753445770678,37.2705414473262,121.96828080011)) ;
#90845=CARTESIAN_POINT('Ctrl Pts',(-19.2323500330995,37.2805321362893,121.914602131553)) ;
#90846=CARTESIAN_POINT('Ctrl Pts',(-19.4960202224024,37.2905700125716,121.9069126897)) ;
#90847=CARTESIAN_POINT('Ctrl Pts',(-19.7520669609929,37.3004143902138,121.943940420464)) ;
#90848=CARTESIAN_POINT('Ctrl Pts',(-20.0014193408441,37.3103991946052,122.025510816322)) ;
#90849=CARTESIAN_POINT('Ctrl Pts',(-20.2318871717339,37.3203387248238,122.148511202845)) ;
#90850=CARTESIAN_POINT('Ctrl Pts',(-20.4394866075736,37.3303784128607,122.311296862849)) ;
#90851=CARTESIAN_POINT('Ctrl Pts',(-20.6131300585679,37.340266702229,122.504635758308)) ;
#90852=CARTESIAN_POINT('Ctrl Pts',(-20.7523750420527,37.3502558259138,122.727153728378)) ;
#90853=CARTESIAN_POINT('Ctrl Pts',(-20.8503938939143,37.3602158355884,122.969841158144)) ;
#90854=CARTESIAN_POINT('Ctrl Pts',(-20.9050687368293,37.3701162652927,123.224212899945)) ;
#90855=CARTESIAN_POINT('Ctrl Pts',(-20.9148721088486,37.3801593466994,123.487941036205)) ;
#90856=CARTESIAN_POINT('Ctrl Pts',(-20.8792246033343,37.390066740607,123.745859387518)) ;
#90857=CARTESIAN_POINT('Ctrl Pts',(-20.7989609173973,37.4000784715962,123.996417274373)) ;
#90858=CARTESIAN_POINT('Ctrl Pts',(-20.6756955451906,37.410110689311,124.22947112403)) ;
#90859=CARTESIAN_POINT('Ctrl Pts',(-20.51702591384,37.4199631985572,124.434050623572)) ;
#90860=CARTESIAN_POINT('Ctrl Pts',(-20.3237233572184,37.4299211351002,124.610450271903)) ;
#90861=CARTESIAN_POINT('Ctrl Pts',(-20.1007000293467,37.4399600051085,124.751331487019)) ;
#90862=CARTESIAN_POINT('Ctrl Pts',(-19.8607616035958,37.4498331602667,124.850169231509)) ;
#90863=CARTESIAN_POINT('Ctrl Pts',(-19.602246757542,37.4599064351164,124.906872980276)) ;
#90864=CARTESIAN_POINT('Ctrl Pts',(-19.3443562287078,37.4697267522938,124.917896850224)) ;
#90865=CARTESIAN_POINT('Ctrl Pts',(-19.0818283552624,37.4798054380873,124.883340221226)) ;
#90866=CARTESIAN_POINT('Ctrl Pts',(-18.8348322832029,37.4896569494704,124.805570098911)) ;
#90867=CARTESIAN_POINT('Ctrl Pts',(-18.599913832951,37.499730395777,124.683655014206)) ;
#90868=CARTESIAN_POINT('Ctrl Pts',(-18.3945253990698,37.5095716709017,124.526446904205)) ;
#90869=CARTESIAN_POINT('Ctrl Pts',(-18.2164310699433,37.5195567705585,124.333775949038)) ;
#90870=CARTESIAN_POINT('Ctrl Pts',(-18.0744621012236,37.5295642466928,124.11237858257)) ;
#90871=CARTESIAN_POINT('Ctrl Pts',(-17.9737434063258,37.5394868344017,123.871874033015)) ;
#90872=CARTESIAN_POINT('Ctrl Pts',(-17.9155198712875,37.5494734386751,123.615951736417)) ;
#90873=CARTESIAN_POINT('Ctrl Pts',(-17.9030442398782,37.5595135670092,123.352424180443)) ;
#90874=CARTESIAN_POINT('Ctrl Pts',(-17.9352929472443,37.5693530015426,123.095845830502)) ;
#90875=CARTESIAN_POINT('Ctrl Pts',(-18.0131166461626,37.5794170560336,122.843116592569)) ;
#90876=CARTESIAN_POINT('Ctrl Pts',(-18.1316981730949,37.5893079752708,122.611787994209)) ;
#90877=CARTESIAN_POINT('Ctrl Pts',(-18.2897770295622,37.5992999685768,122.402140602484)) ;
#90878=CARTESIAN_POINT('Ctrl Pts',(-18.4814669497025,37.6092628325361,122.223821161659)) ;
#90879=CARTESIAN_POINT('Ctrl Pts',(-18.6995802858491,37.6191670923539,122.081762570876)) ;
#90880=CARTESIAN_POINT('Ctrl Pts',(-18.9428624159537,37.6292275829253,121.978356993375)) ;
#90881=CARTESIAN_POINT('Ctrl Pts',(-19.1947597030667,37.6390679325563,121.919723653256)) ;
#90882=CARTESIAN_POINT('Ctrl Pts',(-19.4587639337918,37.6491309080463,121.905087450184)) ;
#90883=CARTESIAN_POINT('Ctrl Pts',(-19.7169360685854,37.6590252281897,121.936206707452)) ;
#90884=CARTESIAN_POINT('Ctrl Pts',(-19.9671186320429,37.6689669413213,122.011348625595)) ;
#90885=CARTESIAN_POINT('Ctrl Pts',(-20.2020080675906,37.6789698311154,122.129443636696)) ;
#90886=CARTESIAN_POINT('Ctrl Pts',(-20.4132615576,37.6890096882759,122.287457794107)) ;
#90887=CARTESIAN_POINT('Ctrl Pts',(-20.5904502427968,37.6988338691135,122.475251891521)) ;
#90888=CARTESIAN_POINT('Ctrl Pts',(-20.735982916264,37.7088908426167,122.69583339334)) ;
#90889=CARTESIAN_POINT('Ctrl Pts',(-20.8393694687883,37.7188189668038,122.93539179218)) ;
#90890=CARTESIAN_POINT('Ctrl Pts',(-20.9004226762574,37.7287726618772,123.18974167518)) ;
#90891=CARTESIAN_POINT('Ctrl Pts',(-20.9161571182402,37.7388188554525,123.453273135493)) ;
#90892=CARTESIAN_POINT('Ctrl Pts',(-20.8867385875313,37.7486669578124,123.710392738064)) ;
#90893=CARTESIAN_POINT('Ctrl Pts',(-20.8130541065125,37.75862854604,123.96157704454)) ;
#90894=CARTESIAN_POINT('Ctrl Pts',(-20.6957843077402,37.7686572161963,124.197608569847)) ;
#90895=CARTESIAN_POINT('Ctrl Pts',(-20.5412434271641,37.778567519078,124.407217781717)) ;
#90896=CARTESIAN_POINT('Ctrl Pts',(-20.352645450369,37.7885024028859,124.58776383537)) ;
#90897=CARTESIAN_POINT('Ctrl Pts',(-20.133119143806,37.7985435445765,124.734158279139)) ;
#90898=CARTESIAN_POINT('Ctrl Pts',(-19.895266526059,37.8084306657405,124.838762309883)) ;
#90899=CARTESIAN_POINT('Ctrl Pts',(-19.6403142341081,37.818423008589,124.901552440905)) ;
#90900=CARTESIAN_POINT('Ctrl Pts',(-19.3794511200074,37.828371309813,124.918971337681)) ;
#90901=CARTESIAN_POINT('Ctrl Pts',(-19.1197938910939,37.8383088874951,124.891242488897)) ;
#90902=CARTESIAN_POINT('Ctrl Pts',(-18.8675519902502,37.8482954619457,124.818740589761)) ;
#90903=CARTESIAN_POINT('Ctrl Pts',(-18.6308845594972,37.8583242718541,124.702791487369)) ;
#90904=CARTESIAN_POINT('Ctrl Pts',(-18.4209911500482,37.8682025931609,124.550044711612)) ;
#90905=CARTESIAN_POINT('Ctrl Pts',(-18.2382893834789,37.8781942405083,124.361450555223)) ;
#90906=CARTESIAN_POINT('Ctrl Pts',(-18.0909361216224,37.8882287639461,124.142780458619)) ;
#90907=CARTESIAN_POINT('Ctrl Pts',(-17.9851082426078,37.8980921208247,123.90613973582)) ;
#90908=CARTESIAN_POINT('Ctrl Pts',(-17.9206158973704,37.908162347505,123.649512993499)) ;
#90909=CARTESIAN_POINT('Ctrl Pts',(-17.9021014477694,37.9180046556397,123.391519278401)) ;
#90910=CARTESIAN_POINT('Ctrl Pts',(-17.9280213893312,37.9279653876631,123.131054268142)) ;
#90911=CARTESIAN_POINT('Ctrl Pts',(-17.9998223639555,37.9380032768612,122.877238454483)) ;
#90912=CARTESIAN_POINT('Ctrl Pts',(-18.1123180047447,37.94787755978,122.643370168163)) ;
#90913=CARTESIAN_POINT('Ctrl Pts',(-18.2666811956989,37.9579473043975,122.428479079685)) ;
#90914=CARTESIAN_POINT('Ctrl Pts',(-18.4515097019627,37.9677806147431,122.247856374346)) ;
#90915=CARTESIAN_POINT('Ctrl Pts',(-18.6687188341038,37.9778108580958,122.098544975013)) ;
#90916=CARTESIAN_POINT('Ctrl Pts',(-18.9089398495734,37.9878431460742,121.989907265577)) ;
#90917=CARTESIAN_POINT('Ctrl Pts',(-19.1589973603507,37.9976703225423,121.925371796745)) ;
#90918=CARTESIAN_POINT('Ctrl Pts',(-19.4210528476622,38.0076757054092,121.904329796489)) ;
#90919=CARTESIAN_POINT('Ctrl Pts',(-19.6822603276462,38.0176583444019,121.929146579502)) ;
#90920=CARTESIAN_POINT('Ctrl Pts',(-19.9365866650456,38.0277024115385,121.999661380241)) ;
#90921=CARTESIAN_POINT('Ctrl Pts',(-20.1697455284941,38.0375236303425,122.110354265076)) ;
#90922=CARTESIAN_POINT('Ctrl Pts',(-20.3851407356152,38.0475604692805,122.262573522578)) ;
#90923=CARTESIAN_POINT('Ctrl Pts',(-20.5700791380799,38.0575848813783,122.450185779491)) ;
#90924=CARTESIAN_POINT('Ctrl Pts',(-20.7175310391498,38.0674369657836,122.663002255422)) ;
#90925=CARTESIAN_POINT('Ctrl Pts',(-20.8276645507075,38.0774278625268,122.901301885871)) ;
#90926=CARTESIAN_POINT('Ctrl Pts',(-20.8944393360025,38.0873458544277,123.153269837169)) ;
#90927=CARTESIAN_POINT('Ctrl Pts',(-20.916752709306,38.0973739698847,123.415831037644)) ;
#90928=CARTESIAN_POINT('Ctrl Pts',(-20.89358187262,38.1072591458268,123.674574253975)) ;
#90929=CARTESIAN_POINT('Ctrl Pts',(-20.8257391871181,38.1172485042337,123.928171654191)) ;
#90930=CARTESIAN_POINT('Ctrl Pts',(-20.7138167717013,38.127289651814,124.167129479311)) ;
#90931=CARTESIAN_POINT('Ctrl Pts',(-20.5656061454427,38.1371222748204,124.378785103182)) ;
#90932=CARTESIAN_POINT('Ctrl Pts',(-20.3804240799344,38.1471163459312,124.565013167833)) ;
#90933=CARTESIAN_POINT('Ctrl Pts',(-20.1646606886898,38.1571450035721,124.716368185705)) ;
#90934=CARTESIAN_POINT('Ctrl Pts',(-19.9294754177371,38.1670293297649,124.826601817947)) ;
#90935=CARTESIAN_POINT('Ctrl Pts',(-19.6768051124309,38.1769950732555,124.89551183432)) ;
#90936=CARTESIAN_POINT('Ctrl Pts',(-19.4143545698229,38.1870234523867,124.919272831667)) ;
#90937=CARTESIAN_POINT('Ctrl Pts',(-19.155026247405,38.1969242985936,124.897774472843)) ;
#90938=CARTESIAN_POINT('Ctrl Pts',(-18.899449911136,38.2069829560107,124.830469885562)) ;
#90939=CARTESIAN_POINT('Ctrl Pts',(-18.6640472589483,38.2168405187926,124.72223521876)) ;
#90940=CARTESIAN_POINT('Ctrl Pts',(-18.4464297173287,38.2269089213458,124.571809104608)) ;
#90941=CARTESIAN_POINT('Ctrl Pts',(-18.262192640318,38.2367643200854,124.389754401548)) ;
#90942=CARTESIAN_POINT('Ctrl Pts',(-18.1096196037123,38.2467591871593,124.175968694404)) ;
#90943=CARTESIAN_POINT('Ctrl Pts',(-17.9965795627306,38.2567904821428,123.937817735641)) ;
#90944=CARTESIAN_POINT('Ctrl Pts',(-17.9273563602029,38.2666570068693,123.687937654047)) ;
#90945=CARTESIAN_POINT('Ctrl Pts',(-17.9018527032758,38.276644477565,123.426751350671)) ;
#90946=CARTESIAN_POINT('Ctrl Pts',(-17.9218607437343,38.2865892371289,123.166140198543)) ;
#90947=CARTESIAN_POINT('Ctrl Pts',(-17.9876155290226,38.2966347930777,122.910504235427)) ;
#90948=CARTESIAN_POINT('Ctrl Pts',(-18.0945121468168,38.3064943814529,122.674449960714)) ;
#90949=CARTESIAN_POINT('Ctrl Pts',(-18.2424996480843,38.3164953365889,122.457313423853)) ;
#90950=CARTESIAN_POINT('Ctrl Pts',(-18.4240798301571,38.3263995638665,122.270788969546)) ;
#90951=CARTESIAN_POINT('Ctrl Pts',(-18.6381236155899,38.3364416407616,122.116493175448)) ;
#90952=CARTESIAN_POINT('Ctrl Pts',(-18.8725441547087,38.3463492534478,122.003091772094)) ;
#90953=CARTESIAN_POINT('Ctrl Pts',(-19.1267212481479,38.3564037840635,121.931068647469)) ;
#90954=CARTESIAN_POINT('Ctrl Pts',(-19.3845339848272,38.3662645706124,121.904631230091)) ;
#90955=CARTESIAN_POINT('Ctrl Pts',(-19.6464652984615,38.3762583256834,121.92312229318)) ;
#90956=CARTESIAN_POINT('Ctrl Pts',(-19.8995750129763,38.3861836859234,121.986273003471)) ;
#90957=CARTESIAN_POINT('Ctrl Pts',(-20.140272020409,38.3962116153187,122.093470120755)) ;
#90958=CARTESIAN_POINT('Ctrl Pts',(-20.3558252995868,38.406097882118,122.238568442777)) ;
#90959=CARTESIAN_POINT('Ctrl Pts',(-20.5456984409777,38.4161296510163,122.42138753169)) ;
#90960=CARTESIAN_POINT('Ctrl Pts',(-20.698877922451,38.4260112468599,122.631132419724)) ;
#90961=CARTESIAN_POINT('Ctrl Pts',(-20.8154213762224,38.4360731323278,122.8684346522)) ;
#90962=CARTESIAN_POINT('Ctrl Pts',(-20.8875986677405,38.4459305663467,123.117253823727)) ;
#90963=CARTESIAN_POINT('Ctrl Pts',(-20.9164045121782,38.4559238093887,123.378246907377)) ;
#90964=CARTESIAN_POINT('Ctrl Pts',(-20.8995775457113,38.465854570275,123.638690081529)) ;
#90965=CARTESIAN_POINT('Ctrl Pts',(-20.816850334482,38.4792035624722,123.979625573362)) ;
#90966=CARTESIAN_POINT('Ctrl Pts',(-20.6476612787041,38.4924719352886,124.289010646964)) ;
#90967=CARTESIAN_POINT('Ctrl Pts',(-20.4070708455003,38.505754876673,124.541958141041)) ;
#90968=CARTESIAN_POINT('Ctrl Pts',(-20.1946437063502,38.5157976625152,124.698532719528)) ;
#90969=CARTESIAN_POINT('Ctrl Pts',(-19.9628978193437,38.5256476050673,124.813858968729)) ;
#90970=CARTESIAN_POINT('Ctrl Pts',(-19.7111423066587,38.5356448379863,124.888916493239)) ;
#90971=CARTESIAN_POINT('Ctrl Pts',(-19.4496444734046,38.5456597333208,124.918770576671)) ;
#90972=CARTESIAN_POINT('Ctrl Pts',(-19.102347554309,38.558899409959,124.897958325602)) ;
#90973=CARTESIAN_POINT('Ctrl Pts',(-18.6847987628518,38.5754466343643,124.759928991449)) ;
#90974=CARTESIAN_POINT('Ctrl Pts',(-18.3371659709119,38.5920940714954,124.486215378783)) ;
#90975=CARTESIAN_POINT('Ctrl Pts',(-18.1282833266673,38.6053835689736,124.206304846633)) ;
#90976=CARTESIAN_POINT('Ctrl Pts',(-18.0108766480719,38.615256976796,123.974924396754)) ;
#90977=CARTESIAN_POINT('Ctrl Pts',(-17.9340194463027,38.6253093543887,123.722198205263)) ;
#90978=CARTESIAN_POINT('Ctrl Pts',(-17.9027887073884,38.6352130079296,123.463801752552)) ;
#90979=CARTESIAN_POINT('Ctrl Pts',(-17.9163242119673,38.6451572769249,123.202860594878)) ;
#90980=CARTESIAN_POINT('Ctrl Pts',(-17.9947872688244,38.6584882852576,122.861360560677)) ;
#90981=CARTESIAN_POINT('Ctrl Pts',(-18.2021257874539,38.6751098657819,122.471340515978)) ;
#90982=CARTESIAN_POINT('Ctrl Pts',(-18.5280196716949,38.6916525364803,122.176175599121)) ;
#90983=CARTESIAN_POINT('Ctrl Pts',(-18.84008875281,38.7050016960432,122.015952826464)) ;
#90984=CARTESIAN_POINT('Ctrl Pts',(-19.1721179105993,38.7182298462027,121.912874830925)) ;
#90985=CARTESIAN_POINT('Ctrl Pts',(-19.6137093351474,38.7348605233402,121.89504706836)) ;
#90986=CARTESIAN_POINT('Ctrl Pts',(-20.1178745686584,38.7547634626283,122.055405875493)) ;
#90987=CARTESIAN_POINT('Ctrl Pts',(-20.5372564996866,38.7746663292316,122.377645054216)) ;
#90988=CARTESIAN_POINT('Ctrl Pts',(-20.8224486031123,38.7945794943364,122.823633412691)) ;
#90989=CARTESIAN_POINT('Ctrl Pts',(-20.9381893408,38.8146153234777,123.343346667635)) ;
#90990=CARTESIAN_POINT('Ctrl Pts',(-20.8706660685584,38.8344338983558,123.865874261203)) ;
#90991=CARTESIAN_POINT('Ctrl Pts',(-20.627922443163,38.8544041993978,124.337692899044)) ;
#90992=CARTESIAN_POINT('Ctrl Pts',(-20.2401234229137,38.8742957317623,124.69730681963)) ;
#90993=CARTESIAN_POINT('Ctrl Pts',(-19.7497967047093,38.8943188295789,124.903871868757)) ;
#90994=CARTESIAN_POINT('Ctrl Pts',(-19.2242573161077,38.9141155824988,124.930795625851)) ;
#90995=CARTESIAN_POINT('Ctrl Pts',(-18.7165907441389,38.9340766709876,124.776879006077)) ;
#90996=CARTESIAN_POINT('Ctrl Pts',(-18.2921488184441,38.9540549399198,124.457746589565)) ;
#90997=CARTESIAN_POINT('Ctrl Pts',(-18.0037947360342,38.9738749547108,124.016952429214)) ;
#90998=CARTESIAN_POINT('Ctrl Pts',(-17.8810979198861,38.9938133639626,123.501394794737)) ;
#90999=CARTESIAN_POINT('Ctrl Pts',(-17.9432262389664,39.013860481355,122.972141220867)) ;
#91000=CARTESIAN_POINT('Ctrl Pts',(-18.179999474083,39.0337067271889,122.500852961374)) ;
#91001=CARTESIAN_POINT('Ctrl Pts',(-18.5620692319856,39.0535556957009,122.137036795423)) ;
#91002=CARTESIAN_POINT('Ctrl Pts',(-19.0504584844477,39.0736059980122,121.923948334636)) ;
#91003=CARTESIAN_POINT('Ctrl Pts',(-19.5767211389698,39.0934409204434,121.8907738155)) ;
#91004=CARTESIAN_POINT('Ctrl Pts',(-20.0851205819504,39.1133713216693,122.038805273945)) ;
#91005=CARTESIAN_POINT('Ctrl Pts',(-20.5122385328754,39.1332562670282,122.350424357377)) ;
#91006=CARTESIAN_POINT('Ctrl Pts',(-20.8092718181263,39.1533288751795,122.793463019832)) ;
#91007=CARTESIAN_POINT('Ctrl Pts',(-20.9356236783323,39.1731201915077,123.304163853874)) ;
#91008=CARTESIAN_POINT('Ctrl Pts',(-20.8812715084831,39.1930849812749,123.831959781897)) ;
#91009=CARTESIAN_POINT('Ctrl Pts',(-20.6486431634336,39.2130679370252,124.309427208045)) ;
#91010=CARTESIAN_POINT('Ctrl Pts',(-20.2711039549004,39.2328764590014,124.676430038506)) ;
#91011=CARTESIAN_POINT('Ctrl Pts',(-19.7870902404589,39.2528620337372,124.894984520865)) ;
#91012=CARTESIAN_POINT('Ctrl Pts',(-19.2600307895484,39.2727446738056,124.934952427669)) ;
#91013=CARTESIAN_POINT('Ctrl Pts',(-18.7492190934437,39.2926999859375,124.792610565746)) ;
#91014=CARTESIAN_POINT('Ctrl Pts',(-18.3190388924115,39.3125743425453,124.485911249285)) ;
#91015=CARTESIAN_POINT('Ctrl Pts',(-18.0175162438669,39.3325565494064,124.048781584885)) ;
#91016=CARTESIAN_POINT('Ctrl Pts',(-17.8838364996547,39.3524876273563,123.536075517646)) ;
#91017=CARTESIAN_POINT('Ctrl Pts',(-17.9330377132969,39.3724146022113,123.008847051512)) ;
#91018=CARTESIAN_POINT('Ctrl Pts',(-18.1572602607085,39.3922470611602,122.531726093143)) ;
#91019=CARTESIAN_POINT('Ctrl Pts',(-18.4706715836701,39.4089047453354,122.219175253551)) ;
#91020=CARTESIAN_POINT('Ctrl Pts',(-18.7724853140679,39.4221539692425,122.045409139846)) ;
#91021=CARTESIAN_POINT('Ctrl Pts',(-19.0206746467771,39.4322029906937,121.95528639923)) ;
#91022=CARTESIAN_POINT('Ctrl Pts',(-19.2758714027625,39.4420629989242,121.910414373671)) ;
#91023=CARTESIAN_POINT('Ctrl Pts',(-19.6249850662901,39.4553465121488,121.909430053781)) ;
#91024=CARTESIAN_POINT('Ctrl Pts',(-20.0524695157253,39.4719924311496,122.023204765113)) ;
#91025=CARTESIAN_POINT('Ctrl Pts',(-20.4138864148045,39.4885464089657,122.274186137911)) ;
#91026=CARTESIAN_POINT('Ctrl Pts',(-20.6406300091737,39.5019061379373,122.542218010001)) ;
#91027=CARTESIAN_POINT('Ctrl Pts',(-20.7717096169385,39.511799189734,122.766754046185)) ;
#91028=CARTESIAN_POINT('Ctrl Pts',(-20.8630087660866,39.521789155015,123.012860662966)) ;
#91029=CARTESIAN_POINT('Ctrl Pts',(-20.9101748143691,39.5317410358759,123.270138684946)) ;
#91030=CARTESIAN_POINT('Ctrl Pts',(-20.9117456673708,39.5417893875677,123.534165997582)) ;
#91031=CARTESIAN_POINT('Ctrl Pts',(-20.8686552536552,39.5516306716739,123.789195920828)) ;
#91032=CARTESIAN_POINT('Ctrl Pts',(-20.7812002337361,39.5616173747996,124.036586790097)) ;
#91033=CARTESIAN_POINT('Ctrl Pts',(-20.6528795142412,39.571552403617,124.264016264375)) ;
#91034=CARTESIAN_POINT('Ctrl Pts',(-20.4848907700779,39.5816081985239,124.46795141361)) ;
#91035=CARTESIAN_POINT('Ctrl Pts',(-20.2887891671277,39.5914365618132,124.636091146284)) ;
#91036=CARTESIAN_POINT('Ctrl Pts',(-20.0614641234576,39.6014975317111,124.771025787529)) ;
#91037=CARTESIAN_POINT('Ctrl Pts',(-19.8176332037188,39.6114118106009,124.862898597772)) ;
#91038=CARTESIAN_POINT('Ctrl Pts',(-19.5592282819904,39.6214208050691,124.912002571716)) ;
#91039=CARTESIAN_POINT('Ctrl Pts',(-19.2956754516133,39.6314506396329,124.914961194742)) ;
#91040=CARTESIAN_POINT('Ctrl Pts',(-19.0399610301937,39.6413088697051,124.873328894269)) ;
#91041=CARTESIAN_POINT('Ctrl Pts',(-18.7918272427075,39.6513075754475,124.787030713098)) ;
#91042=CARTESIAN_POINT('Ctrl Pts',(-18.5646041239284,39.6612022313663,124.660518202869)) ;
#91043=CARTESIAN_POINT('Ctrl Pts',(-18.3594891226658,39.6712652957503,124.493676816178)) ;
#91044=CARTESIAN_POINT('Ctrl Pts',(-18.1900268540481,39.6811049540302,124.298315227073)) ;
#91045=CARTESIAN_POINT('Ctrl Pts',(-18.053792583236,39.691168121112,124.071699946612)) ;
#91046=CARTESIAN_POINT('Ctrl Pts',(-17.960749315,39.7010623662391,123.828876199066)) ;
#91047=CARTESIAN_POINT('Ctrl Pts',(-17.9103583441189,39.7110041878437,123.572554229599)) ;
#91048=CARTESIAN_POINT('Ctrl Pts',(-17.9051091078073,39.7210067187618,123.309715572966)) ;
#91049=CARTESIAN_POINT('Ctrl Pts',(-17.9461034213345,39.7310413452193,123.049236091637)) ;
#91050=CARTESIAN_POINT('Ctrl Pts',(-18.0297068679523,39.7408868802057,122.804375715976)) ;
#91051=CARTESIAN_POINT('Ctrl Pts',(-18.1557911659349,39.7508703050448,122.574330051635)) ;
#91052=CARTESIAN_POINT('Ctrl Pts',(-18.3194197366641,39.7608206954098,122.370358879002)) ;
#91053=CARTESIAN_POINT('Ctrl Pts',(-18.5166895154144,39.7708183357069,122.1968019572)) ;
#91054=CARTESIAN_POINT('Ctrl Pts',(-18.7422717110751,39.7808574162701,122.06004045278)) ;
#91055=CARTESIAN_POINT('Ctrl Pts',(-18.9827757053251,39.7906835670392,121.966001404595)) ;
#91056=CARTESIAN_POINT('Ctrl Pts',(-19.241779151991,39.8007401419683,121.913550884301)) ;
#91057=CARTESIAN_POINT('Ctrl Pts',(-19.5029424763994,39.8106806813486,121.907401203059)) ;
#91058=CARTESIAN_POINT('Ctrl Pts',(-19.7603853137432,39.820585074325,121.945742920367)) ;
#91059=CARTESIAN_POINT('Ctrl Pts',(-20.0107266937267,39.8306317285299,122.029537599121)) ;
#91060=CARTESIAN_POINT('Ctrl Pts',(-20.2393968682051,39.8405272904683,122.153454191526)) ;
#91061=CARTESIAN_POINT('Ctrl Pts',(-20.4464414983218,39.8505893683139,122.317864784386)) ;
#91062=CARTESIAN_POINT('Ctrl Pts',(-20.6181263774124,39.8604320667276,122.511365345899)) ;
#91063=CARTESIAN_POINT('Ctrl Pts',(-20.7561382322086,39.8704228416891,122.734672291079)) ;
#91064=CARTESIAN_POINT('Ctrl Pts',(-20.8526500680807,39.8803507067082,122.97707426249)) ;
#91065=CARTESIAN_POINT('Ctrl Pts',(-20.9063594910296,39.8903394514744,123.234019741878)) ;
#91066=CARTESIAN_POINT('Ctrl Pts',(-20.9142878541207,39.9003722370613,123.497555642552)) ;
#91067=CARTESIAN_POINT('Ctrl Pts',(-20.8772279525817,39.910238921682,123.754170693425)) ;
#91068=CARTESIAN_POINT('Ctrl Pts',(-20.7961043668712,39.9202008138451,124.003076881027)) ;
#91069=CARTESIAN_POINT('Ctrl Pts',(-20.6717493071348,39.9302342907577,124.2355665129)) ;
#91070=CARTESIAN_POINT('Ctrl Pts',(-20.5116325782537,39.940118632006,124.440138606861)) ;
#91071=CARTESIAN_POINT('Ctrl Pts',(-20.3149883606172,39.9501815741271,124.61689780952)) ;
#91072=CARTESIAN_POINT('Ctrl Pts',(-20.0953995131372,39.9600319757467,124.754007658767)) ;
#91073=CARTESIAN_POINT('Ctrl Pts',(-19.8513143447031,39.9700588645364,124.853250471539)) ;
#91074=CARTESIAN_POINT('Ctrl Pts',(-19.5934970141475,39.9800874794926,124.907943166141)) ;
#91075=CARTESIAN_POINT('Ctrl Pts',(-19.3349601607156,39.9899327026126,124.917361759063)) ;
#91076=CARTESIAN_POINT('Ctrl Pts',(-19.0748122096571,39.9999233864186,124.881915578707)) ;
#91077=CARTESIAN_POINT('Ctrl Pts',(-18.8237784515497,40.009961268491,124.800902625927)) ;
#91078=CARTESIAN_POINT('Ctrl Pts',(-18.5948964274932,40.0198056281299,124.68030432098)) ;
#91079=CARTESIAN_POINT('Ctrl Pts',(-18.3872328665451,40.0297904987446,124.519971576075)) ;
#91080=CARTESIAN_POINT('Ctrl Pts',(-18.2112308942488,40.0397297820733,124.326928042325)) ;
#91081=CARTESIAN_POINT('Ctrl Pts',(-18.0701011370966,40.0497703914464,124.10401924585)) ;
#91082=CARTESIAN_POINT('Ctrl Pts',(-17.9711747293191,40.0596552423596,123.863797270785)) ;
#91083=CARTESIAN_POINT('Ctrl Pts',(-17.914507891847,40.0696571985284,123.607177988291)) ;
#91084=CARTESIAN_POINT('Ctrl Pts',(-17.9031408318448,40.0795757952489,123.346733888948)) ;
#91085=CARTESIAN_POINT('Ctrl Pts',(-17.9376487606401,40.0896226173247,123.085016388873)) ;
#91086=CARTESIAN_POINT('Ctrl Pts',(-18.0155031495141,40.0994968984374,122.837438413162)) ;
#91087=CARTESIAN_POINT('Ctrl Pts',(-18.1371591486748,40.109551098482,122.602950598639)) ;
#91088=CARTESIAN_POINT('Ctrl Pts',(-18.2951196454476,40.1194465281173,122.396320882415)) ;
#91089=CARTESIAN_POINT('Ctrl Pts',(-18.4896702718675,40.1295081564346,122.217309891194)) ;
#91090=CARTESIAN_POINT('Ctrl Pts',(-18.7075627861497,40.1393527852645,122.077821066016)) ;
#91091=CARTESIAN_POINT('Ctrl Pts',(-18.9487886325186,40.1493128328701,121.976254285154)) ;
#91092=CARTESIAN_POINT('Ctrl Pts',(-19.2060965362213,40.1593511390442,121.918165822933)) ;
#91093=CARTESIAN_POINT('Ctrl Pts',(-19.4652798129029,40.1692244384768,121.905341126692)) ;
#91094=CARTESIAN_POINT('Ctrl Pts',(-19.7278620306309,40.1792977000631,121.938443177458)) ;
#91095=CARTESIAN_POINT('Ctrl Pts',(-19.9745652121543,40.1891179260198,122.014376604329)) ;
#91096=CARTESIAN_POINT('Ctrl Pts',(-20.210384152523,40.1991969899593,122.134825848413)) ;
#91097=CARTESIAN_POINT('Ctrl Pts',(-20.4170898719692,40.2090470799791,122.290751429487)) ;
#91098=CARTESIAN_POINT('Ctrl Pts',(-20.5976846428322,40.2191258335929,122.484401518764)) ;
#91099=CARTESIAN_POINT('Ctrl Pts',(-20.7384649199968,40.2289473008524,122.700793862279)) ;
#91100=CARTESIAN_POINT('Ctrl Pts',(-20.8423732928383,40.23901289921,122.943977873275)) ;
#91101=CARTESIAN_POINT('Ctrl Pts',(-20.9014655130511,40.2489155549847,123.197477874162)) ;
#91102=CARTESIAN_POINT('Ctrl Pts',(-20.9159315140315,40.2589663808143,123.461152741984)) ;
#91103=CARTESIAN_POINT('Ctrl Pts',(-20.8851862687562,40.2688405851532,123.718866407652)) ;
#91104=CARTESIAN_POINT('Ctrl Pts',(-20.8087033848994,40.2789130351923,123.972210529531)) ;
#91105=CARTESIAN_POINT('Ctrl Pts',(-20.6924508708633,40.2887420519658,124.202923123241)) ;
#91106=CARTESIAN_POINT('Ctrl Pts',(-20.534514449587,40.2988088978806,124.415095541138)) ;
#91107=CARTESIAN_POINT('Ctrl Pts',(-20.3453419288887,40.3086990691824,124.593367187674)) ;
#91108=CARTESIAN_POINT('Ctrl Pts',(-20.126206043176,40.3186912628062,124.738011905012)) ;
#91109=CARTESIAN_POINT('Ctrl Pts',(-19.8858849575961,40.3286540734297,124.841878589706)) ;
#91110=CARTESIAN_POINT('Ctrl Pts',(-19.6328023115127,40.3385583462731,124.902733214097)) ;
#91111=CARTESIAN_POINT('Ctrl Pts',(-19.368941004048,40.3486188380777,124.918739240953)) ;
#91112=CARTESIAN_POINT('Ctrl Pts',(-19.111948949925,40.3584591697501,124.889672424697)) ;
#91113=CARTESIAN_POINT('Ctrl Pts',(-18.8582728174585,40.3685222158418,124.815092864794)) ;
#91114=CARTESIAN_POINT('Ctrl Pts',(-18.6254185641157,40.3784162715369,124.699353388829)) ;
#91115=CARTESIAN_POINT('Ctrl Pts',(-18.414789936686,40.3883589718599,124.544790683395)) ;
#91116=CARTESIAN_POINT('Ctrl Pts',(-18.2329762001901,40.3983647127875,124.354801620633)) ;
#91117=CARTESIAN_POINT('Ctrl Pts',(-18.0869571139645,40.408385623303,124.135661151696)) ;
#91118=CARTESIAN_POINT('Ctrl Pts',(-17.982299068752,40.418276358753,123.897735676412)) ;
#91119=CARTESIAN_POINT('Ctrl Pts',(-17.9195403076832,40.4282678994818,123.64278976609)) ;
#91120=CARTESIAN_POINT('Ctrl Pts',(-17.9021523398952,40.4382157599035,123.381951195381)) ;
#91121=CARTESIAN_POINT('Ctrl Pts',(-17.9298041725074,40.4481624290898,123.122015017719)) ;
#91122=CARTESIAN_POINT('Ctrl Pts',(-18.0031779584756,40.4582105052254,122.868371382531)) ;
#91123=CARTESIAN_POINT('Ctrl Pts',(-18.1169687224454,40.468058103231,122.635944200235)) ;
#91124=CARTESIAN_POINT('Ctrl Pts',(-18.2704811318407,40.4780198263155,122.423910978732)) ;
#91125=CARTESIAN_POINT('Ctrl Pts',(-18.4599935581485,40.4880484613985,122.240750173216)) ;
#91126=CARTESIAN_POINT('Ctrl Pts',(-18.6757822343563,40.4979587697165,122.094962047602)) ;
#91127=CARTESIAN_POINT('Ctrl Pts',(-18.9139355025239,40.5078936668524,121.987961124184)) ;
#91128=CARTESIAN_POINT('Ctrl Pts',(-19.1697997287511,40.517934749795,121.923493244547)) ;
#91129=CARTESIAN_POINT('Ctrl Pts',(-19.428950366049,40.5278220926232,121.904543523959)) ;
#91130=CARTESIAN_POINT('Ctrl Pts',(-19.6901959445774,40.5378136075626,121.930704214457)) ;
#91131=CARTESIAN_POINT('Ctrl Pts',(-19.9419057770973,40.5477649987591,122.001654050665)) ;
#91132=CARTESIAN_POINT('Ctrl Pts',(-20.1772160470658,40.5576975320917,122.114605806638)) ;
#91133=CARTESIAN_POINT('Ctrl Pts',(-20.390773351119,40.5676946899911,122.267599496389)) ;
#91134=CARTESIAN_POINT('Ctrl Pts',(-20.5744051539528,40.5776797001546,122.455089020715)) ;
#91135=CARTESIAN_POINT('Ctrl Pts',(-20.723188468568,40.5877225267244,122.673023900318)) ;
#91136=CARTESIAN_POINT('Ctrl Pts',(-20.8301426365293,40.5975527610294,122.908217068064)) ;
#91137=CARTESIAN_POINT('Ctrl Pts',(-20.8963379142863,40.607628786264,123.164540306248)) ;
#91138=CARTESIAN_POINT('Ctrl Pts',(-20.9167055563444,40.6174810227549,123.422701150021)) ;
#91139=CARTESIAN_POINT('Ctrl Pts',(-20.891615051151,40.627554229189,123.686179366379)) ;
#91140=CARTESIAN_POINT('Ctrl Pts',(-20.8226924038434,40.6373957386962,123.935469529968)) ;
#91141=CARTESIAN_POINT('Ctrl Pts',(-20.7110845119955,40.647356685476,124.172237837628)) ;
#91142=CARTESIAN_POINT('Ctrl Pts',(-20.5584645897465,40.657394514276,124.387376516039)) ;
#91143=CARTESIAN_POINT('Ctrl Pts',(-20.3741751702042,40.6672688240305,124.570098190474)) ;
#91144=CARTESIAN_POINT('Ctrl Pts',(-20.1567868434197,40.6773385217037,124.720922673687)) ;
#91145=CARTESIAN_POINT('Ctrl Pts',(-19.9221561017423,40.6871719929911,124.829257549577)) ;
#91146=CARTESIAN_POINT('Ctrl Pts',(-19.6675134133936,40.697201639521,124.897250208865)) ;
#91147=CARTESIAN_POINT('Ctrl Pts',(-19.404726915787,40.7072361538484,124.919206335434)) ;
#91148=CARTESIAN_POINT('Ctrl Pts',(-19.1475426653616,40.7170614393193,124.896320551621)) ;
#91149=CARTESIAN_POINT('Ctrl Pts',(-18.8935848410147,40.7270656808678,124.828449926807)) ;
#91150=CARTESIAN_POINT('Ctrl Pts',(-18.6557571219536,40.7370483259469,124.717619979883)) ;
#91151=CARTESIAN_POINT('Ctrl Pts',(-18.4396753878514,40.7470935230384,124.566036174496)) ;
#91152=CARTESIAN_POINT('Ctrl Pts',(-18.2569837011254,40.7569166387985,124.383646814928)) ;
#91153=CARTESIAN_POINT('Ctrl Pts',(-18.1050079926846,40.7669512505988,124.168150561838)) ;
#91154=CARTESIAN_POINT('Ctrl Pts',(-17.9935267427077,40.776976259372,123.929445084339)) ;
#91155=CARTESIAN_POINT('Ctrl Pts',(-17.9258202753636,40.7868281842135,123.679551402899)) ;
#91156=CARTESIAN_POINT('Ctrl Pts',(-17.9018056354857,40.7968191225363,123.418132469691)) ;
#91157=CARTESIAN_POINT('Ctrl Pts',(-17.9232248951131,40.8067371076827,123.158348244679)) ;
#91158=CARTESIAN_POINT('Ctrl Pts',(-17.9900857838276,40.8167652085782,122.903464281987)) ;
#91159=CARTESIAN_POINT('Ctrl Pts',(-18.0985313024471,40.8266504495208,122.667402977687)) ;
#91160=CARTESIAN_POINT('Ctrl Pts',(-18.2473410925538,40.8366395624874,122.451144336104)) ;
#91161=CARTESIAN_POINT('Ctrl Pts',(-18.4328177933568,40.8466816268282,122.263433343905)) ;
#91162=CARTESIAN_POINT('Ctrl Pts',(-18.6432373021323,40.8565108282327,122.113605035665)) ;
#91163=CARTESIAN_POINT('Ctrl Pts',(-18.8804063338663,40.8665176689909,122.000080751744)) ;
#91164=CARTESIAN_POINT('Ctrl Pts',(-19.1333087574883,40.8765051931828,121.929728664348)) ;
#91165=CARTESIAN_POINT('Ctrl Pts',(-19.3956374933461,40.8865348389914,121.904438993338)) ;
#91166=CARTESIAN_POINT('Ctrl Pts',(-19.6543707145139,40.8964088697302,121.924454848222)) ;
#91167=CARTESIAN_POINT('Ctrl Pts',(-19.9089008937694,40.9064081925943,121.989579416378)) ;
#91168=CARTESIAN_POINT('Ctrl Pts',(-20.1463240582721,40.9163190281699,122.096753063302)) ;
#91169=CARTESIAN_POINT('Ctrl Pts',(-20.3645193729387,40.9263732761439,122.245676406375)) ;
#91170=CARTESIAN_POINT('Ctrl Pts',(-20.5501419901856,40.9362320204066,122.42647707007)) ;
#91171=CARTESIAN_POINT('Ctrl Pts',(-20.7048457015326,40.9463001064796,122.641065679255)) ;
#91172=CARTESIAN_POINT('Ctrl Pts',(-20.8175173641889,40.9561555896591,122.874289210237)) ;
#91173=CARTESIAN_POINT('Ctrl Pts',(-20.8897275055665,40.9661504354533,123.126813177261)) ;
#91174=CARTESIAN_POINT('Ctrl Pts',(-20.9165302141604,40.9761817311159,123.389064120819)) ;
#91175=CARTESIAN_POINT('Ctrl Pts',(-20.898116848103,40.9860482744057,123.647700931821)) ;
#91176=CARTESIAN_POINT('Ctrl Pts',(-20.8347236238339,40.9960356701691,123.902356200774)) ;
#91177=CARTESIAN_POINT('Ctrl Pts',(-20.7286285702455,41.0059807108991,124.141239921477)) ;
#91178=CARTESIAN_POINT('Ctrl Pts',(-20.5811211598771,41.0160252171158,124.360105227099)) ;
#91179=CARTESIAN_POINT('Ctrl Pts',(-20.4012876880261,41.0258887232531,124.546811663943)) ;
#91180=CARTESIAN_POINT('Ctrl Pts',(-20.1893463018213,41.0358815840892,124.701796997942)) ;
#91181=CARTESIAN_POINT('Ctrl Pts',(-19.9552720707621,41.0458077778081,124.816998522553)) ;
#91182=CARTESIAN_POINT('Ctrl Pts',(-19.7024899327944,41.0558267038407,124.890516309692)) ;
#91183=CARTESIAN_POINT('Ctrl Pts',(-19.4434540809893,41.0657417032083,124.918982353563)) ;
#91184=CARTESIAN_POINT('Ctrl Pts',(-19.179821038914,41.0757964747656,124.901749795245)) ;
#91185=CARTESIAN_POINT('Ctrl Pts',(-18.9280800412219,41.0856554370632,124.840372296681)) ;
#91186=CARTESIAN_POINT('Ctrl Pts',(-18.6874351062413,41.095649680901,124.735268941808)) ;
#91187=CARTESIAN_POINT('Ctrl Pts',(-18.4700684891871,41.1055749103252,124.591037888929)) ;
#91188=CARTESIAN_POINT('Ctrl Pts',(-18.2791378076578,41.1156028742167,124.409455504001)) ;
#91189=CARTESIAN_POINT('Ctrl Pts',(-18.1245883806122,41.1254891338471,124.20057485489)) ;
#91190=CARTESIAN_POINT('Ctrl Pts',(-18.0068635292268,41.1355208969249,123.964745548738)) ;
#91191=CARTESIAN_POINT('Ctrl Pts',(-17.9327293076382,41.1454025232191,123.715825423128)) ;
#91192=CARTESIAN_POINT('Ctrl Pts',(-17.9023394171472,41.1554642927052,123.453203976772)) ;
#91193=CARTESIAN_POINT('Ctrl Pts',(-17.9176211064176,41.1653221602007,123.194569188612)) ;
#91194=CARTESIAN_POINT('Ctrl Pts',(-17.9778112462982,41.1753137853181,122.939023648064)) ;
#91195=CARTESIAN_POINT('Ctrl Pts',(-18.0809522301768,41.1852505844263,122.699110258918)) ;
#91196=CARTESIAN_POINT('Ctrl Pts',(-18.2246372961258,41.1952414139836,122.479365383899)) ;
#91197=CARTESIAN_POINT('Ctrl Pts',(-18.4051031632681,41.2052646496968,122.287492545493)) ;
#91198=CARTESIAN_POINT('Ctrl Pts',(-18.6133310445568,41.215160997726,122.131695698258)) ;
#91199=CARTESIAN_POINT('Ctrl Pts',(-18.8473975521708,41.2251505602285,122.012807543813)) ;
#91200=CARTESIAN_POINT('Ctrl Pts',(-19.0999569107167,41.235190867913,121.936495551711)) ;
#91201=CARTESIAN_POINT('Ctrl Pts',(-19.35673862267,41.2450331712602,121.905316610654)) ;
#91202=CARTESIAN_POINT('Ctrl Pts',(-19.619750139844,41.2550568795393,121.919098001981)) ;
#91203=CARTESIAN_POINT('Ctrl Pts',(-19.9583979422888,41.268279057007,121.997129854709)) ;
#91204=CARTESIAN_POINT('Ctrl Pts',(-20.2706317559911,41.2815716420663,122.162222495001)) ;
#91205=CARTESIAN_POINT('Ctrl Pts',(-20.5265422578919,41.2948564979879,122.399798532575)) ;
#91206=CARTESIAN_POINT('Ctrl Pts',(-20.6848531440753,41.3048287251607,122.608586988607)) ;
#91207=CARTESIAN_POINT('Ctrl Pts',(-20.8041778753836,41.3147373415997,122.840061396327)) ;
#91208=CARTESIAN_POINT('Ctrl Pts',(-20.8825078353512,41.3247905469834,123.092342498857)) ;
#91209=CARTESIAN_POINT('Ctrl Pts',(-20.9153911019207,41.3346556807437,123.349517175633)) ;
#91210=CARTESIAN_POINT('Ctrl Pts',(-20.8994532016943,41.34799473837,123.699671410169)) ;
#91211=CARTESIAN_POINT('Ctrl Pts',(-20.7662682588357,41.3645639257032,124.119498420051)) ;
#91212=CARTESIAN_POINT('Ctrl Pts',(-20.4969289351474,41.3812090655542,124.470369460942)) ;
#91213=CARTESIAN_POINT('Ctrl Pts',(-20.2201112015402,41.3944813680276,124.682651973969)) ;
#91214=CARTESIAN_POINT('Ctrl Pts',(-19.9875982884763,41.4044623314752,124.803972762843)) ;
#91215=CARTESIAN_POINT('Ctrl Pts',(-19.738528944689,41.4144041635445,124.882935891262)) ;
#91216=CARTESIAN_POINT('Ctrl Pts',(-19.3916330563447,41.42772373276,124.929305565793)) ;
#91217=CARTESIAN_POINT('Ctrl Pts',(-18.9557211738586,41.4442538876927,124.873625074331)) ;
#91218=CARTESIAN_POINT('Ctrl Pts',(-18.4827898293542,41.4642756131848,124.629964635199)) ;
#91219=CARTESIAN_POINT('Ctrl Pts',(-18.1247913754587,41.4840870097916,124.243659355812)) ;
#91220=CARTESIAN_POINT('Ctrl Pts',(-17.9175945300158,41.5040722585005,123.754695417451)) ;
#91221=CARTESIAN_POINT('Ctrl Pts',(-17.8901702572938,41.5239663211364,123.226570828249)) ;
#91222=CARTESIAN_POINT('Ctrl Pts',(-18.0441233573117,41.54389800031,122.719693569398)) ;
#91223=CARTESIAN_POINT('Ctrl Pts',(-18.3626064665209,41.563862054782,122.295289089254)) ;
#91224=CARTESIAN_POINT('Ctrl Pts',(-18.8047488016914,41.5837429565449,122.005904879941)) ;
#91225=CARTESIAN_POINT('Ctrl Pts',(-19.320432669292,41.6036816181533,121.883949466073)) ;
#91226=CARTESIAN_POINT('Ctrl Pts',(-19.845694207807,41.6235781434086,121.945081447372)) ;
#91227=CARTESIAN_POINT('Ctrl Pts',(-20.3189427672172,41.6434731818629,122.181005425179)) ;
#91228=CARTESIAN_POINT('Ctrl Pts',(-20.6844409401465,41.663437005169,122.565598444425)) ;
#91229=CARTESIAN_POINT('Ctrl Pts',(-20.8961948389639,41.6833111292981,123.049559754929)) ;
#91230=CARTESIAN_POINT('Ctrl Pts',(-20.930750337764,41.7032862050253,123.5793623284)) ;
#91231=CARTESIAN_POINT('Ctrl Pts',(-20.7818779747331,41.7232397743819,124.088362609543)) ;
#91232=CARTESIAN_POINT('Ctrl Pts',(-20.4708653827436,41.7430776845698,124.514126207426)) ;
#91233=CARTESIAN_POINT('Ctrl Pts',(-20.0305044149458,41.7630535131407,124.810712363069)) ;
#91234=CARTESIAN_POINT('Ctrl Pts',(-19.5167523633582,41.782971557851,124.938278605792)) ;
#91235=CARTESIAN_POINT('Ctrl Pts',(-18.9912886178478,41.8028418036386,124.884326486846)) ;
#91236=CARTESIAN_POINT('Ctrl Pts',(-18.5120647055615,41.8228908067382,124.651624297318)) ;
#91237=CARTESIAN_POINT('Ctrl Pts',(-18.1453880278503,41.842670047979,124.274702004828)) ;
#91238=CARTESIAN_POINT('Ctrl Pts',(-17.9259851440591,41.8627001116879,123.789780611659)) ;
#91239=CARTESIAN_POINT('Ctrl Pts',(-17.8863697134436,41.8825823965899,123.262746959437)) ;
#91240=CARTESIAN_POINT('Ctrl Pts',(-18.0275326386484,41.9024646974829,122.753560552606)) ;
#91241=CARTESIAN_POINT('Ctrl Pts',(-18.3357088896958,41.9224478071012,122.320980688982)) ;
#91242=CARTESIAN_POINT('Ctrl Pts',(-18.7710306130654,41.9423382024791,122.02096992026)) ;
#91243=CARTESIAN_POINT('Ctrl Pts',(-19.2824613005974,41.9622349925134,121.886735352838)) ;
#91244=CARTESIAN_POINT('Ctrl Pts',(-19.8096884308124,41.982152046455,121.934563073507)) ;
#91245=CARTESIAN_POINT('Ctrl Pts',(-20.2909909356095,42.0021555946585,122.16058890975)) ;
#91246=CARTESIAN_POINT('Ctrl Pts',(-20.6644231854792,42.0220938883111,122.53654694601)) ;
#91247=CARTESIAN_POINT('Ctrl Pts',(-20.8870221312374,42.041915375744,123.014039318309)) ;
#91248=CARTESIAN_POINT('Ctrl Pts',(-20.9342135131919,42.0618937687349,123.542870872687)) ;
#91249=CARTESIAN_POINT('Ctrl Pts',(-20.7983116521925,42.0817921503486,124.05406099751)) ;
#91250=CARTESIAN_POINT('Ctrl Pts',(-20.5470876259133,42.0983750810785,124.416078628644)) ;
#91251=CARTESIAN_POINT('Ctrl Pts',(-20.2810340791425,42.1116493166673,124.641785333089)) ;
#91252=CARTESIAN_POINT('Ctrl Pts',(-20.0530711216127,42.1216957341235,124.774894284612)) ;
#91253=CARTESIAN_POINT('Ctrl Pts',(-19.8104700418555,42.1315409593428,124.864850290018)) ;
#91254=CARTESIAN_POINT('Ctrl Pts',(-19.4658985569829,42.1448759303822,124.928521275722)) ;
#91255=CARTESIAN_POINT('Ctrl Pts',(-19.0264447066916,42.1614587871748,124.893669283051)) ;
#91256=CARTESIAN_POINT('Ctrl Pts',(-18.6239261419113,42.1781017895242,124.710472536037)) ;
#91257=CARTESIAN_POINT('Ctrl Pts',(-18.3550087789404,42.1913455205559,124.489421557899)) ;
#91258=CARTESIAN_POINT('Ctrl Pts',(-18.1831612885463,42.2013999152305,124.288789628079)) ;
#91259=CARTESIAN_POINT('Ctrl Pts',(-18.0512749568523,42.2112409766191,124.066279127092)) ;
#91260=CARTESIAN_POINT('Ctrl Pts',(-17.9577303156056,42.2213072009756,123.818889092396)) ;
#91261=CARTESIAN_POINT('Ctrl Pts',(-17.9095286836072,42.2311878138952,123.563707583519)) ;
#91262=CARTESIAN_POINT('Ctrl Pts',(-17.9058337757334,42.2411811070548,123.301162738247)) ;
#91263=CARTESIAN_POINT('Ctrl Pts',(-17.9475195177784,42.2511321152785,123.042958068114)) ;
#91264=CARTESIAN_POINT('Ctrl Pts',(-18.0344126776209,42.2611806296404,122.793630948039)) ;
#91265=CARTESIAN_POINT('Ctrl Pts',(-18.1603920215042,42.2710221357031,122.56773601956)) ;
#91266=CARTESIAN_POINT('Ctrl Pts',(-18.3255845008848,42.2810077883328,122.363897258987)) ;
#91267=CARTESIAN_POINT('Ctrl Pts',(-18.5227313519484,42.2909467971777,122.192513006054)) ;
#91268=CARTESIAN_POINT('Ctrl Pts',(-18.7489176532003,42.3009877224707,122.056676120919)) ;
#91269=CARTESIAN_POINT('Ctrl Pts',(-18.9915477533087,42.3108780442256,121.96343274295)) ;
#91270=CARTESIAN_POINT('Ctrl Pts',(-19.2492897392915,42.320874017559,121.912831427002)) ;
#91271=CARTESIAN_POINT('Ctrl Pts',(-19.510238542724,42.3308054171411,121.90776329539)) ;
#91272=CARTESIAN_POINT('Ctrl Pts',(-19.7700878324599,42.3408109576181,121.948013744856)) ;
#91273=CARTESIAN_POINT('Ctrl Pts',(-20.0195067969403,42.3508439415494,122.033453514433)) ;
#91274=CARTESIAN_POINT('Ctrl Pts',(-20.2464693982846,42.3606995723763,122.158262805078)) ;
#91275=CARTESIAN_POINT('Ctrl Pts',(-20.4514198298294,42.3706989745694,122.322645616245)) ;
#91276=CARTESIAN_POINT('Ctrl Pts',(-20.6231827987995,42.3805934439305,122.517917638285)) ;
#91277=CARTESIAN_POINT('Ctrl Pts',(-20.7606195436203,42.3906565580947,122.743793366782)) ;
#91278=CARTESIAN_POINT('Ctrl Pts',(-20.8549120164977,42.4004962038111,122.984609559958)) ;
#91279=CARTESIAN_POINT('Ctrl Pts',(-20.9074321966083,42.4105593713669,123.243754099235)) ;
#91280=CARTESIAN_POINT('Ctrl Pts',(-20.9138270218801,42.4204536271617,123.503714919927)) ;
#91281=CARTESIAN_POINT('Ctrl Pts',(-20.8755128410189,42.4303954056214,123.762117252756)) ;
#91282=CARTESIAN_POINT('Ctrl Pts',(-20.7924756140901,42.4403980984516,124.011553585451)) ;
#91283=CARTESIAN_POINT('Ctrl Pts',(-20.6666672130897,42.4504321204054,124.243274149404)) ;
#91284=CARTESIAN_POINT('Ctrl Pts',(-20.5058796969663,42.4602799114944,124.446064360107)) ;
#91285=CARTESIAN_POINT('Ctrl Pts',(-20.3101026092512,42.4702614360435,124.62060077918)) ;
#91286=CARTESIAN_POINT('Ctrl Pts',(-20.0876687178098,42.4802106595344,124.758029297087)) ;
#91287=CARTESIAN_POINT('Ctrl Pts',(-19.8436792195384,42.490208315751,124.855531589647)) ;
#91288=CARTESIAN_POINT('Ctrl Pts',(-19.5853068270162,42.500248528806,124.908912389975)) ;
#91289=CARTESIAN_POINT('Ctrl Pts',(-19.3271481560831,42.5100765760823,124.917023207503)) ;
#91290=CARTESIAN_POINT('Ctrl Pts',(-19.065587620381,42.5201309231147,124.879749670527)) ;
#91291=CARTESIAN_POINT('Ctrl Pts',(-18.8174156782774,42.5300720594432,124.798125360101)) ;
#91292=CARTESIAN_POINT('Ctrl Pts',(-18.5876622498009,42.5399762925229,124.675821006536)) ;
#91293=CARTESIAN_POINT('Ctrl Pts',(-18.3798098223478,42.5500229893665,124.513062959193)) ;
#91294=CARTESIAN_POINT('Ctrl Pts',(-18.205809991047,42.5599185406468,124.319751471792)) ;
#91295=CARTESIAN_POINT('Ctrl Pts',(-18.0657424005529,42.5699806184863,124.095520805029)) ;
#91296=CARTESIAN_POINT('Ctrl Pts',(-17.9687323982393,42.5798233275824,123.855713961264)) ;
#91297=CARTESIAN_POINT('Ctrl Pts',(-17.9134293922222,42.5898140598208,123.599092869816)) ;
#91298=CARTESIAN_POINT('Ctrl Pts',(-17.9036266135817,42.5997420850496,123.338364905447)) ;
#91299=CARTESIAN_POINT('Ctrl Pts',(-17.9390160350888,42.6097302317001,123.078277461847)) ;
#91300=CARTESIAN_POINT('Ctrl Pts',(-18.0197861525379,42.6197652495401,122.827237976155)) ;
#91301=CARTESIAN_POINT('Ctrl Pts',(-18.140582591483,42.6296300466453,122.597876275323)) ;
#91302=CARTESIAN_POINT('Ctrl Pts',(-18.3003156640756,42.6395907790014,122.390498248251)) ;
#91303=CARTESIAN_POINT('Ctrl Pts',(-18.4953259743341,42.6496242413984,122.213054154998)) ;
#91304=CARTESIAN_POINT('Ctrl Pts',(-18.7147012146566,42.6595097756098,122.073852925735)) ;
#91305=CARTESIAN_POINT('Ctrl Pts',(-18.9592157983849,42.6695746162898,121.973094770652)) ;
#91306=CARTESIAN_POINT('Ctrl Pts',(-19.211976927808,42.6794227480187,121.917420334612)) ;
#91307=CARTESIAN_POINT('Ctrl Pts',(-19.4752162394926,42.6894502450088,121.905599515675)) ;
#91308=CARTESIAN_POINT('Ctrl Pts',(-19.7364643783176,42.6994786970539,121.940363154748)) ;
#91309=CARTESIAN_POINT('Ctrl Pts',(-19.983240895575,42.709323963618,122.018027966902)) ;
#91310=CARTESIAN_POINT('Ctrl Pts',(-20.2165165477863,42.7193146365589,122.138509322655)) ;
#91311=CARTESIAN_POINT('Ctrl Pts',(-20.42595149829,42.7293525186474,122.298877797518)) ;
#91312=CARTESIAN_POINT('Ctrl Pts',(-20.6012619502332,42.739196889087,122.489133616188)) ;
#91313=CARTESIAN_POINT('Ctrl Pts',(-20.7432777778674,42.7491817164824,122.709727782596)) ;
#91314=CARTESIAN_POINT('Ctrl Pts',(-20.8445084625415,42.7591211618877,122.950553007713)) ;
#91315=CARTESIAN_POINT('Ctrl Pts',(-20.902884175201,42.7691611661736,123.207827740318)) ;
#91316=CARTESIAN_POINT('Ctrl Pts',(-20.9156867364475,42.7790482753592,123.467365079687)) ;
#91317=CARTESIAN_POINT('Ctrl Pts',(-20.8831915581267,42.7890483352617,123.728098704159)) ;
#91318=CARTESIAN_POINT('Ctrl Pts',(-20.8067445599132,42.7989657511764,123.977299323762)) ;
#91319=CARTESIAN_POINT('Ctrl Pts',(-20.686612406926,42.8090125659172,124.212363180922)) ;
#91320=CARTESIAN_POINT('Ctrl Pts',(-20.5303690658562,42.8188880431139,124.419630089936)) ;
#91321=CARTESIAN_POINT('Ctrl Pts',(-20.337202917031,42.8289441388351,124.599902985176)) ;
#91322=CARTESIAN_POINT('Ctrl Pts',(-20.1192329290402,42.8388373008502,124.741697871364)) ;
#91323=CARTESIAN_POINT('Ctrl Pts',(-19.8759728300273,42.8488995368728,124.845270931614)) ;
#91324=CARTESIAN_POINT('Ctrl Pts',(-19.6239615863206,42.8587440025017,124.903774649878)) ;
#91325=CARTESIAN_POINT('Ctrl Pts',(-19.3626527477167,42.8687040952058,124.91873716026)) ;
#91326=CARTESIAN_POINT('Ctrl Pts',(-19.1007442432168,42.8787423841869,124.887345479684)) ;
#91327=CARTESIAN_POINT('Ctrl Pts',(-18.852219395114,42.8886157072931,124.812672988231)) ;
#91328=CARTESIAN_POINT('Ctrl Pts',(-18.6158652448163,42.8986888913782,124.693587821864)) ;
#91329=CARTESIAN_POINT('Ctrl Pts',(-18.408809846254,42.9085094036661,124.539447907291)) ;
#91330=CARTESIAN_POINT('Ctrl Pts',(-18.2269164681603,42.9185873997819,124.347038540938)) ;
#91331=CARTESIAN_POINT('Ctrl Pts',(-18.0843140642102,42.9284414747652,124.130813462835)) ;
#91332=CARTESIAN_POINT('Ctrl Pts',(-17.9790106190544,42.9385053563489,123.888269164773)) ;
#91333=CARTESIAN_POINT('Ctrl Pts',(-17.9185491680014,42.9483887823227,123.635632007947)) ;
#91334=CARTESIAN_POINT('Ctrl Pts',(-17.9022737750403,42.9583893862437,123.373377146627)) ;
#91335=CARTESIAN_POINT('Ctrl Pts',(-17.9313895259165,42.9683091705816,123.114278441424)) ;
#91336=CARTESIAN_POINT('Ctrl Pts',(-18.0060320164047,42.9783565209384,122.861060709944)) ;
#91337=CARTESIAN_POINT('Ctrl Pts',(-18.1212870190588,42.9882338631727,122.628427841327)) ;
#91338=CARTESIAN_POINT('Ctrl Pts',(-18.2781351229889,42.9983037442474,122.415360927794)) ;
#91339=CARTESIAN_POINT('Ctrl Pts',(-18.4649150055318,43.008133449449,122.2368543242)) ;
#91340=CARTESIAN_POINT('Ctrl Pts',(-18.6847596765535,43.0182001106154,122.089792158768)) ;
#91341=CARTESIAN_POINT('Ctrl Pts',(-18.9226931773935,43.0280903324827,121.985125306975)) ;
#91342=CARTESIAN_POINT('Ctrl Pts',(-19.1776048761138,43.0380825085929,121.922176627254)) ;
#91343=CARTESIAN_POINT('Ctrl Pts',(-19.4388303799402,43.0480453387055,121.904745061404)) ;
#91344=CARTESIAN_POINT('Ctrl Pts',(-19.697682792419,43.0579495511058,121.932114404861)) ;
#91345=CARTESIAN_POINT('Ctrl Pts',(-19.951683312586,43.0680102651937,122.005359612903)) ;
#91346=CARTESIAN_POINT('Ctrl Pts',(-20.1841105631504,43.0778497681765,122.118753970002)) ;
#91347=CARTESIAN_POINT('Ctrl Pts',(-20.3982269814349,43.0879159067429,122.274016136349)) ;
#91348=CARTESIAN_POINT('Ctrl Pts',(-20.5787646114016,43.0977984212289,122.460756397599)) ;
#91349=CARTESIAN_POINT('Ctrl Pts',(-20.7261333194938,43.1077907205845,122.678042925821)) ;
#91350=CARTESIAN_POINT('Ctrl Pts',(-20.833206366185,43.1177437875379,122.916721805344)) ;
#91351=CARTESIAN_POINT('Ctrl Pts',(-20.897614117175,43.1277784957431,123.172416207021)) ;
#91352=CARTESIAN_POINT('Ctrl Pts',(-20.9165610195701,43.1376667166473,123.43159275742)) ;
#91353=CARTESIAN_POINT('Ctrl Pts',(-20.8903677843384,43.1476611396777,123.692911928234)) ;
#91354=CARTESIAN_POINT('Ctrl Pts',(-20.8194444690435,43.1576064791239,123.944458675462)) ;
#91355=CARTESIAN_POINT('Ctrl Pts',(-20.7063781227187,43.1675538237352,124.180161559428)) ;
#91356=CARTESIAN_POINT('Ctrl Pts',(-20.5523346077461,43.1776017191462,124.394608128497)) ;
#91357=CARTESIAN_POINT('Ctrl Pts',(-20.3673072274807,43.1874493646256,124.575539263631)) ;
#91358=CARTESIAN_POINT('Ctrl Pts',(-20.1516760965307,43.1974110785396,124.723955111939)) ;
#91359=CARTESIAN_POINT('Ctrl Pts',(-19.9117864879595,43.2074397028305,124.833114513842)) ;
#91360=CARTESIAN_POINT('Ctrl Pts',(-19.6596450451628,43.2173500634872,124.898260239512)) ;
#91361=CARTESIAN_POINT('Ctrl Pts',(-19.3994169455173,43.2272847620605,124.919374953537)) ;
#91362=CARTESIAN_POINT('Ctrl Pts',(-19.1367199893783,43.2373265869147,124.894463864514)) ;
#91363=CARTESIAN_POINT('Ctrl Pts',(-18.886225085537,43.2472111606591,124.825627198555)) ;
#91364=CARTESIAN_POINT('Ctrl Pts',(-18.6486227140851,43.2572130100223,124.713331619215)) ;
#91365=CARTESIAN_POINT('Ctrl Pts',(-18.4357298701924,43.2671323115963,124.562855492148)) ;
#91366=CARTESIAN_POINT('Ctrl Pts',(-18.2499252216547,43.2771764199416,124.375414816484)) ;
#91367=CARTESIAN_POINT('Ctrl Pts',(-18.1017967666107,43.2870608433839,124.162024125329)) ;
#91368=CARTESIAN_POINT('Ctrl Pts',(-17.9909876140739,43.2970772052933,123.923254596581)) ;
#91369=CARTESIAN_POINT('Ctrl Pts',(-17.923859840719,43.3071138607987,123.668202194077)) ;
#91370=CARTESIAN_POINT('Ctrl Pts',(-17.9017809512743,43.316943990988,123.410789908408)) ;
#91371=CARTESIAN_POINT('Ctrl Pts',(-17.9252094807461,43.3270200440779,123.14709156434)) ;
#91372=CARTESIAN_POINT('Ctrl Pts',(-17.9924299188192,43.3368722732637,122.897006470178)) ;
#91373=CARTESIAN_POINT('Ctrl Pts',(-18.1042679823455,43.346945481063,122.657125718903)) ;
#91374=CARTESIAN_POINT('Ctrl Pts',(-18.2526600247285,43.3567869924144,122.445286955059)) ;
#91375=CARTESIAN_POINT('Ctrl Pts',(-18.4370833480714,43.3667479304519,122.259535607649)) ;
#91376=CARTESIAN_POINT('Ctrl Pts',(-18.6529137116503,43.3767857923769,122.107894632329)) ;
#91377=CARTESIAN_POINT('Ctrl Pts',(-18.8877318802292,43.386659978374,121.997399835187)) ;
#91378=CARTESIAN_POINT('Ctrl Pts',(-19.1430767424442,43.3967301379519,121.928047356041)) ;
#91379=CARTESIAN_POINT('Ctrl Pts',(-19.4003939023348,43.4065618853777,121.904482946936)) ;
#91380=CARTESIAN_POINT('Ctrl Pts',(-19.6632619536359,43.416597965449,121.925714449018)) ;
#91381=CARTESIAN_POINT('Ctrl Pts',(-19.9178244791952,43.4266150123015,121.992789588399)) ;
#91382=CARTESIAN_POINT('Ctrl Pts',(-20.1538536760543,43.4364972704681,122.101114447307)) ;
#91383=CARTESIAN_POINT('Ctrl Pts',(-20.3699131764678,43.4464849532645,122.250085365114)) ;
#91384=CARTESIAN_POINT('Ctrl Pts',(-20.5562534234135,43.4564316099812,122.433448480984)) ;
#91385=CARTESIAN_POINT('Ctrl Pts',(-20.7093464656126,43.4664886680613,122.648845014339)) ;
#91386=CARTESIAN_POINT('Ctrl Pts',(-20.8203630654668,43.4763068476108,122.881767028925)) ;
#91387=CARTESIAN_POINT('Ctrl Pts',(-20.8914610512173,43.4863427820498,123.135729585425)) ;
#91388=CARTESIAN_POINT('Ctrl Pts',(-20.9166029199042,43.4963674364788,123.397974203455)) ;
#91389=CARTESIAN_POINT('Ctrl Pts',(-20.8967578932332,43.5062194560583,123.656117782256)) ;
#91390=CARTESIAN_POINT('Ctrl Pts',(-20.831881508292,43.5162103697732,123.910494310723)) ;
#91391=CARTESIAN_POINT('Ctrl Pts',(-20.7247399963963,43.5261283586128,124.148122891889)) ;
#91392=CARTESIAN_POINT('Ctrl Pts',(-20.5764179652717,43.5361564693436,124.365922998669)) ;
#91393=CARTESIAN_POINT('Ctrl Pts',(-20.3952122093275,43.546041667252,124.552066450949)) ;
#91394=CARTESIAN_POINT('Ctrl Pts',(-20.1825938294097,43.55603094252,124.706038954203)) ;
#91395=CARTESIAN_POINT('Ctrl Pts',(-19.9449996926765,43.5660724006895,124.820834858962)) ;
#91396=CARTESIAN_POINT('Ctrl Pts',(-19.6965069343808,43.5759038644778,124.89159240592)) ;
#91397=CARTESIAN_POINT('Ctrl Pts',(-19.4350698137697,43.5859087967817,124.919173839307)) ;
#91398=CARTESIAN_POINT('Ctrl Pts',(-19.1732351295058,43.5958951606764,124.900827612683)) ;
#91399=CARTESIAN_POINT('Ctrl Pts',(-18.9175770787377,43.6059247895623,124.836838031948)) ;
#91400=CARTESIAN_POINT('Ctrl Pts',(-18.6804371598066,43.6158000116707,124.731369996855)) ;
#91401=CARTESIAN_POINT('Ctrl Pts',(-18.4623477415022,43.6258012240678,124.584774106996)) ;
#91402=CARTESIAN_POINT('Ctrl Pts',(-18.2745444168899,43.6357098033033,124.404343207406)) ;
#91403=CARTESIAN_POINT('Ctrl Pts',(-18.1187722259552,43.6457646558593,124.190964881095)) ;
#91404=CARTESIAN_POINT('Ctrl Pts',(-18.004380821327,43.6556232381341,123.958462580893)) ;
#91405=CARTESIAN_POINT('Ctrl Pts',(-17.9304301319305,43.6656913675768,123.704467954817)) ;
#91406=CARTESIAN_POINT('Ctrl Pts',(-17.9023257120292,43.6755468392659,123.446983659363)) ;
#91407=CARTESIAN_POINT('Ctrl Pts',(-17.9188088681527,43.6855416876521,123.18485588981)) ;
#91408=CARTESIAN_POINT('Ctrl Pts',(-17.9813360998204,43.6955729844366,122.928761468334)) ;
#91409=CARTESIAN_POINT('Ctrl Pts',(-18.0852611565216,43.7054395206467,122.691208548975)) ;
#91410=CARTESIAN_POINT('Ctrl Pts',(-18.2302389701534,43.7154269436075,122.472461402679)) ;
#91411=CARTESIAN_POINT('Ctrl Pts',(-18.4101746479847,43.7253718826273,122.282878179321)) ;
#91412=CARTESIAN_POINT('Ctrl Pts',(-18.6224381752842,43.7354167684873,122.125988815331)) ;
#91413=CARTESIAN_POINT('Ctrl Pts',(-18.8545304610227,43.7452853035735,122.010266829846)) ;
#91414=CARTESIAN_POINT('Ctrl Pts',(-19.1054170228572,43.7552511715802,121.935180988231)) ;
#91415=CARTESIAN_POINT('Ctrl Pts',(-19.3670753403128,43.7652738190327,121.904915997745)) ;
#91416=CARTESIAN_POINT('Ctrl Pts',(-19.6273895696262,43.7751974580403,121.920314786866)) ;
#91417=CARTESIAN_POINT('Ctrl Pts',(-19.8817360875412,43.785140183046,121.980191368914)) ;
#91418=CARTESIAN_POINT('Ctrl Pts',(-20.1241540955357,43.7951857890979,122.084667591629)) ;
#91419=CARTESIAN_POINT('Ctrl Pts',(-20.3408919295591,43.805047211619,122.226772581987)) ;
#91420=CARTESIAN_POINT('Ctrl Pts',(-20.5324564346371,43.8150407800682,122.406363357882)) ;
#91421=CARTESIAN_POINT('Ctrl Pts',(-20.6890092975618,43.8249662508235,122.615035530979)) ;
#91422=CARTESIAN_POINT('Ctrl Pts',(-20.8081450016785,43.8349939247794,122.850047539463)) ;
#91423=CARTESIAN_POINT('Ctrl Pts',(-20.8838536120231,43.8448811028211,123.098633773252)) ;
#91424=CARTESIAN_POINT('Ctrl Pts',(-20.9158727010176,43.8549094821892,123.360180929265)) ;
#91425=CARTESIAN_POINT('Ctrl Pts',(-20.9023154130468,43.8648037249107,123.61987110098)) ;
#91426=CARTESIAN_POINT('Ctrl Pts',(-20.8237526627658,43.8781566415616,123.961832644244)) ;
#91427=CARTESIAN_POINT('Ctrl Pts',(-20.659605419344,43.8913591593083,124.272026060151)) ;
#91428=CARTESIAN_POINT('Ctrl Pts',(-20.4209894341323,43.9047150645893,124.529371523142)) ;
#91429=CARTESIAN_POINT('Ctrl Pts',(-20.2138465893309,43.9146117132271,124.686685290461)) ;
#91430=CARTESIAN_POINT('Ctrl Pts',(-19.9790841361338,43.9246598512796,124.807515218539)) ;
#91431=CARTESIAN_POINT('Ctrl Pts',(-19.7308190710791,43.9345508114574,124.884524562432)) ;
#91432=CARTESIAN_POINT('Ctrl Pts',(-19.4703839376697,43.9445436473341,124.918248825918)) ;
#91433=CARTESIAN_POINT('Ctrl Pts',(-19.2068845324014,43.9545827423357,124.905579235426)) ;
#91434=CARTESIAN_POINT('Ctrl Pts',(-18.9545857300593,43.9644200981869,124.849099649171)) ;
#91435=CARTESIAN_POINT('Ctrl Pts',(-18.6296690897415,43.9778130461176,124.713956490856)) ;
#91436=CARTESIAN_POINT('Ctrl Pts',(-18.3520981743961,43.9909797225445,124.500694921199)) ;
#91437=CARTESIAN_POINT('Ctrl Pts',(-18.1378620138643,44.0043645039513,124.221797775786)) ;
#91438=CARTESIAN_POINT('Ctrl Pts',(-18.0179672616378,44.0142262865952,123.991995123024)) ;
#91439=CARTESIAN_POINT('Ctrl Pts',(-17.9383259095293,44.0242254345482,123.741642443432)) ;
#91440=CARTESIAN_POINT('Ctrl Pts',(-17.9034476011342,44.0341282271653,123.483699776961)) ;
#91441=CARTESIAN_POINT('Ctrl Pts',(-17.9141092543276,44.0441778070562,123.219886940427)) ;
#91442=CARTESIAN_POINT('Ctrl Pts',(-17.987359893705,44.0573648808657,122.881047522662)) ;
#91443=CARTESIAN_POINT('Ctrl Pts',(-18.1910325351083,44.0741176708369,122.485294726917)) ;
#91444=CARTESIAN_POINT('Ctrl Pts',(-18.5127079665964,44.0906063229316,122.187409946864)) ;
#91445=CARTESIAN_POINT('Ctrl Pts',(-18.8227881728284,44.103963149115,122.02310778574)) ;
#91446=CARTESIAN_POINT('Ctrl Pts',(-19.0702563997621,44.1138595339929,121.942965399191)) ;
#91447=CARTESIAN_POINT('Ctrl Pts',(-19.3306048043616,44.1238660485134,121.906491121348)) ;
#91448=CARTESIAN_POINT('Ctrl Pts',(-19.6771635039031,44.1370561720298,121.917876124668)) ;
#91449=CARTESIAN_POINT('Ctrl Pts',(-20.1033013954012,44.1538227331793,122.047686667172)) ;
#91450=CARTESIAN_POINT('Ctrl Pts',(-20.5238929989773,44.1736072218874,122.363542810504)) ;
#91451=CARTESIAN_POINT('Ctrl Pts',(-20.815011621917,44.1935526694839,122.806412748844)) ;
#91452=CARTESIAN_POINT('Ctrl Pts',(-20.9368621718498,44.2134643316398,123.321424916447)) ;
#91453=CARTESIAN_POINT('Ctrl Pts',(-20.8768657552607,44.2333565236587,123.846793390736)) ;
#91454=CARTESIAN_POINT('Ctrl Pts',(-20.6387805843268,44.2533976542133,124.323200523711)) ;
#91455=CARTESIAN_POINT('Ctrl Pts',(-20.2567572002547,44.2732159888289,124.686031568202)) ;
#91456=CARTESIAN_POINT('Ctrl Pts',(-19.7707167595738,44.2931885540485,124.899018477373)) ;
#91457=CARTESIAN_POINT('Ctrl Pts',(-19.243012073421,44.3130777702201,124.933377526462)) ;
#91458=CARTESIAN_POINT('Ctrl Pts',(-18.7322499924567,44.3331013445428,124.784342715249)) ;
#91459=CARTESIAN_POINT('Ctrl Pts',(-18.3074523247711,44.352898507631,124.473689351128)) ;
#91460=CARTESIAN_POINT('Ctrl Pts',(-18.0107208479656,44.3728640014548,124.033892370887)) ;
#91461=CARTESIAN_POINT('Ctrl Pts',(-17.8825301084476,44.3928177091962,123.519135613177)) ;
#91462=CARTESIAN_POINT('Ctrl Pts',(-17.9375131053142,44.4127250859228,122.993014954846)) ;
#91463=CARTESIAN_POINT('Ctrl Pts',(-18.1669119070672,44.4325772974714,122.517754743088)) ;
#91464=CARTESIAN_POINT('Ctrl Pts',(-18.5491999521954,44.4526496844171,122.145668046979)) ;
#91465=CARTESIAN_POINT('Ctrl Pts',(-19.0301389700753,44.4724875540574,121.9295612266)) ;
#91466=CARTESIAN_POINT('Ctrl Pts',(-19.556112431027,44.4923382086105,121.888236492257)) ;
#91467=CARTESIAN_POINT('Ctrl Pts',(-20.0695268056747,44.512390142951,122.031046366895)) ;
#91468=CARTESIAN_POINT('Ctrl Pts',(-20.4987446170897,44.532223330517,122.337261350157)) ;
#91469=CARTESIAN_POINT('Ctrl Pts',(-20.7998380093603,44.5521525427477,122.772809047979)) ;
#91470=CARTESIAN_POINT('Ctrl Pts',(-20.9346380609838,44.5720375079621,123.284047944812)) ;
#91471=CARTESIAN_POINT('Ctrl Pts',(-20.8856425940297,44.5921112491067,123.815212598448)) ;
#91472=CARTESIAN_POINT('Ctrl Pts',(-20.6614851629729,44.6119044308871,124.291227274791)) ;
#91473=CARTESIAN_POINT('Ctrl Pts',(-20.2863772074548,44.6318671388898,124.666405427892)) ;
#91474=CARTESIAN_POINT('Ctrl Pts',(-19.8046798286043,44.6518500906322,124.8901432235)) ;
#91475=CARTESIAN_POINT('Ctrl Pts',(-19.2801648941078,44.6716607104044,124.936716143029)) ;
#91476=CARTESIAN_POINT('Ctrl Pts',(-18.7667918531497,44.6916444264373,124.800971420717)) ;
#91477=CARTESIAN_POINT('Ctrl Pts',(-18.332633623527,44.7115258903346,124.499523849295)) ;
#91478=CARTESIAN_POINT('Ctrl Pts',(-18.0261041134591,44.731481220179,124.066823654643)) ;
#91479=CARTESIAN_POINT('Ctrl Pts',(-17.8857718639008,44.7513566809845,123.557460531844)) ;
#91480=CARTESIAN_POINT('Ctrl Pts',(-17.9275871464799,44.771341001036,123.028016369146)) ;
#91481=CARTESIAN_POINT('Ctrl Pts',(-18.1472823916272,44.7912690338256,122.54594681577)) ;
#91482=CARTESIAN_POINT('Ctrl Pts',(-18.4563072638141,44.8078777957654,122.230852995871)) ;
#91483=CARTESIAN_POINT('Ctrl Pts',(-18.7544344166136,44.8210654344555,122.054104346629)) ;
#91484=CARTESIAN_POINT('Ctrl Pts',(-18.9997577413404,44.8310518688156,121.960933276629)) ;
#91485=CARTESIAN_POINT('Ctrl Pts',(-19.2582000487417,44.841061242775,121.911919172374)) ;
#91486=CARTESIAN_POINT('Ctrl Pts',(-19.6074259157018,44.8543512763403,121.90718231146)) ;
#91487=CARTESIAN_POINT('Ctrl Pts',(-20.0350744145889,44.8709452640027,122.015110092288)) ;
#91488=CARTESIAN_POINT('Ctrl Pts',(-20.4010334172279,44.8875775192782,122.263044894367)) ;
#91489=CARTESIAN_POINT('Ctrl Pts',(-20.6289076195677,44.9008199029461,122.52606867887)) ;
#91490=CARTESIAN_POINT('Ctrl Pts',(-20.7634193394176,44.9107341111735,122.749205301052)) ;
#91491=CARTESIAN_POINT('Ctrl Pts',(-20.8581992855926,44.9207907504452,122.995881649194)) ;
#91492=CARTESIAN_POINT('Ctrl Pts',(-20.9079626866539,44.9306365568653,123.249811042525)) ;
#91493=CARTESIAN_POINT('Ctrl Pts',(-20.9134321153544,44.9406815564985,123.513714183674)) ;
#91494=CARTESIAN_POINT('Ctrl Pts',(-20.8594529735354,44.9539625788713,123.85851431483)) ;
#91495=CARTESIAN_POINT('Ctrl Pts',(-20.7185138341195,44.9671600253959,124.179729076087)) ;
#91496=CARTESIAN_POINT('Ctrl Pts',(-20.4978542341181,44.9805743232029,124.454653630732)) ;
#91497=CARTESIAN_POINT('Ctrl Pts',(-20.3035482186063,44.9904133886056,124.625258093541)) ;
#91498=CARTESIAN_POINT('Ctrl Pts',(-20.0797292255048,45.0003965948833,124.762068121514)) ;
#91499=CARTESIAN_POINT('Ctrl Pts',(-19.8362653995539,45.0103478297961,124.857563683997)) ;
#91500=CARTESIAN_POINT('Ctrl Pts',(-19.5787021577369,45.0203488294977,124.90990497468)) ;
#91501=CARTESIAN_POINT('Ctrl Pts',(-19.3151704808666,45.0303801752851,124.916336383632)) ;
#91502=CARTESIAN_POINT('Ctrl Pts',(-19.059076565559,45.0402339399901,124.877961736359)) ;
#91503=CARTESIAN_POINT('Ctrl Pts',(-18.8104579041759,45.0502045936584,124.795331193507)) ;
#91504=CARTESIAN_POINT('Ctrl Pts',(-18.5792936637788,45.0602018373156,124.670414452979)) ;
#91505=CARTESIAN_POINT('Ctrl Pts',(-18.372843216216,45.0702352932598,124.506439042019)) ;
#91506=CARTESIAN_POINT('Ctrl Pts',(-18.2007560512662,45.0800907975602,124.312851502277)) ;
#91507=CARTESIAN_POINT('Ctrl Pts',(-18.0626513107753,45.0900902338463,124.08934966355)) ;
#91508=CARTESIAN_POINT('Ctrl Pts',(-17.966160872868,45.0999846933622,123.847847223486)) ;
#91509=CARTESIAN_POINT('Ctrl Pts',(-17.9122601551696,45.1100478128138,123.588997131048)) ;
#91510=CARTESIAN_POINT('Ctrl Pts',(-17.9040157128179,45.1198874472258,123.330510182851)) ;
#91511=CARTESIAN_POINT('Ctrl Pts',(-17.9412701233928,45.1299506547116,123.068734224408)) ;
#91512=CARTESIAN_POINT('Ctrl Pts',(-18.0222577929814,45.1398447620908,122.821630638561)) ;
#91513=CARTESIAN_POINT('Ctrl Pts',(-18.1448705736183,45.1497870942832,122.590953885684)) ;
#91514=CARTESIAN_POINT('Ctrl Pts',(-18.3065622324811,45.1597877205982,122.383723321206)) ;
#91515=CARTESIAN_POINT('Ctrl Pts',(-18.502862990913,45.1698294548801,122.207402005079)) ;
#91516=CARTESIAN_POINT('Ctrl Pts',(-18.7217059912546,45.1796548808292,122.070339801105)) ;
#91517=CARTESIAN_POINT('Ctrl Pts',(-18.966474765151,45.1897117073569,121.970725354272)) ;
#91518=CARTESIAN_POINT('Ctrl Pts',(-19.2216074988033,45.1996391404784,121.916190939513)) ;
#91519=CARTESIAN_POINT('Ctrl Pts',(-19.4828944941186,45.2095891328847,121.906015436364)) ;
#91520=CARTESIAN_POINT('Ctrl Pts',(-19.7446272926651,45.2196443339587,121.942195083293)) ;
#91521=CARTESIAN_POINT('Ctrl Pts',(-19.9904565700812,45.229466608011,122.020960921677)) ;
#91522=CARTESIAN_POINT('Ctrl Pts',(-20.2244926759389,45.2395225019702,122.143638300963)) ;
#91523=CARTESIAN_POINT('Ctrl Pts',(-20.4310152546762,45.2494632238153,122.303624668569)) ;
#91524=CARTESIAN_POINT('Ctrl Pts',(-20.6065787562621,45.2593675679019,122.495779589979)) ;
#91525=CARTESIAN_POINT('Ctrl Pts',(-20.7479598031112,45.2694142352014,122.718723494218)) ;
#91526=CARTESIAN_POINT('Ctrl Pts',(-20.847214873449,45.2793097936513,122.959126759267)) ;
#91527=CARTESIAN_POINT('Ctrl Pts',(-20.9041452558885,45.289371872356,123.217307547921)) ;
#91528=CARTESIAN_POINT('Ctrl Pts',(-20.9152880545128,45.2992145708218,123.475752573775)) ;
#91529=CARTESIAN_POINT('Ctrl Pts',(-20.8815017658848,45.3092053447163,123.736083691839)) ;
#91530=CARTESIAN_POINT('Ctrl Pts',(-20.803464341165,45.3191332139512,123.985045208885)) ;
#91531=CARTESIAN_POINT('Ctrl Pts',(-20.6830597025419,45.329121942921,124.218310172985)) ;
#91532=CARTESIAN_POINT('Ctrl Pts',(-20.5228027489551,45.3391613449048,124.427867674991)) ;
#91533=CARTESIAN_POINT('Ctrl Pts',(-20.3327730605954,45.3490015126416,124.603267061586)) ;
#91534=CARTESIAN_POINT('Ctrl Pts',(-20.1108060666027,45.3590497230161,124.746272176201)) ;
#91535=CARTESIAN_POINT('Ctrl Pts',(-19.8696532867426,45.3689968933038,124.847160076547)) ;
#91536=CARTESIAN_POINT('Ctrl Pts',(-19.6157459454995,45.3789077415589,124.90519559881)) ;
#91537=CARTESIAN_POINT('Ctrl Pts',(-19.3518125734357,45.3889640692367,124.918205064877)) ;
#91538=CARTESIAN_POINT('Ctrl Pts',(-19.0949419766038,45.3988144820052,124.886084607511)) ;
#91539=CARTESIAN_POINT('Ctrl Pts',(-18.8429458077784,45.4088413678389,124.809102515911)) ;
#91540=CARTESIAN_POINT('Ctrl Pts',(-18.6084007715185,45.4188699834697,124.688897924885)) ;
#91541=CARTESIAN_POINT('Ctrl Pts',(-18.4018578835291,45.4287152068472,124.533108889477)) ;
#91542=CARTESIAN_POINT('Ctrl Pts',(-18.2223677576914,45.4387058889488,124.341493091567)) ;
#91543=CARTESIAN_POINT('Ctrl Pts',(-18.0786949591788,45.4487437775813,124.120270887316)) ;
#91544=CARTESIAN_POINT('Ctrl Pts',(-17.9771820255855,45.4585881126844,123.882309246234)) ;
#91545=CARTESIAN_POINT('Ctrl Pts',(-17.9171992662685,45.4685730748819,123.62689961788)) ;
#91546=CARTESIAN_POINT('Ctrl Pts',(-17.9024172623288,45.4785120164153,123.366094931073)) ;
#91547=CARTESIAN_POINT('Ctrl Pts',(-17.9335377045302,45.4885539013867,123.104071689988)) ;
#91548=CARTESIAN_POINT('Ctrl Pts',(-18.0083583615695,45.498440449295,122.855243316233)) ;
#91549=CARTESIAN_POINT('Ctrl Pts',(-18.1261441567159,45.508434374795,122.620545045069)) ;
#91550=CARTESIAN_POINT('Ctrl Pts',(-18.2819302055561,45.5183704659215,122.410950315548)) ;
#91551=CARTESIAN_POINT('Ctrl Pts',(-18.4735027254418,45.5283997349014,122.229995789476)) ;
#91552=CARTESIAN_POINT('Ctrl Pts',(-18.690241481066,45.5382821174607,122.086859617476)) ;
#91553=CARTESIAN_POINT('Ctrl Pts',(-18.9325349471609,45.5483346345486,121.981703543276)) ;
#91554=CARTESIAN_POINT('Ctrl Pts',(-19.185413729496,45.5582287553725,121.921034104185)) ;
#91555=CARTESIAN_POINT('Ctrl Pts',(-19.4493049697019,45.5682907347929,121.904866941073)) ;
#91556=CARTESIAN_POINT('Ctrl Pts',(-19.7063630081236,45.5781352680218,121.934093132553)) ;
#91557=CARTESIAN_POINT('Ctrl Pts',(-19.9576058706028,45.5880953469281,122.007462571973)) ;
#91558=CARTESIAN_POINT('Ctrl Pts',(-20.1938981415272,45.5981336235007,122.124711964626)) ;
#91559=CARTESIAN_POINT('Ctrl Pts',(-20.4030909048024,45.6080070100386,122.278267729606)) ;
#91560=CARTESIAN_POINT('Ctrl Pts',(-20.5859499300167,45.6180799528056,122.469592306891)) ;
#91561=CARTESIAN_POINT('Ctrl Pts',(-20.7294620067179,45.6279013669339,122.684171707813)) ;
#91562=CARTESIAN_POINT('Ctrl Pts',(-20.836469961144,45.6379759970062,122.92628036698)) ;
#91563=CARTESIAN_POINT('Ctrl Pts',(-20.8984204591589,45.6478426343231,123.178089581566)) ;
#91564=CARTESIAN_POINT('Ctrl Pts',(-20.9166539511471,45.6578661796949,123.440853736035)) ;
#91565=CARTESIAN_POINT('Ctrl Pts',(-20.8883451902421,45.6678919312121,123.702810647261)) ;
#91566=CARTESIAN_POINT('Ctrl Pts',(-20.8166655858108,45.6777455182215,123.951620064222)) ;
#91567=CARTESIAN_POINT('Ctrl Pts',(-20.7020665615135,45.6877224784494,124.187438612339)) ;
#91568=CARTESIAN_POINT('Ctrl Pts',(-20.5472320226334,45.6977436214779,124.400440473039)) ;
#91569=CARTESIAN_POINT('Ctrl Pts',(-20.3607129644231,45.7076262274978,124.581203675269)) ;
#91570=CARTESIAN_POINT('Ctrl Pts',(-20.1416041543845,45.7176946981305,124.729442692636)) ;
#91571=CARTESIAN_POINT('Ctrl Pts',(-19.9058440233542,45.7275247813142,124.835139992)) ;
#91572=CARTESIAN_POINT('Ctrl Pts',(-19.6494558792354,45.7375913409946,124.900127141566)) ;
#91573=CARTESIAN_POINT('Ctrl Pts',(-19.3902123872049,45.7474815908238,124.919112847795)) ;
#91574=CARTESIAN_POINT('Ctrl Pts',(-19.1289348372093,45.7574737565726,124.893103063459)) ;
#91575=CARTESIAN_POINT('Ctrl Pts',(-18.8769434953996,45.7674366001687,124.822088336448)) ;
#91576=CARTESIAN_POINT('Ctrl Pts',(-18.6421852615433,45.7773407689965,124.709652708434)) ;
#91577=CARTESIAN_POINT('Ctrl Pts',(-18.4273528974957,45.7874016438908,124.555606852268)) ;
#91578=CARTESIAN_POINT('Ctrl Pts',(-18.2462968796542,45.7972405472202,124.370967398921)) ;
#91579=CARTESIAN_POINT('Ctrl Pts',(-18.0964786782735,45.8073089235941,124.152936536302)) ;
#91580=CARTESIAN_POINT('Ctrl Pts',(-17.9888851621427,45.8171895402267,123.916582846629)) ;
#91581=CARTESIAN_POINT('Ctrl Pts',(-17.9227453188288,45.8271807004557,123.662532284139)) ;
#91582=CARTESIAN_POINT('Ctrl Pts',(-17.9017535244661,45.8371337738878,123.401780145108)) ;
#91583=CARTESIAN_POINT('Ctrl Pts',(-17.9266404178476,45.8471696095005,123.139247618234)) ;
#91584=CARTESIAN_POINT('Ctrl Pts',(-17.9955552265189,45.8570597362306,122.888631027566)) ;
#91585=CARTESIAN_POINT('Ctrl Pts',(-18.1076934818933,45.8670519179999,122.651211136144)) ;
#91586=CARTESIAN_POINT('Ctrl Pts',(-18.2587304245374,45.8769978579744,122.437900289644)) ;
#91587=CARTESIAN_POINT('Ctrl Pts',(-18.4441704878577,45.8869450417339,122.253645296691)) ;
#91588=CARTESIAN_POINT('Ctrl Pts',(-18.6611101574099,45.8969929800242,122.103131587065)) ;
#91589=CARTESIAN_POINT('Ctrl Pts',(-18.8960272898149,45.9068406148377,121.994572618097)) ;
#91590=CARTESIAN_POINT('Ctrl Pts',(-19.148898873225,45.9168023285357,121.926896838604)) ;
#91591=CARTESIAN_POINT('Ctrl Pts',(-19.4114894160667,45.9268309643569,121.904333417555)) ;
#91592=CARTESIAN_POINT('Ctrl Pts',(-19.6708912056313,45.9367412791087,121.92734461787)) ;
#91593=CARTESIAN_POINT('Ctrl Pts',(-19.9231784918885,45.9466761497713,121.994557839022)) ;
#91594=CARTESIAN_POINT('Ctrl Pts',(-20.1623713001247,45.9567173321731,122.10595274913)) ;
#91595=CARTESIAN_POINT('Ctrl Pts',(-20.3754171966407,45.9666043036378,122.254712550326)) ;
#91596=CARTESIAN_POINT('Ctrl Pts',(-20.5616853384859,45.9766037359004,122.440014625736)) ;
#91597=CARTESIAN_POINT('Ctrl Pts',(-20.7119304588546,45.986523801157,122.65309125952)) ;
#91598=CARTESIAN_POINT('Ctrl Pts',(-20.8242304858689,45.9965606537412,122.891731631287)) ;
#91599=CARTESIAN_POINT('Ctrl Pts',(-20.8925312466949,46.0064733130812,123.143117767075)) ;
#91600=CARTESIAN_POINT('Ctrl Pts',(-20.9169022735991,46.0164645249961,123.404558617935)) ;
#91601=CARTESIAN_POINT('Ctrl Pts',(-20.8948119575861,46.0265061663992,123.667495012575)) ;
#91602=CARTESIAN_POINT('Ctrl Pts',(-20.8294454785966,46.0363349606062,123.917414465479)) ;
#91603=CARTESIAN_POINT('Ctrl Pts',(-20.7191022663443,46.0464113717275,124.158067817818)) ;
#91604=CARTESIAN_POINT('Ctrl Pts',(-20.5720475565284,46.05626350477,124.371223090758)) ;
#91605=CARTESIAN_POINT('Ctrl Pts',(-20.3863654461432,46.0663367391113,124.559830827429)) ;
#91606=CARTESIAN_POINT('Ctrl Pts',(-20.1756244871386,46.0761782404379,124.709777652691)) ;
#91607=CARTESIAN_POINT('Ctrl Pts',(-19.9396627498854,46.0861391920327,124.823081201135)) ;
#91608=CARTESIAN_POINT('Ctrl Pts',(-19.6855248863959,46.0961770097533,124.893729687363)) ;
#91609=CARTESIAN_POINT('Ctrl Pts',(-19.427262518452,46.1060513590104,124.919247547046)) ;
#91610=CARTESIAN_POINT('Ctrl Pts',(-19.1634478041723,46.1161209097526,124.899133803632)) ;
#91611=CARTESIAN_POINT('Ctrl Pts',(-18.9130319171502,46.1259549292612,124.835182189416)) ;
#91612=CARTESIAN_POINT('Ctrl Pts',(-18.6724817634697,46.1359890838408,124.727205773932)) ;
#91613=CARTESIAN_POINT('Ctrl Pts',(-18.4550722737311,46.1460050096632,124.57881549919)) ;
#91614=CARTESIAN_POINT('Ctrl Pts',(-18.2689263313037,46.1558872648575,124.397725200321)) ;
#91615=CARTESIAN_POINT('Ctrl Pts',(-18.1151695920916,46.1658760713684,124.185010592068)) ;
#91616=CARTESIAN_POINT('Ctrl Pts',(-18.0009343743277,46.1758246386311,123.949804922474)) ;
#91617=CARTESIAN_POINT('Ctrl Pts',(-17.9287986502812,46.1858794439331,123.695642276881)) ;
#91618=CARTESIAN_POINT('Ctrl Pts',(-17.9021457183122,46.1956982271967,123.438981604419)) ;
#91619=CARTESIAN_POINT('Ctrl Pts',(-17.920160334372,46.2057339995573,123.175874359375)) ;
#91620=CARTESIAN_POINT('Ctrl Pts',(-17.984249977082,46.2157586985859,122.920340925666)) ;
#91621=CARTESIAN_POINT('Ctrl Pts',(-18.0893591005861,46.225610701845,122.683731790801)) ;
#91622=CARTESIAN_POINT('Ctrl Pts',(-18.2356413391738,46.2356016362422,122.465745544367)) ;
#91623=CARTESIAN_POINT('Ctrl Pts',(-18.4161423749505,46.2455195586733,122.277688444646)) ;
#91624=CARTESIAN_POINT('Ctrl Pts',(-18.6288192425981,46.2555479143556,122.122101309996)) ;
#91625=CARTESIAN_POINT('Ctrl Pts',(-18.8618561314838,46.2654321988662,122.007348465011)) ;
#91626=CARTESIAN_POINT('Ctrl Pts',(-19.1138378721338,46.2754248827741,121.933438370644)) ;
#91627=CARTESIAN_POINT('Ctrl Pts',(-19.3758193880109,46.2854536197818,121.904757212364)) ;
#91628=CARTESIAN_POINT('Ctrl Pts',(-19.6350724012937,46.2953390164107,121.921411675567)) ;
#91629=CARTESIAN_POINT('Ctrl Pts',(-19.8901659266548,46.3053269018246,121.983092596544)) ;
#91630=CARTESIAN_POINT('Ctrl Pts',(-20.1298859961201,46.3152776044852,122.087654097686)) ;
#91631=CARTESIAN_POINT('Ctrl Pts',(-20.3496387002322,46.3253179225826,122.233636338155)) ;
#91632=CARTESIAN_POINT('Ctrl Pts',(-20.5377696612843,46.3351924879158,122.412406684327)) ;
#91633=CARTESIAN_POINT('Ctrl Pts',(-20.6941818778816,46.3451921479769,122.623513973067)) ;
#91634=CARTESIAN_POINT('Ctrl Pts',(-20.8107624841862,46.3551011431446,122.856409152193)) ;
#91635=CARTESIAN_POINT('Ctrl Pts',(-20.8861223158461,46.3651558843079,123.109617925359)) ;
#91636=CARTESIAN_POINT('Ctrl Pts',(-20.9160894530664,46.3750144962217,123.366999052458)) ;
#91637=CARTESIAN_POINT('Ctrl Pts',(-20.90075393306,46.385082618501,123.631095083211)) ;
#91638=CARTESIAN_POINT('Ctrl Pts',(-20.8410490247791,46.3949380892042,123.883133457476)) ;
#91639=CARTESIAN_POINT('Ctrl Pts',(-20.7377739074065,46.4049329486976,124.124622613945)) ;
#91640=CARTESIAN_POINT('Ctrl Pts',(-20.5931317991477,46.4149642020395,124.345013634199)) ;
#91641=CARTESIAN_POINT('Ctrl Pts',(-20.4156811920431,46.4248309009126,124.534077171764)) ;
#91642=CARTESIAN_POINT('Ctrl Pts',(-20.2058603225502,46.4348177166638,124.691672146936)) ;
#91643=CARTESIAN_POINT('Ctrl Pts',(-19.9727878453625,46.4447649218593,124.810106319578)) ;
#91644=CARTESIAN_POINT('Ctrl Pts',(-19.7203014995016,46.4548079099855,124.886878521839)) ;
#91645=CARTESIAN_POINT('Ctrl Pts',(-19.462892547754,46.464675264607,124.918244909157)) ;
#91646=CARTESIAN_POINT('Ctrl Pts',(-19.2013450743715,46.4746411579051,124.905008550705)) ;
#91647=CARTESIAN_POINT('Ctrl Pts',(-18.9446202495613,46.4846649352812,124.845948246086)) ;
#91648=CARTESIAN_POINT('Ctrl Pts',(-18.7044304082566,46.4945904832129,124.744281867912)) ;
#91649=CARTESIAN_POINT('Ctrl Pts',(-18.4848534110883,46.5045309596339,124.60274474947)) ;
#91650=CARTESIAN_POINT('Ctrl Pts',(-18.2913765899753,46.5145771692968,124.423144114639)) ;
#91651=CARTESIAN_POINT('Ctrl Pts',(-18.1347125364933,46.5244384259586,124.216689383634)) ;
#91652=CARTESIAN_POINT('Ctrl Pts',(-18.0143126829843,46.5344320542339,123.983335039586)) ;
#91653=CARTESIAN_POINT('Ctrl Pts',(-17.9366394008495,46.5443574515441,123.734298668841)) ;
#91654=CARTESIAN_POINT('Ctrl Pts',(-17.9030455996264,46.5543853594543,123.472960192196)) ;
#91655=CARTESIAN_POINT('Ctrl Pts',(-17.9149012642186,46.5642716751235,123.213390481439)) ;
#91656=CARTESIAN_POINT('Ctrl Pts',(-17.972325349276,46.5743032700273,122.956144198347)) ;
#91657=CARTESIAN_POINT('Ctrl Pts',(-18.0718482092479,46.584185512979,122.716230515682)) ;
#91658=CARTESIAN_POINT('Ctrl Pts',(-18.2138880944537,46.5942449840088,122.493315287928)) ;
#91659=CARTESIAN_POINT('Ctrl Pts',(-18.3891039122629,46.604111428672,122.302179808622)) ;
#91660=CARTESIAN_POINT('Ctrl Pts',(-18.596403594826,46.6140775531207,122.142134294108)) ;
#91661=CARTESIAN_POINT('Ctrl Pts',(-18.8300357306055,46.6241077965118,122.020104455616)) ;
#91662=CARTESIAN_POINT('Ctrl Pts',(-19.0777840409719,46.6340008314649,121.941221742418)) ;
#91663=CARTESIAN_POINT('Ctrl Pts',(-19.3395213808909,46.6440517457017,121.905936560177)) ;
#91664=CARTESIAN_POINT('Ctrl Pts',(-19.5992144386022,46.6539415719263,121.916434213114)) ;
#91665=CARTESIAN_POINT('Ctrl Pts',(-19.9417614873954,46.6672763869732,121.990497581648)) ;
#91666=CARTESIAN_POINT('Ctrl Pts',(-20.2554096954557,46.6805534781447,122.152105027392)) ;
#91667=CARTESIAN_POINT('Ctrl Pts',(-20.5136667534488,46.693801766743,122.385643139726)) ;
#91668=CARTESIAN_POINT('Ctrl Pts',(-20.6757363842069,46.7038566082371,122.594281387087)) ;
#91669=CARTESIAN_POINT('Ctrl Pts',(-20.7967988624566,46.7136875975446,122.822559708019)) ;
#91670=CARTESIAN_POINT('Ctrl Pts',(-20.8785312557402,46.7237641618679,123.074384834974)) ;
#91671=CARTESIAN_POINT('Ctrl Pts',(-20.9144702982914,46.7336134870018,123.33073485832)) ;
#91672=CARTESIAN_POINT('Ctrl Pts',(-20.9029684187357,46.7469614866391,123.681333495441)) ;
#91673=CARTESIAN_POINT('Ctrl Pts',(-20.7745139330427,46.7635462461757,124.102969724517)) ;
#91674=CARTESIAN_POINT('Ctrl Pts',(-20.5110315388571,46.7801147975237,124.4557847313)) ;
#91675=CARTESIAN_POINT('Ctrl Pts',(-20.23514044175,46.7934746223427,124.672959741583)) ;
#91676=CARTESIAN_POINT('Ctrl Pts',(-20.0058449666823,46.8033800311734,124.796184304861)) ;
#91677=CARTESIAN_POINT('Ctrl Pts',(-19.7574240387125,46.8133400577574,124.878527441293)) ;
#91678=CARTESIAN_POINT('Ctrl Pts',(-19.4127438329402,46.8265976419427,124.929510558515)) ;
#91679=CARTESIAN_POINT('Ctrl Pts',(-18.9730785233433,46.8432488534374,124.87894995727)) ;
#91680=CARTESIAN_POINT('Ctrl Pts',(-18.4995437565153,46.8631670675477,124.642323373345)) ;
#91681=CARTESIAN_POINT('Ctrl Pts',(-18.1350267198472,46.8830448307685,124.259795228635)) ;
#91682=CARTESIAN_POINT('Ctrl Pts',(-17.9219959153182,46.9030574985557,123.772520415574)) ;
#91683=CARTESIAN_POINT('Ctrl Pts',(-17.8878670522062,46.9228700212223,123.246943798671)) ;
#91684=CARTESIAN_POINT('Ctrl Pts',(-18.035546506357,46.9428533212222,122.736872230293)) ;
#91685=CARTESIAN_POINT('Ctrl Pts',(-18.3474461325361,46.9627475983235,122.309804698334)) ;
#91686=CARTESIAN_POINT('Ctrl Pts',(-18.7866677876835,46.9826803600813,122.013601770197)) ;
#91687=CARTESIAN_POINT('Ctrl Pts',(-19.3015657425341,47.002646365846,121.885203552185)) ;
#91688=CARTESIAN_POINT('Ctrl Pts',(-19.8271303436553,47.0225248980109,121.939603120483)) ;
#91689=CARTESIAN_POINT('Ctrl Pts',(-20.3041868868379,47.0424645646712,122.170298147785)) ;
#91690=CARTESIAN_POINT('Ctrl Pts',(-20.6732403950815,47.0623594393166,122.549057326393)) ;
#91691=CARTESIAN_POINT('Ctrl Pts',(-20.8914282381446,47.0822665786099,123.030940138027)) ;
#91692=CARTESIAN_POINT('Ctrl Pts',(-20.9330126326835,47.1021771266884,123.558665033763)) ;
#91693=CARTESIAN_POINT('Ctrl Pts',(-20.7897985089648,47.1222457120455,124.072348596256)) ;
#91694=CARTESIAN_POINT('Ctrl Pts',(-20.4845832960142,47.1420275093603,124.500664842063)) ;
#91695=CARTESIAN_POINT('Ctrl Pts',(-20.0473415775769,47.1620350563049,124.802948543256)) ;
#91696=CARTESIAN_POINT('Ctrl Pts',(-19.5376373388019,47.1818567946077,124.936737621714)) ;
#91697=CARTESIAN_POINT('Ctrl Pts',(-19.0088143994453,47.2018368145119,124.889159509882)) ;
#91698=CARTESIAN_POINT('Ctrl Pts',(-18.5296831814101,47.2217542657741,124.664016484713)) ;
#91699=CARTESIAN_POINT('Ctrl Pts',(-18.156054658413,47.2416291869468,124.290549692997)) ;
#91700=CARTESIAN_POINT('Ctrl Pts',(-17.9309560929439,47.2616535554976,123.808318679437)) ;
#91701=CARTESIAN_POINT('Ctrl Pts',(-17.8844429064027,47.2815202398711,123.282262426708)) ;
#91702=CARTESIAN_POINT('Ctrl Pts',(-18.0199062073946,47.3014640617173,122.769851703785)) ;
#91703=CARTESIAN_POINT('Ctrl Pts',(-18.321723185349,47.3213714309688,122.335270498965)) ;
#91704=CARTESIAN_POINT('Ctrl Pts',(-18.7524373240201,47.3412461287155,122.029471467672)) ;
#91705=CARTESIAN_POINT('Ctrl Pts',(-19.2643995478987,47.3612280712373,121.888115658735)) ;
#91706=CARTESIAN_POINT('Ctrl Pts',(-19.7916438055128,47.3811307381481,121.930221264192)) ;
#91707=CARTESIAN_POINT('Ctrl Pts',(-20.2724952367668,47.4009860956868,122.147830932133)) ;
#91708=CARTESIAN_POINT('Ctrl Pts',(-20.6536636578321,47.4210501344028,122.52065673183)) ;
#91709=CARTESIAN_POINT('Ctrl Pts',(-20.8822481029672,47.4409053141279,122.996516067802)) ;
#91710=CARTESIAN_POINT('Ctrl Pts',(-20.935436165233,47.4608854187923,123.524678358585)) ;
#91711=CARTESIAN_POINT('Ctrl Pts',(-20.8068403946321,47.4806945239621,124.035381850163)) ;
#91712=CARTESIAN_POINT('Ctrl Pts',(-20.5095795524021,47.5006871443028,124.475622450521)) ;
#91713=CARTESIAN_POINT('Ctrl Pts',(-20.1539694207839,47.5172266268069,124.734264236863)) ;
#91714=CARTESIAN_POINT('Ctrl Pts',(-19.8262823346885,47.5305909448711,124.860472249389)) ;
#91715=CARTESIAN_POINT('Ctrl Pts',(-19.485405542771,47.5438085473726,124.927559945783)) ;
#91716=CARTESIAN_POINT('Ctrl Pts',(-19.0437703200357,47.5604661416504,124.898016262381)) ;
#91717=CARTESIAN_POINT('Ctrl Pts',(-18.5604499932118,47.5803318436921,124.685212590745)) ;
#91718=CARTESIAN_POINT('Ctrl Pts',(-18.2406362283115,47.5969615703822,124.380257695188)) ;
#91719=CARTESIAN_POINT('Ctrl Pts',(-18.0589404833083,47.61025068552,124.081950760843)) ;
#91720=CARTESIAN_POINT('Ctrl Pts',(-17.9633474747988,47.6202150324971,123.838187618009)) ;
#91721=CARTESIAN_POINT('Ctrl Pts',(-17.9115445460179,47.6301434004986,123.582486569596)) ;
#91722=CARTESIAN_POINT('Ctrl Pts',(-17.9020103793018,47.6434268335873,123.233497874318)) ;
#91723=CARTESIAN_POINT('Ctrl Pts',(-18.005095080809,47.6600789113277,122.803114333347)) ;
#91724=CARTESIAN_POINT('Ctrl Pts',(-18.247209882945,47.6766302806285,122.435837759358)) ;
#91725=CARTESIAN_POINT('Ctrl Pts',(-18.50783847541,47.6899177087775,122.203427580766)) ;
#91726=CARTESIAN_POINT('Ctrl Pts',(-18.7324805385707,47.6999622484776,122.064856373526)) ;
#91727=CARTESIAN_POINT('Ctrl Pts',(-18.9727568592771,47.7098050903014,121.969045673601)) ;
#91728=CARTESIAN_POINT('Ctrl Pts',(-19.2294948681427,47.7197893745484,121.915068774287)) ;
#91729=CARTESIAN_POINT('Ctrl Pts',(-19.4908350255121,47.7297390199475,121.906573088993)) ;
#91730=CARTESIAN_POINT('Ctrl Pts',(-19.7510324518848,47.7397387816359,121.943450958025)) ;
#91731=CARTESIAN_POINT('Ctrl Pts',(-20.001511154546,47.7497701275948,122.025612884837)) ;
#91732=CARTESIAN_POINT('Ctrl Pts',(-20.2300186287295,47.7596250820719,122.147499644092)) ;
#91733=CARTESIAN_POINT('Ctrl Pts',(-20.4366754769559,47.7695976200724,122.308615609026)) ;
#91734=CARTESIAN_POINT('Ctrl Pts',(-20.612644360831,47.7795926138074,122.503667729469)) ;
#91735=CARTESIAN_POINT('Ctrl Pts',(-20.7523101013191,47.7896266726015,122.727299317315)) ;
#91736=CARTESIAN_POINT('Ctrl Pts',(-20.8496668786128,47.7994820154245,122.967319880366)) ;
#91737=CARTESIAN_POINT('Ctrl Pts',(-20.904992548046,47.8094814947701,123.224157421193)) ;
#91738=CARTESIAN_POINT('Ctrl Pts',(-20.9150779626639,47.8193759435254,123.484026654786)) ;
#91739=CARTESIAN_POINT('Ctrl Pts',(-20.879224101965,47.8294390629599,123.745986877431)) ;
#91740=CARTESIAN_POINT('Ctrl Pts',(-20.8004688342771,47.8392787082011,123.992322380341)) ;
#91741=CARTESIAN_POINT('Ctrl Pts',(-20.6777398160996,47.8493418723872,124.226526704695)) ;
#91742=CARTESIAN_POINT('Ctrl Pts',(-20.5187066498922,47.859236142136,124.432268221858)) ;
#91743=CARTESIAN_POINT('Ctrl Pts',(-20.3259668872383,47.8691778681498,124.608589479913)) ;
#91744=CARTESIAN_POINT('Ctrl Pts',(-20.1041808999464,47.8791807568092,124.749765186793)) ;
#91745=CARTESIAN_POINT('Ctrl Pts',(-19.8602299792522,47.8892206056032,124.850187093091)) ;
#91746=CARTESIAN_POINT('Ctrl Pts',(-19.6081642424219,47.8990448210641,124.906094643254)) ;
#91747=CARTESIAN_POINT('Ctrl Pts',(-19.3441702977261,47.9091016645576,124.918019813108)) ;
#91748=CARTESIAN_POINT('Ctrl Pts',(-19.0854703555384,47.9190302739536,124.884016066394)) ;
#91749=CARTESIAN_POINT('Ctrl Pts',(-18.835802023627,47.9289821579915,124.806127703608)) ;
#91750=CARTESIAN_POINT('Ctrl Pts',(-18.6013347301841,47.9390351107991,124.684442693465)) ;
#91751=CARTESIAN_POINT('Ctrl Pts',(-18.3960367832778,47.9488579872653,124.527928911458)) ;
#91752=CARTESIAN_POINT('Ctrl Pts',(-18.2165695066782,47.9589137198354,124.333990312506)) ;
#91753=CARTESIAN_POINT('Ctrl Pts',(-18.0755119524271,47.9688544848231,124.114102984926)) ;
#91754=CARTESIAN_POINT('Ctrl Pts',(-17.97439677815,47.9787588177287,123.874266207495)) ;
#91755=CARTESIAN_POINT('Ctrl Pts',(-17.9157978478123,47.9888054866094,123.616858452994)) ;
#91756=CARTESIAN_POINT('Ctrl Pts',(-17.9027391893822,47.9987010499152,123.357099240434)) ;
#91757=CARTESIAN_POINT('Ctrl Pts',(-17.9355139727328,48.0087631076155,123.094756208375)) ;
#91758=CARTESIAN_POINT('Ctrl Pts',(-18.0115247975341,48.018605885243,122.847487885336)) ;
#91759=CARTESIAN_POINT('Ctrl Pts',(-18.130499270546,48.0285963634949,122.613492148444)) ;
#91760=CARTESIAN_POINT('Ctrl Pts',(-18.2873849531134,48.0385253361384,122.404982545336)) ;
#91761=CARTESIAN_POINT('Ctrl Pts',(-18.4789956662502,48.048516473018,122.225477178445)) ;
#91762=CARTESIAN_POINT('Ctrl Pts',(-18.6997215251481,48.0585385905069,122.081788244482)) ;
#91763=CARTESIAN_POINT('Ctrl Pts',(-18.9390060894404,48.0684391009091,121.979633386977)) ;
#91764=CARTESIAN_POINT('Ctrl Pts',(-19.1945602868354,48.0784280936552,121.9196516612)) ;
#91765=CARTESIAN_POINT('Ctrl Pts',(-19.4560251777434,48.0883933377058,121.905170872972)) ;
#91766=CARTESIAN_POINT('Ctrl Pts',(-19.714544749918,48.098297602219,121.935512588317)) ;
#91767=CARTESIAN_POINT('Ctrl Pts',(-19.9676521572524,48.1083556939172,122.01159018475)) ;
#91768=CARTESIAN_POINT('Ctrl Pts',(-20.1989410280847,48.1182056343456,122.127843264376)) ;
#91769=CARTESIAN_POINT('Ctrl Pts',(-20.4106352779193,48.1282326455192,122.284734900046)) ;
#91770=CARTESIAN_POINT('Ctrl Pts',(-20.5914129661359,48.1382612321312,122.476515291714)) ;
#91771=CARTESIAN_POINT('Ctrl Pts',(-20.7338940826546,48.1481064462439,122.692453451488)) ;
#91772=CARTESIAN_POINT('Ctrl Pts',(-20.8388889355934,48.1580971944235,122.933098046713)) ;
#91773=CARTESIAN_POINT('Ctrl Pts',(-20.9002278538488,48.168134828009,123.189645406397)) ;
#91774=CARTESIAN_POINT('Ctrl Pts',(-20.9162157833847,48.1779801172218,123.447878692139)) ;
#91775=CARTESIAN_POINT('Ctrl Pts',(-20.8873032918651,48.1879615180277,123.708561008633)) ;
#91776=CARTESIAN_POINT('Ctrl Pts',(-20.8137139164343,48.1979137510176,123.959536527466)) ;
#91777=CARTESIAN_POINT('Ctrl Pts',(-20.6974226162219,48.2079125624742,124.195182186014)) ;
#91778=CARTESIAN_POINT('Ctrl Pts',(-20.5409679874558,48.2179516664049,124.40758088976)) ;
#91779=CARTESIAN_POINT('Ctrl Pts',(-20.3544447338278,48.2277766088242,124.58612785741)) ;
#91780=CARTESIAN_POINT('Ctrl Pts',(-20.1350015577314,48.2378312963002,124.733273340073)) ;
#91781=CARTESIAN_POINT('Ctrl Pts',(-19.8958290741237,48.247774098657,124.838493759771)) ;
#91782=CARTESIAN_POINT('Ctrl Pts',(-19.6432087007226,48.2576778945968,124.901118420341)) ;
#91783=CARTESIAN_POINT('Ctrl Pts',(-19.3798197798372,48.2677246739718,124.919026044654)) ;
#91784=CARTESIAN_POINT('Ctrl Pts',(-19.1211868057863,48.2776203322664,124.891570258685)) ;
#91785=CARTESIAN_POINT('Ctrl Pts',(-18.8671159689922,48.287681899517,124.818466322481)) ;
#91786=CARTESIAN_POINT('Ctrl Pts',(-18.6346672337003,48.2975265439543,124.704882074842)) ;
#91787=CARTESIAN_POINT('Ctrl Pts',(-18.4224774448849,48.307486590197,124.551645752143)) ;
#91788=CARTESIAN_POINT('Ctrl Pts',(-18.2390630273348,48.3175248862154,124.362065332604)) ;
#91789=CARTESIAN_POINT('Ctrl Pts',(-18.0933378214402,48.3273982276337,124.147345292635)) ;
#91790=CARTESIAN_POINT('Ctrl Pts',(-17.9850701345174,48.337471331433,123.905844629381)) ;
#91791=CARTESIAN_POINT('Ctrl Pts',(-17.9216618145417,48.3472921465519,123.655621239189)) ;
#91792=CARTESIAN_POINT('Ctrl Pts',(-17.9018739629238,48.3573690116299,123.391601343181)) ;
#91793=CARTESIAN_POINT('Ctrl Pts',(-17.9277813877702,48.3672337512852,123.133631857944)) ;
#91794=CARTESIAN_POINT('Ctrl Pts',(-17.9985353622652,48.3772561545265,122.879946100013)) ;
#91795=CARTESIAN_POINT('Ctrl Pts',(-18.1129061323741,48.387281878815,122.642581869023)) ;
#91796=CARTESIAN_POINT('Ctrl Pts',(-18.2637423254893,48.3971366618363,122.432087433426)) ;
#91797=CARTESIAN_POINT('Ctrl Pts',(-18.4507029295602,48.4071155055596,122.248197667358)) ;
#91798=CARTESIAN_POINT('Ctrl Pts',(-18.6678616263483,48.4171343977962,122.099352690164)) ;
#91799=CARTESIAN_POINT('Ctrl Pts',(-18.9041396211026,48.4270176068372,121.991439850928)) ;
#91800=CARTESIAN_POINT('Ctrl Pts',(-19.1602260657838,48.4370859161774,121.925097919403)) ;
#91801=CARTESIAN_POINT('Ctrl Pts',(-19.4177670696848,48.4469160415101,121.904413532861)) ;
#91802=CARTESIAN_POINT('Ctrl Pts',(-19.6811181172093,48.4569825938871,121.928996874006)) ;
#91803=CARTESIAN_POINT('Ctrl Pts',(-19.9317618895005,48.4668728307808,121.997882966823)) ;
#91804=CARTESIAN_POINT('Ctrl Pts',(-20.1692610222621,48.4768650555748,122.109851831293)) ;
#91805=CARTESIAN_POINT('Ctrl Pts',(-20.3829445510021,48.4868276759257,122.261113657658)) ;
#91806=CARTESIAN_POINT('Ctrl Pts',(-20.5665261218062,48.4967326786889,122.445666071956)) ;
#91807=CARTESIAN_POINT('Ctrl Pts',(-20.7173958030492,48.506790441087,122.662655601088)) ;
#91808=CARTESIAN_POINT('Ctrl Pts',(-20.8262238273378,48.5166409604658,122.897552034887)) ;
#91809=CARTESIAN_POINT('Ctrl Pts',(-20.8943829996658,48.526672537464,123.152189944527)) ;
#91810=CARTESIAN_POINT('Ctrl Pts',(-20.9167426169127,48.5366822725689,123.414312273892)) ;
#91811=CARTESIAN_POINT('Ctrl Pts',(-20.8937179531658,48.5465918491952,123.673683390135)) ;
#91812=CARTESIAN_POINT('Ctrl Pts',(-20.8265228052753,48.5565192350519,123.925774756106)) ;
#91813=CARTESIAN_POINT('Ctrl Pts',(-20.7150907300863,48.5665641695422,124.165059353475)) ;
#91814=CARTESIAN_POINT('Ctrl Pts',(-20.5663090616085,48.5764501017301,124.378048058078)) ;
#91815=CARTESIAN_POINT('Ctrl Pts',(-20.3811550715041,48.5864434076831,124.564263272707)) ;
#91816=CARTESIAN_POINT('Ctrl Pts',(-20.1674323885774,48.596389045465,124.714704721664)) ;
#91817=CARTESIAN_POINT('Ctrl Pts',(-19.9310127579831,48.6063363138109,124.826259865705)) ;
#91818=CARTESIAN_POINT('Ctrl Pts',(-19.6762062907194,48.616384215948,124.895474138505)) ;
#91819=CARTESIAN_POINT('Ctrl Pts',(-19.4185018206962,48.6262319107882,124.919135372387)) ;
#91820=CARTESIAN_POINT('Ctrl Pts',(-19.157566898572,48.6361934205326,124.898267563706)) ;
#91821=CARTESIAN_POINT('Ctrl Pts',(-18.9025619508575,48.6462228121415,124.831614773843)) ;
#91822=CARTESIAN_POINT('Ctrl Pts',(-18.6658627752509,48.6561303076962,124.723165141493)) ;
#91823=CARTESIAN_POINT('Ctrl Pts',(-18.4504930203598,48.6660756993592,124.575141126783)) ;
#91824=CARTESIAN_POINT('Ctrl Pts',(-18.2628876791554,48.6760776169566,124.391000597497)) ;
#91825=CARTESIAN_POINT('Ctrl Pts',(-18.1099535759632,48.6861176845088,124.176032718824)) ;
#91826=CARTESIAN_POINT('Ctrl Pts',(-17.9985528130765,48.6959419959486,123.943106599342)) ;
#91827=CARTESIAN_POINT('Ctrl Pts',(-17.9273154063796,48.7059982371047,123.688649150822)) ;
#91828=CARTESIAN_POINT('Ctrl Pts',(-17.9019656863292,48.7159291588403,123.428879136997)) ;
#91829=CARTESIAN_POINT('Ctrl Pts',(-17.9215938866681,48.7258723949166,123.168352780034)) ;
#91830=CARTESIAN_POINT('Ctrl Pts',(-17.9861802002328,48.735853678929,122.914090093812)) ;
#91831=CARTESIAN_POINT('Ctrl Pts',(-18.0949989715361,48.7458979805547,122.673647794656)) ;
#91832=CARTESIAN_POINT('Ctrl Pts',(-18.2402534708388,48.7557260617741,122.460043836669)) ;
#91833=CARTESIAN_POINT('Ctrl Pts',(-18.4247849710024,48.7658026646233,122.270203460101)) ;
#91834=CARTESIAN_POINT('Ctrl Pts',(-18.6347065996334,48.7756547437418,122.118569547531)) ;
#91835=CARTESIAN_POINT('Ctrl Pts',(-18.8728105251633,48.7857280020508,122.002995475702)) ;
#91836=CARTESIAN_POINT('Ctrl Pts',(-19.1215857423761,48.7955694614311,121.932239761547)) ;
#91837=CARTESIAN_POINT('Ctrl Pts',(-19.3818649812545,48.8055305568434,121.904458482012)) ;
#91838=CARTESIAN_POINT('Ctrl Pts',(-19.6449795161499,48.8155678412401,121.922944960723)) ;
#91839=CARTESIAN_POINT('Ctrl Pts',(-19.8969273677844,48.8254441799754,121.985379683799)) ;
#91840=CARTESIAN_POINT('Ctrl Pts',(-20.1386336262622,48.8355063061287,122.092521249283)) ;
#91841=CARTESIAN_POINT('Ctrl Pts',(-20.3539244509202,48.8453744801052,122.237144739534)) ;
#91842=CARTESIAN_POINT('Ctrl Pts',(-20.543755011927,48.855380028609,122.419026520356)) ;
#91843=CARTESIAN_POINT('Ctrl Pts',(-20.6987419364052,48.8653626605046,122.630740739498)) ;
#91844=CARTESIAN_POINT('Ctrl Pts',(-20.8150482287937,48.8754066029264,122.867653599729)) ;
#91845=CARTESIAN_POINT('Ctrl Pts',(-20.8872135170498,48.8852347509536,123.115640682786)) ;
#91846=CARTESIAN_POINT('Ctrl Pts',(-20.9165222913364,48.8952246183279,123.376523659417)) ;
#91847=CARTESIAN_POINT('Ctrl Pts',(-20.8993147872527,48.9052683572834,123.639900737698)) ;
#91848=CARTESIAN_POINT('Ctrl Pts',(-20.8385460028974,48.9150901058214,123.890749443944)) ;
#91849=CARTESIAN_POINT('Ctrl Pts',(-20.7334926344583,48.9251250834311,124.132629488794)) ;
#91850=CARTESIAN_POINT('Ctrl Pts',(-20.5875669348054,48.9351499961888,124.351974416172)) ;
#91851=CARTESIAN_POINT('Ctrl Pts',(-20.4093201184437,48.9450019392826,124.539749635484)) ;
#91852=CARTESIAN_POINT('Ctrl Pts',(-20.1985093079883,48.9549929006117,124.696195980077)) ;
#91853=CARTESIAN_POINT('Ctrl Pts',(-19.9654731355136,48.9649107754802,124.812985422573)) ;
#91854=CARTESIAN_POINT('Ctrl Pts',(-19.7129807407904,48.9749392944814,124.888406605347)) ;
#91855=CARTESIAN_POINT('Ctrl Pts',(-19.4549910732823,48.9848229732793,124.918538485184)) ;
#91856=CARTESIAN_POINT('Ctrl Pts',(-19.1927471785049,48.994817916719,124.903825171715)) ;
#91857=CARTESIAN_POINT('Ctrl Pts',(-18.9363271652186,49.0048447705414,124.84316892203)) ;
#91858=CARTESIAN_POINT('Ctrl Pts',(-18.6976274329194,49.0147289348803,124.740719075366)) ;
#91859=CARTESIAN_POINT('Ctrl Pts',(-18.4778974629818,49.0247170329227,124.597194644998)) ;
#91860=CARTESIAN_POINT('Ctrl Pts',(-18.2869925249069,49.0346681393798,124.418428962904)) ;
#91861=CARTESIAN_POINT('Ctrl Pts',(-18.1286921061756,49.0447131905479,124.207206823015)) ;
#91862=CARTESIAN_POINT('Ctrl Pts',(-18.0115110053641,49.0545749509062,123.976053919716)) ;
#91863=CARTESIAN_POINT('Ctrl Pts',(-17.9347018565793,49.0645377677367,123.725760547945)) ;
#91864=CARTESIAN_POINT('Ctrl Pts',(-17.9027372037974,49.0745724490174,123.464015962194)) ;
#91865=CARTESIAN_POINT('Ctrl Pts',(-17.9160561245772,49.0844574787982,123.204553334292)) ;
#91866=CARTESIAN_POINT('Ctrl Pts',(-17.9753271704611,49.0945230721962,122.946810192394)) ;
#91867=CARTESIAN_POINT('Ctrl Pts',(-18.0759231780919,49.1043622405577,122.708574067968)) ;
#91868=CARTESIAN_POINT('Ctrl Pts',(-18.2192006262921,49.1144248382992,122.486356375471)) ;
#91869=CARTESIAN_POINT('Ctrl Pts',(-18.3961652533745,49.1243218507061,122.2957392912)) ;
#91870=CARTESIAN_POINT('Ctrl Pts',(-18.6037154643153,49.1342531725317,122.137521228201)) ;
#91871=CARTESIAN_POINT('Ctrl Pts',(-18.8382964268997,49.1442949352862,122.016665264985)) ;
#91872=CARTESIAN_POINT('Ctrl Pts',(-19.0864079744247,49.1541831341769,121.939390497466)) ;
#91873=CARTESIAN_POINT('Ctrl Pts',(-19.3468353464452,49.1641770727768,121.905608425672)) ;
#91874=CARTESIAN_POINT('Ctrl Pts',(-19.6078151277302,49.1741178938136,121.91751361713)) ;
#91875=CARTESIAN_POINT('Ctrl Pts',(-19.8632816579453,49.1840772761019,121.974327396906)) ;
#91876=CARTESIAN_POINT('Ctrl Pts',(-20.1060322896982,49.1940750357542,122.074891251936)) ;
#91877=CARTESIAN_POINT('Ctrl Pts',(-20.3282620364892,49.2041111719565,122.21690786839)) ;
#91878=CARTESIAN_POINT('Ctrl Pts',(-20.5190808378173,49.2139619694474,122.391836817215)) ;
#91879=CARTESIAN_POINT('Ctrl Pts',(-20.6790012985683,49.2239228345237,122.599055308519)) ;
#91880=CARTESIAN_POINT('Ctrl Pts',(-20.8010708002223,49.2339517021541,122.832645696346)) ;
#91881=CARTESIAN_POINT('Ctrl Pts',(-20.879853818226,49.2438619382905,123.080862806442)) ;
#91882=CARTESIAN_POINT('Ctrl Pts',(-20.9151078932877,49.253796891605,123.339559285952)) ;
#91883=CARTESIAN_POINT('Ctrl Pts',(-20.9045592317714,49.2638378220146,123.603207119489)) ;
#91884=CARTESIAN_POINT('Ctrl Pts',(-20.8494077535675,49.2737257187962,123.857140794924)) ;
#91885=CARTESIAN_POINT('Ctrl Pts',(-20.7504505562724,49.2837151704549,124.100280633098)) ;
#91886=CARTESIAN_POINT('Ctrl Pts',(-20.6110277047872,49.2936742608203,124.321756486501)) ;
#91887=CARTESIAN_POINT('Ctrl Pts',(-20.4368338343713,49.3035715731266,124.514921157602)) ;
#91888=CARTESIAN_POINT('Ctrl Pts',(-20.2284024122809,49.3136279990268,124.677354927092)) ;
#91889=CARTESIAN_POINT('Ctrl Pts',(-19.9992830178138,49.3234980016166,124.798974471006)) ;
#91890=CARTESIAN_POINT('Ctrl Pts',(-19.7493901780766,49.3335019347938,124.880531822233)) ;
#91891=CARTESIAN_POINT('Ctrl Pts',(-19.4894780018953,49.3434891952577,124.917271202357)) ;
#91892=CARTESIAN_POINT('Ctrl Pts',(-19.2261559513639,49.3535162468434,124.908135759446)) ;
#91893=CARTESIAN_POINT('Ctrl Pts',(-18.9718205949569,49.3634073366695,124.854401512994)) ;
#91894=CARTESIAN_POINT('Ctrl Pts',(-18.6475387787366,49.3767050914506,124.724316756299)) ;
#91895=CARTESIAN_POINT('Ctrl Pts',(-18.3663439177842,49.3899031510587,124.514527900887)) ;
#91896=CARTESIAN_POINT('Ctrl Pts',(-18.1484048267078,49.4032998916279,124.238071111464)) ;
#91897=CARTESIAN_POINT('Ctrl Pts',(-18.0253527815644,49.4131708037013,124.009661322498)) ;
#91898=CARTESIAN_POINT('Ctrl Pts',(-17.9421985890326,49.4232443654695,123.758399347314)) ;
#91899=CARTESIAN_POINT('Ctrl Pts',(-17.9045673262481,49.4330657780578,123.502999840485)) ;
#91900=CARTESIAN_POINT('Ctrl Pts',(-17.9117874809025,49.4431397952888,123.238428805641)) ;
#91901=CARTESIAN_POINT('Ctrl Pts',(-17.9808625993538,49.4562985822534,122.899526034126)) ;
#91902=CARTESIAN_POINT('Ctrl Pts',(-18.1386493012278,49.4696646853476,122.58136729471)) ;
#91903=CARTESIAN_POINT('Ctrl Pts',(-18.3706579537025,49.4829786202367,122.319337160576)) ;
#91904=CARTESIAN_POINT('Ctrl Pts',(-18.5739338777232,49.4928786596841,122.157029405636)) ;
#91905=CARTESIAN_POINT('Ctrl Pts',(-18.8036238095851,49.5028430628186,122.031257984843)) ;
#91906=CARTESIAN_POINT('Ctrl Pts',(-19.05335921375,49.5128730299398,121.946955300818)) ;
#91907=CARTESIAN_POINT('Ctrl Pts',(-19.3105895258516,49.5227753065488,121.907692131419)) ;
#91908=CARTESIAN_POINT('Ctrl Pts',(-19.6591707264257,49.536041235718,121.91483615231)) ;
#91909=CARTESIAN_POINT('Ctrl Pts',(-20.0833606626239,49.5526627668244,122.037946979199)) ;
#91910=CARTESIAN_POINT('Ctrl Pts',(-20.5104593674055,49.5725375954691,122.348915166531)) ;
#91911=CARTESIAN_POINT('Ctrl Pts',(-20.7582535736872,49.5892108035709,122.716248365857)) ;
#91912=CARTESIAN_POINT('Ctrl Pts',(-20.8714352247518,49.6024619285522,123.045592382337)) ;
#91913=CARTESIAN_POINT('Ctrl Pts',(-20.9269354813126,49.615704247373,123.389194785708)) ;
#91914=CARTESIAN_POINT('Ctrl Pts',(-20.8811511581855,49.6324374877125,123.831492590155)) ;
#91915=CARTESIAN_POINT('Ctrl Pts',(-20.6511878464973,49.6522666359005,124.305812689138)) ;
#91916=CARTESIAN_POINT('Ctrl Pts',(-20.2723991280832,49.6721913310011,124.675727471051)) ;
#91917=CARTESIAN_POINT('Ctrl Pts',(-19.7899488954886,49.6921145595845,124.894193343067)) ;
#91918=CARTESIAN_POINT('Ctrl Pts',(-19.2619611266706,49.7120416987106,124.935069014905)) ;
#91919=CARTESIAN_POINT('Ctrl Pts',(-18.7527411075181,49.7319181613263,124.794310345686)) ;
#91920=CARTESIAN_POINT('Ctrl Pts',(-18.3198072271694,49.7518953899316,124.486931020539)) ;
#91921=CARTESIAN_POINT('Ctrl Pts',(-18.018710731692,49.7718302479053,124.050908756306)) ;
#91922=CARTESIAN_POINT('Ctrl Pts',(-17.8842375144528,49.7917266968361,123.539519466163)) ;
#91923=CARTESIAN_POINT('Ctrl Pts',(-17.9318221676816,49.8116479809027,123.012164589738)) ;
#91924=CARTESIAN_POINT('Ctrl Pts',(-18.1570615290371,49.8316046305737,122.531918504927)) ;
#91925=CARTESIAN_POINT('Ctrl Pts',(-18.5309830443767,49.8514819236853,122.158801133981)) ;
#91926=CARTESIAN_POINT('Ctrl Pts',(-19.0095255521828,49.8713683959137,121.934252429302)) ;
#91927=CARTESIAN_POINT('Ctrl Pts',(-19.5406391317515,49.8914299618377,121.886868078949)) ;
#91928=CARTESIAN_POINT('Ctrl Pts',(-20.0501878146875,49.9112703693785,122.022537685724)) ;
#91929=CARTESIAN_POINT('Ctrl Pts',(-20.4843856180674,49.9311216933514,122.322319927731)) ;
#91930=CARTESIAN_POINT('Ctrl Pts',(-20.7926218042951,49.9511749633028,122.757047288943)) ;
#91931=CARTESIAN_POINT('Ctrl Pts',(-20.9325314728205,49.9709956206862,123.265078314232)) ;
#91932=CARTESIAN_POINT('Ctrl Pts',(-20.8912422361684,49.9909670420167,123.794102750068)) ;
#91933=CARTESIAN_POINT('Ctrl Pts',(-20.672728228111,50.0108605343804,124.275780483601)) ;
#91934=CARTESIAN_POINT('Ctrl Pts',(-20.3004875803372,50.0308846206214,124.65599343755)) ;
#91935=CARTESIAN_POINT('Ctrl Pts',(-19.8260699488102,50.0506894997343,124.884165170859)) ;
#91936=CARTESIAN_POINT('Ctrl Pts',(-19.2984073272745,50.0706485154322,124.938579634073)) ;
#91937=CARTESIAN_POINT('Ctrl Pts',(-18.7834458131184,50.0906345390612,124.808287005669)) ;
#91938=CARTESIAN_POINT('Ctrl Pts',(-18.3471380862029,50.1104430348217,124.513561025804)) ;
#91939=CARTESIAN_POINT('Ctrl Pts',(-18.034433731144,50.1304256739273,124.08441134622)) ;
#91940=CARTESIAN_POINT('Ctrl Pts',(-17.8877548058213,50.1503071217213,123.576622519046)) ;
#91941=CARTESIAN_POINT('Ctrl Pts',(-17.9228590595857,50.1702635884589,123.047489138174)) ;
#91942=CARTESIAN_POINT('Ctrl Pts',(-18.135325664709,50.1901409854144,122.563692670579)) ;
#91943=CARTESIAN_POINT('Ctrl Pts',(-18.5017404753757,50.2101229315897,122.179326787256)) ;
#91944=CARTESIAN_POINT('Ctrl Pts',(-18.9763311717451,50.2300520306265,121.94386229144)) ;
#91945=CARTESIAN_POINT('Ctrl Pts',(-19.5025542136779,50.2499806538391,121.884425032197)) ;
#91946=CARTESIAN_POINT('Ctrl Pts',(-20.0154098113017,50.2698149779455,122.006618943828)) ;
#91947=CARTESIAN_POINT('Ctrl Pts',(-20.3852796718983,50.2864672653289,122.249530478733)) ;
#91948=CARTESIAN_POINT('Ctrl Pts',(-20.6170613698565,50.2997277663511,122.509825199118)) ;
#91949=CARTESIAN_POINT('Ctrl Pts',(-20.7555282047836,50.3097292435524,122.733215342447)) ;
#91950=CARTESIAN_POINT('Ctrl Pts',(-20.8529948357394,50.3197612644119,122.978175098663)) ;
#91951=CARTESIAN_POINT('Ctrl Pts',(-20.9058575761444,50.3296248081375,123.231923138614)) ;
#91952=CARTESIAN_POINT('Ctrl Pts',(-20.9146380480463,50.3395935218076,123.493747759478)) ;
#91953=CARTESIAN_POINT('Ctrl Pts',(-20.8648603610188,50.3529392692113,123.840886646443)) ;
#91954=CARTESIAN_POINT('Ctrl Pts',(-20.7281950716831,50.366089824284,124.162613928907)) ;
#91955=CARTESIAN_POINT('Ctrl Pts',(-20.5118305427497,50.3794752048338,124.439920066173)) ;
#91956=CARTESIAN_POINT('Ctrl Pts',(-20.3188172284818,50.3893631408267,124.613934022329)) ;
#91957=CARTESIAN_POINT('Ctrl Pts',(-20.0965116250302,50.3993543306393,124.753570663319)) ;
#91958=CARTESIAN_POINT('Ctrl Pts',(-19.8542622927966,50.4093064291776,124.852232186328)) ;
#91959=CARTESIAN_POINT('Ctrl Pts',(-19.5961633789181,50.4193526856281,124.907673196293)) ;
#91960=CARTESIAN_POINT('Ctrl Pts',(-19.3375104748675,50.4292021330222,124.917455726656)) ;
#91961=CARTESIAN_POINT('Ctrl Pts',(-19.0780426601325,50.4391647855174,124.882591527256)) ;
#91962=CARTESIAN_POINT('Ctrl Pts',(-18.8271559377994,50.4491878711595,124.802384290233)) ;
#91963=CARTESIAN_POINT('Ctrl Pts',(-18.5961209801117,50.4591129869164,124.681281420803)) ;
#91964=CARTESIAN_POINT('Ctrl Pts',(-18.3870807334424,50.4691654653163,124.519806842714)) ;
#91965=CARTESIAN_POINT('Ctrl Pts',(-18.2126501072753,50.479016964019,124.32847873655)) ;
#91966=CARTESIAN_POINT('Ctrl Pts',(-18.0718501454337,50.4889887032215,124.107511530402)) ;
#91967=CARTESIAN_POINT('Ctrl Pts',(-17.9713211447881,50.4989839109872,123.864801095388)) ;
#91968=CARTESIAN_POINT('Ctrl Pts',(-17.9145692121074,50.5090179124563,123.607321569366)) ;
#91969=CARTESIAN_POINT('Ctrl Pts',(-17.9031710447773,50.5188732705486,123.348557997671)) ;
#91970=CARTESIAN_POINT('Ctrl Pts',(-17.9370086645265,50.5288727461419,123.088017414384)) ;
#91971=CARTESIAN_POINT('Ctrl Pts',(-18.0144915110239,50.538767194637,122.839763225874)) ;
#91972=CARTESIAN_POINT('Ctrl Pts',(-18.1359636490848,50.5488303188647,122.604915926376)) ;
#91973=CARTESIAN_POINT('Ctrl Pts',(-18.2926316435237,50.5586699451933,122.399152962944)) ;
#91974=CARTESIAN_POINT('Ctrl Pts',(-18.486678321847,50.5687331802363,122.219538927624)) ;
#91975=CARTESIAN_POINT('Ctrl Pts',(-18.7053988201739,50.5786271854703,122.078904883828)) ;
#91976=CARTESIAN_POINT('Ctrl Pts',(-18.9460659097001,50.5885698986861,121.977250669726)) ;
#91977=CARTESIAN_POINT('Ctrl Pts',(-19.2023861460661,50.5985756384843,121.918495735838)) ;
#91978=CARTESIAN_POINT('Ctrl Pts',(-19.4653940518091,50.6085965406307,121.9054168295)) ;
#91979=CARTESIAN_POINT('Ctrl Pts',(-19.7233358092848,50.6184873106796,121.937482828107)) ;
#91980=CARTESIAN_POINT('Ctrl Pts',(-19.9744185614306,50.6284787214593,122.014246082198)) ;
#91981=CARTESIAN_POINT('Ctrl Pts',(-20.2073144805598,50.6384270671238,122.133004263277)) ;
#91982=CARTESIAN_POINT('Ctrl Pts',(-20.4163335012571,50.648371925185,122.289918302436)) ;
#91983=CARTESIAN_POINT('Ctrl Pts',(-20.5965902441456,50.6584267605779,122.483081634732)) ;
#91984=CARTESIAN_POINT('Ctrl Pts',(-20.7376425347096,50.6682491326794,122.69928261909)) ;
#91985=CARTESIAN_POINT('Ctrl Pts',(-20.8418429067607,50.6783050001231,122.942107997445)) ;
#91986=CARTESIAN_POINT('Ctrl Pts',(-20.9011591134657,50.688245729981,123.196526972203)) ;
#91987=CARTESIAN_POINT('Ctrl Pts',(-20.9161606255222,50.6981500685321,123.456374885143)) ;
#91988=CARTESIAN_POINT('Ctrl Pts',(-20.8852161971234,50.7081967499607,123.718548743211)) ;
#91989=CARTESIAN_POINT('Ctrl Pts',(-20.8105731784495,50.7180922574299,123.967693866746)) ;
#91990=CARTESIAN_POINT('Ctrl Pts',(-20.6918696445542,50.7281545259285,124.203934788214)) ;
#91991=CARTESIAN_POINT('Ctrl Pts',(-20.5374931111289,50.7379965161991,124.411487122097)) ;
#91992=CARTESIAN_POINT('Ctrl Pts',(-20.3469886042085,50.7479899330801,124.592192301977)) ;
#91993=CARTESIAN_POINT('Ctrl Pts',(-20.129467915059,50.7579144209322,124.736132155614)) ;
#91994=CARTESIAN_POINT('Ctrl Pts',(-19.8886030526091,50.7679140548407,124.841138181418)) ;
#91995=CARTESIAN_POINT('Ctrl Pts',(-19.6334526076263,50.7779001650975,124.902666745097)) ;
#91996=CARTESIAN_POINT('Ctrl Pts',(-19.370234794874,50.7879361162846,124.9187595243)) ;
#91997=CARTESIAN_POINT('Ctrl Pts',(-19.1128081761444,50.7977927546194,124.889819939285)) ;
#91998=CARTESIAN_POINT('Ctrl Pts',(-18.8606967834269,50.8077917146974,124.815928138923)) ;
#91999=CARTESIAN_POINT('Ctrl Pts',(-18.6274830798784,50.8176869450112,124.700806449973)) ;
#92000=CARTESIAN_POINT('Ctrl Pts',(-18.4143788196718,50.8277474574798,124.544393204072)) ;
#92001=CARTESIAN_POINT('Ctrl Pts',(-18.2353627908807,50.837596749026,124.357426939128)) ;
#92002=CARTESIAN_POINT('Ctrl Pts',(-18.0883925533693,50.8476239349582,124.138724931857)) ;
#92003=CARTESIAN_POINT('Ctrl Pts',(-17.9822394761601,50.8576524714175,123.897495737677)) ;
#92004=CARTESIAN_POINT('Ctrl Pts',(-17.9202588837812,50.8674977113825,123.646321073152)) ;
#92005=CARTESIAN_POINT('Ctrl Pts',(-17.9018714931078,50.8774884063057,123.384414305504)) ;
#92006=CARTESIAN_POINT('Ctrl Pts',(-17.9299486548859,50.8875262270643,123.122130520275)) ;
#92007=CARTESIAN_POINT('Ctrl Pts',(-18.0013103641566,50.8973708208412,122.873455872908)) ;
#92008=CARTESIAN_POINT('Ctrl Pts',(-18.1158568183376,50.9073548162173,122.637438180659)) ;
#92009=CARTESIAN_POINT('Ctrl Pts',(-18.2691496553917,50.9173038647787,122.425625938668)) ;
#92010=CARTESIAN_POINT('Ctrl Pts',(-18.4576995104374,50.9273063037532,122.242469851909)) ;
#92011=CARTESIAN_POINT('Ctrl Pts',(-18.675790127976,50.9373275450496,122.094857283506)) ;
#92012=CARTESIAN_POINT('Ctrl Pts',(-18.9129857115445,50.9472202234891,121.988448302435)) ;
#92013=CARTESIAN_POINT('Ctrl Pts',(-19.1674288630117,50.9572102774367,121.923807401294)) ;
#92014=CARTESIAN_POINT('Ctrl Pts',(-19.42840760001,50.9671686385852,121.904576356759)) ;
#92015=CARTESIAN_POINT('Ctrl Pts',(-19.6873151025459,50.97706826547,121.930161648276)) ;
#92016=CARTESIAN_POINT('Ctrl Pts',(-19.9415317404535,50.9871161622734,122.001441737826)) ;
#92017=CARTESIAN_POINT('Ctrl Pts',(-20.1760473918664,50.9970115199094,122.11388903272)) ;
#92018=CARTESIAN_POINT('Ctrl Pts',(-20.3909934475873,51.0070731723661,122.267820853643)) ;
#92019=CARTESIAN_POINT('Ctrl Pts',(-20.5720124432176,51.016917776638,122.452660571482)) ;
#92020=CARTESIAN_POINT('Ctrl Pts',(-20.7206679475832,51.026877898336,122.668085454437)) ;
#92021=CARTESIAN_POINT('Ctrl Pts',(-20.8300463265181,51.0369159326985,122.908118283207)) ;
#92022=CARTESIAN_POINT('Ctrl Pts',(-20.8954797450795,51.046790245285,123.159253141407)) ;
#92023=CARTESIAN_POINT('Ctrl Pts',(-20.9167078074931,51.0568597260677,123.422979437591)) ;
#92024=CARTESIAN_POINT('Ctrl Pts',(-20.8925366127019,51.0666940620848,123.68030532245)) ;
#92025=CARTESIAN_POINT('Ctrl Pts',(-20.8233738618489,51.076727019813,123.934719313341)) ;
#92026=CARTESIAN_POINT('Ctrl Pts',(-20.7105654023123,51.0867474183882,124.172661102908)) ;
#92027=CARTESIAN_POINT('Ctrl Pts',(-20.5610356799522,51.0966129921594,124.384475866047)) ;
#92028=CARTESIAN_POINT('Ctrl Pts',(-20.3732440668846,51.1066818668155,124.570842766502)) ;
#92029=CARTESIAN_POINT('Ctrl Pts',(-20.1607562670967,51.116527297721,124.718478795522)) ;
#92030=CARTESIAN_POINT('Ctrl Pts',(-19.9230357260641,51.1265069225917,124.829213605734)) ;
#92031=CARTESIAN_POINT('Ctrl Pts',(-19.6685786829973,51.1365256055058,124.896772999361)) ;
#92032=CARTESIAN_POINT('Ctrl Pts',(-19.4098095174621,51.1464088706896,124.919373434)) ;
#92033=CARTESIAN_POINT('Ctrl Pts',(-19.1462888986317,51.156477164781,124.896167375007)) ;
#92034=CARTESIAN_POINT('Ctrl Pts',(-18.8966808735186,51.1663072949663,124.829451529774)) ;
#92035=CARTESIAN_POINT('Ctrl Pts',(-18.6567504696124,51.1763738431815,124.718134366409)) ;
#92036=CARTESIAN_POINT('Ctrl Pts',(-18.4436238223543,51.1862640918701,124.569323332905)) ;
#92037=CARTESIAN_POINT('Ctrl Pts',(-18.2573048544974,51.1962562736461,124.384316168399)) ;
#92038=CARTESIAN_POINT('Ctrl Pts',(-18.1065797448196,51.2062190542739,124.170249228209)) ;
#92039=CARTESIAN_POINT('Ctrl Pts',(-17.9953654455778,51.2161234589477,123.934908116965)) ;
#92040=CARTESIAN_POINT('Ctrl Pts',(-17.925826600637,51.2261834534267,123.679876469333)) ;
#92041=CARTESIAN_POINT('Ctrl Pts',(-17.9019091868143,51.2360320753965,123.422152612981)) ;
#92042=CARTESIAN_POINT('Ctrl Pts',(-17.9229023529744,51.2460625148083,123.15941586086)) ;
#92043=CARTESIAN_POINT('Ctrl Pts',(-17.9895839704234,51.2560722304431,122.904933300777)) ;
#92044=CARTESIAN_POINT('Ctrl Pts',(-18.0981009034146,51.2659829831357,122.668199754966)) ;
#92045=CARTESIAN_POINT('Ctrl Pts',(-18.2458319639415,51.2759122560821,122.453101902059)) ;
#92046=CARTESIAN_POINT('Ctrl Pts',(-18.4308984169478,51.2859549474748,122.264969338689)) ;
#92047=CARTESIAN_POINT('Ctrl Pts',(-18.6424005039535,51.2958414806923,122.114056148567)) ;
#92048=CARTESIAN_POINT('Ctrl Pts',(-18.8792033416488,51.3058346256243,122.000563484601)) ;
#92049=CARTESIAN_POINT('Ctrl Pts',(-19.1309552845419,51.3157803064608,121.930339339444)) ;
#92050=CARTESIAN_POINT('Ctrl Pts',(-19.3910775718894,51.3257275636094,121.904356869132)) ;
#92051=CARTESIAN_POINT('Ctrl Pts',(-19.6543533589848,51.3357754674813,121.924427076619)) ;
#92052=CARTESIAN_POINT('Ctrl Pts',(-19.9051120288232,51.3456231665793,121.988392795178)) ;
#92053=CARTESIAN_POINT('Ctrl Pts',(-20.144008897239,51.355584657558,122.095399647996)) ;
#92054=CARTESIAN_POINT('Ctrl Pts',(-20.3619945141337,51.3656141199719,122.24356719647)) ;
#92055=CARTESIAN_POINT('Ctrl Pts',(-20.5487308944332,51.3755213510718,122.424986082512)) ;
#92056=CARTESIAN_POINT('Ctrl Pts',(-20.7021540436023,51.3854677297493,122.636582411564)) ;
#92057=CARTESIAN_POINT('Ctrl Pts',(-20.8172786899295,51.3954724985581,122.872977021104)) ;
#92058=CARTESIAN_POINT('Ctrl Pts',(-20.889429832364,51.4054936195783,123.126239425325)) ;
#92059=CARTESIAN_POINT('Ctrl Pts',(-20.9164566681768,51.4153844854309,123.384761481474)) ;
#92060=CARTESIAN_POINT('Ctrl Pts',(-20.8983887932973,51.4253752941902,123.646672004827)) ;
#92061=CARTESIAN_POINT('Ctrl Pts',(-20.835318400747,51.4353259523705,123.900458111221)) ;
#92062=CARTESIAN_POINT('Ctrl Pts',(-20.7296282507546,51.4452621620126,124.139202828454)) ;
#92063=CARTESIAN_POINT('Ctrl Pts',(-20.5836546019347,51.4552453287375,124.357227797165)) ;
#92064=CARTESIAN_POINT('Ctrl Pts',(-20.4006303942084,51.4652891259478,124.547361584233)) ;
#92065=CARTESIAN_POINT('Ctrl Pts',(-20.192254850081,51.4751173421161,124.700025669877)) ;
#92066=CARTESIAN_POINT('Ctrl Pts',(-19.9548227665226,51.4851939095853,124.81714527759)) ;
#92067=CARTESIAN_POINT('Ctrl Pts',(-19.7062541409025,51.4950459952747,124.889764801909)) ;
#92068=CARTESIAN_POINT('Ctrl Pts',(-19.4431990726262,51.5051192626801,124.918970553885)) ;
#92069=CARTESIAN_POINT('Ctrl Pts',(-19.1850914917787,51.5149606791037,124.902372431121)) ;
#92070=CARTESIAN_POINT('Ctrl Pts',(-18.9305244646705,51.5249219372464,124.841424401148)) ;
#92071=CARTESIAN_POINT('Ctrl Pts',(-18.6887877930121,51.5349586136784,124.735942523709)) ;
#92072=CARTESIAN_POINT('Ctrl Pts',(-18.4722292764915,51.5448372215422,124.592733444186)) ;
#92073=CARTESIAN_POINT('Ctrl Pts',(-18.2803671864941,51.554897450181,124.410900084706)) ;
#92074=CARTESIAN_POINT('Ctrl Pts',(-18.1259134655434,51.5647644343418,124.202585813997)) ;
#92075=CARTESIAN_POINT('Ctrl Pts',(-18.0079247984675,51.5747700005945,123.96764851309)) ;
#92076=CARTESIAN_POINT('Ctrl Pts',(-17.9327258735387,51.5847537890091,123.716244471843)) ;
#92077=CARTESIAN_POINT('Ctrl Pts',(-17.9024259130523,51.5947996458117,123.454016015245)) ;
#92078=CARTESIAN_POINT('Ctrl Pts',(-17.917439480721,51.6046255230277,123.196237952779)) ;
#92079=CARTESIAN_POINT('Ctrl Pts',(-17.9771454730441,51.614615998869,122.940577894991)) ;
#92080=CARTESIAN_POINT('Ctrl Pts',(-18.0815215144472,51.6246595747678,122.698158310666)) ;
#92081=CARTESIAN_POINT('Ctrl Pts',(-18.2227516785276,51.6344813670658,122.482120314041)) ;
#92082=CARTESIAN_POINT('Ctrl Pts',(-18.40270986864,51.6445163326917,122.289358503398)) ;
#92083=CARTESIAN_POINT('Ctrl Pts',(-18.6136393360001,51.6545412496248,122.13151278075)) ;
#92084=CARTESIAN_POINT('Ctrl Pts',(-18.8444580637235,51.6643931880009,122.014234397312)) ;
#92085=CARTESIAN_POINT('Ctrl Pts',(-19.0954754548516,51.6743841640256,121.9373786769)) ;
#92086=CARTESIAN_POINT('Ctrl Pts',(-19.3541618616858,51.6843019848293,121.905328500858)) ;
#92087=CARTESIAN_POINT('Ctrl Pts',(-19.617334158459,51.6943307053939,121.918784864329)) ;
#92088=CARTESIAN_POINT('Ctrl Pts',(-19.8705294306841,51.7042136320031,121.976713058442)) ;
#92089=CARTESIAN_POINT('Ctrl Pts',(-20.1128710137296,51.7142179171226,122.078557970596)) ;
#92090=CARTESIAN_POINT('Ctrl Pts',(-20.3334390737872,51.7242015983304,122.220706430317)) ;
#92091=CARTESIAN_POINT('Ctrl Pts',(-20.526827334217,51.7342425970603,122.400195572372)) ;
#92092=CARTESIAN_POINT('Ctrl Pts',(-20.6831082514724,51.7440750419275,122.60596620502)) ;
#92093=CARTESIAN_POINT('Ctrl Pts',(-20.8039234261917,51.7540700403578,122.839180993671)) ;
#92094=CARTESIAN_POINT('Ctrl Pts',(-20.8821642141018,51.7641015891074,123.090935669259)) ;
#92095=CARTESIAN_POINT('Ctrl Pts',(-20.915271599229,51.7739669674129,123.348051007155)) ;
#92096=CARTESIAN_POINT('Ctrl Pts',(-20.9038525681082,51.7839288148732,123.609596824492)) ;
#92097=CARTESIAN_POINT('Ctrl Pts',(-20.8463633745007,51.7939637556874,123.866947061797)) ;
#92098=CARTESIAN_POINT('Ctrl Pts',(-20.7469611887257,51.8038487167046,124.106982513468)) ;
#92099=CARTESIAN_POINT('Ctrl Pts',(-20.6048348390858,51.8139143256234,124.330017808425)) ;
#92100=CARTESIAN_POINT('Ctrl Pts',(-20.4302962655908,51.8237535006651,124.520838097593)) ;
#92101=CARTESIAN_POINT('Ctrl Pts',(-20.2209018146829,51.833816056165,124.682277389154)) ;
#92102=CARTESIAN_POINT('Ctrl Pts',(-19.9903358407335,51.843713230858,124.802662438006)) ;
#92103=CARTESIAN_POINT('Ctrl Pts',(-19.7418135968401,51.8536439457813,124.882280836008)) ;
#92104=CARTESIAN_POINT('Ctrl Pts',(-19.4802517626863,51.8636879738589,124.917639362177)) ;
#92105=CARTESIAN_POINT('Ctrl Pts',(-19.2206361067492,51.8735741757122,124.907413635339)) ;
#92106=CARTESIAN_POINT('Ctrl Pts',(-18.9639533078119,51.8835673421791,124.852066742979)) ;
#92107=CARTESIAN_POINT('Ctrl Pts',(-18.7220007871068,51.8935068131662,124.753573074232)) ;
#92108=CARTESIAN_POINT('Ctrl Pts',(-18.4991343218233,51.9035233275204,124.613563016952)) ;
#92109=CARTESIAN_POINT('Ctrl Pts',(-18.3054534957154,51.9134533539972,124.438628708333)) ;
#92110=CARTESIAN_POINT('Ctrl Pts',(-18.1432387360808,51.9235058895067,124.230157322887)) ;
#92111=CARTESIAN_POINT('Ctrl Pts',(-18.02207359166,51.9333522927264,124.001515921378)) ;
#92112=CARTESIAN_POINT('Ctrl Pts',(-17.9407164669733,51.9433143355804,123.752702026381)) ;
#92113=CARTESIAN_POINT('Ctrl Pts',(-17.9038854280585,51.9533428863711,123.491731120395)) ;
#92114=CARTESIAN_POINT('Ctrl Pts',(-17.912731672611,51.9632532120887,123.231460267867)) ;
#92115=CARTESIAN_POINT('Ctrl Pts',(-17.966105221735,51.9731881239183,122.975886847945)) ;
#92116=CARTESIAN_POINT('Ctrl Pts',(-18.0642983867156,51.9832291306864,122.730978652853)) ;
#92117=CARTESIAN_POINT('Ctrl Pts',(-18.2012613019034,51.9931167635186,122.510155194213)) ;
#92118=CARTESIAN_POINT('Ctrl Pts',(-18.3759219646091,52.0031071946166,122.314162879866)) ;
#92119=CARTESIAN_POINT('Ctrl Pts',(-18.5813424888858,52.0130626311739,122.152141812982)) ;
#92120=CARTESIAN_POINT('Ctrl Pts',(-18.8104988520299,52.0229735792732,122.028393562061)) ;
#92121=CARTESIAN_POINT('Ctrl Pts',(-19.0601248152919,52.0329856553709,121.945174289692)) ;
#92122=CARTESIAN_POINT('Ctrl Pts',(-19.3208342889526,52.0430129774459,121.907035972771)) ;
#92123=CARTESIAN_POINT('Ctrl Pts',(-19.5798702658014,52.0528717524,121.913965038983)) ;
#92124=CARTESIAN_POINT('Ctrl Pts',(-19.9254189752122,52.0662979452124,121.984776021455)) ;
#92125=CARTESIAN_POINT('Ctrl Pts',(-20.2369069489131,52.0793819609939,122.139699278538)) ;
#92126=CARTESIAN_POINT('Ctrl Pts',(-20.5025007000134,52.0928554097491,122.373739586692)) ;
#92127=CARTESIAN_POINT('Ctrl Pts',(-20.663502478955,52.1026883675549,122.575893701772)) ;
#92128=CARTESIAN_POINT('Ctrl Pts',(-20.7895447714591,52.1126516410056,122.80536324698)) ;
#92129=CARTESIAN_POINT('Ctrl Pts',(-20.8739174433946,52.1226887148236,123.055264793137)) ;
#92130=CARTESIAN_POINT('Ctrl Pts',(-20.913466812998,52.1325637178352,123.311769299998)) ;
#92131=CARTESIAN_POINT('Ctrl Pts',(-20.907759863983,52.1426313974614,123.576238886036)) ;
#92132=CARTESIAN_POINT('Ctrl Pts',(-20.8575136474615,52.1524722476791,123.829949405008)) ;
#92133=CARTESIAN_POINT('Ctrl Pts',(-20.7314604670083,52.1658084461551,124.156927153833)) ;
#92134=CARTESIAN_POINT('Ctrl Pts',(-20.5246587062285,52.1790259699695,124.440942087782)) ;
#92135=CARTESIAN_POINT('Ctrl Pts',(-20.2524006445835,52.1923608964608,124.661535277277)) ;
#92136=CARTESIAN_POINT('Ctrl Pts',(-20.0229908221438,52.2023439970554,124.788885516254)) ;
#92137=CARTESIAN_POINT('Ctrl Pts',(-19.7733578676333,52.212388772955,124.874606471109)) ;
#92138=CARTESIAN_POINT('Ctrl Pts',(-19.5185625305117,52.2222066961409,124.91526712013)) ;
#92139=CARTESIAN_POINT('Ctrl Pts',(-19.2545108614186,52.2322560100963,124.911509845062)) ;
#92140=CARTESIAN_POINT('Ctrl Pts',(-18.9112692834644,52.2455597507188,124.845226243308)) ;
#92141=CARTESIAN_POINT('Ctrl Pts',(-18.5163692561841,52.2620499461955,124.6549048869)) ;
#92142=CARTESIAN_POINT('Ctrl Pts',(-18.2061367720864,52.2787691111201,124.336934261931)) ;
#92143=CARTESIAN_POINT('Ctrl Pts',(-18.0368883651409,52.2919301047903,124.035235554106)) ;
#92144=CARTESIAN_POINT('Ctrl Pts',(-17.9492083451138,52.3019263268955,123.78763251036)) ;
#92145=CARTESIAN_POINT('Ctrl Pts',(-17.9063157112242,52.3119501664292,123.527728946304)) ;
#92146=CARTESIAN_POINT('Ctrl Pts',(-17.9093488352234,52.3251434884225,123.181008469196)) ;
#92147=CARTESIAN_POINT('Ctrl Pts',(-18.0271239216375,52.3418026601998,122.754229453944)) ;
#92148=CARTESIAN_POINT('Ctrl Pts',(-18.3339431995994,52.3617128356855,122.323055504623)) ;
#92149=CARTESIAN_POINT('Ctrl Pts',(-18.7684450300349,52.3816028235299,122.021837292416)) ;
#92150=CARTESIAN_POINT('Ctrl Pts',(-19.2825994094008,52.4016082715447,121.886694009092)) ;
#92151=CARTESIAN_POINT('Ctrl Pts',(-19.8078170341868,52.421444665572,121.934185674863)) ;
#92152=CARTESIAN_POINT('Ctrl Pts',(-20.289256959109,52.4414524594687,122.159679285256)) ;
#92153=CARTESIAN_POINT('Ctrl Pts',(-20.6617455226346,52.4612790957627,122.532558034168)) ;
#92154=CARTESIAN_POINT('Ctrl Pts',(-20.8871676648136,52.4812580387165,123.013320567925)) ;
#92155=CARTESIAN_POINT('Ctrl Pts',(-20.9339425757462,52.5011898405856,123.540934620001)) ;
#92156=CARTESIAN_POINT('Ctrl Pts',(-20.8002546271562,52.5210141410831,124.050758632293)) ;
#92157=CARTESIAN_POINT('Ctrl Pts',(-20.495952731629,52.5411101424229,124.489450915891)) ;
#92158=CARTESIAN_POINT('Ctrl Pts',(-20.0674306833606,52.5608685585269,124.793545669361)) ;
#92159=CARTESIAN_POINT('Ctrl Pts',(-19.5529252626636,52.580962251411,124.935529369241)) ;
#92160=CARTESIAN_POINT('Ctrl Pts',(-19.2053368719646,52.5940732173177,124.907896808842)) ;
#92161=CARTESIAN_POINT('Ctrl Pts',(-19.0351230767564,52.6007865921055,124.864328531831)) ;
#92162=CARTESIAN_POINT('Ctrl Pts',(-20.5445227346514,11.6199309704797,123.023213403245)) ;
#92163=CARTESIAN_POINT('Ctrl Pts',(-20.5894944903278,11.6265578212978,123.154538008635)) ;
#92164=CARTESIAN_POINT('Ctrl Pts',(-20.6334264846015,11.6397884477788,123.432369762605)) ;
#92165=CARTESIAN_POINT('Ctrl Pts',(-20.5528870652718,11.6597640690375,123.849424031788)) ;
#92166=CARTESIAN_POINT('Ctrl Pts',(-20.335194670966,11.6796814039394,124.212661043596)) ;
#92167=CARTESIAN_POINT('Ctrl Pts',(-20.0078996672985,11.6995546806554,124.480006178853)) ;
#92168=CARTESIAN_POINT('Ctrl Pts',(-19.6059595960299,11.7195791708194,124.620366670198)) ;
#92169=CARTESIAN_POINT('Ctrl Pts',(-19.1834847167275,11.7394470119701,124.615091675808)) ;
#92170=CARTESIAN_POINT('Ctrl Pts',(-18.7864894845612,11.7593926628497,124.466037547562)) ;
#92171=CARTESIAN_POINT('Ctrl Pts',(-18.4649119653887,11.7792980634666,124.190860821467)) ;
#92172=CARTESIAN_POINT('Ctrl Pts',(-18.2561386171959,11.799172291283,123.823451738956)) ;
#92173=CARTESIAN_POINT('Ctrl Pts',(-18.1848458737542,11.8191580821606,123.404512084067)) ;
#92174=CARTESIAN_POINT('Ctrl Pts',(-18.2606755610484,11.8390523248204,122.988387677173)) ;
#92175=CARTESIAN_POINT('Ctrl Pts',(-18.4728669365122,11.8589310408924,122.622775076827)) ;
#92176=CARTESIAN_POINT('Ctrl Pts',(-18.799957735148,11.878970490737,122.349782358275)) ;
#92177=CARTESIAN_POINT('Ctrl Pts',(-19.1972060310392,11.8988336522749,122.205994913541)) ;
#92178=CARTESIAN_POINT('Ctrl Pts',(-19.6218870457641,11.9188130202891,122.20615905977)) ;
#92179=CARTESIAN_POINT('Ctrl Pts',(-20.0180120514052,11.9386236008119,122.34965257654)) ;
#92180=CARTESIAN_POINT('Ctrl Pts',(-20.3444465319008,11.9586045290975,122.621438236603)) ;
#92181=CARTESIAN_POINT('Ctrl Pts',(-20.5574196891661,11.9784972009669,122.986936080641)) ;
#92182=CARTESIAN_POINT('Ctrl Pts',(-20.6337267052267,11.9984235312541,123.403693647051)) ;
#92183=CARTESIAN_POINT('Ctrl Pts',(-20.5626962506009,12.0183940853463,123.822338761092)) ;
#92184=CARTESIAN_POINT('Ctrl Pts',(-20.3894978612787,12.034925924434,124.128191012563)) ;
#92185=CARTESIAN_POINT('Ctrl Pts',(-20.1931346813434,12.0482656632615,124.328472306739)) ;
#92186=CARTESIAN_POINT('Ctrl Pts',(-20.0213926302728,12.0582979054801,124.450877152138)) ;
#92187=CARTESIAN_POINT('Ctrl Pts',(-19.8344383779008,12.0681556061236,124.540321539624)) ;
#92188=CARTESIAN_POINT('Ctrl Pts',(-19.6322019782122,12.0781474707628,124.597064388761)) ;
#92189=CARTESIAN_POINT('Ctrl Pts',(-19.4246153322092,12.088070020523,124.617642787167)) ;
#92190=CARTESIAN_POINT('Ctrl Pts',(-19.1462130031105,12.1013477940164,124.597251023731)) ;
#92191=CARTESIAN_POINT('Ctrl Pts',(-18.8783247840957,12.114695132957,124.503674877243)) ;
#92192=CARTESIAN_POINT('Ctrl Pts',(-18.6486087161095,12.1279023647502,124.347609590522)) ;
#92193=CARTESIAN_POINT('Ctrl Pts',(-18.4978177422815,12.1378894808399,124.201561840989)) ;
#92194=CARTESIAN_POINT('Ctrl Pts',(-18.3749666561639,12.1478403864197,124.032184068499)) ;
#92195=CARTESIAN_POINT('Ctrl Pts',(-18.2826817593171,12.1578954884271,123.842034948984)) ;
#92196=CARTESIAN_POINT('Ctrl Pts',(-18.2257950816562,12.1677171617482,123.643518261886)) ;
#92197=CARTESIAN_POINT('Ctrl Pts',(-18.2033811742633,12.1777756328231,123.433271579607)) ;
#92198=CARTESIAN_POINT('Ctrl Pts',(-18.2179067683536,12.1877002439996,123.225110804427)) ;
#92199=CARTESIAN_POINT('Ctrl Pts',(-18.2846782998038,12.2009775829,122.954100941105)) ;
#92200=CARTESIAN_POINT('Ctrl Pts',(-18.4211173081076,12.2142764621376,122.706459212318)) ;
#92201=CARTESIAN_POINT('Ctrl Pts',(-18.6137339222405,12.2275153343083,122.505496739314)) ;
#92202=CARTESIAN_POINT('Ctrl Pts',(-18.7832480718907,12.2375219524449,122.380910624351)) ;
#92203=CARTESIAN_POINT('Ctrl Pts',(-18.9724531322104,12.2475528975064,122.28779225172)) ;
#92204=CARTESIAN_POINT('Ctrl Pts',(-19.1713357060114,12.2574090708583,122.229594631958)) ;
#92205=CARTESIAN_POINT('Ctrl Pts',(-19.3802130015109,12.2674083418211,122.206224196306)) ;
#92206=CARTESIAN_POINT('Ctrl Pts',(-19.587865646609,12.2773027935785,122.21909984271)) ;
#92207=CARTESIAN_POINT('Ctrl Pts',(-19.7934896821476,12.2873661093878,122.268715027323)) ;
#92208=CARTESIAN_POINT('Ctrl Pts',(-19.9832142650933,12.2972049661274,122.351202095469)) ;
#92209=CARTESIAN_POINT('Ctrl Pts',(-20.1597895100835,12.307271087945,122.467780803607)) ;
#92210=CARTESIAN_POINT('Ctrl Pts',(-20.3106265987992,12.3171543156693,122.610717010097)) ;
#92211=CARTESIAN_POINT('Ctrl Pts',(-20.4360240844988,12.3271437769481,122.779153372951)) ;
#92212=CARTESIAN_POINT('Ctrl Pts',(-20.5299739138694,12.3371074873745,122.966382465082)) ;
#92213=CARTESIAN_POINT('Ctrl Pts',(-20.5903897233038,12.3471024901054,123.167652551721)) ;
#92214=CARTESIAN_POINT('Ctrl Pts',(-20.6147102753088,12.3571388211157,123.377230955125)) ;
#92215=CARTESIAN_POINT('Ctrl Pts',(-20.6028463785135,12.366985050458,123.583902306401)) ;
#92216=CARTESIAN_POINT('Ctrl Pts',(-20.55499669517,12.3769705487333,123.78826882071)) ;
#92217=CARTESIAN_POINT('Ctrl Pts',(-20.4729187867284,12.3869054517162,123.980370474057)) ;
#92218=CARTESIAN_POINT('Ctrl Pts',(-20.357202174755,12.3969629548115,124.157299802648)) ;
#92219=CARTESIAN_POINT('Ctrl Pts',(-20.2161112271615,12.406784611182,124.308089113549)) ;
#92220=CARTESIAN_POINT('Ctrl Pts',(-20.0473094933482,12.4168406738471,124.435340831555)) ;
#92221=CARTESIAN_POINT('Ctrl Pts',(-19.8609443801348,12.4267813385503,124.529924426438)) ;
#92222=CARTESIAN_POINT('Ctrl Pts',(-19.661913020913,12.4366857424989,124.591112791133)) ;
#92223=CARTESIAN_POINT('Ctrl Pts',(-19.4523192188681,12.4467322274924,124.61704985095)) ;
#92224=CARTESIAN_POINT('Ctrl Pts',(-19.244505090046,12.4566284553041,124.606538219516)) ;
#92225=CARTESIAN_POINT('Ctrl Pts',(-19.038368143445,12.4666880388676,124.559383118642)) ;
#92226=CARTESIAN_POINT('Ctrl Pts',(-18.8475319973023,12.4765400485364,124.478858162415)) ;
#92227=CARTESIAN_POINT('Ctrl Pts',(-18.6712600321161,12.486502579976,124.365762071947)) ;
#92228=CARTESIAN_POINT('Ctrl Pts',(-18.5164450101254,12.4965341282154,124.2225425962)) ;
#92229=CARTESIAN_POINT('Ctrl Pts',(-18.3904774875118,12.5064255394284,124.057089554792)) ;
#92230=CARTESIAN_POINT('Ctrl Pts',(-18.293606379704,12.5164417931364,123.870112765132)) ;
#92231=CARTESIAN_POINT('Ctrl Pts',(-18.2310247401732,12.5264718959811,123.668752585858)) ;
#92232=CARTESIAN_POINT('Ctrl Pts',(-18.2044223869209,12.5363283449348,123.463240844313)) ;
#92233=CARTESIAN_POINT('Ctrl Pts',(-18.2137782919258,12.5463273557071,123.253271994429)) ;
#92234=CARTESIAN_POINT('Ctrl Pts',(-18.2587650999899,12.5562225726251,123.050131413911)) ;
#92235=CARTESIAN_POINT('Ctrl Pts',(-18.3396685918713,12.5662830879825,122.854741766294)) ;
#92236=CARTESIAN_POINT('Ctrl Pts',(-18.4508077372585,12.5761323813695,122.680014247902)) ;
#92237=CARTESIAN_POINT('Ctrl Pts',(-18.5927131357453,12.5861595570495,122.524134244484)) ;
#92238=CARTESIAN_POINT('Ctrl Pts',(-18.7599030448378,12.5961881326767,122.395673642162)) ;
#92239=CARTESIAN_POINT('Ctrl Pts',(-18.9432361413831,12.6060332262226,122.299636183444)) ;
#92240=CARTESIAN_POINT('Ctrl Pts',(-19.143231548689,12.6160244676544,122.235427961324)) ;
#92241=CARTESIAN_POINT('Ctrl Pts',(-19.3523277802074,12.6260602487976,122.207228145607)) ;
#92242=CARTESIAN_POINT('Ctrl Pts',(-19.5592861451502,12.6359124545273,122.21533000764)) ;
#92243=CARTESIAN_POINT('Ctrl Pts',(-19.7640842288228,12.6458745486443,122.259137338286)) ;
#92244=CARTESIAN_POINT('Ctrl Pts',(-19.9592496327906,12.6558971094714,122.338556576803)) ;
#92245=CARTESIAN_POINT('Ctrl Pts',(-20.1360993033801,12.665824881123,122.449432036472)) ;
#92246=CARTESIAN_POINT('Ctrl Pts',(-20.2927583986931,12.6758672652478,122.590938510581)) ;
#92247=CARTESIAN_POINT('Ctrl Pts',(-20.4205737162939,12.6857564893184,122.754925391399)) ;
#92248=CARTESIAN_POINT('Ctrl Pts',(-20.5192984754898,12.6957457374858,122.940270425406)) ;
#92249=CARTESIAN_POINT('Ctrl Pts',(-20.5839903499472,12.7057043145277,123.139379566424)) ;
#92250=CARTESIAN_POINT('Ctrl Pts',(-20.6134664462127,12.715603883619,123.345414238047)) ;
#92251=CARTESIAN_POINT('Ctrl Pts',(-20.6065457688213,12.725651795703,123.556518045616)) ;
#92252=CARTESIAN_POINT('Ctrl Pts',(-20.5638845268326,12.7355471500102,123.760161210046)) ;
#92253=CARTESIAN_POINT('Ctrl Pts',(-20.4852609822995,12.7456088005014,123.956508878827)) ;
#92254=CARTESIAN_POINT('Ctrl Pts',(-20.3761562392932,12.7554534159639,124.132387479674)) ;
#92255=CARTESIAN_POINT('Ctrl Pts',(-20.2371197672901,12.7654134948653,124.288952076224)) ;
#92256=CARTESIAN_POINT('Ctrl Pts',(-20.0714719977901,12.7754516892237,124.419691962734)) ;
#92257=CARTESIAN_POINT('Ctrl Pts',(-19.8888380147407,12.7853254046233,124.518402099819)) ;
#92258=CARTESIAN_POINT('Ctrl Pts',(-19.6879341559414,12.7953971141575,124.585176374158)) ;
#92259=CARTESIAN_POINT('Ctrl Pts',(-19.4834367028135,12.80522955461,124.615443528027)) ;
#92260=CARTESIAN_POINT('Ctrl Pts',(-19.2726059179426,12.8152613755354,124.610216782179)) ;
#92261=CARTESIAN_POINT('Ctrl Pts',(-19.066233358849,12.825281745421,124.567919596225)) ;
#92262=CARTESIAN_POINT('Ctrl Pts',(-18.8731330036246,12.8351485165548,124.492120682358)) ;
#92263=CARTESIAN_POINT('Ctrl Pts',(-18.6925009420882,12.8452192877441,124.381720161414)) ;
#92264=CARTESIAN_POINT('Ctrl Pts',(-18.5373294413364,12.8550624482657,124.244796187377)) ;
#92265=CARTESIAN_POINT('Ctrl Pts',(-18.405965860316,12.8650426814522,124.081200769751)) ;
#92266=CARTESIAN_POINT('Ctrl Pts',(-18.3049709875459,12.8750612014873,123.896379551838)) ;
#92267=CARTESIAN_POINT('Ctrl Pts',(-18.2380816514897,12.884944509871,123.699636080652)) ;
#92268=CARTESIAN_POINT('Ctrl Pts',(-18.2058768851209,12.8950127940418,123.49046826295)) ;
#92269=CARTESIAN_POINT('Ctrl Pts',(-18.2101289812869,12.9048429207095,123.283817080971)) ;
#92270=CARTESIAN_POINT('Ctrl Pts',(-18.2508798494434,12.914909492916,123.076180845837)) ;
#92271=CARTESIAN_POINT('Ctrl Pts',(-18.3258687904528,12.9247996491567,122.882224430381)) ;
#92272=CARTESIAN_POINT('Ctrl Pts',(-18.4340994943442,12.9347921767331,122.702192267854)) ;
#92273=CARTESIAN_POINT('Ctrl Pts',(-18.5716617642104,12.9447536666074,122.544287781033)) ;
#92274=CARTESIAN_POINT('Ctrl Pts',(-18.7334032826049,12.9546628884946,122.412979815522)) ;
#92275=CARTESIAN_POINT('Ctrl Pts',(-18.9180668962006,12.964711468305,122.310402911689)) ;
#92276=CARTESIAN_POINT('Ctrl Pts',(-19.1144428404073,12.974594442775,122.242506577825)) ;
#92277=CARTESIAN_POINT('Ctrl Pts',(-19.3218591967594,12.9845893539177,122.208921815214)) ;
#92278=CARTESIAN_POINT('Ctrl Pts',(-19.5325086925485,12.9946097404913,122.212159430771)) ;
#92279=CARTESIAN_POINT('Ctrl Pts',(-19.7371141602649,13.0045198443484,122.251364318688)) ;
#92280=CARTESIAN_POINT('Ctrl Pts',(-19.9323647416642,13.0144475565583,122.325127276843)) ;
#92281=CARTESIAN_POINT('Ctrl Pts',(-20.1138238542012,13.0244906663255,122.43305488188)) ;
#92282=CARTESIAN_POINT('Ctrl Pts',(-20.271392834906,13.0343770867811,122.568612045325)) ;
#92283=CARTESIAN_POINT('Ctrl Pts',(-20.4047144556346,13.0443702643867,122.730961891438)) ;
#92284=CARTESIAN_POINT('Ctrl Pts',(-20.5072674195486,13.0543159272906,122.913174162945)) ;
#92285=CARTESIAN_POINT('Ctrl Pts',(-20.5770419750784,13.0642632234958,123.110324439017)) ;
#92286=CARTESIAN_POINT('Ctrl Pts',(-20.6116395103525,13.0743109890737,123.318702092503)) ;
#92287=CARTESIAN_POINT('Ctrl Pts',(-20.609736311941,13.0841592022913,123.525730665591)) ;
#92288=CARTESIAN_POINT('Ctrl Pts',(-20.5721675728708,13.0941187750854,123.731713474569)) ;
#92289=CARTESIAN_POINT('Ctrl Pts',(-20.49849609699,13.1041553961179,123.929428907478)) ;
#92290=CARTESIAN_POINT('Ctrl Pts',(-20.3935412625952,13.1140359109283,124.108708072959)) ;
#92291=CARTESIAN_POINT('Ctrl Pts',(-20.256803522262,13.1240885622353,124.269810817987)) ;
#92292=CARTESIAN_POINT('Ctrl Pts',(-20.0967179660429,13.1339839605153,124.402720826304)) ;
#92293=CARTESIAN_POINT('Ctrl Pts',(-19.9132627916011,13.1440340822214,124.507479233927)) ;
#92294=CARTESIAN_POINT('Ctrl Pts',(-19.7176528780897,13.1539183617633,124.577663668273)) ;
#92295=CARTESIAN_POINT('Ctrl Pts',(-19.5106451886869,13.1639131430553,124.613591987952)) ;
#92296=CARTESIAN_POINT('Ctrl Pts',(-19.3014971588943,13.173860988242,124.612953430792)) ;
#92297=CARTESIAN_POINT('Ctrl Pts',(-19.0958408347169,13.1837979516294,124.576354555244)) ;
#92298=CARTESIAN_POINT('Ctrl Pts',(-18.8986217867637,13.1937809163667,124.504501871259)) ;
#92299=CARTESIAN_POINT('Ctrl Pts',(-18.7160044802564,13.2038247677823,124.398546770036)) ;
#92300=CARTESIAN_POINT('Ctrl Pts',(-18.5576688200036,13.213652969117,124.265752345939)) ;
#92301=CARTESIAN_POINT('Ctrl Pts',(-18.4214089685337,13.2237295417151,124.103605374704)) ;
#92302=CARTESIAN_POINT('Ctrl Pts',(-18.3176012012084,13.2335816217226,123.924323648453)) ;
#92303=CARTESIAN_POINT('Ctrl Pts',(-18.2447624006463,13.2436549067267,123.72550920738)) ;
#92304=CARTESIAN_POINT('Ctrl Pts',(-18.208451810443,13.2534962584372,123.521808408546)) ;
#92305=CARTESIAN_POINT('Ctrl Pts',(-18.2072839695112,13.2634577578337,123.312402302002)) ;
#92306=CARTESIAN_POINT('Ctrl Pts',(-18.2431243993998,13.2734935339637,123.104477477949)) ;
#92307=CARTESIAN_POINT('Ctrl Pts',(-18.313266330403,13.2833819606013,122.908785022229)) ;
#92308=CARTESIAN_POINT('Ctrl Pts',(-18.4173025005469,13.2933972826762,122.725719708377)) ;
#92309=CARTESIAN_POINT('Ctrl Pts',(-18.5521194854302,13.3034276315764,122.563574882499)) ;
#92310=CARTESIAN_POINT('Ctrl Pts',(-18.7097686111955,13.3132710071831,122.429528077292)) ;
#92311=CARTESIAN_POINT('Ctrl Pts',(-18.8914413302913,13.3233004440802,122.322502843686)) ;
#92312=CARTESIAN_POINT('Ctrl Pts',(-19.0891909613697,13.3333323220132,122.249169485467)) ;
#92313=CARTESIAN_POINT('Ctrl Pts',(-19.2923910333282,13.3431619451186,122.211639193978)) ;
#92314=CARTESIAN_POINT('Ctrl Pts',(-19.502393832661,13.3531514162717,122.209303795918)) ;
#92315=CARTESIAN_POINT('Ctrl Pts',(-19.7106448636121,13.3631952650341,122.244181269422)) ;
#92316=CARTESIAN_POINT('Ctrl Pts',(-19.9054181897071,13.3730169705658,122.312725988821)) ;
#92317=CARTESIAN_POINT('Ctrl Pts',(-20.0894923568458,13.3830520103936,122.415798365004)) ;
#92318=CARTESIAN_POINT('Ctrl Pts',(-20.2523425372492,13.3930767172851,122.549585325473)) ;
#92319=CARTESIAN_POINT('Ctrl Pts',(-20.3874635134863,13.4029294216258,122.706578422699)) ;
#92320=CARTESIAN_POINT('Ctrl Pts',(-20.4950348439509,13.4129175438335,122.886895979639)) ;
#92321=CARTESIAN_POINT('Ctrl Pts',(-20.5692346947087,13.4228460139408,123.081995305985)) ;
#92322=CARTESIAN_POINT('Ctrl Pts',(-20.6090140362735,13.432834991108,123.288203344706)) ;
#92323=CARTESIAN_POINT('Ctrl Pts',(-20.6120399406672,13.4428727983877,123.499202411649)) ;
#92324=CARTESIAN_POINT('Ctrl Pts',(-20.5793586418842,13.452719099251,123.703608133179)) ;
#92325=CARTESIAN_POINT('Ctrl Pts',(-20.5108933572167,13.4627448426303,123.902954077039)) ;
#92326=CARTESIAN_POINT('Ctrl Pts',(-20.4083206395446,13.4727757090693,124.087214524616)) ;
#92327=CARTESIAN_POINT('Ctrl Pts',(-20.2782096665818,13.4826130678681,124.247959027508)) ;
#92328=CARTESIAN_POINT('Ctrl Pts',(-20.1200757179898,13.4926050288019,124.386233234674)) ;
#92329=CARTESIAN_POINT('Ctrl Pts',(-19.9393814428224,13.5026373913584,124.49503121546)) ;
#92330=CARTESIAN_POINT('Ctrl Pts',(-19.7459291056501,13.5125025519328,124.569766299206)) ;
#92331=CARTESIAN_POINT('Ctrl Pts',(-19.5405428766504,13.5224644565105,124.610756191711)) ;
#92332=CARTESIAN_POINT('Ctrl Pts',(-19.3296341394368,13.5324993865863,124.615150409196)) ;
#92333=CARTESIAN_POINT('Ctrl Pts',(-19.1241882593552,13.5423843334399,124.583680283996)) ;
#92334=CARTESIAN_POINT('Ctrl Pts',(-18.9238050394512,13.5524500097513,124.515772546314)) ;
#92335=CARTESIAN_POINT('Ctrl Pts',(-18.7422738965292,13.5622889293862,124.416547647665)) ;
#92336=CARTESIAN_POINT('Ctrl Pts',(-18.5769211989035,13.5723524391207,124.284614914722)) ;
#92337=CARTESIAN_POINT('Ctrl Pts',(-18.4394438861558,13.5822460522824,124.128499673236)) ;
#92338=CARTESIAN_POINT('Ctrl Pts',(-18.3301649112488,13.5921900590958,123.950314429451)) ;
#92339=CARTESIAN_POINT('Ctrl Pts',(-18.2529317702578,13.6021910134501,123.754727546131)) ;
#92340=CARTESIAN_POINT('Ctrl Pts',(-18.2110520035819,13.6122297711424,123.547897327596)) ;
#92341=CARTESIAN_POINT('Ctrl Pts',(-18.2053814428901,13.6220539553124,123.341422778142)) ;
#92342=CARTESIAN_POINT('Ctrl Pts',(-18.2360559572279,13.6321120209118,123.132225921939)) ;
#92343=CARTESIAN_POINT('Ctrl Pts',(-18.3020120677171,13.6420420676865,122.934144610065)) ;
#92344=CARTESIAN_POINT('Ctrl Pts',(-18.4010833770443,13.6519935100237,122.749875864742)) ;
#92345=CARTESIAN_POINT('Ctrl Pts',(-18.5321101585894,13.6620403072029,122.584217084689)) ;
#92346=CARTESIAN_POINT('Ctrl Pts',(-18.6866603271967,13.671888247883,122.446457937948)) ;
#92347=CARTESIAN_POINT('Ctrl Pts',(-18.8644655503016,13.6818498792256,122.335821822434)) ;
#92348=CARTESIAN_POINT('Ctrl Pts',(-19.0602066261718,13.6918785386015,122.257452037881)) ;
#92349=CARTESIAN_POINT('Ctrl Pts',(-19.2641111645517,13.7017888414897,122.214707825771)) ;
#92350=CARTESIAN_POINT('Ctrl Pts',(-19.4728545144785,13.7117237360519,122.20745340348)) ;
#92351=CARTESIAN_POINT('Ctrl Pts',(-19.6818574037471,13.7217648347188,122.237057214757)) ;
#92352=CARTESIAN_POINT('Ctrl Pts',(-19.8795330996557,13.7316521172232,122.301367089129)) ;
#92353=CARTESIAN_POINT('Ctrl Pts',(-20.0651234113588,13.7416438577337,122.399728612142)) ;
#92354=CARTESIAN_POINT('Ctrl Pts',(-20.2301072815395,13.7515944069691,122.528359355941)) ;
#92355=CARTESIAN_POINT('Ctrl Pts',(-20.3702567984072,13.7615300846039,122.683224869918)) ;
#92356=CARTESIAN_POINT('Ctrl Pts',(-20.4821496556636,13.7715155023967,122.860862904044)) ;
#92357=CARTESIAN_POINT('Ctrl Pts',(-20.5615945408518,13.7815442952672,123.0561577358)) ;
#92358=CARTESIAN_POINT('Ctrl Pts',(-20.6054790317027,13.7914238064952,123.259164226479)) ;
#92359=CARTESIAN_POINT('Ctrl Pts',(-20.6140230823703,13.8014173431681,123.469094191305)) ;
#92360=CARTESIAN_POINT('Ctrl Pts',(-20.585445224323,13.811449611432,123.678050048262)) ;
#92361=CARTESIAN_POINT('Ctrl Pts',(-20.5225142881585,13.8213135734378,123.87566527456)) ;
#92362=CARTESIAN_POINT('Ctrl Pts',(-20.4242668998113,13.8313836347827,124.063166872024)) ;
#92363=CARTESIAN_POINT('Ctrl Pts',(-20.2978535284329,13.8412259991315,124.226991218957)) ;
#92364=CARTESIAN_POINT('Ctrl Pts',(-20.1436080829852,13.8511866716339,124.368614446249)) ;
#92365=CARTESIAN_POINT('Ctrl Pts',(-19.9655216287888,13.8612247427017,124.481821965117)) ;
#92366=CARTESIAN_POINT('Ctrl Pts',(-19.7737943270889,13.8710983576622,124.561451063385)) ;
#92367=CARTESIAN_POINT('Ctrl Pts',(-19.5671347818474,13.8811705922434,124.607418828005)) ;
#92368=CARTESIAN_POINT('Ctrl Pts',(-19.3607740702346,13.8909946106922,124.616812785889)) ;
#92369=CARTESIAN_POINT('Ctrl Pts',(-19.1509484011636,13.9010595316682,124.58986547138)) ;
#92370=CARTESIAN_POINT('Ctrl Pts',(-18.885742263977,13.914269829963,124.507190963404)) ;
#92371=CARTESIAN_POINT('Ctrl Pts',(-18.6462438685015,13.9275852766949,124.356328792661)) ;
#92372=CARTESIAN_POINT('Ctrl Pts',(-18.4564443634539,13.9408755219622,124.151228756277)) ;
#92373=CARTESIAN_POINT('Ctrl Pts',(-18.342158496396,13.9509262715693,123.973546314054)) ;
#92374=CARTESIAN_POINT('Ctrl Pts',(-18.2619972946885,13.9607388785516,123.783433874635)) ;
#92375=CARTESIAN_POINT('Ctrl Pts',(-18.2145910925196,13.9708099765458,123.577110199186)) ;
#92376=CARTESIAN_POINT('Ctrl Pts',(-18.2041343921619,13.9806995493207,123.369451365273)) ;
#92377=CARTESIAN_POINT('Ctrl Pts',(-18.2378551925476,13.993969656124,123.092490222189)) ;
#92378=CARTESIAN_POINT('Ctrl Pts',(-18.3698703473456,14.0105863430465,122.764819038362)) ;
#92379=CARTESIAN_POINT('Ctrl Pts',(-18.6050453003926,14.0271603863627,122.502296275381)) ;
#92380=CARTESIAN_POINT('Ctrl Pts',(-18.8388900954275,14.0404569537945,122.349191219826)) ;
#92381=CARTESIAN_POINT('Ctrl Pts',(-19.0327140636966,14.0504870173719,122.266120699076)) ;
#92382=CARTESIAN_POINT('Ctrl Pts',(-19.2351925600069,14.0603809092212,122.218606664563)) ;
#92383=CARTESIAN_POINT('Ctrl Pts',(-19.5133779733471,14.0736336650067,122.202020467964)) ;
#92384=CARTESIAN_POINT('Ctrl Pts',(-19.861630213909,14.0903617699992,122.274027261423)) ;
#92385=CARTESIAN_POINT('Ctrl Pts',(-20.2206980924579,14.1101926064777,122.495229552412)) ;
#92386=CARTESIAN_POINT('Ctrl Pts',(-20.4846805942354,14.1301179983678,122.82648134403)) ;
#92387=CARTESIAN_POINT('Ctrl Pts',(-20.6197806891536,14.1500432117198,123.228098261421)) ;
#92388=CARTESIAN_POINT('Ctrl Pts',(-20.6098292151628,14.1699682252049,123.651592199698)) ;
#92389=CARTESIAN_POINT('Ctrl Pts',(-20.4568502730151,14.1898446969049,124.045589490744)) ;
#92390=CARTESIAN_POINT('Ctrl Pts',(-20.1773267785576,14.2098240148138,124.365478534255)) ;
#92391=CARTESIAN_POINT('Ctrl Pts',(-19.8060955662964,14.2297570183898,124.57004462274)) ;
#92392=CARTESIAN_POINT('Ctrl Pts',(-19.3882614282935,14.2496522884175,124.635961689666)) ;
#92393=CARTESIAN_POINT('Ctrl Pts',(-18.9723460075604,14.2695736263233,124.555651033609)) ;
#92394=CARTESIAN_POINT('Ctrl Pts',(-18.6081837258384,14.2895312495895,124.337753529704)) ;
#92395=CARTESIAN_POINT('Ctrl Pts',(-18.3412613634703,14.3094110815467,124.010077065692)) ;
#92396=CARTESIAN_POINT('Ctrl Pts',(-18.2010168508074,14.3292929328436,123.611189475518)) ;
#92397=CARTESIAN_POINT('Ctrl Pts',(-18.2061577248165,14.3493639499474,123.184511236421)) ;
#92398=CARTESIAN_POINT('Ctrl Pts',(-18.3545971695844,14.3691711737005,122.790298921947)) ;
#92399=CARTESIAN_POINT('Ctrl Pts',(-18.6302230516465,14.3891523092693,122.46703788842)) ;
#92400=CARTESIAN_POINT('Ctrl Pts',(-18.9990325033521,14.4090798026085,122.258519623265)) ;
#92401=CARTESIAN_POINT('Ctrl Pts',(-19.414530819844,14.4289004639663,122.187301272222)) ;
#92402=CARTESIAN_POINT('Ctrl Pts',(-19.8347873766851,14.4489976531881,122.263805862817)) ;
#92403=CARTESIAN_POINT('Ctrl Pts',(-20.198042463916,14.4687613321965,122.475491438185)) ;
#92404=CARTESIAN_POINT('Ctrl Pts',(-20.4713802055925,14.4888186108695,122.802607800385)) ;
#92405=CARTESIAN_POINT('Ctrl Pts',(-20.6146598595421,14.5086140346169,123.198496313193)) ;
#92406=CARTESIAN_POINT('Ctrl Pts',(-20.6155549975082,14.5285776793445,123.622927843257)) ;
#92407=CARTESIAN_POINT('Ctrl Pts',(-20.4704264877456,14.5485611706186,124.022283184246)) ;
#92408=CARTESIAN_POINT('Ctrl Pts',(-20.2007731307762,14.5683686657679,124.345851921621)) ;
#92409=CARTESIAN_POINT('Ctrl Pts',(-19.8340285534317,14.588351256488,124.560210082333)) ;
#92410=CARTESIAN_POINT('Ctrl Pts',(-19.4180417092248,14.6082339104793,124.636132918058)) ;
#92411=CARTESIAN_POINT('Ctrl Pts',(-18.9996610722391,14.6281921553423,124.565621343336)) ;
#92412=CARTESIAN_POINT('Ctrl Pts',(-18.6317274635194,14.6480677423839,124.357590409106)) ;
#92413=CARTESIAN_POINT('Ctrl Pts',(-18.3552455165215,14.6680486305192,124.03505471784)) ;
#92414=CARTESIAN_POINT('Ctrl Pts',(-18.2060499281887,14.6879837716302,123.638243803978)) ;
#92415=CARTESIAN_POINT('Ctrl Pts',(-18.2009208909695,14.7078957896413,123.214931994148)) ;
#92416=CARTESIAN_POINT('Ctrl Pts',(-18.3399791205184,14.7277840078848,122.815553042048)) ;
#92417=CARTESIAN_POINT('Ctrl Pts',(-18.5625223078794,14.7443823117317,122.541718669557)) ;
#92418=CARTESIAN_POINT('Ctrl Pts',(-18.7884690167792,14.7576549016346,122.377905209627)) ;
#92419=CARTESIAN_POINT('Ctrl Pts',(-18.9775554419719,14.7676623165854,122.28567841915)) ;
#92420=CARTESIAN_POINT('Ctrl Pts',(-19.1798597979953,14.777669663318,122.227857687537)) ;
#92421=CARTESIAN_POINT('Ctrl Pts',(-19.4571939480099,14.7909360231196,122.198758994379)) ;
#92422=CARTESIAN_POINT('Ctrl Pts',(-19.8041248709221,14.8074506807426,122.253102924327)) ;
#92423=CARTESIAN_POINT('Ctrl Pts',(-20.1135388548329,14.8240481139852,122.422674400155)) ;
#92424=CARTESIAN_POINT('Ctrl Pts',(-20.31615452797,14.8373961111302,122.616914640427)) ;
#92425=CARTESIAN_POINT('Ctrl Pts',(-20.4392738972615,14.8472918654818,122.784604403516)) ;
#92426=CARTESIAN_POINT('Ctrl Pts',(-20.5324949220167,14.8572798194132,122.972739489712)) ;
#92427=CARTESIAN_POINT('Ctrl Pts',(-20.5915500287685,14.8672370431179,123.173594463917)) ;
#92428=CARTESIAN_POINT('Ctrl Pts',(-20.6149140597736,14.8772725896746,123.383260968004)) ;
#92429=CARTESIAN_POINT('Ctrl Pts',(-20.6018719765782,14.8871597009507,123.590723482903)) ;
#92430=CARTESIAN_POINT('Ctrl Pts',(-20.552821477757,14.8971511060515,123.794956581303)) ;
#92431=CARTESIAN_POINT('Ctrl Pts',(-20.4693756424494,14.9070967272663,123.98667131504)) ;
#92432=CARTESIAN_POINT('Ctrl Pts',(-20.354214645291,14.9170459755346,124.161292960662)) ;
#92433=CARTESIAN_POINT('Ctrl Pts',(-20.2089133571514,14.9270924707032,124.314566354854)) ;
#92434=CARTESIAN_POINT('Ctrl Pts',(-20.0426093916053,14.9369438134948,124.43801767961)) ;
#92435=CARTESIAN_POINT('Ctrl Pts',(-19.8554010834805,14.9469155936221,124.532309421632)) ;
#92436=CARTESIAN_POINT('Ctrl Pts',(-19.6541309256762,14.9569107935998,124.592800420983)) ;
#92437=CARTESIAN_POINT('Ctrl Pts',(-19.4446257916061,14.9669447852959,124.617258985423)) ;
#92438=CARTESIAN_POINT('Ctrl Pts',(-19.2377471565128,14.9768001902684,124.60551410532)) ;
#92439=CARTESIAN_POINT('Ctrl Pts',(-19.0330947053247,14.9867994881141,124.557625447812)) ;
#92440=CARTESIAN_POINT('Ctrl Pts',(-18.8417260095209,14.9966946007193,124.475969739033)) ;
#92441=CARTESIAN_POINT('Ctrl Pts',(-18.6645920863028,15.0067552462543,124.360440257622)) ;
#92442=CARTESIAN_POINT('Ctrl Pts',(-18.5133454930013,15.0166041232435,124.219009634951)) ;
#92443=CARTESIAN_POINT('Ctrl Pts',(-18.3862687789312,15.0266328343371,124.050778467038)) ;
#92444=CARTESIAN_POINT('Ctrl Pts',(-18.290833943396,15.0366622355932,123.8627585743)) ;
#92445=CARTESIAN_POINT('Ctrl Pts',(-18.2302119029256,15.0465024273892,123.664964952641)) ;
#92446=CARTESIAN_POINT('Ctrl Pts',(-18.2040500545488,15.0565058565822,123.456316133071)) ;
#92447=CARTESIAN_POINT('Ctrl Pts',(-18.2145657258036,15.0664913690484,123.246616906617)) ;
#92448=CARTESIAN_POINT('Ctrl Pts',(-18.26178794317,15.0765324654324,123.040892381752)) ;
#92449=CARTESIAN_POINT('Ctrl Pts',(-18.3421420908844,15.0863756613834,122.850175892976)) ;
#92450=CARTESIAN_POINT('Ctrl Pts',(-18.4556407699615,15.0963619724378,122.673598924012)) ;
#92451=CARTESIAN_POINT('Ctrl Pts',(-18.5972860801751,15.1062966576955,122.520057462546)) ;
#92452=CARTESIAN_POINT('Ctrl Pts',(-18.7655513685597,15.1163542189126,122.392067431198)) ;
#92453=CARTESIAN_POINT('Ctrl Pts',(-18.9489772358709,15.1261758605212,122.29720460344)) ;
#92454=CARTESIAN_POINT('Ctrl Pts',(-19.1506365364957,15.1362319241121,122.233796786245)) ;
#92455=CARTESIAN_POINT('Ctrl Pts',(-19.3579112071296,15.1461725998739,122.207051934719)) ;
#92456=CARTESIAN_POINT('Ctrl Pts',(-19.5659421416025,15.1560769586623,122.21601478593)) ;
#92457=CARTESIAN_POINT('Ctrl Pts',(-19.7721296999546,15.1661236132381,122.261734136403)) ;
#92458=CARTESIAN_POINT('Ctrl Pts',(-19.964427665596,15.1760192078809,122.341192189689)) ;
#92459=CARTESIAN_POINT('Ctrl Pts',(-20.1429244158312,15.1860811545378,122.454662033842)) ;
#92460=CARTESIAN_POINT('Ctrl Pts',(-20.2957651291665,15.19593077847,122.59438375581)) ;
#92461=CARTESIAN_POINT('Ctrl Pts',(-20.42401435777,15.2058940174998,122.759973307204)) ;
#92462=CARTESIAN_POINT('Ctrl Pts',(-20.5219183117083,15.2159185922756,122.946614153896)) ;
#92463=CARTESIAN_POINT('Ctrl Pts',(-20.5853737220608,15.2258371549633,123.145237954804)) ;
#92464=CARTESIAN_POINT('Ctrl Pts',(-20.6139543237281,15.2358293416873,123.35336433036)) ;
#92465=CARTESIAN_POINT('Ctrl Pts',(-20.6055500370855,15.2458641402715,123.564151637776)) ;
#92466=CARTESIAN_POINT('Ctrl Pts',(-20.561819537419,15.2557193309452,123.766687353874)) ;
#92467=CARTESIAN_POINT('Ctrl Pts',(-20.4827219328532,15.2657186790982,123.961418906488)) ;
#92468=CARTESIAN_POINT('Ctrl Pts',(-20.3723321552261,15.2756138047733,124.137780670391)) ;
#92469=CARTESIAN_POINT('Ctrl Pts',(-20.2306926442198,15.2856743477214,124.294818432688)) ;
#92470=CARTESIAN_POINT('Ctrl Pts',(-20.0674780549609,15.2955236219883,124.422264719081)) ;
#92471=CARTESIAN_POINT('Ctrl Pts',(-19.8815798759222,15.3055508465582,124.521651781092)) ;
#92472=CARTESIAN_POINT('Ctrl Pts',(-19.6810377994886,15.315579245746,124.586740132725)) ;
#92473=CARTESIAN_POINT('Ctrl Pts',(-19.4761222822697,15.3254249961595,124.615862633411)) ;
#92474=CARTESIAN_POINT('Ctrl Pts',(-19.2662142458841,15.3354137865603,124.609449914559)) ;
#92475=CARTESIAN_POINT('Ctrl Pts',(-19.0595807364649,15.34545871496,124.565927889753)) ;
#92476=CARTESIAN_POINT('Ctrl Pts',(-18.8677446724703,15.3552831997489,124.489355662704)) ;
#92477=CARTESIAN_POINT('Ctrl Pts',(-18.687818222948,15.3653405972901,124.378336136723)) ;
#92478=CARTESIAN_POINT('Ctrl Pts',(-18.5321217638704,15.3752666888763,124.239371247625)) ;
#92479=CARTESIAN_POINT('Ctrl Pts',(-18.4021311831631,15.3852214740209,124.075359071023)) ;
#92480=CARTESIAN_POINT('Ctrl Pts',(-18.3019733073139,15.3952588436785,123.889627376393)) ;
#92481=CARTESIAN_POINT('Ctrl Pts',(-18.2364143071113,15.4051476538001,123.69233545093)) ;
#92482=CARTESIAN_POINT('Ctrl Pts',(-18.2054278164718,15.4151370128512,123.48463093245)) ;
#92483=CARTESIAN_POINT('Ctrl Pts',(-18.2111153558979,15.4250955603073,123.275354647825)) ;
#92484=CARTESIAN_POINT('Ctrl Pts',(-18.2523061561099,15.4349951368583,123.071338456214)) ;
#92485=CARTESIAN_POINT('Ctrl Pts',(-18.3294907665845,15.445043048689,122.874729180045)) ;
#92486=CARTESIAN_POINT('Ctrl Pts',(-18.4378567487714,15.4549383965496,122.697113519463)) ;
#92487=CARTESIAN_POINT('Ctrl Pts',(-18.5776691245229,15.4650000730808,122.538410375695)) ;
#92488=CARTESIAN_POINT('Ctrl Pts',(-18.739350149088,15.4748445908299,122.409198110722)) ;
#92489=CARTESIAN_POINT('Ctrl Pts',(-18.9227807417284,15.4848050345447,122.308206356016)) ;
#92490=CARTESIAN_POINT('Ctrl Pts',(-19.1226076666943,15.4948418673629,122.24045140119)) ;
#92491=CARTESIAN_POINT('Ctrl Pts',(-19.3278520306524,15.5047206641097,122.208586054028)) ;
#92492=CARTESIAN_POINT('Ctrl Pts',(-19.5392660626703,15.5147799802381,122.212851541918)) ;
#92493=CARTESIAN_POINT('Ctrl Pts',(-19.742865967899,15.5246504269913,122.252995247253)) ;
#92494=CARTESIAN_POINT('Ctrl Pts',(-19.9389930492034,15.5346430652493,122.328273329601)) ;
#92495=CARTESIAN_POINT('Ctrl Pts',(-20.1195385360491,15.5446750807973,122.437273842859)) ;
#92496=CARTESIAN_POINT('Ctrl Pts',(-20.2761009054303,15.5545409371038,122.573347746441)) ;
#92497=CARTESIAN_POINT('Ctrl Pts',(-20.4093380126393,15.564610226573,122.737816255523)) ;
#92498=CARTESIAN_POINT('Ctrl Pts',(-20.5097308345635,15.5744537841243,122.918789549077)) ;
#92499=CARTESIAN_POINT('Ctrl Pts',(-20.5787544431515,15.5844339109121,123.116917366312)) ;
#92500=CARTESIAN_POINT('Ctrl Pts',(-20.6120581084781,15.594452459512,123.324883592933)) ;
#92501=CARTESIAN_POINT('Ctrl Pts',(-20.6092324216664,15.6043357600352,123.532667468491)) ;
#92502=CARTESIAN_POINT('Ctrl Pts',(-20.5695642818333,15.6144040470834,123.74054907884)) ;
#92503=CARTESIAN_POINT('Ctrl Pts',(-20.4963848100476,15.624234170102,123.933856050978)) ;
#92504=CARTESIAN_POINT('Ctrl Pts',(-20.3884819764366,15.6343007540273,124.115873435557)) ;
#92505=CARTESIAN_POINT('Ctrl Pts',(-20.2528965593543,15.6441908670418,124.273541533496)) ;
#92506=CARTESIAN_POINT('Ctrl Pts',(-20.0906428612495,15.6541835558044,124.406954200408)) ;
#92507=CARTESIAN_POINT('Ctrl Pts',(-19.9081751825224,15.6641444441602,124.509724862271)) ;
#92508=CARTESIAN_POINT('Ctrl Pts',(-19.7116275705627,15.6740623890402,124.579282836513)) ;
#92509=CARTESIAN_POINT('Ctrl Pts',(-19.5041324121698,15.6840701421364,124.61421493708)) ;
#92510=CARTESIAN_POINT('Ctrl Pts',(-19.2932685807458,15.6941012360955,124.612157280621)) ;
#92511=CARTESIAN_POINT('Ctrl Pts',(-19.0896398763648,15.7039492041234,124.574676428328)) ;
#92512=CARTESIAN_POINT('Ctrl Pts',(-18.8913605611505,15.7140111602493,124.501020788793)) ;
#92513=CARTESIAN_POINT('Ctrl Pts',(-18.7119475879741,15.7239083718504,124.395627509335)) ;
#92514=CARTESIAN_POINT('Ctrl Pts',(-18.5525797792541,15.7338395385151,124.260752918388)) ;
#92515=CARTESIAN_POINT('Ctrl Pts',(-18.4177343552575,15.7438817227192,124.098313868556)) ;
#92516=CARTESIAN_POINT('Ctrl Pts',(-18.3146251620328,15.7537683909724,123.917832449407)) ;
#92517=CARTESIAN_POINT('Ctrl Pts',(-18.243339460562,15.7637615029506,123.720221201578)) ;
#92518=CARTESIAN_POINT('Ctrl Pts',(-18.2076942595841,15.7737071805665,123.514192378456)) ;
#92519=CARTESIAN_POINT('Ctrl Pts',(-18.2079375211867,15.7836544835514,123.305059117356)) ;
#92520=CARTESIAN_POINT('Ctrl Pts',(-18.2450857165185,15.7937022072982,123.097121744275)) ;
#92521=CARTESIAN_POINT('Ctrl Pts',(-18.3161807824206,15.8035505810607,122.902670809947)) ;
#92522=CARTESIAN_POINT('Ctrl Pts',(-18.4205216430959,15.8135095535064,122.721154082513)) ;
#92523=CARTESIAN_POINT('Ctrl Pts',(-18.5561610131422,15.8235484153876,122.559473819216)) ;
#92524=CARTESIAN_POINT('Ctrl Pts',(-18.7150408738432,15.8334270195594,122.425695002758)) ;
#92525=CARTESIAN_POINT('Ctrl Pts',(-18.8977929149903,15.8434785607627,122.319658597131)) ;
#92526=CARTESIAN_POINT('Ctrl Pts',(-19.0931359801776,15.853373958743,122.248009867756)) ;
#92527=CARTESIAN_POINT('Ctrl Pts',(-19.3010940919877,15.8634251912883,122.210689226876)) ;
#92528=CARTESIAN_POINT('Ctrl Pts',(-19.5089537259741,15.8733113819126,122.210030665111)) ;
#92529=CARTESIAN_POINT('Ctrl Pts',(-19.7159988935587,15.8833039212284,122.245467028621)) ;
#92530=CARTESIAN_POINT('Ctrl Pts',(-19.9128808209097,15.8932523671231,122.316077247556)) ;
#92531=CARTESIAN_POINT('Ctrl Pts',(-20.0944193281804,15.903189169655,122.419404585991)) ;
#92532=CARTESIAN_POINT('Ctrl Pts',(-20.2562110175083,15.9131721771063,122.553127824227)) ;
#92533=CARTESIAN_POINT('Ctrl Pts',(-20.3928269463298,15.9232160185211,122.714098594079)) ;
#92534=CARTESIAN_POINT('Ctrl Pts',(-20.497578377328,15.933044217145,122.892232453388)) ;
#92535=CARTESIAN_POINT('Ctrl Pts',(-20.5717018245707,15.9431208105873,123.090636598625)) ;
#92536=CARTESIAN_POINT('Ctrl Pts',(-20.60951097072,15.9529728099288,123.29432257899)) ;
#92537=CARTESIAN_POINT('Ctrl Pts',(-20.6115947155634,15.9630463967527,123.506054649006)) ;
#92538=CARTESIAN_POINT('Ctrl Pts',(-20.5776393618552,15.9728866218502,123.710139972596)) ;
#92539=CARTESIAN_POINT('Ctrl Pts',(-20.5085933061261,15.9828523258788,123.907927922325)) ;
#92540=CARTESIAN_POINT('Ctrl Pts',(-20.4053465886935,15.9928789591854,124.091716966723)) ;
#92541=CARTESIAN_POINT('Ctrl Pts',(-20.2733736049024,16.0027932548972,124.253036026863)) ;
#92542=CARTESIAN_POINT('Ctrl Pts',(-20.1144504097341,16.0127815435897,124.390304177468)) ;
#92543=CARTESIAN_POINT('Ctrl Pts',(-19.9330154783584,16.022820276748,124.498096907349)) ;
#92544=CARTESIAN_POINT('Ctrl Pts',(-19.7395811261346,16.0326636085756,124.57162559323)) ;
#92545=CARTESIAN_POINT('Ctrl Pts',(-19.5326001890915,16.0426913344552,124.61165647205)) ;
#92546=CARTESIAN_POINT('Ctrl Pts',(-19.3217012772387,16.0527236708437,124.614568734802)) ;
#92547=CARTESIAN_POINT('Ctrl Pts',(-19.1176631555562,16.0625531711444,124.58191586368)) ;
#92548=CARTESIAN_POINT('Ctrl Pts',(-18.918992265536,16.0725426750611,124.513822087023)) ;
#92549=CARTESIAN_POINT('Ctrl Pts',(-18.7344293125495,16.0825865155735,124.411248264033)) ;
#92550=CARTESIAN_POINT('Ctrl Pts',(-18.5738358453558,16.0924082213416,124.281460878498)) ;
#92551=CARTESIAN_POINT('Ctrl Pts',(-18.4348819010564,16.102443268474,124.122718726248)) ;
#92552=CARTESIAN_POINT('Ctrl Pts',(-18.3262087689728,16.1124679459109,123.942139001591)) ;
#92553=CARTESIAN_POINT('Ctrl Pts',(-18.2514329563652,16.1223207607653,123.748970519295)) ;
#92554=CARTESIAN_POINT('Ctrl Pts',(-18.2104254293155,16.1323084703729,123.543056586751)) ;
#92555=CARTESIAN_POINT('Ctrl Pts',(-18.2058105598047,16.1422384803669,123.334340214107)) ;
#92556=CARTESIAN_POINT('Ctrl Pts',(-18.2373758696945,16.1522282355861,123.126705726276)) ;
#92557=CARTESIAN_POINT('Ctrl Pts',(-18.305019353964,16.162254844269,122.927059279513)) ;
#92558=CARTESIAN_POINT('Ctrl Pts',(-18.4046805537866,16.1721387842908,122.744731978536)) ;
#92559=CARTESIAN_POINT('Ctrl Pts',(-18.5354936500919,16.1821280118293,122.580436411234)) ;
#92560=CARTESIAN_POINT('Ctrl Pts',(-18.6939750793531,16.192170882353,122.440936931886)) ;
#92561=CARTESIAN_POINT('Ctrl Pts',(-18.8703193497203,16.2020032691084,122.33309622009)) ;
#92562=CARTESIAN_POINT('Ctrl Pts',(-19.0656339202826,16.21199656228,122.255709959275)) ;
#92563=CARTESIAN_POINT('Ctrl Pts',(-19.2723178754718,16.2220285679285,122.213677943216)) ;
#92564=CARTESIAN_POINT('Ctrl Pts',(-19.4796281174885,16.2318938238974,122.208007210553)) ;
#92565=CARTESIAN_POINT('Ctrl Pts',(-19.6868865960668,16.2418557038049,122.23813162295)) ;
#92566=CARTESIAN_POINT('Ctrl Pts',(-19.8870996977889,16.2518906371668,122.304588583264)) ;
#92567=CARTESIAN_POINT('Ctrl Pts',(-20.0701600670117,16.2617755955461,122.403012887225)) ;
#92568=CARTESIAN_POINT('Ctrl Pts',(-20.236252850506,16.2718412224688,122.534076878473)) ;
#92569=CARTESIAN_POINT('Ctrl Pts',(-20.3740988627179,16.2816803281331,122.688345897485)) ;
#92570=CARTESIAN_POINT('Ctrl Pts',(-20.4857489174629,16.2917431431385,122.868002488116)) ;
#92571=CARTESIAN_POINT('Ctrl Pts',(-20.5630460710818,16.3016393491872,123.061183039418)) ;
#92572=CARTESIAN_POINT('Ctrl Pts',(-20.6063783438916,16.3115801722124,123.265604158338)) ;
#92573=CARTESIAN_POINT('Ctrl Pts',(-20.6136572717799,16.3215847551911,123.475829776473)) ;
#92574=CARTESIAN_POINT('Ctrl Pts',(-20.5840255669465,16.3316056496358,123.684401378321)) ;
#92575=CARTESIAN_POINT('Ctrl Pts',(-20.5197138580458,16.3414975702252,123.882172231323)) ;
#92576=CARTESIAN_POINT('Ctrl Pts',(-20.4213081312752,16.3514910025706,124.067785910372)) ;
#92577=CARTESIAN_POINT('Ctrl Pts',(-20.2927295521724,16.3614366074705,124.232664564836)) ;
#92578=CARTESIAN_POINT('Ctrl Pts',(-20.1377257011545,16.371383880952,124.373060345475)) ;
#92579=CARTESIAN_POINT('Ctrl Pts',(-19.9587972936868,16.3814317954284,124.485325647766)) ;
#92580=CARTESIAN_POINT('Ctrl Pts',(-19.7670525971543,16.3912794357757,124.563399294681)) ;
#92581=CARTESIAN_POINT('Ctrl Pts',(-19.5624702538789,16.4012411511523,124.608137599496)) ;
#92582=CARTESIAN_POINT('Ctrl Pts',(-19.3517882231378,16.4112697747251,124.616465588715)) ;
#92583=CARTESIAN_POINT('Ctrl Pts',(-19.1453379508177,16.4211801367915,124.588489760527)) ;
#92584=CARTESIAN_POINT('Ctrl Pts',(-18.9462094865371,16.4311148304439,124.525456505747)) ;
#92585=CARTESIAN_POINT('Ctrl Pts',(-18.759167106785,16.4411566735718,124.427586025699)) ;
#92586=CARTESIAN_POINT('Ctrl Pts',(-18.5944416876923,16.4510411791422,124.300871709702)) ;
#92587=CARTESIAN_POINT('Ctrl Pts',(-18.4524057546357,16.4610432829274,124.145859449179)) ;
#92588=CARTESIAN_POINT('Ctrl Pts',(-18.3402079875807,16.4709616343424,123.970062250184)) ;
#92589=CARTESIAN_POINT('Ctrl Pts',(-18.259272916945,16.4810092903633,123.774984953265)) ;
#92590=CARTESIAN_POINT('Ctrl Pts',(-18.214000026434,16.4908804833915,123.572415370534)) ;
#92591=CARTESIAN_POINT('Ctrl Pts',(-18.2043727827825,16.500946196535,123.361070103728)) ;
#92592=CARTESIAN_POINT('Ctrl Pts',(-18.2307852503669,16.5107986571077,123.155574634655)) ;
#92593=CARTESIAN_POINT('Ctrl Pts',(-18.3149326179074,16.5242271198303,122.886171955467)) ;
#92594=CARTESIAN_POINT('Ctrl Pts',(-18.4633058127872,16.5373080673473,122.650748595137)) ;
#92595=CARTESIAN_POINT('Ctrl Pts',(-18.6709271702637,16.5507825655819,122.45819153009)) ;
#92596=CARTESIAN_POINT('Ctrl Pts',(-18.844772245183,16.5606146691914,122.346294242523)) ;
#92597=CARTESIAN_POINT('Ctrl Pts',(-19.0376048516113,16.570580572318,122.264442649281)) ;
#92598=CARTESIAN_POINT('Ctrl Pts',(-19.2431084492467,16.5806079816283,122.217330837706)) ;
#92599=CARTESIAN_POINT('Ctrl Pts',(-19.4511660916749,16.5905190129948,122.206685716486)) ;
#92600=CARTESIAN_POINT('Ctrl Pts',(-19.7276789075163,16.6037633206159,122.240089314737)) ;
#92601=CARTESIAN_POINT('Ctrl Pts',(-20.0569137775014,16.620463803287,122.372795345681)) ;
#92602=CARTESIAN_POINT('Ctrl Pts',(-20.3183354751437,16.6369706324428,122.607173302249)) ;
#92603=CARTESIAN_POINT('Ctrl Pts',(-20.4717078563946,16.6502812606804,122.841129281592)) ;
#92604=CARTESIAN_POINT('Ctrl Pts',(-20.5546945603432,16.6602738242205,123.034165773958)) ;
#92605=CARTESIAN_POINT('Ctrl Pts',(-20.6028174061506,16.6703039072221,123.239432220823)) ;
#92606=CARTESIAN_POINT('Ctrl Pts',(-20.6188287734652,16.6834775112198,123.515992234632)) ;
#92607=CARTESIAN_POINT('Ctrl Pts',(-20.5476980246839,16.7001152164512,123.862375258934)) ;
#92608=CARTESIAN_POINT('Ctrl Pts',(-20.3266353919911,16.7199969790187,124.222885277575)) ;
#92609=CARTESIAN_POINT('Ctrl Pts',(-20.0488095001874,16.7366933312352,124.443797374202)) ;
#92610=CARTESIAN_POINT('Ctrl Pts',(-19.7952425804301,16.7498503590243,124.554332607942)) ;
#92611=CARTESIAN_POINT('Ctrl Pts',(-19.5219786846243,16.7632277136678,124.620786198231)) ;
#92612=CARTESIAN_POINT('Ctrl Pts',(-19.1705567065255,16.7797585479266,124.612580136977)) ;
#92613=CARTESIAN_POINT('Ctrl Pts',(-18.7748001955681,16.7997232376697,124.459120947067)) ;
#92614=CARTESIAN_POINT('Ctrl Pts',(-18.456169900626,16.8196397310933,124.180166285516)) ;
#92615=CARTESIAN_POINT('Ctrl Pts',(-18.2513765417998,16.8395294504429,123.810101465255)) ;
#92616=CARTESIAN_POINT('Ctrl Pts',(-18.1851276829267,16.8595361800907,123.389957374541)) ;
#92617=CARTESIAN_POINT('Ctrl Pts',(-18.2652600268736,16.8793742337376,122.975738508735)) ;
#92618=CARTESIAN_POINT('Ctrl Pts',(-18.4831734060332,16.8993675719512,122.610816739563)) ;
#92619=CARTESIAN_POINT('Ctrl Pts',(-18.811001815802,16.9192503713578,122.343752254667)) ;
#92620=CARTESIAN_POINT('Ctrl Pts',(-19.2100490940889,16.9391425522766,122.203910312485)) ;
#92621=CARTESIAN_POINT('Ctrl Pts',(-19.6333307049043,16.9590447307716,122.207929486996)) ;
#92622=CARTESIAN_POINT('Ctrl Pts',(-20.0320401542686,16.9790820419754,122.357765050694)) ;
#92623=CARTESIAN_POINT('Ctrl Pts',(-20.3526643510395,16.9988944835162,122.631302217642)) ;
#92624=CARTESIAN_POINT('Ctrl Pts',(-20.5630417913117,17.0189597242511,123.002232943253)) ;
#92625=CARTESIAN_POINT('Ctrl Pts',(-20.6335141763589,17.038716929107,123.41657830206)) ;
#92626=CARTESIAN_POINT('Ctrl Pts',(-20.558006365627,17.0587502017527,123.83557544901)) ;
#92627=CARTESIAN_POINT('Ctrl Pts',(-20.3461518752294,17.0785631102065,124.199927876101)) ;
#92628=CARTESIAN_POINT('Ctrl Pts',(-20.0203444599083,17.0985592563339,124.472800792273)) ;
#92629=CARTESIAN_POINT('Ctrl Pts',(-19.6233799466001,17.1184210095564,124.617465604791)) ;
#92630=CARTESIAN_POINT('Ctrl Pts',(-19.1967646146023,17.1384895266845,124.617721479536)) ;
#92631=CARTESIAN_POINT('Ctrl Pts',(-18.8003376032294,17.1583203996814,124.473776890643)) ;
#92632=CARTESIAN_POINT('Ctrl Pts',(-18.474755985943,17.178242310498,124.202953838831)) ;
#92633=CARTESIAN_POINT('Ctrl Pts',(-18.2610777094718,17.1981717539333,123.836937803985)) ;
#92634=CARTESIAN_POINT('Ctrl Pts',(-18.1850738363319,17.2180814240497,123.420547760837)) ;
#92635=CARTESIAN_POINT('Ctrl Pts',(-18.2548695109545,17.2379547813126,123.003739169527)) ;
#92636=CARTESIAN_POINT('Ctrl Pts',(-18.4639625203726,17.2579463159305,122.633712831633)) ;
#92637=CARTESIAN_POINT('Ctrl Pts',(-18.7847202958821,17.2778119333413,122.358779484358)) ;
#92638=CARTESIAN_POINT('Ctrl Pts',(-19.1821149054444,17.2977928631695,122.208575251661)) ;
#92639=CARTESIAN_POINT('Ctrl Pts',(-19.6060391887632,17.3177313252526,122.203480342946)) ;
#92640=CARTESIAN_POINT('Ctrl Pts',(-20.0055818061372,17.3376235184743,122.342419897881)) ;
#92641=CARTESIAN_POINT('Ctrl Pts',(-20.334784776262,17.3575942335097,122.610483376116)) ;
#92642=CARTESIAN_POINT('Ctrl Pts',(-20.5517123729197,17.3774039051758,122.971652127387)) ;
#92643=CARTESIAN_POINT('Ctrl Pts',(-20.6333779841196,17.397397121867,123.38868425828)) ;
#92644=CARTESIAN_POINT('Ctrl Pts',(-20.5685930892492,17.4172480340634,123.805942383604)) ;
#92645=CARTESIAN_POINT('Ctrl Pts',(-20.362939525817,17.4373226403824,124.179848021517)) ;
#92646=CARTESIAN_POINT('Ctrl Pts',(-20.0986114574795,17.4538392722657,124.411232690189)) ;
#92647=CARTESIAN_POINT('Ctrl Pts',(-19.8472361244034,17.4671779799598,124.535422018461)) ;
#92648=CARTESIAN_POINT('Ctrl Pts',(-19.648695502256,17.4770203542681,124.59379753623)) ;
#92649=CARTESIAN_POINT('Ctrl Pts',(-19.4386608921935,17.4870753742509,124.617501313402)) ;
#92650=CARTESIAN_POINT('Ctrl Pts',(-19.1610336465222,17.5003075309084,124.600234914191)) ;
#92651=CARTESIAN_POINT('Ctrl Pts',(-18.8258946716868,17.5169224982536,124.488350036976)) ;
#92652=CARTESIAN_POINT('Ctrl Pts',(-18.5495768861815,17.5335170852648,124.269022343617)) ;
#92653=CARTESIAN_POINT('Ctrl Pts',(-18.3833597626593,17.5467506536201,124.045859160823)) ;
#92654=CARTESIAN_POINT('Ctrl Pts',(-18.2885301460445,17.5567942714288,123.857229876977)) ;
#92655=CARTESIAN_POINT('Ctrl Pts',(-18.2287562532625,17.5666811956636,123.658135390516)) ;
#92656=CARTESIAN_POINT('Ctrl Pts',(-18.2038373026383,17.5766718501104,123.449600371017)) ;
#92657=CARTESIAN_POINT('Ctrl Pts',(-18.2155183685981,17.5866336085644,123.240489044656)) ;
#92658=CARTESIAN_POINT('Ctrl Pts',(-18.279242571354,17.5999734736316,122.967369587735)) ;
#92659=CARTESIAN_POINT('Ctrl Pts',(-18.4130348186502,17.6132822565449,122.718034113314)) ;
#92660=CARTESIAN_POINT('Ctrl Pts',(-18.6026066359748,17.626478013989,122.515468739054)) ;
#92661=CARTESIAN_POINT('Ctrl Pts',(-18.7697373043821,17.6364398976655,122.389261069262)) ;
#92662=CARTESIAN_POINT('Ctrl Pts',(-18.9579188750606,17.6464830071801,122.293522035345)) ;
#92663=CARTESIAN_POINT('Ctrl Pts',(-19.1559640195152,17.6563352571794,122.232844539116)) ;
#92664=CARTESIAN_POINT('Ctrl Pts',(-19.3639322621533,17.6663067941298,122.2066607369)) ;
#92665=CARTESIAN_POINT('Ctrl Pts',(-19.5738409368387,17.6763020596074,122.217029727047)) ;
#92666=CARTESIAN_POINT('Ctrl Pts',(-19.779447249497,17.686336032481,122.26411039526)) ;
#92667=CARTESIAN_POINT('Ctrl Pts',(-19.9704605312748,17.6961914472433,122.344426643971)) ;
#92668=CARTESIAN_POINT('Ctrl Pts',(-20.1472770617746,17.7061907247522,122.458056115993)) ;
#92669=CARTESIAN_POINT('Ctrl Pts',(-20.3002748821021,17.7160859089151,122.599059950491)) ;
#92670=CARTESIAN_POINT('Ctrl Pts',(-20.4285143353315,17.7261462885559,122.767212180967)) ;
#92671=CARTESIAN_POINT('Ctrl Pts',(-20.5237126912126,17.735996157564,122.951130309144)) ;
#92672=CARTESIAN_POINT('Ctrl Pts',(-20.5871207120821,17.7460277187719,123.152253498345)) ;
#92673=CARTESIAN_POINT('Ctrl Pts',(-20.614169464625,17.7560381676542,123.360978680568)) ;
#92674=CARTESIAN_POINT('Ctrl Pts',(-20.6048963808325,17.7659449070712,123.569036052388)) ;
#92675=CARTESIAN_POINT('Ctrl Pts',(-20.5598938017532,17.7758829231397,123.773047845721)) ;
#92676=CARTESIAN_POINT('Ctrl Pts',(-20.4797271625852,17.7858881695908,123.96753801668)) ;
#92677=CARTESIAN_POINT('Ctrl Pts',(-20.3663978026102,17.7959222306471,124.14544500573)) ;
#92678=CARTESIAN_POINT('Ctrl Pts',(-20.2268317347825,17.8057673117052,124.298300993795)) ;
#92679=CARTESIAN_POINT('Ctrl Pts',(-20.0607767182021,17.8157531176587,124.42668993648)) ;
#92680=CARTESIAN_POINT('Ctrl Pts',(-19.8759066227852,17.8256879382129,124.523963674661)) ;
#92681=CARTESIAN_POINT('Ctrl Pts',(-19.6745057962594,17.8357454633451,124.588245908723)) ;
#92682=CARTESIAN_POINT('Ctrl Pts',(-19.4699075152098,17.8455671139965,124.616238143836)) ;
#92683=CARTESIAN_POINT('Ctrl Pts',(-19.2586565360455,17.8556231775012,124.608486329999)) ;
#92684=CARTESIAN_POINT('Ctrl Pts',(-19.0543868810221,17.8655638445652,124.564306967429)) ;
#92685=CARTESIAN_POINT('Ctrl Pts',(-18.8613551760711,17.8754682382312,124.486226474479)) ;
#92686=CARTESIAN_POINT('Ctrl Pts',(-18.6823712514696,17.8855147619942,124.374127325253)) ;
#92687=CARTESIAN_POINT('Ctrl Pts',(-18.5277423281328,17.8954108450105,124.234883371212)) ;
#92688=CARTESIAN_POINT('Ctrl Pts',(-18.3975181430784,17.9054775442406,124.068106619042)) ;
#92689=CARTESIAN_POINT('Ctrl Pts',(-18.3003841394302,17.9153011546416,123.885816198438)) ;
#92690=CARTESIAN_POINT('Ctrl Pts',(-18.2345288001946,17.9253570148191,123.684957633441)) ;
#92691=CARTESIAN_POINT('Ctrl Pts',(-18.2051746045371,17.9352901611241,123.478179415023)) ;
#92692=CARTESIAN_POINT('Ctrl Pts',(-18.2117492800176,17.9452354168947,123.269226637619)) ;
#92693=CARTESIAN_POINT('Ctrl Pts',(-18.2545138749042,17.9552187153331,123.063722393022)) ;
#92694=CARTESIAN_POINT('Ctrl Pts',(-18.332982546595,17.9652558954798,122.867858865701)) ;
#92695=CARTESIAN_POINT('Ctrl Pts',(-18.4419876923002,17.9751104481892,122.691657865086)) ;
#92696=CARTESIAN_POINT('Ctrl Pts',(-18.5817046930857,17.9851099666366,122.534632669291)) ;
#92697=CARTESIAN_POINT('Ctrl Pts',(-18.7447605573555,17.9950050490986,122.405396565275)) ;
#92698=CARTESIAN_POINT('Ctrl Pts',(-18.9307947177022,18.0050655946047,122.304828643302)) ;
#92699=CARTESIAN_POINT('Ctrl Pts',(-19.1272549252657,18.0149149018527,122.239367986776)) ;
#92700=CARTESIAN_POINT('Ctrl Pts',(-19.3356951723123,18.0249419919401,122.207938380922)) ;
#92701=CARTESIAN_POINT('Ctrl Pts',(-19.5464637005293,18.034970896077,122.213739547083)) ;
#92702=CARTESIAN_POINT('Ctrl Pts',(-19.7492771163832,18.0448147611763,122.254862768678)) ;
#92703=CARTESIAN_POINT('Ctrl Pts',(-19.9450396627883,18.0548105878847,122.331265516331)) ;
#92704=CARTESIAN_POINT('Ctrl Pts',(-20.1248922039138,18.0648358045337,122.441153300508)) ;
#92705=CARTESIAN_POINT('Ctrl Pts',(-20.2809828150676,18.0747256366913,122.578506474062)) ;
#92706=CARTESIAN_POINT('Ctrl Pts',(-20.41239798799,18.0847164927761,122.742346642746)) ;
#92707=CARTESIAN_POINT('Ctrl Pts',(-20.5128750333095,18.0946615873689,122.925697207635)) ;
#92708=CARTESIAN_POINT('Ctrl Pts',(-20.5804101806714,18.104613491137,123.123726265295)) ;
#92709=CARTESIAN_POINT('Ctrl Pts',(-20.6126233193585,18.1146498906065,123.332244159599)) ;
#92710=CARTESIAN_POINT('Ctrl Pts',(-20.6083596579032,18.1245389606951,123.540106535664)) ;
#92711=CARTESIAN_POINT('Ctrl Pts',(-20.5680335657877,18.134528250066,123.746199619181)) ;
#92712=CARTESIAN_POINT('Ctrl Pts',(-20.4926226175527,18.1444868162757,123.941500160299)) ;
#92713=CARTESIAN_POINT('Ctrl Pts',(-20.3855172756073,18.1543863874925,124.119959362233)) ;
#92714=CARTESIAN_POINT('Ctrl Pts',(-20.2469737795764,18.1644343019068,124.279390768898)) ;
#92715=CARTESIAN_POINT('Ctrl Pts',(-20.0854054780524,18.1743296447674,124.410486987501)) ;
#92716=CARTESIAN_POINT('Ctrl Pts',(-19.9005352677414,18.1843913387148,124.513234865981)) ;
#92717=CARTESIAN_POINT('Ctrl Pts',(-19.7049301084551,18.194235791799,124.580875659365)) ;
#92718=CARTESIAN_POINT('Ctrl Pts',(-19.4982739713939,18.2041964767574,124.614633529283)) ;
#92719=CARTESIAN_POINT('Ctrl Pts',(-19.2873016161751,18.2142324092659,124.611621181168)) ;
#92720=CARTESIAN_POINT('Ctrl Pts',(-19.0830713036951,18.224121024954,124.572810361902)) ;
#92721=CARTESIAN_POINT('Ctrl Pts',(-18.8860432075107,18.2341354340964,124.498576095596)) ;
#92722=CARTESIAN_POINT('Ctrl Pts',(-18.7048498609844,18.2441692430542,124.39059329917)) ;
#92723=CARTESIAN_POINT('Ctrl Pts',(-18.5479908132321,18.2539996973104,124.255995858726)) ;
#92724=CARTESIAN_POINT('Ctrl Pts',(-18.4135763511044,18.2640773648886,124.092282642532)) ;
#92725=CARTESIAN_POINT('Ctrl Pts',(-18.3118235018209,18.2739292330109,123.911832242753)) ;
#92726=CARTESIAN_POINT('Ctrl Pts',(-18.2412636867744,18.2840022705762,123.712204349942)) ;
#92727=CARTESIAN_POINT('Ctrl Pts',(-18.2072562031298,18.2938448239271,123.508079054221)) ;
#92728=CARTESIAN_POINT('Ctrl Pts',(-18.2085295943525,18.3038252194205,123.298272684557)) ;
#92729=CARTESIAN_POINT('Ctrl Pts',(-18.2467612388088,18.3138436973983,123.091156447569)) ;
#92730=CARTESIAN_POINT('Ctrl Pts',(-18.3189753705069,18.3237270117044,122.8963045179)) ;
#92731=CARTESIAN_POINT('Ctrl Pts',(-18.4259403030239,18.3337953142431,122.713693116947)) ;
#92732=CARTESIAN_POINT('Ctrl Pts',(-18.5596026738779,18.3436253615166,122.556032941135)) ;
#92733=CARTESIAN_POINT('Ctrl Pts',(-18.7222139779359,18.3536922329321,122.420633676743)) ;
#92734=CARTESIAN_POINT('Ctrl Pts',(-18.9027321027321,18.3635812717311,122.317447011611)) ;
#92735=CARTESIAN_POINT('Ctrl Pts',(-19.1003668831419,18.3735779698652,122.246036932868)) ;
#92736=CARTESIAN_POINT('Ctrl Pts',(-19.3065323749865,18.3835303955772,122.210267849344)) ;
#92737=CARTESIAN_POINT('Ctrl Pts',(-19.5155137773644,18.3934716978101,122.210548411513)) ;
#92738=CARTESIAN_POINT('Ctrl Pts',(-19.7222189729129,18.4034549368941,122.247050235139)) ;
#92739=CARTESIAN_POINT('Ctrl Pts',(-19.9203917704967,18.4134937384627,122.319582320814)) ;
#92740=CARTESIAN_POINT('Ctrl Pts',(-20.0997259303789,18.4233418445843,122.423079545611)) ;
#92741=CARTESIAN_POINT('Ctrl Pts',(-20.2618814150769,18.4334020401596,122.558833845978)) ;
#92742=CARTESIAN_POINT('Ctrl Pts',(-20.3956744568318,18.4432997234711,122.718208693815)) ;
#92743=CARTESIAN_POINT('Ctrl Pts',(-20.5006998407244,18.453230763845,122.898646677112)) ;
#92744=CARTESIAN_POINT('Ctrl Pts',(-20.5733935717876,18.4632729815016,123.096852667896)) ;
#92745=CARTESIAN_POINT('Ctrl Pts',(-20.6101416798205,18.4731596422356,123.301436558527)) ;
#92746=CARTESIAN_POINT('Ctrl Pts',(-20.6111685275753,18.4831527508381,123.511509867575)) ;
#92747=CARTESIAN_POINT('Ctrl Pts',(-20.5757926440106,18.4930984494763,123.717585350536)) ;
#92748=CARTESIAN_POINT('Ctrl Pts',(-20.5055613986537,18.5030456717474,123.914572326248)) ;
#92749=CARTESIAN_POINT('Ctrl Pts',(-20.4009471294435,18.5130936973275,124.098082350297)) ;
#92750=CARTESIAN_POINT('Ctrl Pts',(-20.2688858815582,18.5229409444704,124.257508846386)) ;
#92751=CARTESIAN_POINT('Ctrl Pts',(-20.1097243873236,18.5329041215612,124.39366353997)) ;
#92752=CARTESIAN_POINT('Ctrl Pts',(-19.9279709104709,18.5429338425946,124.500552449565)) ;
#92753=CARTESIAN_POINT('Ctrl Pts',(-19.7329558518841,18.5528383101275,124.573584975196)) ;
#92754=CARTESIAN_POINT('Ctrl Pts',(-19.5257968398549,18.5628627959572,124.612170958543)) ;
#92755=CARTESIAN_POINT('Ctrl Pts',(-19.3175695775789,18.5727666310811,124.614349950138)) ;
#92756=CARTESIAN_POINT('Ctrl Pts',(-19.1091146716,18.5828178217911,124.579889396335)) ;
#92757=CARTESIAN_POINT('Ctrl Pts',(-18.9130619976657,18.5927022644494,124.510943603526)) ;
#92758=CARTESIAN_POINT('Ctrl Pts',(-18.7298124080229,18.6026952723013,124.408243913293)) ;
#92759=CARTESIAN_POINT('Ctrl Pts',(-18.5679260386757,18.6126435920176,124.275805094592)) ;
#92760=CARTESIAN_POINT('Ctrl Pts',(-18.4314461503668,18.622580430727,124.117671389572)) ;
#92761=CARTESIAN_POINT('Ctrl Pts',(-18.3237491434459,18.6325634196466,123.937505549307)) ;
#92762=CARTESIAN_POINT('Ctrl Pts',(-18.2488966463023,18.6426072990107,123.740090399413)) ;
#92763=CARTESIAN_POINT('Ctrl Pts',(-18.209813068051,18.6524353643691,123.537170757403)) ;
#92764=CARTESIAN_POINT('Ctrl Pts',(-18.206385155789,18.6625124529241,123.325393218201)) ;
#92765=CARTESIAN_POINT('Ctrl Pts',(-18.238909571519,18.6723626050803,123.120828018811)) ;
#92766=CARTESIAN_POINT('Ctrl Pts',(-18.3079228948117,18.6824430855327,122.920512684699)) ;
#92767=CARTESIAN_POINT('Ctrl Pts',(-18.4078474591112,18.6922575833015,122.739938990814)) ;
#92768=CARTESIAN_POINT('Ctrl Pts',(-18.540643272446,18.7023258793217,122.575174082538)) ;
#92769=CARTESIAN_POINT('Ctrl Pts',(-18.6974620081295,18.7122247118044,122.438290139689)) ;
#92770=CARTESIAN_POINT('Ctrl Pts',(-18.8783200201035,18.722277591819,122.329027980495)) ;
#92771=CARTESIAN_POINT('Ctrl Pts',(-19.071821712519,18.7321474073151,122.254003571519)) ;
#92772=CARTESIAN_POINT('Ctrl Pts',(-19.2795064905227,18.7422200883979,122.212846727025)) ;
#92773=CARTESIAN_POINT('Ctrl Pts',(-19.4861884068662,18.7520525669689,122.208399678899)) ;
#92774=CARTESIAN_POINT('Ctrl Pts',(-19.6946842005538,18.762083200955,122.239936671409)) ;
#92775=CARTESIAN_POINT('Ctrl Pts',(-19.8943770937063,18.7721147581741,122.307793552659)) ;
#92776=CARTESIAN_POINT('Ctrl Pts',(-20.0757189680045,18.7819444670458,122.406859087493)) ;
#92777=CARTESIAN_POINT('Ctrl Pts',(-20.240134989661,18.7919339158479,122.537526730082)) ;
#92778=CARTESIAN_POINT('Ctrl Pts',(-20.3797167170314,18.801977768248,122.695962331067)) ;
#92779=CARTESIAN_POINT('Ctrl Pts',(-20.4876019724467,18.81179948158,122.872018741494)) ;
#92780=CARTESIAN_POINT('Ctrl Pts',(-20.5654043884981,18.8218344865687,123.068115037575)) ;
#92781=CARTESIAN_POINT('Ctrl Pts',(-20.6073616902904,18.8318593250163,123.274657332635)) ;
#92782=CARTESIAN_POINT('Ctrl Pts',(-20.6131682480769,18.8417115379715,123.481700357491)) ;
#92783=CARTESIAN_POINT('Ctrl Pts',(-20.5828695031209,18.8517014941653,123.689507408445)) ;
#92784=CARTESIAN_POINT('Ctrl Pts',(-20.5173663478567,18.8616296044486,123.887689661944)) ;
#92785=CARTESIAN_POINT('Ctrl Pts',(-20.4181397973166,18.8716182045281,124.072765157157)) ;
#92786=CARTESIAN_POINT('Ctrl Pts',(-20.287563655019,18.8816447964556,124.238246495347)) ;
#92787=CARTESIAN_POINT('Ctrl Pts',(-20.1326099286412,18.8915299245198,124.376719376746)) ;
#92788=CARTESIAN_POINT('Ctrl Pts',(-19.9543134225387,18.9015210419933,124.487770822266)) ;
#92789=CARTESIAN_POINT('Ctrl Pts',(-19.7583197977327,18.9115616578451,124.566149255982)) ;
#92790=CARTESIAN_POINT('Ctrl Pts',(-19.5560396588162,18.9213946486988,124.608747665617)) ;
#92791=CARTESIAN_POINT('Ctrl Pts',(-19.3460913770336,18.9313877801491,124.616289970544)) ;
#92792=CARTESIAN_POINT('Ctrl Pts',(-19.1372600770967,18.9414198285845,124.586714093607)) ;
#92793=CARTESIAN_POINT('Ctrl Pts',(-18.9400108926563,18.9512850751269,124.522664185328)) ;
#92794=CARTESIAN_POINT('Ctrl Pts',(-18.7547919702159,18.9612469499537,124.424901736679)) ;
#92795=CARTESIAN_POINT('Ctrl Pts',(-18.5883738302612,18.971281913065,124.2952601066)) ;
#92796=CARTESIAN_POINT('Ctrl Pts',(-18.448819046263,18.9811667575274,124.141239790597)) ;
#92797=CARTESIAN_POINT('Ctrl Pts',(-18.3361799499564,18.9912328103682,123.962131075838)) ;
#92798=CARTESIAN_POINT('Ctrl Pts',(-18.257920565973,19.0010703262771,123.770652739752)) ;
#92799=CARTESIAN_POINT('Ctrl Pts',(-18.2128628976887,19.011139074386,123.563864375363)) ;
#92800=CARTESIAN_POINT('Ctrl Pts',(-18.2046274740072,19.021019591417,123.35627632858)) ;
#92801=CARTESIAN_POINT('Ctrl Pts',(-18.2324438398586,19.0310107783515,123.14811114272)) ;
#92802=CARTESIAN_POINT('Ctrl Pts',(-18.2957268717079,19.0409638446264,122.948631979712)) ;
#92803=CARTESIAN_POINT('Ctrl Pts',(-18.3935294235557,19.050999682159,122.761704016059)) ;
#92804=CARTESIAN_POINT('Ctrl Pts',(-18.5203397037647,19.0608898083705,122.596912724645)) ;
#92805=CARTESIAN_POINT('Ctrl Pts',(-18.6751751381442,19.0708819902784,122.454963144696)) ;
#92806=CARTESIAN_POINT('Ctrl Pts',(-18.8515331380732,19.080827930217,122.342630525861)) ;
#92807=CARTESIAN_POINT('Ctrl Pts',(-19.0445885349267,19.0907751139811,122.262219655988)) ;
#92808=CARTESIAN_POINT('Ctrl Pts',(-19.2507744154612,19.1008230522886,122.2163232578)) ;
#92809=CARTESIAN_POINT('Ctrl Pts',(-19.4575916342668,19.1106706870288,122.206936574544)) ;
#92810=CARTESIAN_POINT('Ctrl Pts',(-19.6653476661059,19.1206324010027,122.233259211876)) ;
#92811=CARTESIAN_POINT('Ctrl Pts',(-19.8666639016408,19.1306610357935,122.29593385509)) ;
#92812=CARTESIAN_POINT('Ctrl Pts',(-20.051840008439,19.1405713543906,122.391400489081)) ;
#92813=CARTESIAN_POINT('Ctrl Pts',(-20.2183835287999,19.1505062107021,122.517455364573)) ;
#92814=CARTESIAN_POINT('Ctrl Pts',(-20.3618707267679,19.1605474466628,122.672277305996)) ;
#92815=CARTESIAN_POINT('Ctrl Pts',(-20.4746969685949,19.1704342182428,122.84686466971)) ;
#92816=CARTESIAN_POINT('Ctrl Pts',(-20.5566359490332,19.180434396949,123.040441287818)) ;
#92817=CARTESIAN_POINT('Ctrl Pts',(-20.6035192128641,19.1903516751586,123.243629824238)) ;
#92818=CARTESIAN_POINT('Ctrl Pts',(-20.6144848714803,19.2003989215723,123.45454051426)) ;
#92819=CARTESIAN_POINT('Ctrl Pts',(-20.5893212820512,19.2102728105536,123.66062268631)) ;
#92820=CARTESIAN_POINT('Ctrl Pts',(-20.5277315285585,19.2203348281341,123.862966148539)) ;
#92821=CARTESIAN_POINT('Ctrl Pts',(-20.4337173847183,19.2302058898684,124.047986049992)) ;
#92822=CARTESIAN_POINT('Ctrl Pts',(-20.3079299377085,19.2401999532287,124.216278219142)) ;
#92823=CARTESIAN_POINT('Ctrl Pts',(-20.1539324571469,19.2502321112621,124.360376363104)) ;
#92824=CARTESIAN_POINT('Ctrl Pts',(-19.9804428304959,19.2600959875023,124.474010306699)) ;
#92825=CARTESIAN_POINT('Ctrl Pts',(-19.785918102539,19.2701665021406,124.557511631259)) ;
#92826=CARTESIAN_POINT('Ctrl Pts',(-19.5845187324554,19.2800071390815,124.604891315488)) ;
#92827=CARTESIAN_POINT('Ctrl Pts',(-19.3753707846235,19.2899742679217,124.617420940457)) ;
#92828=CARTESIAN_POINT('Ctrl Pts',(-19.166242834232,19.2999882410463,124.593109638195)) ;
#92829=CARTESIAN_POINT('Ctrl Pts',(-18.8985887014101,19.3132729749095,124.51325325629)) ;
#92830=CARTESIAN_POINT('Ctrl Pts',(-18.6588871766436,19.3264982396243,124.366249593857)) ;
#92831=CARTESIAN_POINT('Ctrl Pts',(-18.4660700120822,19.3398087621792,124.163476304628)) ;
#92832=CARTESIAN_POINT('Ctrl Pts',(-18.3496595368789,19.3498374070813,123.987691601634)) ;
#92833=CARTESIAN_POINT('Ctrl Pts',(-18.2666103013183,19.3597184394352,123.797281986948)) ;
#92834=CARTESIAN_POINT('Ctrl Pts',(-18.2169671242081,19.3696994121153,123.59340792941)) ;
#92835=CARTESIAN_POINT('Ctrl Pts',(-18.2036560598774,19.3796805397013,123.384012285161)) ;
#92836=CARTESIAN_POINT('Ctrl Pts',(-18.2339327119865,19.3929237299627,123.107171028627)) ;
#92837=CARTESIAN_POINT('Ctrl Pts',(-18.3623905823458,19.4095917253235,122.776996485116)) ;
#92838=CARTESIAN_POINT('Ctrl Pts',(-18.5937075244846,19.4261122253356,122.512484155667)) ;
#92839=CARTESIAN_POINT('Ctrl Pts',(-18.8258991005238,19.4394252416516,122.356364000433)) ;
#92840=CARTESIAN_POINT('Ctrl Pts',(-19.0164084985625,19.4493417998846,122.271584814231)) ;
#92841=CARTESIAN_POINT('Ctrl Pts',(-19.220935191191,19.4593694681874,122.220706883488)) ;
#92842=CARTESIAN_POINT('Ctrl Pts',(-19.4974374171098,19.4725500579321,122.20084547395)) ;
#92843=CARTESIAN_POINT('Ctrl Pts',(-19.8469033690404,19.4892981970515,122.268339913805)) ;
#92844=CARTESIAN_POINT('Ctrl Pts',(-20.2084084568038,19.509092939562,122.484283598971)) ;
#92845=CARTESIAN_POINT('Ctrl Pts',(-20.4779908515016,19.5291373323708,122.814197913215)) ;
#92846=CARTESIAN_POINT('Ctrl Pts',(-20.6171058529899,19.5489765146695,123.21255429909)) ;
#92847=CARTESIAN_POINT('Ctrl Pts',(-20.612955760874,19.5689018383624,123.636097734435)) ;
#92848=CARTESIAN_POINT('Ctrl Pts',(-20.464422625464,19.5888254764139,124.032909263132)) ;
#92849=CARTESIAN_POINT('Ctrl Pts',(-20.1895544218666,19.6087503498795,124.355231271546)) ;
#92850=CARTESIAN_POINT('Ctrl Pts',(-19.8222577775006,19.6286289569584,124.564437287591)) ;
#92851=CARTESIAN_POINT('Ctrl Pts',(-19.4036149738155,19.6486063997904,124.636299304902)) ;
#92852=CARTESIAN_POINT('Ctrl Pts',(-18.9865388828078,19.668538247875,124.560857265651)) ;
#92853=CARTESIAN_POINT('Ctrl Pts',(-18.6207629984845,19.6884335162176,124.348399195064)) ;
#92854=CARTESIAN_POINT('Ctrl Pts',(-18.3486870513789,19.7083560146297,124.023705471699)) ;
#92855=CARTESIAN_POINT('Ctrl Pts',(-18.2035743919588,19.7283154965057,123.624866853166)) ;
#92856=CARTESIAN_POINT('Ctrl Pts',(-18.2031996570763,19.7481932489651,123.202277382126)) ;
#92857=CARTESIAN_POINT('Ctrl Pts',(-18.3460020872728,19.7680750396997,122.804297775666)) ;
#92858=CARTESIAN_POINT('Ctrl Pts',(-18.6192054318381,19.7881483785506,122.476459335084)) ;
#92859=CARTESIAN_POINT('Ctrl Pts',(-18.9830159386754,19.8079528457864,122.264237742757)) ;
#92860=CARTESIAN_POINT('Ctrl Pts',(-19.4008365480292,19.8279361861942,122.187322330753)) ;
#92861=CARTESIAN_POINT('Ctrl Pts',(-19.8183361695826,19.8478511507922,122.258043599631)) ;
#92862=CARTESIAN_POINT('Ctrl Pts',(-20.1864345402117,19.8677196855086,122.465512844636)) ;
#92863=CARTESIAN_POINT('Ctrl Pts',(-20.4635252854284,19.8877720697203,122.789401568453)) ;
#92864=CARTESIAN_POINT('Ctrl Pts',(-20.6120084940387,19.9075460335095,123.182939631322)) ;
#92865=CARTESIAN_POINT('Ctrl Pts',(-20.6176871989571,19.9276004125309,123.609141307482)) ;
#92866=CARTESIAN_POINT('Ctrl Pts',(-20.4791319038262,19.9473971501041,124.006748510168)) ;
#92867=CARTESIAN_POINT('Ctrl Pts',(-20.2119683630544,19.9673649624556,124.336599946701)) ;
#92868=CARTESIAN_POINT('Ctrl Pts',(-19.8479480211113,19.9873239385206,124.554908158912)) ;
#92869=CARTESIAN_POINT('Ctrl Pts',(-19.43276586831,20.007218856798,124.63587693085)) ;
#92870=CARTESIAN_POINT('Ctrl Pts',(-19.0147876330479,20.0271151692483,124.57082106987)) ;
#92871=CARTESIAN_POINT('Ctrl Pts',(-18.6435959232996,20.0470231026225,124.3672967635)) ;
#92872=CARTESIAN_POINT('Ctrl Pts',(-18.3636276541747,20.0669729929109,124.048670462292)) ;
#92873=CARTESIAN_POINT('Ctrl Pts',(-18.2093280448244,20.0868502234122,123.655155528142)) ;
#92874=CARTESIAN_POINT('Ctrl Pts',(-18.1983048045241,20.1068328922832,123.230434038346)) ;
#92875=CARTESIAN_POINT('Ctrl Pts',(-18.3328374001003,20.1267657788636,122.828470876827)) ;
#92876=CARTESIAN_POINT('Ctrl Pts',(-18.5959298858172,20.1466785248815,122.496768303889)) ;
#92877=CARTESIAN_POINT('Ctrl Pts',(-18.8956764765838,20.1632482462234,122.311681543742)) ;
#92878=CARTESIAN_POINT('Ctrl Pts',(-19.1634853725372,20.1765482575283,122.231185626866)) ;
#92879=CARTESIAN_POINT('Ctrl Pts',(-19.4404546659707,20.1898184452782,122.19809994678)) ;
#92880=CARTESIAN_POINT('Ctrl Pts',(-19.7904976855071,20.2064458276436,122.24823930975)) ;
#92881=CARTESIAN_POINT('Ctrl Pts',(-20.1021495885334,20.2230681173888,122.414851945115)) ;
#92882=CARTESIAN_POINT('Ctrl Pts',(-20.3055386175486,20.2363133317834,122.605073534047)) ;
#92883=CARTESIAN_POINT('Ctrl Pts',(-20.4311937960424,20.246225296744,122.771317113162)) ;
#92884=CARTESIAN_POINT('Ctrl Pts',(-20.5272487078393,20.2562839199085,122.959681452955)) ;
#92885=CARTESIAN_POINT('Ctrl Pts',(-20.5881006030648,20.2661240340243,123.157431331348)) ;
#92886=CARTESIAN_POINT('Ctrl Pts',(-20.6144821807902,20.2761898189819,123.367363495084)) ;
#92887=CARTESIAN_POINT('Ctrl Pts',(-20.6041090142429,20.2860731367698,123.574910063301)) ;
#92888=CARTESIAN_POINT('Ctrl Pts',(-20.5578169059943,20.2960625746284,123.779732855571)) ;
#92889=CARTESIAN_POINT('Ctrl Pts',(-20.4767917203888,20.3060262886811,123.972907200865)) ;
#92890=CARTESIAN_POINT('Ctrl Pts',(-20.3632827563932,20.3160213003403,124.149756073502)) ;
#92891=CARTESIAN_POINT('Ctrl Pts',(-20.2199777193418,20.3260575920346,124.304604687197)) ;
#92892=CARTESIAN_POINT('Ctrl Pts',(-20.0553288039776,20.335903969728,124.43008623397)) ;
#92893=CARTESIAN_POINT('Ctrl Pts',(-19.8690271796921,20.3458889138787,124.526746895698)) ;
#92894=CARTESIAN_POINT('Ctrl Pts',(-19.6697103347289,20.3558258850087,124.589424862788)) ;
#92895=CARTESIAN_POINT('Ctrl Pts',(-19.4602253129189,20.3658756696404,124.616732470545)) ;
#92896=CARTESIAN_POINT('Ctrl Pts',(-19.2533240604051,20.3757261317179,124.60759574013)) ;
#92897=CARTESIAN_POINT('Ctrl Pts',(-19.0485801942449,20.3856981452383,124.5626614221)) ;
#92898=CARTESIAN_POINT('Ctrl Pts',(-18.8542534156056,20.3956932923577,124.482625679858)) ;
#92899=CARTESIAN_POINT('Ctrl Pts',(-18.6762666665279,20.4057272620938,124.369439159579)) ;
#92900=CARTESIAN_POINT('Ctrl Pts',(-18.5231567827763,20.4155828077644,124.229814805404)) ;
#92901=CARTESIAN_POINT('Ctrl Pts',(-18.3945758011845,20.4255815647777,124.063565077421)) ;
#92902=CARTESIAN_POINT('Ctrl Pts',(-18.2976014683267,20.4354787000148,123.879441178517)) ;
#92903=CARTESIAN_POINT('Ctrl Pts',(-18.2330490446719,20.4455317958545,123.678215667784)) ;
#92904=CARTESIAN_POINT('Ctrl Pts',(-18.2048744098774,20.4554153045851,123.472337909635)) ;
#92905=CARTESIAN_POINT('Ctrl Pts',(-18.2124727941934,20.4654101772312,123.262357966266)) ;
#92906=CARTESIAN_POINT('Ctrl Pts',(-18.2568500139879,20.4754301388669,123.05642219874)) ;
#92907=CARTESIAN_POINT('Ctrl Pts',(-18.3352337516257,20.4853355026667,122.863498934385)) ;
#92908=CARTESIAN_POINT('Ctrl Pts',(-18.4459506926061,20.4952760902742,122.686271473277)) ;
#92909=CARTESIAN_POINT('Ctrl Pts',(-18.5865698044583,20.5052789083749,122.529879028359)) ;
#92910=CARTESIAN_POINT('Ctrl Pts',(-18.7529194278954,20.515313620099,122.400158061147)) ;
#92911=CARTESIAN_POINT('Ctrl Pts',(-18.9355983775793,20.5251585268363,122.302840174493)) ;
#92912=CARTESIAN_POINT('Ctrl Pts',(-19.1350505969826,20.5351443794053,122.237440607211)) ;
#92913=CARTESIAN_POINT('Ctrl Pts',(-19.341816666676,20.5450791878184,122.207660399939)) ;
#92914=CARTESIAN_POINT('Ctrl Pts',(-19.5531166856646,20.5551367148994,122.214501577073)) ;
#92915=CARTESIAN_POINT('Ctrl Pts',(-19.7552823842387,20.5649583698965,122.25660977831)) ;
#92916=CARTESIAN_POINT('Ctrl Pts',(-19.9517518356033,20.5750144140696,122.334626537221)) ;
#92917=CARTESIAN_POINT('Ctrl Pts',(-20.129451145617,20.5849551541147,122.444634049195)) ;
#92918=CARTESIAN_POINT('Ctrl Pts',(-20.2852058385497,20.5948592751876,122.582819934933)) ;
#92919=CARTESIAN_POINT('Ctrl Pts',(-20.4163627074734,20.6049068163418,122.748380027418)) ;
#92920=CARTESIAN_POINT('Ctrl Pts',(-20.5154483150305,20.6148055679422,122.931410766274)) ;
#92921=CARTESIAN_POINT('Ctrl Pts',(-20.5823151997651,20.624854046908,123.131775210439)) ;
#92922=CARTESIAN_POINT('Ctrl Pts',(-20.6129012294485,20.6347415439918,123.337400833468)) ;
#92923=CARTESIAN_POINT('Ctrl Pts',(-20.6076505390634,20.6447346342898,123.547403029367)) ;
#92924=CARTESIAN_POINT('Ctrl Pts',(-20.5661097282757,20.6546868043501,123.752476414149)) ;
#92925=CARTESIAN_POINT('Ctrl Pts',(-20.4899748034318,20.6646252242646,123.947032280125)) ;
#92926=CARTESIAN_POINT('Ctrl Pts',(-20.3808873625602,20.6746103543502,124.126405169006)) ;
#92927=CARTESIAN_POINT('Ctrl Pts',(-20.2413837782578,20.6846470437643,124.284693812174)) ;
#92928=CARTESIAN_POINT('Ctrl Pts',(-20.079686612651,20.6945017277568,124.414245628095)) ;
#92929=CARTESIAN_POINT('Ctrl Pts',(-19.8954680780183,20.7045012118047,124.515444101744)) ;
#92930=CARTESIAN_POINT('Ctrl Pts',(-19.6985589528749,20.7143963005816,124.582645265439)) ;
#92931=CARTESIAN_POINT('Ctrl Pts',(-19.4895929944476,20.7244568552277,124.615139995607)) ;
#92932=CARTESIAN_POINT('Ctrl Pts',(-19.2825548327521,20.7343061196006,124.611063575598)) ;
#92933=CARTESIAN_POINT('Ctrl Pts',(-19.075615702001,20.7443333720484,124.57090628253)) ;
#92934=CARTESIAN_POINT('Ctrl Pts',(-18.8789572197511,20.7543616696186,124.494897181618)) ;
#92935=CARTESIAN_POINT('Ctrl Pts',(-18.7015724822061,20.7642077986246,124.38822692672)) ;
#92936=CARTESIAN_POINT('Ctrl Pts',(-18.5427085218804,20.7742017039867,124.250730190685)) ;
#92937=CARTESIAN_POINT('Ctrl Pts',(-18.4100202997382,20.7842258016697,124.087002462897)) ;
#92938=CARTESIAN_POINT('Ctrl Pts',(-18.3089182753878,20.7941156295238,123.905320005835)) ;
#92939=CARTESIAN_POINT('Ctrl Pts',(-18.2399098922842,20.8041076109542,123.706924571269)) ;
#92940=CARTESIAN_POINT('Ctrl Pts',(-18.2065962288079,20.81405461572,123.500477659669)) ;
#92941=CARTESIAN_POINT('Ctrl Pts',(-18.2092510420346,20.8240042671098,123.291312990658)) ;
#92942=CARTESIAN_POINT('Ctrl Pts',(-18.2486917521182,20.8340412700872,123.084028440035)) ;
#92943=CARTESIAN_POINT('Ctrl Pts',(-18.3222881522907,20.8439301785222,122.889587486507)) ;
#92944=CARTESIAN_POINT('Ctrl Pts',(-18.4292737419995,20.8539195109997,122.708880730536)) ;
#92945=CARTESIAN_POINT('Ctrl Pts',(-18.5657078577571,20.8638780664368,122.550089103636)) ;
#92946=CARTESIAN_POINT('Ctrl Pts',(-18.7263705662023,20.8737776376373,122.417776084193)) ;
#92947=CARTESIAN_POINT('Ctrl Pts',(-18.9102889662095,20.8838255628893,122.313916753173)) ;
#92948=CARTESIAN_POINT('Ctrl Pts',(-19.106418162168,20.8937208624153,122.244464761771)) ;
#92949=CARTESIAN_POINT('Ctrl Pts',(-19.3150200502788,20.9037827188633,122.20952718984)) ;
#92950=CARTESIAN_POINT('Ctrl Pts',(-19.5219709300208,20.9136265652799,122.211259221192)) ;
#92951=CARTESIAN_POINT('Ctrl Pts',(-19.7280504585221,20.923589514408,122.248639607825)) ;
#92952=CARTESIAN_POINT('Ctrl Pts',(-19.9258060260669,20.933623550836,122.322083785571)) ;
#92953=CARTESIAN_POINT('Ctrl Pts',(-20.1052484445707,20.943510977794,122.426997611352)) ;
#92954=CARTESIAN_POINT('Ctrl Pts',(-20.2660567174591,20.9535254121304,122.562908261672)) ;
#92955=CARTESIAN_POINT('Ctrl Pts',(-20.4006745637189,20.9635603567653,122.725323843914)) ;
#92956=CARTESIAN_POINT('Ctrl Pts',(-20.5034505527534,20.9733927067963,122.904697980723)) ;
#92957=CARTESIAN_POINT('Ctrl Pts',(-20.5752878262504,20.9834681459136,123.103919059865)) ;
#92958=CARTESIAN_POINT('Ctrl Pts',(-20.6107746352119,20.9933206111482,123.308030768185)) ;
#92959=CARTESIAN_POINT('Ctrl Pts',(-20.6104406120429,21.003393488725,123.519758493893)) ;
#92960=CARTESIAN_POINT('Ctrl Pts',(-20.574159530213,21.0132360849175,123.723492672765)) ;
#92961=CARTESIAN_POINT('Ctrl Pts',(-20.5027305980759,21.0232164690328,123.920769582225)) ;
#92962=CARTESIAN_POINT('Ctrl Pts',(-20.3973760508536,21.0332349496816,124.103140675449)) ;
#92963=CARTESIAN_POINT('Ctrl Pts',(-20.2641044963282,21.043118264682,124.262579969479)) ;
#92964=CARTESIAN_POINT('Ctrl Pts',(-20.1021843516698,21.0531865617724,124.39885224005)) ;
#92965=CARTESIAN_POINT('Ctrl Pts',(-19.9234578857869,21.0630166301447,124.502677746142)) ;
#92966=CARTESIAN_POINT('Ctrl Pts',(-19.7249073728143,21.0730834226131,124.575830404009)) ;
#92967=CARTESIAN_POINT('Ctrl Pts',(-19.5202526014126,21.0829727561017,124.612656971211)) ;
#92968=CARTESIAN_POINT('Ctrl Pts',(-19.3100164219051,21.0929748875177,124.613728177772)) ;
#92969=CARTESIAN_POINT('Ctrl Pts',(-19.104313532682,21.1028987571387,124.578676687678)) ;
#92970=CARTESIAN_POINT('Ctrl Pts',(-18.9055379818956,21.1129422726559,124.507558469863)) ;
#92971=CARTESIAN_POINT('Ctrl Pts',(-18.7248962749074,21.1228244855442,124.404861360721)) ;
#92972=CARTESIAN_POINT('Ctrl Pts',(-18.5618819563526,21.1328925627636,124.269913203078)) ;
#92973=CARTESIAN_POINT('Ctrl Pts',(-18.4277131905557,21.1427310674978,124.112452222884)) ;
#92974=CARTESIAN_POINT('Ctrl Pts',(-18.3203059258031,21.1527938359272,123.930225142098)) ;
#92975=CARTESIAN_POINT('Ctrl Pts',(-18.2475914361445,21.16269082921,123.735266093475)) ;
#92976=CARTESIAN_POINT('Ctrl Pts',(-18.2090196056802,21.1726220568447,123.53007978399)) ;
#92977=CARTESIAN_POINT('Ctrl Pts',(-18.206865902174,21.1826642154869,123.318975246632)) ;
#92978=CARTESIAN_POINT('Ctrl Pts',(-18.2407188874795,21.1925509250179,123.113892030568)) ;
#92979=CARTESIAN_POINT('Ctrl Pts',(-18.31006688254,21.2025438974465,122.915594107731)) ;
#92980=CARTESIAN_POINT('Ctrl Pts',(-18.4123920866279,21.2124900919831,122.733245377864)) ;
#92981=CARTESIAN_POINT('Ctrl Pts',(-18.5444723439432,21.2224354668346,122.571139731623)) ;
#92982=CARTESIAN_POINT('Ctrl Pts',(-18.7046180314311,21.2324903861945,122.433199211354)) ;
#92983=CARTESIAN_POINT('Ctrl Pts',(-18.8819052194526,21.242311905638,122.32730255838)) ;
#92984=CARTESIAN_POINT('Ctrl Pts',(-19.0795341225873,21.2523776744049,122.251751654709)) ;
#92985=CARTESIAN_POINT('Ctrl Pts',(-19.2839833999298,21.26227959606,122.21237155369)) ;
#92986=CARTESIAN_POINT('Ctrl Pts',(-19.4950720949198,21.272322654881,122.208856213682)) ;
#92987=CARTESIAN_POINT('Ctrl Pts',(-19.7007256999796,21.2822286489237,122.241706218892)) ;
#92988=CARTESIAN_POINT('Ctrl Pts',(-19.8983768064677,21.2921664220055,122.309400713787)) ;
#92989=CARTESIAN_POINT('Ctrl Pts',(-20.0830478736539,21.3022067857378,122.411625288748)) ;
#92990=CARTESIAN_POINT('Ctrl Pts',(-20.2447725390836,21.3120941294613,122.542225491342)) ;
#92991=CARTESIAN_POINT('Ctrl Pts',(-20.3830581645172,21.32208636003,122.700338499816)) ;
#92992=CARTESIAN_POINT('Ctrl Pts',(-20.4912786799857,21.3320348878136,122.879326370199)) ;
#92993=CARTESIAN_POINT('Ctrl Pts',(-20.5669519562482,21.3419716715369,123.074021933852)) ;
#92994=CARTESIAN_POINT('Ctrl Pts',(-20.6081294035069,21.3519546723339,123.27984423291)) ;
#92995=CARTESIAN_POINT('Ctrl Pts',(-20.612582513455,21.3619985591746,123.490926845496)) ;
#92996=CARTESIAN_POINT('Ctrl Pts',(-20.5814885242902,21.3718265827492,123.695222667967)) ;
#92997=CARTESIAN_POINT('Ctrl Pts',(-20.5138274751525,21.3819038309628,123.895933159285)) ;
#92998=CARTESIAN_POINT('Ctrl Pts',(-20.4147142104138,21.3917533862681,124.077802364795)) ;
#92999=CARTESIAN_POINT('Ctrl Pts',(-20.2825949674431,21.4018360944658,124.243492472331)) ;
#93000=CARTESIAN_POINT('Ctrl Pts',(-20.1280211187702,21.4116486873923,124.380174251512)) ;
#93001=CARTESIAN_POINT('Ctrl Pts',(-19.9477576259279,21.4217158796502,124.490980574694)) ;
#93002=CARTESIAN_POINT('Ctrl Pts',(-19.7541625513692,21.4316147091128,124.567467521575)) ;
#93003=CARTESIAN_POINT('Ctrl Pts',(-19.5471445694448,21.441668700303,124.609901982404)) ;
#93004=CARTESIAN_POINT('Ctrl Pts',(-19.3396514879245,21.4515404250862,124.615828021974)) ;
#93005=CARTESIAN_POINT('Ctrl Pts',(-19.1302180618309,21.4616108672164,124.585090730345)) ;
#93006=CARTESIAN_POINT('Ctrl Pts',(-18.9339576917746,21.4714439456467,124.520098552817)) ;
#93007=CARTESIAN_POINT('Ctrl Pts',(-18.7480491375377,21.4814744191481,124.420590545696)) ;
#93008=CARTESIAN_POINT('Ctrl Pts',(-18.5825887816303,21.4915060184468,124.289804563175)) ;
#93009=CARTESIAN_POINT('Ctrl Pts',(-18.4448685819792,21.501335719485,124.135752812325)) ;
#93010=CARTESIAN_POINT('Ctrl Pts',(-18.33367553148,21.5113251575414,123.95758788387)) ;
#93011=CARTESIAN_POINT('Ctrl Pts',(-18.2551799398272,21.5213690607575,123.761568607706)) ;
#93012=CARTESIAN_POINT('Ctrl Pts',(-18.2124473470775,21.531190581571,123.559558762886)) ;
#93013=CARTESIAN_POINT('Ctrl Pts',(-18.2047822889441,21.5412263058181,123.34872005525)) ;
#93014=CARTESIAN_POINT('Ctrl Pts',(-18.234346097043,21.5512484597506,123.140091282783)) ;
#93015=CARTESIAN_POINT('Ctrl Pts',(-18.2983110621091,21.5611106915079,122.942886810719)) ;
#93016=CARTESIAN_POINT('Ctrl Pts',(-18.3959902964386,21.5710697619658,122.757690821319)) ;
#93017=CARTESIAN_POINT('Ctrl Pts',(-18.5255720550115,21.581104934342,122.591216512545)) ;
#93018=CARTESIAN_POINT('Ctrl Pts',(-18.6794900206826,21.5909853195003,122.451700738858)) ;
#93019=CARTESIAN_POINT('Ctrl Pts',(-18.8583520010264,21.6010420340942,122.339007617028)) ;
#93020=CARTESIAN_POINT('Ctrl Pts',(-19.0506455463803,21.6109213026663,122.260495050718)) ;
#93021=CARTESIAN_POINT('Ctrl Pts',(-19.2558150100151,21.6209122601519,122.215517104527)) ;
#93022=CARTESIAN_POINT('Ctrl Pts',(-19.4667419928137,21.6309529187871,122.207269166301)) ;
#93023=CARTESIAN_POINT('Ctrl Pts',(-19.671611306749,21.6407858984951,122.234836706111)) ;
#93024=CARTESIAN_POINT('Ctrl Pts',(-19.8719733222595,21.6507790317448,122.29800611631)) ;
#93025=CARTESIAN_POINT('Ctrl Pts',(-20.0588577647068,21.6608110841282,122.395778370731)) ;
#93026=CARTESIAN_POINT('Ctrl Pts',(-20.2232889185199,21.6706763130795,122.522158713432)) ;
#93027=CARTESIAN_POINT('Ctrl Pts',(-20.3650985195692,21.6806382543227,122.676281555765)) ;
#93028=CARTESIAN_POINT('Ctrl Pts',(-20.4785231200122,21.6906729693595,122.854145180264)) ;
#93029=CARTESIAN_POINT('Ctrl Pts',(-20.5584654849309,21.7005587397035,123.046012225195)) ;
#93030=CARTESIAN_POINT('Ctrl Pts',(-20.6046775909707,21.7106213370923,123.252424731187)) ;
#93031=CARTESIAN_POINT('Ctrl Pts',(-20.6142383738088,21.7204717489275,123.459306777541)) ;
#93032=CARTESIAN_POINT('Ctrl Pts',(-20.587797478846,21.7304989182135,123.668438871735)) ;
#93033=CARTESIAN_POINT('Ctrl Pts',(-20.5249128780641,21.7405263989276,123.869661185407)) ;
#93034=CARTESIAN_POINT('Ctrl Pts',(-20.4301887540128,21.7503694515069,124.053631115925)) ;
#93035=CARTESIAN_POINT('Ctrl Pts',(-20.3034636380379,21.7603633549455,124.221213703478)) ;
#93036=CARTESIAN_POINT('Ctrl Pts',(-20.1487862324558,21.7703904777219,124.364442194746)) ;
#93037=CARTESIAN_POINT('Ctrl Pts',(-19.9741429213597,21.780281182614,124.47730256004)) ;
#93038=CARTESIAN_POINT('Ctrl Pts',(-19.780720987989,21.7902732094643,124.559229104381)) ;
#93039=CARTESIAN_POINT('Ctrl Pts',(-19.5769360767532,21.8002191909528,124.606050632827)) ;
#93040=CARTESIAN_POINT('Ctrl Pts',(-19.3681010650657,21.8101663635748,124.617200646608)) ;
#93041=CARTESIAN_POINT('Ctrl Pts',(-19.1584464126587,21.8202143049009,124.591432573086)) ;
#93042=CARTESIAN_POINT('Ctrl Pts',(-18.9604177626516,21.8300619387087,124.531049432518)) ;
#93043=CARTESIAN_POINT('Ctrl Pts',(-18.7734573807133,21.8400236533937,124.436702689739)) ;
#93044=CARTESIAN_POINT('Ctrl Pts',(-18.6047340145598,21.8500522862723,124.310256630304)) ;
#93045=CARTESIAN_POINT('Ctrl Pts',(-18.4621942150218,21.8599626118074,124.158312586549)) ;
#93046=CARTESIAN_POINT('Ctrl Pts',(-18.3474585442045,21.8698974422791,123.983782756746)) ;
#93047=CARTESIAN_POINT('Ctrl Pts',(-18.2640502912331,21.8799387746611,123.78985926928)) ;
#93048=CARTESIAN_POINT('Ctrl Pts',(-18.2162240830318,21.8898316480999,123.58745555314)) ;
#93049=CARTESIAN_POINT('Ctrl Pts',(-18.2036438407707,21.8998008139178,123.378240612157)) ;
#93050=CARTESIAN_POINT('Ctrl Pts',(-18.2280682294196,21.9098295476343,123.168844784421)) ;
#93051=CARTESIAN_POINT('Ctrl Pts',(-18.3069945112889,21.9230220664055,122.902886831599)) ;
#93052=CARTESIAN_POINT('Ctrl Pts',(-18.4552999600095,21.9363819344482,122.660697707315)) ;
#93053=CARTESIAN_POINT('Ctrl Pts',(-18.6570216056765,21.949607271597,122.469325654628)) ;
#93054=CARTESIAN_POINT('Ctrl Pts',(-18.8316797947684,21.9595884974377,122.353021524023)) ;
#93055=CARTESIAN_POINT('Ctrl Pts',(-19.0250825772389,21.9696240644205,122.268736505731)) ;
#93056=CARTESIAN_POINT('Ctrl Pts',(-19.2265882388558,21.9794871423826,122.219744505604)) ;
#93057=CARTESIAN_POINT('Ctrl Pts',(-19.4378387744727,21.9895574411837,122.206163830183)) ;
#93058=CARTESIAN_POINT('Ctrl Pts',(-19.643505555205,21.9993997397515,122.228957332354)) ;
#93059=CARTESIAN_POINT('Ctrl Pts',(-19.8446819721285,22.0093604379213,122.287067936604)) ;
#93060=CARTESIAN_POINT('Ctrl Pts',(-20.033984583094,22.0193984721008,122.38031752728)) ;
#93061=CARTESIAN_POINT('Ctrl Pts',(-20.2016926408589,22.0292722089473,122.502684395899)) ;
#93062=CARTESIAN_POINT('Ctrl Pts',(-20.348434425126,22.0393439928725,122.655289376748)) ;
#93063=CARTESIAN_POINT('Ctrl Pts',(-20.4637741378317,22.0491761140737,122.826843918411)) ;
#93064=CARTESIAN_POINT('Ctrl Pts',(-20.5497920398545,22.0592091380992,123.01942208058)) ;
#93065=CARTESIAN_POINT('Ctrl Pts',(-20.6004603830163,22.0692250182958,123.223814326905)) ;
#93066=CARTESIAN_POINT('Ctrl Pts',(-20.6150640025834,22.07910853739,123.431083510187)) ;
#93067=CARTESIAN_POINT('Ctrl Pts',(-20.593494061192,22.0890989497537,123.639987676486)) ;
#93068=CARTESIAN_POINT('Ctrl Pts',(-20.5172182747527,22.1023621129571,123.908212271559)) ;
#93069=CARTESIAN_POINT('Ctrl Pts',(-20.3727555111962,22.1156396832083,124.150777474727)) ;
#93070=CARTESIAN_POINT('Ctrl Pts',(-20.1718123417911,22.1289699857149,124.346093874613)) ;
#93071=CARTESIAN_POINT('Ctrl Pts',(-19.9998410396279,22.1388686675313,124.463290461051)) ;
#93072=CARTESIAN_POINT('Ctrl Pts',(-19.8085084880358,22.1488581825789,124.549850711102)) ;
#93073=CARTESIAN_POINT('Ctrl Pts',(-19.6058755401531,22.1588062343539,124.601655314269)) ;
#93074=CARTESIAN_POINT('Ctrl Pts',(-19.3975125045008,22.1687476376324,124.617740356275)) ;
#93075=CARTESIAN_POINT('Ctrl Pts',(-19.1194368110391,22.1820343024133,124.590882680961)) ;
#93076=CARTESIAN_POINT('Ctrl Pts',(-18.7886603018455,22.1986447240681,124.467217873756)) ;
#93077=CARTESIAN_POINT('Ctrl Pts',(-18.4662721824699,22.2185559863189,124.192767655879)) ;
#93078=CARTESIAN_POINT('Ctrl Pts',(-18.2564052108504,22.2385001154838,123.824248329154)) ;
#93079=CARTESIAN_POINT('Ctrl Pts',(-18.1850298167595,22.258423278089,123.406724031906)) ;
#93080=CARTESIAN_POINT('Ctrl Pts',(-18.2596166140788,22.2783134004955,122.990368787933)) ;
#93081=CARTESIAN_POINT('Ctrl Pts',(-18.4732461778433,22.2983183540956,122.622623813905)) ;
#93082=CARTESIAN_POINT('Ctrl Pts',(-18.7967224956911,22.3181566111112,122.351774759817)) ;
#93083=CARTESIAN_POINT('Ctrl Pts',(-19.1960528209252,22.3381509118978,122.206072263074)) ;
#93084=CARTESIAN_POINT('Ctrl Pts',(-19.6188774949697,22.3580361539422,122.205770409329)) ;
#93085=CARTESIAN_POINT('Ctrl Pts',(-20.0166123708548,22.3779111004182,122.348576452915)) ;
#93086=CARTESIAN_POINT('Ctrl Pts',(-20.3441439289911,22.3979441703592,122.620968139664)) ;
#93087=CARTESIAN_POINT('Ctrl Pts',(-20.5570158953908,22.4178326772596,122.986324907579)) ;
#93088=CARTESIAN_POINT('Ctrl Pts',(-20.63376602721,22.4376875370409,123.401523750881)) ;
#93089=CARTESIAN_POINT('Ctrl Pts',(-20.5628771445942,22.4577383708286,123.821821360625)) ;
#93090=CARTESIAN_POINT('Ctrl Pts',(-20.3561025774124,22.4775043127179,124.187848336613)) ;
#93091=CARTESIAN_POINT('Ctrl Pts',(-20.0335850425227,22.4975170441772,124.465242851692)) ;
#93092=CARTESIAN_POINT('Ctrl Pts',(-19.6377262102583,22.5174098791208,124.614575343707)) ;
#93093=CARTESIAN_POINT('Ctrl Pts',(-19.2145950747695,22.5373169024603,124.620562106581)) ;
#93094=CARTESIAN_POINT('Ctrl Pts',(-18.8143052159409,22.557232167361,124.482124393492)) ;
#93095=CARTESIAN_POINT('Ctrl Pts',(-18.4838083293935,22.5772638595207,124.213504396817)) ;
#93096=CARTESIAN_POINT('Ctrl Pts',(-18.266814494246,22.5971069060937,123.851612989797)) ;
#93097=CARTESIAN_POINT('Ctrl Pts',(-18.1851080172229,22.6170234539935,123.436153599146)) ;
#93098=CARTESIAN_POINT('Ctrl Pts',(-18.2502202399435,22.6369556969848,123.017333953264)) ;
#93099=CARTESIAN_POINT('Ctrl Pts',(-18.4538259242092,22.6568595317941,122.646346956215)) ;
#93100=CARTESIAN_POINT('Ctrl Pts',(-18.7714168946977,22.6767599319816,122.366744911555)) ;
#93101=CARTESIAN_POINT('Ctrl Pts',(-19.166285915724,22.6967096083609,122.211749714372)) ;
#93102=CARTESIAN_POINT('Ctrl Pts',(-19.589972383929,22.7166421325813,122.200906821069)) ;
#93103=CARTESIAN_POINT('Ctrl Pts',(-19.9918128903869,22.7365621415675,122.334876945434)) ;
#93104=CARTESIAN_POINT('Ctrl Pts',(-20.3243318664466,22.7565190477437,122.598424801624)) ;
#93105=CARTESIAN_POINT('Ctrl Pts',(-20.5465556808839,22.7764048872452,122.958240044023)) ;
#93106=CARTESIAN_POINT('Ctrl Pts',(-20.6329370095497,22.796376059381,123.373906325153)) ;
#93107=CARTESIAN_POINT('Ctrl Pts',(-20.5733229208069,22.8161902563654,123.791036866964)) ;
#93108=CARTESIAN_POINT('Ctrl Pts',(-20.3738395604906,22.8361714423337,124.16606417652)) ;
#93109=CARTESIAN_POINT('Ctrl Pts',(-20.1119254984363,22.8527469477229,124.401935987589)) ;
#93110=CARTESIAN_POINT('Ctrl Pts',(-19.8627907051398,22.8660563955865,124.529374391931)) ;
#93111=CARTESIAN_POINT('Ctrl Pts',(-19.5941634357807,22.8794240933631,124.611788225759)) ;
#93112=CARTESIAN_POINT('Ctrl Pts',(-19.2437164503592,22.895914665029,124.624712075177)) ;
#93113=CARTESIAN_POINT('Ctrl Pts',(-18.8402567476097,22.9158349373618,124.496012765143)) ;
#93114=CARTESIAN_POINT('Ctrl Pts',(-18.5605856920532,22.9324519730828,124.280092618968)) ;
#93115=CARTESIAN_POINT('Ctrl Pts',(-18.3909770737706,22.9457428233639,124.057986522721)) ;
#93116=CARTESIAN_POINT('Ctrl Pts',(-18.2945642787171,22.9557118685184,123.871929176122)) ;
#93117=CARTESIAN_POINT('Ctrl Pts',(-18.2319237526866,22.965615259152,123.673347903885)) ;
#93118=CARTESIAN_POINT('Ctrl Pts',(-18.2044109629437,22.9756730452647,123.46372521076)) ;
#93119=CARTESIAN_POINT('Ctrl Pts',(-18.2133455804091,22.9855250819144,123.256767938928)) ;
#93120=CARTESIAN_POINT('Ctrl Pts',(-18.2735481450176,22.9988902060576,122.982370184821)) ;
#93121=CARTESIAN_POINT('Ctrl Pts',(-18.4029730647199,23.0121162690207,122.732648967479)) ;
#93122=CARTESIAN_POINT('Ctrl Pts',(-18.5911586333151,23.0254199173029,122.525747384851)) ;
#93123=CARTESIAN_POINT('Ctrl Pts',(-18.7572840479438,23.0354114484659,122.397160345166)) ;
#93124=CARTESIAN_POINT('Ctrl Pts',(-18.9442034529857,23.0454508962652,122.29917135121)) ;
#93125=CARTESIAN_POINT('Ctrl Pts',(-19.1413113374311,23.0552946717791,122.236069991854)) ;
#93126=CARTESIAN_POINT('Ctrl Pts',(-19.3492334981036,23.0652803131667,122.207338844066)) ;
#93127=CARTESIAN_POINT('Ctrl Pts',(-19.5580294696131,23.0752170975285,122.21499628788)) ;
#93128=CARTESIAN_POINT('Ctrl Pts',(-19.7645716223827,23.0852669319959,122.2593847219)) ;
#93129=CARTESIAN_POINT('Ctrl Pts',(-19.956478859204,23.095117381499,122.337250989053)) ;
#93130=CARTESIAN_POINT('Ctrl Pts',(-20.1343708699036,23.1050893954811,122.448127388525)) ;
#93131=CARTESIAN_POINT('Ctrl Pts',(-20.2906970657554,23.1150845533282,122.588593762462)) ;
#93132=CARTESIAN_POINT('Ctrl Pts',(-20.4205292649936,23.1251184796919,122.754827851092)) ;
#93133=CARTESIAN_POINT('Ctrl Pts',(-20.5180699479816,23.1349741881243,122.937651944192)) ;
#93134=CARTESIAN_POINT('Ctrl Pts',(-20.5835848106388,23.144972337463,123.137338627828)) ;
#93135=CARTESIAN_POINT('Ctrl Pts',(-20.6133315601013,23.1548717406366,123.343349279498)) ;
#93136=CARTESIAN_POINT('Ctrl Pts',(-20.6068042955674,23.164922937525,123.554533958808)) ;
#93137=CARTESIAN_POINT('Ctrl Pts',(-20.5644542804558,23.1748052613379,123.757945285797)) ;
#93138=CARTESIAN_POINT('Ctrl Pts',(-20.4869988566023,23.1848001569945,123.953265947771)) ;
#93139=CARTESIAN_POINT('Ctrl Pts',(-20.3762451153194,23.194821256377,124.13249196555)) ;
#93140=CARTESIAN_POINT('Ctrl Pts',(-20.2377780682512,23.2047285242391,124.288078667815)) ;
#93141=CARTESIAN_POINT('Ctrl Pts',(-20.0741559131026,23.2146668680644,124.41798671846)) ;
#93142=CARTESIAN_POINT('Ctrl Pts',(-19.8892906416545,23.2246702873648,124.518297175793)) ;
#93143=CARTESIAN_POINT('Ctrl Pts',(-19.6891176860214,23.2347048380719,124.584849932306)) ;
#93144=CARTESIAN_POINT('Ctrl Pts',(-19.4844008567411,23.2445497876775,124.615406104496)) ;
#93145=CARTESIAN_POINT('Ctrl Pts',(-19.2745631934654,23.2545356297904,124.610269779593)) ;
#93146=CARTESIAN_POINT('Ctrl Pts',(-19.0697563387047,23.2644704371595,124.569121010592)) ;
#93147=CARTESIAN_POINT('Ctrl Pts',(-18.8729354077247,23.2745279788728,124.49194530849)) ;
#93148=CARTESIAN_POINT('Ctrl Pts',(-18.6965271275385,23.284349576385,124.384596043654)) ;
#93149=CARTESIAN_POINT('Ctrl Pts',(-18.537505207443,23.2944058358654,124.245310914228)) ;
#93150=CARTESIAN_POINT('Ctrl Pts',(-18.4068828184235,23.3043457721658,124.082183809851)) ;
#93151=CARTESIAN_POINT('Ctrl Pts',(-18.3063569604988,23.3142528929102,123.899773364579)) ;
#93152=CARTESIAN_POINT('Ctrl Pts',(-18.238182102266,23.3242957988355,123.699954793539)) ;
#93153=CARTESIAN_POINT('Ctrl Pts',(-18.2061315888392,23.3342035799347,123.494134506193)) ;
#93154=CARTESIAN_POINT('Ctrl Pts',(-18.2099782467636,23.3442139489371,123.283713240502)) ;
#93155=CARTESIAN_POINT('Ctrl Pts',(-18.2508047878305,23.3542447875059,123.076824776893)) ;
#93156=CARTESIAN_POINT('Ctrl Pts',(-18.3252380526444,23.3640976271456,122.883518211052)) ;
#93157=CARTESIAN_POINT('Ctrl Pts',(-18.4332307006835,23.3740856283106,122.703457545309)) ;
#93158=CARTESIAN_POINT('Ctrl Pts',(-18.570043155712,23.3840144472898,122.545803263845)) ;
#93159=CARTESIAN_POINT('Ctrl Pts',(-18.7328941528992,23.3940021500121,122.413240967094)) ;
#93160=CARTESIAN_POINT('Ctrl Pts',(-18.9173305839693,23.4040381498147,122.310793637475)) ;
#93161=CARTESIAN_POINT('Ctrl Pts',(-19.1130661739556,23.4138930196162,122.242836710272)) ;
#93162=CARTESIAN_POINT('Ctrl Pts',(-19.3205318000607,23.4238924500397,122.209140767178)) ;
#93163=CARTESIAN_POINT('Ctrl Pts',(-19.5285765182959,23.433787567505,122.211727966587)) ;
#93164=CARTESIAN_POINT('Ctrl Pts',(-19.7363643453883,23.4438480610219,122.251054376304)) ;
#93165=CARTESIAN_POINT('Ctrl Pts',(-19.9300969267165,23.4536975412231,122.324201636643)) ;
#93166=CARTESIAN_POINT('Ctrl Pts',(-20.1116481432256,23.4637239914869,122.431297533579)) ;
#93167=CARTESIAN_POINT('Ctrl Pts',(-20.2715506693218,23.473755281965,122.568801972181)) ;
#93168=CARTESIAN_POINT('Ctrl Pts',(-20.4029659088239,23.4835966696168,122.728604725613)) ;
#93169=CARTESIAN_POINT('Ctrl Pts',(-20.5066563534772,23.4936000705081,122.911544063028)) ;
#93170=CARTESIAN_POINT('Ctrl Pts',(-20.5768108983585,23.5035844532992,123.109415497325)) ;
#93171=CARTESIAN_POINT('Ctrl Pts',(-20.6115256227708,23.5136235433126,123.317573246483)) ;
#93172=CARTESIAN_POINT('Ctrl Pts',(-20.6098969894375,23.5234693522218,123.52457158236)) ;
#93173=CARTESIAN_POINT('Ctrl Pts',(-20.5722509395659,23.5334537750408,123.731041347267)) ;
#93174=CARTESIAN_POINT('Ctrl Pts',(-20.4997174059433,23.543393400282,123.927042123842)) ;
#93175=CARTESIAN_POINT('Ctrl Pts',(-20.3931719197641,23.5534330898006,124.109223143745)) ;
#93176=CARTESIAN_POINT('Ctrl Pts',(-20.2587341895538,23.5633212782192,124.267797382914)) ;
#93177=CARTESIAN_POINT('Ctrl Pts',(-20.0974322543525,23.5733108042213,124.402272320034)) ;
#93178=CARTESIAN_POINT('Ctrl Pts',(-19.9157158970275,23.5832693055765,124.506233898799)) ;
#93179=CARTESIAN_POINT('Ctrl Pts',(-19.7200317318683,23.5931688995801,124.577135520212)) ;
#93180=CARTESIAN_POINT('Ctrl Pts',(-19.511958597003,23.6032167877014,124.613440420387)) ;
#93181=CARTESIAN_POINT('Ctrl Pts',(-19.3038931117637,23.613112212947,124.613234240594)) ;
#93182=CARTESIAN_POINT('Ctrl Pts',(-19.0956394360566,23.6231736036475,124.576334619288)) ;
#93183=CARTESIAN_POINT('Ctrl Pts',(-18.9011715211872,23.6330191873342,124.505414756995)) ;
#93184=CARTESIAN_POINT('Ctrl Pts',(-18.7195047168646,23.6429821606434,124.401196107756)) ;
#93185=CARTESIAN_POINT('Ctrl Pts',(-18.5578392233142,23.6530078274692,124.265939530275)) ;
#93186=CARTESIAN_POINT('Ctrl Pts',(-18.4235465577687,23.6629223053355,124.106543747631)) ;
#93187=CARTESIAN_POINT('Ctrl Pts',(-18.3178150771585,23.6729108200105,123.9250945317)) ;
#93188=CARTESIAN_POINT('Ctrl Pts',(-18.2452273886237,23.6829549309259,123.726824520025)) ;
#93189=CARTESIAN_POINT('Ctrl Pts',(-18.2084622209874,23.6927830685205,123.523473745696)) ;
#93190=CARTESIAN_POINT('Ctrl Pts',(-18.2074439778871,23.7028596365794,123.31167785126)) ;
#93191=CARTESIAN_POINT('Ctrl Pts',(-18.2423298104587,23.7127117984836,123.107467698959)) ;
#93192=CARTESIAN_POINT('Ctrl Pts',(-18.3135158811486,23.7227847604404,122.908064141033)) ;
#93193=CARTESIAN_POINT('Ctrl Pts',(-18.4159003030267,23.7326273224433,122.728227460704)) ;
#93194=CARTESIAN_POINT('Ctrl Pts',(-18.5492444985137,23.7426077589371,122.56624045852)) ;
#93195=CARTESIAN_POINT('Ctrl Pts',(-18.7095634099869,23.7526260642615,122.429654359688)) ;
#93196=CARTESIAN_POINT('Ctrl Pts',(-18.888529532284,23.762510028181,122.324026238617)) ;
#93197=CARTESIAN_POINT('Ctrl Pts',(-19.0866746849107,23.7725759049195,122.249802045763)) ;
#93198=CARTESIAN_POINT('Ctrl Pts',(-19.2900277703076,23.7824150057804,122.211839220089)) ;
#93199=CARTESIAN_POINT('Ctrl Pts',(-19.5009280169213,23.7924480886462,122.209188897855)) ;
#93200=CARTESIAN_POINT('Ctrl Pts',(-19.7087890814224,23.8024697739216,122.243680915572)) ;
#93201=CARTESIAN_POINT('Ctrl Pts',(-19.9045118580242,23.8123364690201,122.31233133179)) ;
#93202=CARTESIAN_POINT('Ctrl Pts',(-20.0873423992775,23.8222963587547,122.414410667244)) ;
#93203=CARTESIAN_POINT('Ctrl Pts',(-20.2506734014014,23.8323313465801,122.547919056241)) ;
#93204=CARTESIAN_POINT('Ctrl Pts',(-20.3865972372764,23.8422180506544,122.705203000666)) ;
#93205=CARTESIAN_POINT('Ctrl Pts',(-20.4949915022532,23.8522831948873,122.886893090087)) ;
#93206=CARTESIAN_POINT('Ctrl Pts',(-20.5687253459054,23.8621224856159,123.080191817205)) ;
#93207=CARTESIAN_POINT('Ctrl Pts',(-20.6089362319602,23.8721850430543,123.28785664052)) ;
#93208=CARTESIAN_POINT('Ctrl Pts',(-20.6121978990031,23.8820820943064,123.495909786969)) ;
#93209=CARTESIAN_POINT('Ctrl Pts',(-20.5798621479707,23.8920133010547,123.702170605702)) ;
#93210=CARTESIAN_POINT('Ctrl Pts',(-20.5112278120771,23.9020554852735,123.901818256384)) ;
#93211=CARTESIAN_POINT('Ctrl Pts',(-20.4106814625519,23.9119421133844,124.083739072873)) ;
#93212=CARTESIAN_POINT('Ctrl Pts',(-20.2789510402383,23.9219353859168,124.247385499214)) ;
#93213=CARTESIAN_POINT('Ctrl Pts',(-20.1215140193318,23.9318804614583,124.384961368838)) ;
#93214=CARTESIAN_POINT('Ctrl Pts',(-19.9427040588716,23.9418300121866,124.493512735114)) ;
#93215=CARTESIAN_POINT('Ctrl Pts',(-19.7459483725956,23.9518693470345,124.569858320534)) ;
#93216=CARTESIAN_POINT('Ctrl Pts',(-19.5420958579486,23.9617554859785,124.610447514314)) ;
#93217=CARTESIAN_POINT('Ctrl Pts',(-19.3319860693722,23.9717535989522,124.61534345927)) ;
#93218=CARTESIAN_POINT('Ctrl Pts',(-19.1257788355429,23.9816733613046,124.584048463693)) ;
#93219=CARTESIAN_POINT('Ctrl Pts',(-18.9257658599301,23.9917127569173,124.516694255687)) ;
#93220=CARTESIAN_POINT('Ctrl Pts',(-18.7429093614432,24.0016219427055,124.416883451877)) ;
#93221=CARTESIAN_POINT('Ctrl Pts',(-18.5793682570161,24.011557126863,124.286955917705)) ;
#93222=CARTESIAN_POINT('Ctrl Pts',(-18.4395550076449,24.0215981842489,124.12880714073)) ;
#93223=CARTESIAN_POINT('Ctrl Pts',(-18.3308792312625,24.0314853422822,123.95160799929)) ;
#93224=CARTESIAN_POINT('Ctrl Pts',(-18.2534953404692,24.0414776219581,123.756326967307)) ;
#93225=CARTESIAN_POINT('Ctrl Pts',(-18.2114309389755,24.0514261390032,123.551439534161)) ;
#93226=CARTESIAN_POINT('Ctrl Pts',(-18.2052935463612,24.0613629165736,123.342645080243)) ;
#93227=CARTESIAN_POINT('Ctrl Pts',(-18.2353874848655,24.0713459527205,123.134912288496)) ;
#93228=CARTESIAN_POINT('Ctrl Pts',(-18.3018447079775,24.0813897043143,122.934516760273)) ;
#93229=CARTESIAN_POINT('Ctrl Pts',(-18.3995390927353,24.0912182335268,122.75241029189)) ;
#93230=CARTESIAN_POINT('Ctrl Pts',(-18.5304446989063,24.1012935944355,122.585941046542)) ;
#93231=CARTESIAN_POINT('Ctrl Pts',(-18.6848541056234,24.1111501933227,122.447684995541)) ;
#93232=CARTESIAN_POINT('Ctrl Pts',(-18.8644224668532,24.1212131873406,122.335908353526)) ;
#93233=CARTESIAN_POINT('Ctrl Pts',(-19.0571387458606,24.1310911216301,122.258444830493)) ;
#93234=CARTESIAN_POINT('Ctrl Pts',(-19.2627622836008,24.1410917691882,122.214785949569)) ;
#93235=CARTESIAN_POINT('Ctrl Pts',(-19.4711725606285,24.1510096156262,122.207393834254)) ;
#93236=CARTESIAN_POINT('Ctrl Pts',(-19.6803970262427,24.1610607326319,122.236738184022)) ;
#93237=CARTESIAN_POINT('Ctrl Pts',(-19.8778824262284,24.1709314679425,122.30059392637)) ;
#93238=CARTESIAN_POINT('Ctrl Pts',(-20.064951432352,24.1810021751855,122.399666043339)) ;
#93239=CARTESIAN_POINT('Ctrl Pts',(-20.2281336989988,24.1908351826373,122.526602593629)) ;
#93240=CARTESIAN_POINT('Ctrl Pts',(-20.3700097469884,24.2008656749396,122.682600116585)) ;
#93241=CARTESIAN_POINT('Ctrl Pts',(-20.4821469033699,24.210897270013,122.861226293759)) ;
#93242=CARTESIAN_POINT('Ctrl Pts',(-20.5603565412622,24.2207269691513,123.052490631286)) ;
#93243=CARTESIAN_POINT('Ctrl Pts',(-20.605497599656,24.2307164190328,123.257597882604)) ;
#93244=CARTESIAN_POINT('Ctrl Pts',(-20.6138517566313,24.2407602768485,123.468583717357)) ;
#93245=CARTESIAN_POINT('Ctrl Pts',(-20.5864978803967,24.2505819674387,123.67324701416)) ;
#93246=CARTESIAN_POINT('Ctrl Pts',(-20.523154702789,24.2606170579791,123.874478638428)) ;
#93247=CARTESIAN_POINT('Ctrl Pts',(-20.4254304104399,24.2706415769618,124.061214670623)) ;
#93248=CARTESIAN_POINT('Ctrl Pts',(-20.2991788111832,24.280501422372,124.225596457457)) ;
#93249=CARTESIAN_POINT('Ctrl Pts',(-20.1451299023672,24.2904611986877,124.367416555609)) ;
#93250=CARTESIAN_POINT('Ctrl Pts',(-19.967433449482,24.3004893960023,124.48086059044)) ;
#93251=CARTESIAN_POINT('Ctrl Pts',(-19.7751577866426,24.3103969382926,124.560990104297)) ;
#93252=CARTESIAN_POINT('Ctrl Pts',(-19.5693703408195,24.3204295888565,124.607155031469)) ;
#93253=CARTESIAN_POINT('Ctrl Pts',(-19.3617967608512,24.3303135452832,124.616805532041)) ;
#93254=CARTESIAN_POINT('Ctrl Pts',(-19.1534319572427,24.340303246645,124.590503035312)) ;
#93255=CARTESIAN_POINT('Ctrl Pts',(-18.9519051680494,24.350344241921,124.527673626041)) ;
#93256=CARTESIAN_POINT('Ctrl Pts',(-18.7680835678611,24.3601771311894,124.433119432297)) ;
#93257=CARTESIAN_POINT('Ctrl Pts',(-18.6004240971246,24.3701702895568,124.30652665652)) ;
#93258=CARTESIAN_POINT('Ctrl Pts',(-18.4570479671225,24.3802023319089,124.151838394843)) ;
#93259=CARTESIAN_POINT('Ctrl Pts',(-18.3444058748891,24.3900675758674,123.977707913837)) ;
#93260=CARTESIAN_POINT('Ctrl Pts',(-18.2623662487685,24.4000294671134,123.785008650239)) ;
#93261=CARTESIAN_POINT('Ctrl Pts',(-18.2150227216315,24.4100643671318,123.579434985754)) ;
#93262=CARTESIAN_POINT('Ctrl Pts',(-18.2039108267018,24.4199494475464,123.371890116164)) ;
#93263=CARTESIAN_POINT('Ctrl Pts',(-18.2294765751654,24.4300146196713,123.161866621655)) ;
#93264=CARTESIAN_POINT('Ctrl Pts',(-18.2896850181631,24.4398618543947,122.963774150421)) ;
#93265=CARTESIAN_POINT('Ctrl Pts',(-18.3846631867251,24.4498926657125,122.775510294794)) ;
#93266=CARTESIAN_POINT('Ctrl Pts',(-18.5109890562497,24.459902281626,122.607182353693)) ;
#93267=CARTESIAN_POINT('Ctrl Pts',(-18.662934415357,24.4698130610297,122.464645988719)) ;
#93268=CARTESIAN_POINT('Ctrl Pts',(-18.8373840590184,24.4797423268187,122.349990522936)) ;
#93269=CARTESIAN_POINT('Ctrl Pts',(-19.0313351993538,24.4897850201314,122.266594737188)) ;
#93270=CARTESIAN_POINT('Ctrl Pts',(-19.2336139949417,24.4996715528261,122.218758536611)) ;
#93271=CARTESIAN_POINT('Ctrl Pts',(-19.4433196957446,24.5096646979294,122.206287817069)) ;
#93272=CARTESIAN_POINT('Ctrl Pts',(-19.651016738765,24.5196103786034,122.230384482874)) ;
#93273=CARTESIAN_POINT('Ctrl Pts',(-19.8515383300851,24.5295576362302,122.289780446404)) ;
#93274=CARTESIAN_POINT('Ctrl Pts',(-20.0404730317858,24.5396055383516,122.384240055457)) ;
#93275=CARTESIAN_POINT('Ctrl Pts',(-20.2068658200132,24.5494532439733,122.507427686497)) ;
#93276=CARTESIAN_POINT('Ctrl Pts',(-20.3514609588066,24.5594147106074,122.658908405433)) ;
#93277=CARTESIAN_POINT('Ctrl Pts',(-20.4681229484062,24.5694442638756,122.834556332122)) ;
#93278=CARTESIAN_POINT('Ctrl Pts',(-20.5515899993242,24.579351155903,123.025376842839)) ;
#93279=CARTESIAN_POINT('Ctrl Pts',(-20.6012474646981,24.5892988000161,123.228509354833)) ;
#93280=CARTESIAN_POINT('Ctrl Pts',(-20.6150856716365,24.5992988430449,123.438313400664)) ;
#93281=CARTESIAN_POINT('Ctrl Pts',(-20.5918280654159,24.6093376090389,123.648058203408)) ;
#93282=CARTESIAN_POINT('Ctrl Pts',(-20.5341801356447,24.6191626710612,123.846419055393)) ;
#93283=CARTESIAN_POINT('Ctrl Pts',(-20.4411613876781,24.6292172183875,124.036215827864)) ;
#93284=CARTESIAN_POINT('Ctrl Pts',(-20.3176758980808,24.6391604618367,124.204890744429)) ;
#93285=CARTESIAN_POINT('Ctrl Pts',(-20.1678533644699,24.6490626334446,124.349428636448)) ;
#93286=CARTESIAN_POINT('Ctrl Pts',(-19.992519974302,24.6591154690548,124.467412207897)) ;
#93287=CARTESIAN_POINT('Ctrl Pts',(-19.8028366254906,24.6689885267404,124.551709340961)) ;
#93288=CARTESIAN_POINT('Ctrl Pts',(-19.5990412262366,24.678983788266,124.602912203678)) ;
#93289=CARTESIAN_POINT('Ctrl Pts',(-19.3887859392486,24.6890091576865,124.617620934042)) ;
#93290=CARTESIAN_POINT('Ctrl Pts',(-19.1819726876381,24.6988989902131,124.596169219307)) ;
#93291=CARTESIAN_POINT('Ctrl Pts',(-18.9130614669707,24.7121969610225,124.519808891188)) ;
#93292=CARTESIAN_POINT('Ctrl Pts',(-18.6717642855586,24.7253953561317,124.376402129123)) ;
#93293=CARTESIAN_POINT('Ctrl Pts',(-18.4752738471407,24.7387907984112,124.174746595898)) ;
#93294=CARTESIAN_POINT('Ctrl Pts',(-18.358224596792,24.7486666366501,124.003215096803)) ;
#93295=CARTESIAN_POINT('Ctrl Pts',(-18.2710748545679,24.7587280392479,123.810519368002)) ;
#93296=CARTESIAN_POINT('Ctrl Pts',(-18.2196533486992,24.768593096183,123.609567259137)) ;
#93297=CARTESIAN_POINT('Ctrl Pts',(-18.2032987696929,24.7786051921318,123.399749506451)) ;
#93298=CARTESIAN_POINT('Ctrl Pts',(-18.2303147037854,24.7918825012772,123.121871295648)) ;
#93299=CARTESIAN_POINT('Ctrl Pts',(-18.3537922199677,24.8084815267845,122.791296707492)) ;
#93300=CARTESIAN_POINT('Ctrl Pts',(-18.5827030725049,24.8250805748176,122.522606050233)) ;
#93301=CARTESIAN_POINT('Ctrl Pts',(-18.8116927441516,24.8383239868485,122.36428598268)) ;
#93302=CARTESIAN_POINT('Ctrl Pts',(-19.0034240176672,24.8483614145369,122.276149956217)) ;
#93303=CARTESIAN_POINT('Ctrl Pts',(-19.2048453140622,24.8582657164925,122.223388070652)) ;
#93304=CARTESIAN_POINT('Ctrl Pts',(-19.4827946985258,24.8715325564677,122.199905670602)) ;
#93305=CARTESIAN_POINT('Ctrl Pts',(-19.8307376184793,24.8881587545576,122.262279593846)) ;
#93306=CARTESIAN_POINT('Ctrl Pts',(-20.1971584959203,24.9080778699411,122.474694806873)) ;
#93307=CARTESIAN_POINT('Ctrl Pts',(-20.4241107575517,24.9246842930753,122.745253284733)) ;
#93308=CARTESIAN_POINT('Ctrl Pts',(-20.5421825626076,24.937980513571,122.998571458746)) ;
#93309=CARTESIAN_POINT('Ctrl Pts',(-20.6149656124445,24.9512493459124,123.267944637777)) ;
#93310=CARTESIAN_POINT('Ctrl Pts',(-20.6152703456339,24.9679405939455,123.622747521554)) ;
#93311=CARTESIAN_POINT('Ctrl Pts',(-20.4723050323629,24.9877503256183,124.019012698152)) ;
#93312=CARTESIAN_POINT('Ctrl Pts',(-20.2011037571206,25.0077279329469,124.345923766588)) ;
#93313=CARTESIAN_POINT('Ctrl Pts',(-19.8352018509868,25.0276542420047,124.559424873862)) ;
#93314=CARTESIAN_POINT('Ctrl Pts',(-19.4208025231487,25.0474711021694,124.636316301746)) ;
#93315=CARTESIAN_POINT('Ctrl Pts',(-18.9994693482614,25.0675709177634,124.565580439574)) ;
#93316=CARTESIAN_POINT('Ctrl Pts',(-18.6335309066038,25.087327881646,124.358919176826)) ;
#93317=CARTESIAN_POINT('Ctrl Pts',(-18.3557823456024,25.1073648077154,124.036055559741)) ;
#93318=CARTESIAN_POINT('Ctrl Pts',(-18.2066757173654,25.127234390097,123.640645069707)) ;
#93319=CARTESIAN_POINT('Ctrl Pts',(-18.2003787407319,25.1471389618501,123.217548707811)) ;
#93320=CARTESIAN_POINT('Ctrl Pts',(-18.3392640527357,25.1670915640486,122.816604006415)) ;
#93321=CARTESIAN_POINT('Ctrl Pts',(-18.606064346536,25.1870010550189,122.488044036896)) ;
#93322=CARTESIAN_POINT('Ctrl Pts',(-18.9674597842372,25.2068524237183,122.269771232825)) ;
#93323=CARTESIAN_POINT('Ctrl Pts',(-19.3863525061292,25.2269326198543,122.187636259562)) ;
#93324=CARTESIAN_POINT('Ctrl Pts',(-19.8024619383338,25.2467335634297,122.252489157475)) ;
#93325=CARTESIAN_POINT('Ctrl Pts',(-20.1751760750366,25.2667175399392,122.456396705223)) ;
#93326=CARTESIAN_POINT('Ctrl Pts',(-20.4545282748226,25.2866335029148,122.774650929317)) ;
#93327=CARTESIAN_POINT('Ctrl Pts',(-20.6092751092114,25.3065039377368,123.167880061189)) ;
#93328=CARTESIAN_POINT('Ctrl Pts',(-20.6199281147208,25.3265542229698,123.593946344125)) ;
#93329=CARTESIAN_POINT('Ctrl Pts',(-20.4868920076711,25.3463281917291,123.992971200165)) ;
#93330=CARTESIAN_POINT('Ctrl Pts',(-20.2223887661916,25.3663846498487,124.327269621061)) ;
#93331=CARTESIAN_POINT('Ctrl Pts',(-19.8640906712415,25.3861795328397,124.548347828565)) ;
#93332=CARTESIAN_POINT('Ctrl Pts',(-19.4487333833075,25.406146188142,124.635759283439)) ;
#93333=CARTESIAN_POINT('Ctrl Pts',(-19.0285707159707,25.4261051582185,124.575488744381)) ;
#93334=CARTESIAN_POINT('Ctrl Pts',(-18.6553223916141,25.4460012458087,124.376405999239)) ;
#93335=CARTESIAN_POINT('Ctrl Pts',(-18.372020461912,25.4658994157202,124.062217905803)) ;
#93336=CARTESIAN_POINT('Ctrl Pts',(-18.2124360175169,25.4858052510873,123.670170425234)) ;
#93337=CARTESIAN_POINT('Ctrl Pts',(-18.196193662723,25.5057551760253,123.246330053742)) ;
#93338=CARTESIAN_POINT('Ctrl Pts',(-18.3247479722757,25.5256343659356,122.843621213655)) ;
#93339=CARTESIAN_POINT('Ctrl Pts',(-18.5841090164375,25.5456156902162,122.507162512338)) ;
#93340=CARTESIAN_POINT('Ctrl Pts',(-18.9420163018406,25.5655454744246,122.280112521784)) ;
#93341=CARTESIAN_POINT('Ctrl Pts',(-19.3555125525114,25.5854654638154,122.188825953791)) ;
#93342=CARTESIAN_POINT('Ctrl Pts',(-19.7742961587421,25.6053206591694,122.243020656991)) ;
#93343=CARTESIAN_POINT('Ctrl Pts',(-20.1526865947328,25.6253666608287,122.43900938881)) ;
#93344=CARTESIAN_POINT('Ctrl Pts',(-20.3906126005556,25.6418664080385,122.696940295105)) ;
#93345=CARTESIAN_POINT('Ctrl Pts',(-20.5216824764747,25.6552550124866,122.946016251658)) ;
#93346=CARTESIAN_POINT('Ctrl Pts',(-20.5849012167548,25.6651168408215,123.143472150751)) ;
#93347=CARTESIAN_POINT('Ctrl Pts',(-20.6138255672022,25.6750829835791,123.351002241802)) ;
#93348=CARTESIAN_POINT('Ctrl Pts',(-20.6032059149139,25.688444729704,123.631608389714)) ;
#93349=CARTESIAN_POINT('Ctrl Pts',(-20.5008843479732,25.7048990586591,123.966371588591)) ;
#93350=CARTESIAN_POINT('Ctrl Pts',(-20.2867255675478,25.7216663037074,124.25115815757)) ;
#93351=CARTESIAN_POINT('Ctrl Pts',(-20.0681057515217,25.7348528689815,124.421840372913)) ;
#93352=CARTESIAN_POINT('Ctrl Pts',(-19.8829958093437,25.7448423277261,124.520903011801)) ;
#93353=CARTESIAN_POINT('Ctrl Pts',(-19.6841239651198,25.7547961002072,124.586158616998)) ;
#93354=CARTESIAN_POINT('Ctrl Pts',(-19.4750312685853,25.7648439167398,124.615997659692)) ;
#93355=CARTESIAN_POINT('Ctrl Pts',(-19.2682136272315,25.7746854498623,124.609461719131)) ;
#93356=CARTESIAN_POINT('Ctrl Pts',(-19.0626573534037,25.784671692082,124.566942362516)) ;
#93357=CARTESIAN_POINT('Ctrl Pts',(-18.8684723007839,25.7946083155069,124.489834630106)) ;
#93358=CARTESIAN_POINT('Ctrl Pts',(-18.6887022668486,25.8046581928899,124.378870939841)) ;
#93359=CARTESIAN_POINT('Ctrl Pts',(-18.5339300730627,25.8145086316675,124.241258946451)) ;
#93360=CARTESIAN_POINT('Ctrl Pts',(-18.4034137139114,25.8244806456362,124.077232539093)) ;
#93361=CARTESIAN_POINT('Ctrl Pts',(-18.3031245285065,25.8344758142623,123.892541794129)) ;
#93362=CARTESIAN_POINT('Ctrl Pts',(-18.2364238705708,25.8445096975235,123.692438326714)) ;
#93363=CARTESIAN_POINT('Ctrl Pts',(-18.205714018985,25.8543655675869,123.487510321506)) ;
#93364=CARTESIAN_POINT('Ctrl Pts',(-18.2107938731432,25.864363113504,123.277414588518)) ;
#93365=CARTESIAN_POINT('Ctrl Pts',(-18.2518456767253,25.8742712404033,123.073191361483)) ;
#93366=CARTESIAN_POINT('Ctrl Pts',(-18.3281771028742,25.8842816119255,122.877061463729)) ;
#93367=CARTESIAN_POINT('Ctrl Pts',(-18.4380159492977,25.8943120546729,122.697063911336)) ;
#93368=CARTESIAN_POINT('Ctrl Pts',(-18.5745552119274,25.9041600072262,122.5414142025)) ;
#93369=CARTESIAN_POINT('Ctrl Pts',(-18.7394363200053,25.9142226762471,122.408905143924)) ;
#93370=CARTESIAN_POINT('Ctrl Pts',(-18.9218264083034,25.9241170517111,122.308852272964)) ;
#93371=CARTESIAN_POINT('Ctrl Pts',(-19.1195394323681,25.9340588500292,122.241151655408)) ;
#93372=CARTESIAN_POINT('Ctrl Pts',(-19.3273054241059,25.9440613437565,122.208523083542)) ;
#93373=CARTESIAN_POINT('Ctrl Pts',(-19.5382116668081,25.9540961422634,122.212809762193)) ;
#93374=CARTESIAN_POINT('Ctrl Pts',(-19.7413463382716,25.9639410262428,122.252542610422)) ;
#93375=CARTESIAN_POINT('Ctrl Pts',(-19.9373601162425,25.9739268830608,122.327621634574)) ;
#93376=CARTESIAN_POINT('Ctrl Pts',(-20.1165785383608,25.9838616972356,122.434952368301)) ;
#93377=CARTESIAN_POINT('Ctrl Pts',(-20.2762122449541,25.9939191970209,122.573557383154)) ;
#93378=CARTESIAN_POINT('Ctrl Pts',(-20.4065114706152,26.0037409554392,122.733766868605)) ;
#93379=CARTESIAN_POINT('Ctrl Pts',(-20.5097347090899,26.0137966132232,122.918234290482)) ;
#93380=CARTESIAN_POINT('Ctrl Pts',(-20.5782258756147,26.0237387954033,123.115721371548)) ;
#93381=CARTESIAN_POINT('Ctrl Pts',(-20.6118871272014,26.033644004098,123.321218153653)) ;
#93382=CARTESIAN_POINT('Ctrl Pts',(-20.6092537917906,26.0436857950604,123.532308255911)) ;
#93383=CARTESIAN_POINT('Ctrl Pts',(-20.5705521089808,26.0535935695326,123.73698203017)) ;
#93384=CARTESIAN_POINT('Ctrl Pts',(-20.4964939731295,26.0636050697602,123.934001627949)) ;
#93385=CARTESIAN_POINT('Ctrl Pts',(-20.3887491022585,26.0736378301529,124.115324540153)) ;
#93386=CARTESIAN_POINT('Ctrl Pts',(-20.2539283372818,26.0834883992878,124.272523599289)) ;
#93387=CARTESIAN_POINT('Ctrl Pts',(-20.0918867933303,26.0934770088177,124.406059622827)) ;
#93388=CARTESIAN_POINT('Ctrl Pts',(-19.9101964338395,26.1034056648418,124.508820927901)) ;
#93389=CARTESIAN_POINT('Ctrl Pts',(-19.7123664598678,26.1133934110196,124.579225538772)) ;
#93390=CARTESIAN_POINT('Ctrl Pts',(-19.5042772685736,26.1234293999554,124.614026056989)) ;
#93391=CARTESIAN_POINT('Ctrl Pts',(-19.2970856456385,26.133284269769,124.612543958889)) ;
#93392=CARTESIAN_POINT('Ctrl Pts',(-19.0903087822269,26.1432837110107,124.574850516544)) ;
#93393=CARTESIAN_POINT('Ctrl Pts',(-18.8951319256074,26.1531787851908,124.502774169454)) ;
#93394=CARTESIAN_POINT('Ctrl Pts',(-18.712492759328,26.1632394410305,124.396160191167)) ;
#93395=CARTESIAN_POINT('Ctrl Pts',(-18.5544270484986,26.1730883152261,124.262395161111)) ;
#93396=CARTESIAN_POINT('Ctrl Pts',(-18.4191734859892,26.1831170271894,124.100664930615)) ;
#93397=CARTESIAN_POINT('Ctrl Pts',(-18.3145428694467,26.1931464277725,123.917602948853)) ;
#93398=CARTESIAN_POINT('Ctrl Pts',(-18.2441983081728,26.2029866213893,123.723055479142)) ;
#93399=CARTESIAN_POINT('Ctrl Pts',(-18.2077335916709,26.2129900439645,123.515958829332)) ;
#93400=CARTESIAN_POINT('Ctrl Pts',(-18.207849919895,26.2229755810576,123.305996114384)) ;
#93401=CARTESIAN_POINT('Ctrl Pts',(-18.2448224450821,26.2330165855444,123.098185958019)) ;
#93402=CARTESIAN_POINT('Ctrl Pts',(-18.315637546413,26.2428601244856,122.903720935698)) ;
#93403=CARTESIAN_POINT('Ctrl Pts',(-18.4202262131104,26.2528451554764,122.721750406657)) ;
#93404=CARTESIAN_POINT('Ctrl Pts',(-18.5541826302326,26.2627846179984,122.561338916307)) ;
#93405=CARTESIAN_POINT('Ctrl Pts',(-18.7155638139311,26.2728243502222,122.425330541335)) ;
#93406=CARTESIAN_POINT('Ctrl Pts',(-18.8953261424376,26.2827125305394,122.320904799776)) ;
#93407=CARTESIAN_POINT('Ctrl Pts',(-19.0923360066842,26.2927020462419,122.248179871716)) ;
#93408=CARTESIAN_POINT('Ctrl Pts',(-19.29836965637,26.3026605968966,122.211042573258)) ;
#93409=CARTESIAN_POINT('Ctrl Pts',(-19.506496121546,26.3125600040016,122.20972967354)) ;
#93410=CARTESIAN_POINT('Ctrl Pts',(-19.7147275262977,26.3226085904179,122.245179238404)) ;
#93411=CARTESIAN_POINT('Ctrl Pts',(-19.9106882308818,26.3325014093824,122.314976928487)) ;
#93412=CARTESIAN_POINT('Ctrl Pts',(-20.0947008159812,26.3425725269122,122.419616587146)) ;
#93413=CARTESIAN_POINT('Ctrl Pts',(-20.2538532201277,26.3523882208783,122.551030461718)) ;
#93414=CARTESIAN_POINT('Ctrl Pts',(-20.3913677815839,26.3624545983756,122.711830813516)) ;
#93415=CARTESIAN_POINT('Ctrl Pts',(-20.497080515863,26.3723535844574,122.891149584899)) ;
#93416=CARTESIAN_POINT('Ctrl Pts',(-20.5712377326743,26.3824077644509,123.089035325503)) ;
#93417=CARTESIAN_POINT('Ctrl Pts',(-20.6094217264944,26.3922785773836,123.293057111888)) ;
#93418=CARTESIAN_POINT('Ctrl Pts',(-20.6116385942479,26.4023524782374,123.504781098235)) ;
#93419=CARTESIAN_POINT('Ctrl Pts',(-20.5781656742403,26.4121726336241,123.708548551579)) ;
#93420=CARTESIAN_POINT('Ctrl Pts',(-20.5082435413236,26.4222513405763,123.908510156717)) ;
#93421=CARTESIAN_POINT('Ctrl Pts',(-20.4070109794574,26.4321029291151,124.089251298327)) ;
#93422=CARTESIAN_POINT('Ctrl Pts',(-20.2731855957276,26.4421760456401,124.253326756013)) ;
#93423=CARTESIAN_POINT('Ctrl Pts',(-20.1165101320345,26.4520185627359,124.388517157775)) ;
#93424=CARTESIAN_POINT('Ctrl Pts',(-19.9366357026689,26.4619990242899,124.49652523591)) ;
#93425=CARTESIAN_POINT('Ctrl Pts',(-19.7398462849515,26.4720172742807,124.571568687572)) ;
#93426=CARTESIAN_POINT('Ctrl Pts',(-19.5358433540864,26.4819014344744,124.611196186289)) ;
#93427=CARTESIAN_POINT('Ctrl Pts',(-19.3242969728162,26.4919665814494,124.614819305316)) ;
#93428=CARTESIAN_POINT('Ctrl Pts',(-19.1199162896328,26.5018084050902,124.582500426852)) ;
#93429=CARTESIAN_POINT('Ctrl Pts',(-18.9203549014018,26.5118378775511,124.51444423306)) ;
#93430=CARTESIAN_POINT('Ctrl Pts',(-18.7359669975799,26.5218647328131,124.412277185117)) ;
#93431=CARTESIAN_POINT('Ctrl Pts',(-18.5748099226721,26.5317079829236,124.282461831563)) ;
#93432=CARTESIAN_POINT('Ctrl Pts',(-18.4355916456644,26.5417564225068,124.123583572549)) ;
#93433=CARTESIAN_POINT('Ctrl Pts',(-18.3274329386578,26.5517059167547,123.944547268293)) ;
#93434=CARTESIAN_POINT('Ctrl Pts',(-18.2517329103904,26.5616137724807,123.750483520398)) ;
#93435=CARTESIAN_POINT('Ctrl Pts',(-18.2104800380329,26.5716732491306,123.543086602686)) ;
#93436=CARTESIAN_POINT('Ctrl Pts',(-18.2056838550714,26.5815140585393,123.336232067944)) ;
#93437=CARTESIAN_POINT('Ctrl Pts',(-18.2373097240745,26.5915762088401,123.127093681525)) ;
#93438=CARTESIAN_POINT('Ctrl Pts',(-18.3038768776856,26.6014733699627,122.929948794933)) ;
#93439=CARTESIAN_POINT('Ctrl Pts',(-18.4033896561337,26.6114045443667,122.746410755063)) ;
#93440=CARTESIAN_POINT('Ctrl Pts',(-18.5348932882933,26.6214467480918,122.581254053194)) ;
#93441=CARTESIAN_POINT('Ctrl Pts',(-18.6905332621863,26.6313333305222,122.443483756373)) ;
#93442=CARTESIAN_POINT('Ctrl Pts',(-18.8694457020264,26.6413267662705,122.333371781551)) ;
#93443=CARTESIAN_POINT('Ctrl Pts',(-19.0638389458024,26.6512712346287,122.25643179021)) ;
#93444=CARTESIAN_POINT('Ctrl Pts',(-19.2687173484361,26.6612230508743,122.213994242932)) ;
#93445=CARTESIAN_POINT('Ctrl Pts',(-19.4796376314532,26.6712604869887,122.207914894634)) ;
#93446=CARTESIAN_POINT('Ctrl Pts',(-19.6852953687343,26.6811454461651,122.237889874322)) ;
#93447=CARTESIAN_POINT('Ctrl Pts',(-19.8849208385928,26.691143564377,122.303615139944)) ;
#93448=CARTESIAN_POINT('Ctrl Pts',(-20.0687823899887,26.701064496889,122.40213114507)) ;
#93449=CARTESIAN_POINT('Ctrl Pts',(-20.2347433719469,26.7111057971111,122.532576201675)) ;
#93450=CARTESIAN_POINT('Ctrl Pts',(-20.3736041235756,26.721012715501,122.687807479836)) ;
#93451=CARTESIAN_POINT('Ctrl Pts',(-20.4842302721718,26.7309485072101,122.864990307838)) ;
#93452=CARTESIAN_POINT('Ctrl Pts',(-20.5630380467698,26.740989401788,123.060813841052)) ;
#93453=CARTESIAN_POINT('Ctrl Pts',(-20.606131212989,26.7508766035018,123.264168783375)) ;
#93454=CARTESIAN_POINT('Ctrl Pts',(-20.6136841228083,26.7608688712634,123.474087428869)) ;
#93455=CARTESIAN_POINT('Ctrl Pts',(-20.5847396526001,26.7708173922852,123.681235914656)) ;
#93456=CARTESIAN_POINT('Ctrl Pts',(-20.5206329141074,26.7807541658629,123.880040207961)) ;
#93457=CARTESIAN_POINT('Ctrl Pts',(-20.4227399059421,26.790737214004,124.065715809931)) ;
#93458=CARTESIAN_POINT('Ctrl Pts',(-20.2930387524076,26.800780921614,124.232307345616)) ;
#93459=CARTESIAN_POINT('Ctrl Pts',(-20.1400189052404,26.8106096147673,124.371201732946)) ;
#93460=CARTESIAN_POINT('Ctrl Pts',(-19.9609582162376,26.8206843638968,124.484270411322)) ;
#93461=CARTESIAN_POINT('Ctrl Pts',(-19.7689924318858,26.8305496896923,124.562839075184)) ;
#93462=CARTESIAN_POINT('Ctrl Pts',(-19.5632221684136,26.8405718640493,124.608103780006)) ;
#93463=CARTESIAN_POINT('Ctrl Pts',(-19.3525933509381,26.8505979172562,124.616438892034)) ;
#93464=CARTESIAN_POINT('Ctrl Pts',(-19.1472930179978,26.8604516141025,124.588899906443)) ;
#93465=CARTESIAN_POINT('Ctrl Pts',(-18.9475623242253,26.8704110188554,124.526053167389)) ;
#93466=CARTESIAN_POINT('Ctrl Pts',(-18.7604973127127,26.8804492645603,124.428392120626)) ;
#93467=CARTESIAN_POINT('Ctrl Pts',(-18.595707038093,26.8903234487224,124.302108746629)) ;
#93468=CARTESIAN_POINT('Ctrl Pts',(-18.4526112031336,26.9003932318603,124.146135573112)) ;
#93469=CARTESIAN_POINT('Ctrl Pts',(-18.3413269230795,26.910226486881,123.971898783901)) ;
#93470=CARTESIAN_POINT('Ctrl Pts',(-18.2598539373914,26.9202569130127,123.777409910827)) ;
#93471=CARTESIAN_POINT('Ctrl Pts',(-18.2139770922715,26.9302885251997,123.571552183316)) ;
#93472=CARTESIAN_POINT('Ctrl Pts',(-18.2043014628448,26.9401182220543,123.365141874546)) ;
#93473=CARTESIAN_POINT('Ctrl Pts',(-18.2304203523033,26.9501076639568,123.156756810279)) ;
#93474=CARTESIAN_POINT('Ctrl Pts',(-18.2931717636035,26.9601515559725,122.955144115483)) ;
#93475=CARTESIAN_POINT('Ctrl Pts',(-18.3874551637717,26.9699731177417,122.771448988579)) ;
#93476=CARTESIAN_POINT('Ctrl Pts',(-18.5145023549983,26.9800086893659,122.603007690826)) ;
#93477=CARTESIAN_POINT('Ctrl Pts',(-18.6691989364535,26.9900379636477,122.459740110803)) ;
#93478=CARTESIAN_POINT('Ctrl Pts',(-18.8426716613453,26.9998718007664,122.347266613141)) ;
#93479=CARTESIAN_POINT('Ctrl Pts',(-19.0371543491445,27.0099241968545,122.26460097273)) ;
#93480=CARTESIAN_POINT('Ctrl Pts',(-19.2407489171137,27.0198609638051,122.217766396637)) ;
#93481=CARTESIAN_POINT('Ctrl Pts',(-19.4492892613563,27.0297951987843,122.206457880832)) ;
#93482=CARTESIAN_POINT('Ctrl Pts',(-19.6584787688609,27.0398189621111,122.231885051993)) ;
#93483=CARTESIAN_POINT('Ctrl Pts',(-19.8573566469168,27.0497053034958,122.292260658762)) ;
#93484=CARTESIAN_POINT('Ctrl Pts',(-20.044884241241,27.0596943522627,122.386795146687)) ;
#93485=CARTESIAN_POINT('Ctrl Pts',(-20.2137587515915,27.0697355729601,122.513457842224)) ;
#93486=CARTESIAN_POINT('Ctrl Pts',(-20.3553226201596,27.079568213138,122.664084460365)) ;
#93487=CARTESIAN_POINT('Ctrl Pts',(-20.4709452079467,27.089562142446,122.839511283669)) ;
#93488=CARTESIAN_POINT('Ctrl Pts',(-20.5542369537336,27.0995913501265,123.033209534524)) ;
#93489=CARTESIAN_POINT('Ctrl Pts',(-20.6022223085313,27.1094671618306,123.235220662591)) ;
#93490=CARTESIAN_POINT('Ctrl Pts',(-20.6147833778332,27.119466388802,123.445032111531)) ;
#93491=CARTESIAN_POINT('Ctrl Pts',(-20.5911307340941,27.1293758699577,123.652044212278)) ;
#93492=CARTESIAN_POINT('Ctrl Pts',(-20.5310228623009,27.1394291002586,123.85464405997)) ;
#93493=CARTESIAN_POINT('Ctrl Pts',(-20.4384382021735,27.1492997168097,124.040371924575)) ;
#93494=CARTESIAN_POINT('Ctrl Pts',(-20.3135085808993,27.1593213785417,124.210019681239)) ;
#93495=CARTESIAN_POINT('Ctrl Pts',(-20.1606599163486,27.1693441917228,124.355074884069)) ;
#93496=CARTESIAN_POINT('Ctrl Pts',(-19.9878844325135,27.1792113561828,124.469859477735)) ;
#93497=CARTESIAN_POINT('Ctrl Pts',(-19.7955493981892,27.1892047984027,124.554411463994)) ;
#93498=CARTESIAN_POINT('Ctrl Pts',(-19.5905834003514,27.199236472003,124.604073131123)) ;
#93499=CARTESIAN_POINT('Ctrl Pts',(-19.3835855502156,27.209102907116,124.617490989983)) ;
#93500=CARTESIAN_POINT('Ctrl Pts',(-19.174870121098,27.2190903576491,124.594828115843)) ;
#93501=CARTESIAN_POINT('Ctrl Pts',(-18.9740333028024,27.2290352874771,124.536610653904)) ;
#93502=CARTESIAN_POINT('Ctrl Pts',(-18.7845669174795,27.2390801825322,124.443394505868)) ;
#93503=CARTESIAN_POINT('Ctrl Pts',(-18.6171298557573,27.248942244218,124.321093509513)) ;
#93504=CARTESIAN_POINT('Ctrl Pts',(-18.4713020979858,27.2589339670049,124.16992654863)) ;
#93505=CARTESIAN_POINT('Ctrl Pts',(-18.3546885531147,27.2688661812449,123.996714378362)) ;
#93506=CARTESIAN_POINT('Ctrl Pts',(-18.269419645282,27.2788054998106,123.805941861315)) ;
#93507=CARTESIAN_POINT('Ctrl Pts',(-18.2182240150851,27.2888496745865,123.601084899487)) ;
#93508=CARTESIAN_POINT('Ctrl Pts',(-18.2035200670347,27.2987202286514,123.394096871546)) ;
#93509=CARTESIAN_POINT('Ctrl Pts',(-18.2245812279825,27.3086852110056,123.185662484473)) ;
#93510=CARTESIAN_POINT('Ctrl Pts',(-18.2821983669197,27.3187159138954,122.982815593457)) ;
#93511=CARTESIAN_POINT('Ctrl Pts',(-18.3726338901219,27.3286082539206,122.795512181265)) ;
#93512=CARTESIAN_POINT('Ctrl Pts',(-18.4961446714917,27.3386614870806,122.624043166509)) ;
#93513=CARTESIAN_POINT('Ctrl Pts',(-18.6449201037129,27.3485427315573,122.479010000241)) ;
#93514=CARTESIAN_POINT('Ctrl Pts',(-18.8191075332246,27.3585758524284,122.360127390189)) ;
#93515=CARTESIAN_POINT('Ctrl Pts',(-19.0083749934577,27.3684570627034,122.274409088522)) ;
#93516=CARTESIAN_POINT('Ctrl Pts',(-19.2132499375298,27.3785191384728,122.221874637997)) ;
#93517=CARTESIAN_POINT('Ctrl Pts',(-19.4198941729344,27.3883761968545,122.205962714109)) ;
#93518=CARTESIAN_POINT('Ctrl Pts',(-19.6290171503523,27.3983707521435,122.226026766799)) ;
#93519=CARTESIAN_POINT('Ctrl Pts',(-19.8301684040698,27.408296639679,122.281656756404)) ;
#93520=CARTESIAN_POINT('Ctrl Pts',(-20.0204729359765,27.4183216596743,122.372190073882)) ;
#93521=CARTESIAN_POINT('Ctrl Pts',(-20.1900416051017,27.428219036778,122.492787717248)) ;
#93522=CARTESIAN_POINT('Ctrl Pts',(-20.337791395253,27.4382092738588,122.642064176377)) ;
#93523=CARTESIAN_POINT('Ctrl Pts',(-20.4575937675202,27.4482458866676,122.815752566344)) ;
#93524=CARTESIAN_POINT('Ctrl Pts',(-20.5440949710146,27.4580957700856,123.003904331342)) ;
#93525=CARTESIAN_POINT('Ctrl Pts',(-20.5978342575629,27.4680993869881,123.207208424136)) ;
#93526=CARTESIAN_POINT('Ctrl Pts',(-20.6153220020921,27.4780887987532,123.416522213151)) ;
#93527=CARTESIAN_POINT('Ctrl Pts',(-20.596019200136,27.4881075600981,123.626239460963)) ;
#93528=CARTESIAN_POINT('Ctrl Pts',(-20.5232688664798,27.5013262354791,123.894499714109)) ;
#93529=CARTESIAN_POINT('Ctrl Pts',(-20.3813539407397,27.5146365427238,124.139308036254)) ;
#93530=CARTESIAN_POINT('Ctrl Pts',(-20.1842224998878,27.5278742089498,124.33573047354)) ;
#93531=CARTESIAN_POINT('Ctrl Pts',(-20.0135550279124,27.5377939043605,124.45559248642)) ;
#93532=CARTESIAN_POINT('Ctrl Pts',(-19.8220507976566,27.5478467713591,124.544956171201)) ;
#93533=CARTESIAN_POINT('Ctrl Pts',(-19.6219766811352,27.5577021796884,124.598870302969)) ;
#93534=CARTESIAN_POINT('Ctrl Pts',(-19.4118114679212,27.5677408113649,124.617912525349)) ;
#93535=CARTESIAN_POINT('Ctrl Pts',(-19.1331437800941,27.581042993632,124.594057344109)) ;
#93536=CARTESIAN_POINT('Ctrl Pts',(-18.8021120088637,27.5975880067148,124.475053992695)) ;
#93537=CARTESIAN_POINT('Ctrl Pts',(-18.5297401940674,27.614240022791,124.2488161865)) ;
#93538=CARTESIAN_POINT('Ctrl Pts',(-18.3691043286755,27.6274631136963,124.021959188954)) ;
#93539=CARTESIAN_POINT('Ctrl Pts',(-18.279074765685,27.6374240732556,123.832881312923)) ;
#93540=CARTESIAN_POINT('Ctrl Pts',(-18.2231429882255,27.6474488700067,123.62969511615)) ;
#93541=CARTESIAN_POINT('Ctrl Pts',(-18.1966274879579,27.6606733174025,123.352901549836)) ;
#93542=CARTESIAN_POINT('Ctrl Pts',(-18.2547427228421,27.6773071021016,123.004090311411)) ;
#93543=CARTESIAN_POINT('Ctrl Pts',(-18.462654194708,27.6972097688266,122.635456439597)) ;
#93544=CARTESIAN_POINT('Ctrl Pts',(-18.7834264639891,27.7171099966084,122.359556189311)) ;
#93545=CARTESIAN_POINT('Ctrl Pts',(-19.1793576793878,27.7370274841399,122.209266164679)) ;
#93546=CARTESIAN_POINT('Ctrl Pts',(-19.6030851389282,27.7569570099568,122.20284220471)) ;
#93547=CARTESIAN_POINT('Ctrl Pts',(-20.0042034113001,27.7769192778431,122.341703290719)) ;
#93548=CARTESIAN_POINT('Ctrl Pts',(-20.3326268774774,27.7968094727953,122.608069909733)) ;
#93549=CARTESIAN_POINT('Ctrl Pts',(-20.5514322995273,27.8166997175416,122.970098508782)) ;
#93550=CARTESIAN_POINT('Ctrl Pts',(-20.6334273803088,27.836774090104,123.388925968865)) ;
#93551=CARTESIAN_POINT('Ctrl Pts',(-20.5686426007761,27.8565594674643,123.804655277717)) ;
#93552=CARTESIAN_POINT('Ctrl Pts',(-20.3652778235273,27.8765213415315,124.177163759721)) ;
#93553=CARTESIAN_POINT('Ctrl Pts',(-20.0460050432722,27.896501317022,124.45743847941)) ;
#93554=CARTESIAN_POINT('Ctrl Pts',(-19.6538578338986,27.9163137468999,124.61141438612)) ;
#93555=CARTESIAN_POINT('Ctrl Pts',(-19.229262390193,27.9362938549902,124.622968495663)) ;
#93556=CARTESIAN_POINT('Ctrl Pts',(-18.8278347516187,27.9561882385874,124.48928119194)) ;
#93557=CARTESIAN_POINT('Ctrl Pts',(-18.4954921617374,27.9761151665647,124.22662108976)) ;
#93558=CARTESIAN_POINT('Ctrl Pts',(-18.2725085713634,27.9960100238659,123.867030699903)) ;
#93559=CARTESIAN_POINT('Ctrl Pts',(-18.1854382342553,28.0160492174695,123.449977253235)) ;
#93560=CARTESIAN_POINT('Ctrl Pts',(-18.2454140966573,28.0358891853803,123.032366941405)) ;
#93561=CARTESIAN_POINT('Ctrl Pts',(-18.4440438223456,28.0558040023444,122.658441047315)) ;
#93562=CARTESIAN_POINT('Ctrl Pts',(-18.7589841925782,28.0757462477406,122.374568986743)) ;
#93563=CARTESIAN_POINT('Ctrl Pts',(-19.1503542322998,28.0956182958551,122.215058271776)) ;
#93564=CARTESIAN_POINT('Ctrl Pts',(-19.5753982482705,28.1156293608092,122.198881833983)) ;
#93565=CARTESIAN_POINT('Ctrl Pts',(-19.976924777418,28.1354408851129,122.326892971449)) ;
#93566=CARTESIAN_POINT('Ctrl Pts',(-20.3149986104091,28.1555360970762,122.587908851649)) ;
#93567=CARTESIAN_POINT('Ctrl Pts',(-20.540244932059,28.175316820996,122.943300131366)) ;
#93568=CARTESIAN_POINT('Ctrl Pts',(-20.632541211871,28.1953078966388,123.358060932043)) ;
#93569=CARTESIAN_POINT('Ctrl Pts',(-20.5777379932695,28.2151898356818,123.777357946779)) ;
#93570=CARTESIAN_POINT('Ctrl Pts',(-20.3829565043216,28.2351424401851,124.154169171674)) ;
#93571=CARTESIAN_POINT('Ctrl Pts',(-20.0720352876919,28.2550413089158,124.441191772874)) ;
#93572=CARTESIAN_POINT('Ctrl Pts',(-19.6822521549889,28.2749347087253,124.605274930316)) ;
#93573=CARTESIAN_POINT('Ctrl Pts',(-19.2594119704509,28.2948438395654,124.627173961872)) ;
#93574=CARTESIAN_POINT('Ctrl Pts',(-18.8522720945946,28.3148759393289,124.502181134798)) ;
#93575=CARTESIAN_POINT('Ctrl Pts',(-18.5715058354891,28.3314080124984,124.290597893153)) ;
#93576=CARTESIAN_POINT('Ctrl Pts',(-18.3986989765231,28.3447433531043,124.06986111569)) ;
#93577=CARTESIAN_POINT('Ctrl Pts',(-18.3010384376066,28.3545859116441,123.887414284966)) ;
#93578=CARTESIAN_POINT('Ctrl Pts',(-18.2349738070104,28.364637818494,123.686701670905)) ;
#93579=CARTESIAN_POINT('Ctrl Pts',(-18.1952065129706,28.3778863328849,123.411043207663)) ;
#93580=CARTESIAN_POINT('Ctrl Pts',(-18.2364119327605,28.3944855078326,123.060489114664)) ;
#93581=CARTESIAN_POINT('Ctrl Pts',(-18.3945320732476,28.4110742936277,122.745246270374)) ;
#93582=CARTESIAN_POINT('Ctrl Pts',(-18.5797843255288,28.4243501099696,122.536445693784)) ;
#93583=CARTESIAN_POINT('Ctrl Pts',(-18.7438859525293,28.4343239607634,122.4059105653)) ;
#93584=CARTESIAN_POINT('Ctrl Pts',(-18.9292775705451,28.4443529928558,122.305499193489)) ;
#93585=CARTESIAN_POINT('Ctrl Pts',(-19.1264647249251,28.4542431183577,122.239514286115)) ;
#93586=CARTESIAN_POINT('Ctrl Pts',(-19.3341633471274,28.4642355966292,122.208177516446)) ;
#93587=CARTESIAN_POINT('Ctrl Pts',(-19.5433409170049,28.4741868117266,122.213247363974)) ;
#93588=CARTESIAN_POINT('Ctrl Pts',(-19.7503773115582,28.4842353134817,122.255121671424)) ;
#93589=CARTESIAN_POINT('Ctrl Pts',(-19.9430718837078,28.4940766630984,122.330508480184)) ;
#93590=CARTESIAN_POINT('Ctrl Pts',(-20.1225389941562,28.5040629541187,122.439381413048)) ;
#93591=CARTESIAN_POINT('Ctrl Pts',(-20.2797114114342,28.5139995658473,122.577040974791)) ;
#93592=CARTESIAN_POINT('Ctrl Pts',(-20.4119681889468,28.5240494412148,122.74177821394)) ;
#93593=CARTESIAN_POINT('Ctrl Pts',(-20.5117487646178,28.5338998997503,122.923259406257)) ;
#93594=CARTESIAN_POINT('Ctrl Pts',(-20.5798319652677,28.543871836703,123.121510243996)) ;
#93595=CARTESIAN_POINT('Ctrl Pts',(-20.6125111709449,28.5538672936351,123.329122137551)) ;
#93596=CARTESIAN_POINT('Ctrl Pts',(-20.6083934035512,28.5639001006882,123.539989223304)) ;
#93597=CARTESIAN_POINT('Ctrl Pts',(-20.5686972957421,28.5737599872782,123.743449587553)) ;
#93598=CARTESIAN_POINT('Ctrl Pts',(-20.493679365146,28.5837490678434,123.939575708559)) ;
#93599=CARTESIAN_POINT('Ctrl Pts',(-20.3863550900639,28.5936805470526,124.118678024695)) ;
#93600=CARTESIAN_POINT('Ctrl Pts',(-20.2490702128718,28.6036664064985,124.277521451169)) ;
#93601=CARTESIAN_POINT('Ctrl Pts',(-20.0852249792083,28.6137045571457,124.410502596884)) ;
#93602=CARTESIAN_POINT('Ctrl Pts',(-19.9044472059089,28.6235526476501,124.51145879854)) ;
#93603=CARTESIAN_POINT('Ctrl Pts',(-19.7047579306307,28.6336135561681,124.581118064971)) ;
#93604=CARTESIAN_POINT('Ctrl Pts',(-19.4993889315201,28.6435084033261,124.614351432884)) ;
#93605=CARTESIAN_POINT('Ctrl Pts',(-19.290422284636,28.6534500753711,124.61196471871)) ;
#93606=CARTESIAN_POINT('Ctrl Pts',(-19.0837190965764,28.6634526024966,124.573165459585)) ;
#93607=CARTESIAN_POINT('Ctrl Pts',(-18.8864143900725,28.673487393684,124.498528915288)) ;
#93608=CARTESIAN_POINT('Ctrl Pts',(-18.7082976391662,28.6833322735432,124.393092627413)) ;
#93609=CARTESIAN_POINT('Ctrl Pts',(-18.5487226700083,28.6933181541616,124.256732099038)) ;
#93610=CARTESIAN_POINT('Ctrl Pts',(-18.41576941784,28.7032528772548,124.095604644476)) ;
#93611=CARTESIAN_POINT('Ctrl Pts',(-18.3117412138791,28.713310717566,123.911553889218)) ;
#93612=CARTESIAN_POINT('Ctrl Pts',(-18.2425809970135,28.7231312049625,123.716996800082)) ;
#93613=CARTESIAN_POINT('Ctrl Pts',(-18.207077110529,28.7331916063077,123.508522426706)) ;
#93614=CARTESIAN_POINT('Ctrl Pts',(-18.2085773478426,28.7431225718606,123.299723942256)) ;
#93615=CARTESIAN_POINT('Ctrl Pts',(-18.245873377285,28.753061434197,123.094155479306)) ;
#93616=CARTESIAN_POINT('Ctrl Pts',(-18.3185218475417,28.7630471651232,122.897169941774)) ;
#93617=CARTESIAN_POINT('Ctrl Pts',(-18.4248524147212,28.7730715505507,122.715235116159)) ;
#93618=CARTESIAN_POINT('Ctrl Pts',(-18.5592956161916,28.7829748349039,122.556229872053)) ;
#93619=CARTESIAN_POINT('Ctrl Pts',(-18.7218419116847,28.7930348394819,122.420962440775)) ;
#93620=CARTESIAN_POINT('Ctrl Pts',(-18.9014184995494,28.802878108551,122.31808641314)) ;
#93621=CARTESIAN_POINT('Ctrl Pts',(-19.098834322819,28.8128686741587,122.246460343991)) ;
#93622=CARTESIAN_POINT('Ctrl Pts',(-19.3044348672317,28.8227968059375,122.210453578129)) ;
#93623=CARTESIAN_POINT('Ctrl Pts',(-19.5144210408558,28.8327846930185,122.210327947691)) ;
#93624=CARTESIAN_POINT('Ctrl Pts',(-19.7221546515197,28.8428206425871,122.247189649512)) ;
#93625=CARTESIAN_POINT('Ctrl Pts',(-19.9168982030281,28.852675528966,122.317939833791)) ;
#93626=CARTESIAN_POINT('Ctrl Pts',(-20.099129252199,28.8626749433138,122.422673266323)) ;
#93627=CARTESIAN_POINT('Ctrl Pts',(-20.2589220409907,28.8725701085043,122.555925365975)) ;
#93628=CARTESIAN_POINT('Ctrl Pts',(-20.3953335885789,28.8826304271963,122.717517984113)) ;
#93629=CARTESIAN_POINT('Ctrl Pts',(-20.4995231303443,28.8924805589724,122.896499760927)) ;
#93630=CARTESIAN_POINT('Ctrl Pts',(-20.5728206210608,28.9025111294226,123.094215195434)) ;
#93631=CARTESIAN_POINT('Ctrl Pts',(-20.6101551335493,28.9125252800954,123.301419328339)) ;
#93632=CARTESIAN_POINT('Ctrl Pts',(-20.6112719043652,28.9224182136408,123.509400270056)) ;
#93633=CARTESIAN_POINT('Ctrl Pts',(-20.5761577703993,28.9324077276311,123.71643445623)) ;
#93634=CARTESIAN_POINT('Ctrl Pts',(-20.5059948079295,28.9423614982835,123.913612659648)) ;
#93635=CARTESIAN_POINT('Ctrl Pts',(-20.4015456859858,28.9524092669441,124.097194214206)) ;
#93636=CARTESIAN_POINT('Ctrl Pts',(-20.2697350876435,28.9622509933839,124.256700935986)) ;
#93637=CARTESIAN_POINT('Ctrl Pts',(-20.1102649496919,28.9722365102067,124.393174748905)) ;
#93638=CARTESIAN_POINT('Ctrl Pts',(-19.9303421294312,28.9821758419022,124.499490582477)) ;
#93639=CARTESIAN_POINT('Ctrl Pts',(-19.7327438594632,28.9922156115997,124.573634327147)) ;
#93640=CARTESIAN_POINT('Ctrl Pts',(-19.5283969535556,29.0021037728485,124.611863915237)) ;
#93641=CARTESIAN_POINT('Ctrl Pts',(-19.3184081587635,29.0120933273509,124.614447514576)) ;
#93642=CARTESIAN_POINT('Ctrl Pts',(-19.111830298825,29.0220517418745,124.580478875303)) ;
#93643=CARTESIAN_POINT('Ctrl Pts',(-18.9152650713988,29.0319516547039,124.512040435847)) ;
#93644=CARTESIAN_POINT('Ctrl Pts',(-18.7309320569869,29.0419983543538,124.408967920607)) ;
#93645=CARTESIAN_POINT('Ctrl Pts',(-18.5695640219657,29.0518982146594,124.277476297858)) ;
#93646=CARTESIAN_POINT('Ctrl Pts',(-18.4313829008868,29.0619496188649,124.117644033422)) ;
#93647=CARTESIAN_POINT('Ctrl Pts',(-18.3247938377839,29.071830655786,123.939309454891)) ;
#93648=CARTESIAN_POINT('Ctrl Pts',(-18.2496549087805,29.0818304879635,123.743005230981)) ;
#93649=CARTESIAN_POINT('Ctrl Pts',(-18.2098864002276,29.0917484909484,123.538288222219)) ;
#93650=CARTESIAN_POINT('Ctrl Pts',(-18.2062893402772,29.101799796823,123.327044380579)) ;
#93651=CARTESIAN_POINT('Ctrl Pts',(-18.2385895898733,29.1116696202145,123.122034275269)) ;
#93652=CARTESIAN_POINT('Ctrl Pts',(-18.3073743298631,29.1217437862648,122.921775498464)) ;
#93653=CARTESIAN_POINT('Ctrl Pts',(-18.4071229719738,29.1315638704064,122.740968848258)) ;
#93654=CARTESIAN_POINT('Ctrl Pts',(-18.5399452806073,29.1416425971423,122.575947060432)) ;
#93655=CARTESIAN_POINT('Ctrl Pts',(-18.6958377939681,29.1514941777918,122.439518109468)) ;
#93656=CARTESIAN_POINT('Ctrl Pts',(-18.8768647285279,29.1615673060902,122.329703311083)) ;
#93657=CARTESIAN_POINT('Ctrl Pts',(-19.0697539715149,29.1714097839817,122.254755402957)) ;
#93658=CARTESIAN_POINT('Ctrl Pts',(-19.2754083401487,29.1813903905797,122.213189337778)) ;
#93659=CARTESIAN_POINT('Ctrl Pts',(-19.4859556253967,29.1914080995985,122.208340236175)) ;
#93660=CARTESIAN_POINT('Ctrl Pts',(-19.6914902087443,29.2012942786359,122.239308640532)) ;
#93661=CARTESIAN_POINT('Ctrl Pts',(-19.891914245863,29.2113518912083,122.306617578102)) ;
#93662=CARTESIAN_POINT('Ctrl Pts',(-20.0742975022799,29.2212282845804,122.405879044779)) ;
#93663=CARTESIAN_POINT('Ctrl Pts',(-20.2389379215443,29.2312233127309,122.536433065238)) ;
#93664=CARTESIAN_POINT('Ctrl Pts',(-20.3785081239884,29.2412440595769,122.694246111613)) ;
#93665=CARTESIAN_POINT('Ctrl Pts',(-20.4874550726902,29.2511461282432,122.871631017611)) ;
#93666=CARTESIAN_POINT('Ctrl Pts',(-20.5649217144082,29.2611368680629,123.066861291378)) ;
#93667=CARTESIAN_POINT('Ctrl Pts',(-20.6070427330823,29.2711000642732,123.272029769209)) ;
#93668=CARTESIAN_POINT('Ctrl Pts',(-20.6133815278886,29.2810042485733,123.480169259069)) ;
#93669=CARTESIAN_POINT('Ctrl Pts',(-20.5828416977269,29.2910647089642,123.689429189581)) ;
#93670=CARTESIAN_POINT('Ctrl Pts',(-20.5181178875756,29.300905254835,123.885951501947)) ;
#93671=CARTESIAN_POINT('Ctrl Pts',(-20.418311802327,29.3109674755468,124.072440554193)) ;
#93672=CARTESIAN_POINT('Ctrl Pts',(-20.2895938220547,29.3208646185633,124.23593029093)) ;
#93673=CARTESIAN_POINT('Ctrl Pts',(-20.1343856308271,29.3307957949805,124.375570781385)) ;
#93674=CARTESIAN_POINT('Ctrl Pts',(-19.9551847138739,29.3408380087591,124.487181178999)) ;
#93675=CARTESIAN_POINT('Ctrl Pts',(-19.7624071884746,29.3507245489619,124.564908193393)) ;
#93676=CARTESIAN_POINT('Ctrl Pts',(-19.5569568086276,29.3607181435673,124.608773532661)) ;
#93677=CARTESIAN_POINT('Ctrl Pts',(-19.3480261657817,29.3706620187248,124.616231477838)) ;
#93678=CARTESIAN_POINT('Ctrl Pts',(-19.1406146804274,29.3806225548397,124.587525954481)) ;
#93679=CARTESIAN_POINT('Ctrl Pts',(-18.9405437862277,29.3906191581624,124.523120304653)) ;
#93680=CARTESIAN_POINT('Ctrl Pts',(-18.7541801489327,29.4006522411169,124.424343515166)) ;
#93681=CARTESIAN_POINT('Ctrl Pts',(-18.5906535250111,29.4105034098184,124.297265234718)) ;
#93682=CARTESIAN_POINT('Ctrl Pts',(-18.4496497544564,29.4204659005173,124.142407012302)) ;
#93683=CARTESIAN_POINT('Ctrl Pts',(-18.3371454253762,29.4304943289351,123.964090346421)) ;
#93684=CARTESIAN_POINT('Ctrl Pts',(-18.258197296594,29.4404046962996,123.771290942474)) ;
#93685=CARTESIAN_POINT('Ctrl Pts',(-18.2132772397129,29.4503395639147,123.56731028171)) ;
#93686=CARTESIAN_POINT('Ctrl Pts',(-18.2045597757948,29.4603807058938,123.35640066755)) ;
#93687=CARTESIAN_POINT('Ctrl Pts',(-18.2320230286963,29.4702678420969,123.150352720058)) ;
#93688=CARTESIAN_POINT('Ctrl Pts',(-18.295171910792,29.4802601245003,122.950015162677)) ;
#93689=CARTESIAN_POINT('Ctrl Pts',(-18.3917861917968,29.4902086524655,122.76450500273)) ;
#93690=CARTESIAN_POINT('Ctrl Pts',(-18.5187400411332,29.5001453836277,122.598627806259)) ;
#93691=CARTESIAN_POINT('Ctrl Pts',(-18.6731408343567,29.5101285944876,122.45643033864)) ;
#93692=CARTESIAN_POINT('Ctrl Pts',(-18.851110948505,29.5201716936375,122.342866870043)) ;
#93693=CARTESIAN_POINT('Ctrl Pts',(-19.0418426894045,29.5300026579124,122.263194748433)) ;
#93694=CARTESIAN_POINT('Ctrl Pts',(-19.2483822535319,29.5400755102984,122.21659540203)) ;
#93695=CARTESIAN_POINT('Ctrl Pts',(-19.4555494026138,29.5499396380101,122.206807368119)) ;
#93696=CARTESIAN_POINT('Ctrl Pts',(-19.6646004617306,29.559961840145,122.233040551303)) ;
#93697=CARTESIAN_POINT('Ctrl Pts',(-19.8658933921423,29.5699890331134,122.295687395274)) ;
#93698=CARTESIAN_POINT('Ctrl Pts',(-20.0501682924116,29.5798446270804,122.390377333857)) ;
#93699=CARTESIAN_POINT('Ctrl Pts',(-20.2172985588075,29.5898017989457,122.516433218997)) ;
#93700=CARTESIAN_POINT('Ctrl Pts',(-20.3608933785458,29.5998406429441,122.671082957337)) ;
#93701=CARTESIAN_POINT('Ctrl Pts',(-20.4739033940063,29.6097146668197,122.845240474739)) ;
#93702=CARTESIAN_POINT('Ctrl Pts',(-20.5565361370567,29.6197844928101,123.040115238253)) ;
#93703=CARTESIAN_POINT('Ctrl Pts',(-20.6030779835527,29.6296177367074,123.241551193442)) ;
#93704=CARTESIAN_POINT('Ctrl Pts',(-20.6147495285708,29.6396481644804,123.452092271116)) ;
#93705=CARTESIAN_POINT('Ctrl Pts',(-20.5890726666387,29.6496797812255,123.661431321394)) ;
#93706=CARTESIAN_POINT('Ctrl Pts',(-20.52909832052,29.6595094582063,123.859172832372)) ;
#93707=CARTESIAN_POINT('Ctrl Pts',(-20.4347319780937,29.6694989750462,124.046795681918)) ;
#93708=CARTESIAN_POINT('Ctrl Pts',(-20.3081181811144,29.679542587186,124.2157670466)) ;
#93709=CARTESIAN_POINT('Ctrl Pts',(-20.1577705367842,29.6893651935213,124.357328493109)) ;
#93710=CARTESIAN_POINT('Ctrl Pts',(-19.981608723437,29.6994034234205,124.473517346011)) ;
#93711=CARTESIAN_POINT('Ctrl Pts',(-19.7882588157214,29.7094144582124,124.556686172734)) ;
#93712=CARTESIAN_POINT('Ctrl Pts',(-19.5858185589827,29.7193121891796,124.604791883907)) ;
#93713=CARTESIAN_POINT('Ctrl Pts',(-19.3761865286974,29.72930181703,124.617404592721)) ;
#93714=CARTESIAN_POINT('Ctrl Pts',(-19.1682644871485,29.739257607476,124.593435204746)) ;
#93715=CARTESIAN_POINT('Ctrl Pts',(-18.9681109946795,29.7491850060381,124.53427779116)) ;
#93716=CARTESIAN_POINT('Ctrl Pts',(-18.7794620969067,29.759210601148,124.440297308764)) ;
#93717=CARTESIAN_POINT('Ctrl Pts',(-18.6122766523615,29.7690964518175,124.316833192583)) ;
#93718=CARTESIAN_POINT('Ctrl Pts',(-18.4672078455864,29.7790856316617,124.164980786501)) ;
#93719=CARTESIAN_POINT('Ctrl Pts',(-18.3504739229804,29.7891268187653,123.989097081875)) ;
#93720=CARTESIAN_POINT('Ctrl Pts',(-18.2674956322341,29.7989594622413,123.799773766715)) ;
#93721=CARTESIAN_POINT('Ctrl Pts',(-18.2172642416538,29.8089534119507,123.595763802256)) ;
#93722=CARTESIAN_POINT('Ctrl Pts',(-18.2036130491131,29.8189825347273,123.385360239602)) ;
#93723=CARTESIAN_POINT('Ctrl Pts',(-18.2260199316204,29.8288586656459,123.178935368539)) ;
#93724=CARTESIAN_POINT('Ctrl Pts',(-18.2843970103714,29.838856700663,122.977040721748)) ;
#93725=CARTESIAN_POINT('Ctrl Pts',(-18.3760423191995,29.8487706304217,122.789820229446)) ;
#93726=CARTESIAN_POINT('Ctrl Pts',(-18.5003433731899,29.8588138181595,122.619168157881)) ;
#93727=CARTESIAN_POINT('Ctrl Pts',(-18.6502274266148,29.8687136602998,122.474753639408)) ;
#93728=CARTESIAN_POINT('Ctrl Pts',(-18.8242469481258,29.8787049271078,122.357118255651)) ;
#93729=CARTESIAN_POINT('Ctrl Pts',(-19.0169820186433,29.8887370292398,122.27146823907)) ;
#93730=CARTESIAN_POINT('Ctrl Pts',(-19.2182167130968,29.8986039101946,122.221158081447)) ;
#93731=CARTESIAN_POINT('Ctrl Pts',(-19.4277225562127,29.9085957014827,122.205867869987)) ;
#93732=CARTESIAN_POINT('Ctrl Pts',(-19.6374978319252,29.9186278173942,122.227678697654)) ;
#93733=CARTESIAN_POINT('Ctrl Pts',(-19.8370434622058,29.9284941341943,122.284323905425)) ;
#93734=CARTESIAN_POINT('Ctrl Pts',(-20.0261335324257,29.9384816156679,122.37554305375)) ;
#93735=CARTESIAN_POINT('Ctrl Pts',(-20.1958973076224,29.9484265400468,122.497628705408)) ;
#93736=CARTESIAN_POINT('Ctrl Pts',(-20.3432317683155,29.9584714259575,122.648887749471)) ;
#93737=CARTESIAN_POINT('Ctrl Pts',(-20.4600715091523,29.96833352967,122.820180932939)) ;
#93738=CARTESIAN_POINT('Ctrl Pts',(-20.5468880523419,29.9783250934945,123.011437822122)) ;
#93739=CARTESIAN_POINT('Ctrl Pts',(-20.5987893949161,29.9882579015574,123.213703298745)) ;
#93740=CARTESIAN_POINT('Ctrl Pts',(-20.6153024480754,29.9981950037937,123.42197176182)) ;
#93741=CARTESIAN_POINT('Ctrl Pts',(-20.5948955430994,30.0082474500641,123.632302018946)) ;
#93742=CARTESIAN_POINT('Ctrl Pts',(-20.5397174255888,30.0180935656457,123.831827142723)) ;
#93743=CARTESIAN_POINT('Ctrl Pts',(-20.4492191323458,30.0281415853606,124.022684697215)) ;
#93744=CARTESIAN_POINT('Ctrl Pts',(-20.3279940404039,30.0380835369896,124.192964442128)) ;
#93745=CARTESIAN_POINT('Ctrl Pts',(-20.1794617902803,30.0480223179886,124.339923783225)) ;
#93746=CARTESIAN_POINT('Ctrl Pts',(-20.0060824903379,30.0580483667147,124.459764500437)) ;
#93747=CARTESIAN_POINT('Ctrl Pts',(-19.8172623374216,30.0679352271229,124.546716323164)) ;
#93748=CARTESIAN_POINT('Ctrl Pts',(-19.6133595715434,30.0779665022547,124.600410234333)) ;
#93749=CARTESIAN_POINT('Ctrl Pts',(-19.406276769601,30.0878494795551,124.617843641432)) ;
#93750=CARTESIAN_POINT('Ctrl Pts',(-19.1957687734416,30.0979063329623,124.598739082674)) ;
#93751=CARTESIAN_POINT('Ctrl Pts',(-18.9283788438819,30.1110745740382,124.526647204317)) ;
#93752=CARTESIAN_POINT('Ctrl Pts',(-18.6818038862875,30.1244756032648,124.384037954286)) ;
#93753=CARTESIAN_POINT('Ctrl Pts',(-18.4857400702449,30.1376885199956,124.187208658776)) ;
#93754=CARTESIAN_POINT('Ctrl Pts',(-18.3657914331037,30.1476169144488,124.016432936301)) ;
#93755=CARTESIAN_POINT('Ctrl Pts',(-18.27667684773,30.157598414577,123.826421025304)) ;
#93756=CARTESIAN_POINT('Ctrl Pts',(-18.2218764202102,30.1676389578471,123.622585918991)) ;
#93757=CARTESIAN_POINT('Ctrl Pts',(-18.2033813668389,30.1774882896302,123.416346847631)) ;
#93758=CARTESIAN_POINT('Ctrl Pts',(-18.2206996479079,30.1874836941018,123.206928562474)) ;
#93759=CARTESIAN_POINT('Ctrl Pts',(-18.2745929305749,30.1975000215504,123.00336725188)) ;
#93760=CARTESIAN_POINT('Ctrl Pts',(-18.3909391324748,30.210723678717,122.750841262503)) ;
#93761=CARTESIAN_POINT('Ctrl Pts',(-18.5712709750288,30.2240179701063,122.533213120822)) ;
#93762=CARTESIAN_POINT('Ctrl Pts',(-18.7990627197262,30.2373023210378,122.371616517048)) ;
#93763=CARTESIAN_POINT('Ctrl Pts',(-18.9884333932997,30.2472747020996,122.281709419626)) ;
#93764=CARTESIAN_POINT('Ctrl Pts',(-19.1891893546642,30.2571830817252,122.226046303007)) ;
#93765=CARTESIAN_POINT('Ctrl Pts',(-19.3995715842747,30.2672370804733,122.205891859953)) ;
#93766=CARTESIAN_POINT('Ctrl Pts',(-19.6062894044217,30.2770992775896,122.222096038525)) ;
#93767=CARTESIAN_POINT('Ctrl Pts',(-19.8780882299461,30.2904464039637,122.291836869342)) ;
#93768=CARTESIAN_POINT('Ctrl Pts',(-20.1845057827148,30.3069833696052,122.464304689986)) ;
#93769=CARTESIAN_POINT('Ctrl Pts',(-20.4154425890932,30.3236179737791,122.732190513317)) ;
#93770=CARTESIAN_POINT('Ctrl Pts',(-20.5367456008995,30.3369077670217,122.983880984554)) ;
#93771=CARTESIAN_POINT('Ctrl Pts',(-20.5937491456457,30.3468603982811,123.185188491695)) ;
#93772=CARTESIAN_POINT('Ctrl Pts',(-20.6151760929136,30.3568123655858,123.393329243809)) ;
#93773=CARTESIAN_POINT('Ctrl Pts',(-20.594811477217,30.3701796240496,123.673593988513)) ;
#93774=CARTESIAN_POINT('Ctrl Pts',(-20.4800576800383,30.3866964359988,124.005597356428)) ;
#93775=CARTESIAN_POINT('Ctrl Pts',(-20.2120200574859,30.4067223310052,124.33630959658)) ;
#93776=CARTESIAN_POINT('Ctrl Pts',(-19.8510357062947,30.4265330611353,124.553553092756)) ;
#93777=CARTESIAN_POINT('Ctrl Pts',(-19.4344067851742,30.4465102772652,124.636126295456)) ;
#93778=CARTESIAN_POINT('Ctrl Pts',(-19.0157736830144,30.4664371526604,124.570966794701)) ;
#93779=CARTESIAN_POINT('Ctrl Pts',(-18.6457429963977,30.4862586141367,124.369093095067)) ;
#93780=CARTESIAN_POINT('Ctrl Pts',(-18.363548673946,30.506332931946,124.048939383576)) ;
#93781=CARTESIAN_POINT('Ctrl Pts',(-18.2096218900021,30.5261809009539,123.65586546792)) ;
#93782=CARTESIAN_POINT('Ctrl Pts',(-18.1981503669756,30.5461279350171,123.231985052549)) ;
#93783=CARTESIAN_POINT('Ctrl Pts',(-18.3318134408227,30.5660238859893,122.830579187293)) ;
#93784=CARTESIAN_POINT('Ctrl Pts',(-18.5938415450344,30.5859193656075,122.498499856498)) ;
#93785=CARTESIAN_POINT('Ctrl Pts',(-18.9545567012551,30.6058754765723,122.274979593225)) ;
#93786=CARTESIAN_POINT('Ctrl Pts',(-19.3687580575178,30.6257800246123,122.188333583499)) ;
#93787=CARTESIAN_POINT('Ctrl Pts',(-19.787309036188,30.6456541489314,122.247107330277)) ;
#93788=CARTESIAN_POINT('Ctrl Pts',(-20.1636515869746,30.6657086789304,122.447450821914)) ;
#93789=CARTESIAN_POINT('Ctrl Pts',(-20.4457200252673,30.6855161926904,122.760325311286)) ;
#93790=CARTESIAN_POINT('Ctrl Pts',(-20.6062681553037,30.7054995484582,123.153662234623)) ;
#93791=CARTESIAN_POINT('Ctrl Pts',(-20.6222628106825,30.7254178510421,123.576872328483)) ;
#93792=CARTESIAN_POINT('Ctrl Pts',(-20.4942581051629,30.7452860664878,123.979555005816)) ;
#93793=CARTESIAN_POINT('Ctrl Pts',(-20.2337561496977,30.7653363832841,124.31687450115)) ;
#93794=CARTESIAN_POINT('Ctrl Pts',(-19.8787615933975,30.7851124451666,124.542563590445)) ;
#93795=CARTESIAN_POINT('Ctrl Pts',(-19.4626826204921,30.8051670508591,124.635079577957)) ;
#93796=CARTESIAN_POINT('Ctrl Pts',(-19.0452264153691,30.8249607400149,124.580607497338)) ;
#93797=CARTESIAN_POINT('Ctrl Pts',(-18.6678121500625,30.8449274316093,124.386388946373)) ;
#93798=CARTESIAN_POINT('Ctrl Pts',(-18.3797967323023,30.8648874773603,124.074567315355)) ;
#93799=CARTESIAN_POINT('Ctrl Pts',(-18.2157690972036,30.8847857375105,123.684593681658)) ;
#93800=CARTESIAN_POINT('Ctrl Pts',(-18.1941557059431,30.9046806530597,123.262145127519)) ;
#93801=CARTESIAN_POINT('Ctrl Pts',(-18.3177212165592,30.9245908334733,122.857238599372)) ;
#93802=CARTESIAN_POINT('Ctrl Pts',(-18.5722267685181,30.9445266325876,122.518239395623)) ;
#93803=CARTESIAN_POINT('Ctrl Pts',(-18.9271455247788,30.9644644942417,122.286400946768)) ;
#93804=CARTESIAN_POINT('Ctrl Pts',(-19.3394522574525,30.9843835408794,122.189424102124)) ;
#93805=CARTESIAN_POINT('Ctrl Pts',(-19.7607105590053,31.0043324389335,122.238978391336)) ;
#93806=CARTESIAN_POINT('Ctrl Pts',(-20.1390295702679,31.0242382663766,122.428816668531)) ;
#93807=CARTESIAN_POINT('Ctrl Pts',(-20.3815086749295,31.0408209617419,122.684686173166)) ;
#93808=CARTESIAN_POINT('Ctrl Pts',(-20.5148524519088,31.0540951754655,122.929906849042)) ;
#93809=CARTESIAN_POINT('Ctrl Pts',(-20.5818785615782,31.0641418946649,123.130173465987)) ;
#93810=CARTESIAN_POINT('Ctrl Pts',(-20.612716569486,31.0739859293105,123.334840505386)) ;
#93811=CARTESIAN_POINT('Ctrl Pts',(-20.6063535960019,31.0873203142151,123.615037179933)) ;
#93812=CARTESIAN_POINT('Ctrl Pts',(-20.507219363072,31.1039075315148,123.953619647069)) ;
#93813=CARTESIAN_POINT('Ctrl Pts',(-20.298254731138,31.1205407435527,124.238840949928)) ;
#93814=CARTESIAN_POINT('Ctrl Pts',(-20.0804677766212,31.1338231858249,124.413704891428)) ;
#93815=CARTESIAN_POINT('Ctrl Pts',(-19.8981272530352,31.1437290737391,124.514266945286)) ;
#93816=CARTESIAN_POINT('Ctrl Pts',(-19.6995096734775,31.1537174918443,124.582464176278)) ;
#93817=CARTESIAN_POINT('Ctrl Pts',(-19.4913126073824,31.163740919083,124.615029422645)) ;
#93818=CARTESIAN_POINT('Ctrl Pts',(-19.2831318881171,31.1736453502,124.611113982746)) ;
#93819=CARTESIAN_POINT('Ctrl Pts',(-19.0093613876071,31.1869085028104,124.55827225687)) ;
#93820=CARTESIAN_POINT('Ctrl Pts',(-18.7546009692031,31.2002334007143,124.434360468631)) ;
#93821=CARTESIAN_POINT('Ctrl Pts',(-18.5439609812997,31.2134891443299,124.251809930995)) ;
#93822=CARTESIAN_POINT('Ctrl Pts',(-18.411728227131,31.2234485177772,124.08951227342)) ;
#93823=CARTESIAN_POINT('Ctrl Pts',(-18.3095841664041,31.2333923417042,123.907084589066)) ;
#93824=CARTESIAN_POINT('Ctrl Pts',(-18.2401310461763,31.2434402858515,123.707606262789)) ;
#93825=CARTESIAN_POINT('Ctrl Pts',(-18.2068457678084,31.2532912570697,123.503187613083)) ;
#93826=CARTESIAN_POINT('Ctrl Pts',(-18.20905246238,31.2632630745117,123.293584227072)) ;
#93827=CARTESIAN_POINT('Ctrl Pts',(-18.2477548076841,31.2732584968038,123.087014109771)) ;
#93828=CARTESIAN_POINT('Ctrl Pts',(-18.3222090846656,31.2832915619275,122.889672405857)) ;
#93829=CARTESIAN_POINT('Ctrl Pts',(-18.4278263479908,31.2931568945927,122.711184480995)) ;
#93830=CARTESIAN_POINT('Ctrl Pts',(-18.5636713784596,31.3031174371903,122.551819024002)) ;
#93831=CARTESIAN_POINT('Ctrl Pts',(-18.7265249519125,31.313151122692,122.417766687849)) ;
#93832=CARTESIAN_POINT('Ctrl Pts',(-18.9073121476128,31.3230359546823,122.315233347034)) ;
#93833=CARTESIAN_POINT('Ctrl Pts',(-19.1067295589491,31.3331033814421,122.244429547417)) ;
#93834=CARTESIAN_POINT('Ctrl Pts',(-19.3107004512961,31.342941870601,122.209912168655)) ;
#93835=CARTESIAN_POINT('Ctrl Pts',(-19.5222335142052,31.3530053517911,122.211086088931)) ;
#93836=CARTESIAN_POINT('Ctrl Pts',(-19.7268674194447,31.3628995096062,122.248520775876)) ;
#93837=CARTESIAN_POINT('Ctrl Pts',(-19.9229838875696,31.3728413663505,122.320715620495)) ;
#93838=CARTESIAN_POINT('Ctrl Pts',(-20.1047748499077,31.3828438440219,122.426467358544)) ;
#93839=CARTESIAN_POINT('Ctrl Pts',(-20.2657147069535,31.3928786483262,122.562842390076)) ;
#93840=CARTESIAN_POINT('Ctrl Pts',(-20.3982636565813,31.4027235251719,122.721817859034)) ;
#93841=CARTESIAN_POINT('Ctrl Pts',(-20.5029887534451,31.4127094047274,122.903726837913)) ;
#93842=CARTESIAN_POINT('Ctrl Pts',(-20.5743391725136,31.4226441350859,123.10006380969)) ;
#93843=CARTESIAN_POINT('Ctrl Pts',(-20.6107539159003,31.4327019473988,123.308316182202)) ;
#93844=CARTESIAN_POINT('Ctrl Pts',(-20.6108179022155,31.4425225395232,123.514810058563)) ;
#93845=CARTESIAN_POINT('Ctrl Pts',(-20.5744003078764,31.452589125133,123.72324139053)) ;
#93846=CARTESIAN_POINT('Ctrl Pts',(-20.5034740799045,31.4624887057148,123.918955059756)) ;
#93847=CARTESIAN_POINT('Ctrl Pts',(-20.3981618169355,31.472540305393,124.102114221002)) ;
#93848=CARTESIAN_POINT('Ctrl Pts',(-20.2651091885193,31.48241449181,124.261505375485)) ;
#93849=CARTESIAN_POINT('Ctrl Pts',(-20.1036202261952,31.4924709676909,124.397897467867)) ;
#93850=CARTESIAN_POINT('Ctrl Pts',(-19.9238419339266,31.5023638989935,124.502558096768)) ;
#93851=CARTESIAN_POINT('Ctrl Pts',(-19.7253582990717,31.5124266777062,124.575658467027)) ;
#93852=CARTESIAN_POINT('Ctrl Pts',(-19.5217145691087,31.5222692032873,124.612477742698)) ;
#93853=CARTESIAN_POINT('Ctrl Pts',(-19.3117088928933,31.5322599687122,124.613893836297)) ;
#93854=CARTESIAN_POINT('Ctrl Pts',(-19.1059168231698,31.5421880447102,124.579001619905)) ;
#93855=CARTESIAN_POINT('Ctrl Pts',(-18.9080017720923,31.5521759550973,124.508830986681)) ;
#93856=CARTESIAN_POINT('Ctrl Pts',(-18.7245905279759,31.5622118672222,124.404561299914)) ;
#93857=CARTESIAN_POINT('Ctrl Pts',(-18.5647630549477,31.5720668800699,124.272702953155)) ;
#93858=CARTESIAN_POINT('Ctrl Pts',(-18.4281031702416,31.5820658259861,124.113022565623)) ;
#93859=CARTESIAN_POINT('Ctrl Pts',(-18.3221273012406,31.5919627384341,123.933932741942)) ;
#93860=CARTESIAN_POINT('Ctrl Pts',(-18.2476926082371,31.6020165365276,123.736138071533)) ;
#93861=CARTESIAN_POINT('Ctrl Pts',(-18.2093337816089,31.6118974573543,123.531959013268)) ;
#93862=CARTESIAN_POINT('Ctrl Pts',(-18.2066019685682,31.6219019833521,123.321674479705)) ;
#93863=CARTESIAN_POINT('Ctrl Pts',(-18.2404263407543,31.6318859469695,123.114487635351)) ;
#93864=CARTESIAN_POINT('Ctrl Pts',(-18.3102692992162,31.6419255875208,122.91532989079)) ;
#93865=CARTESIAN_POINT('Ctrl Pts',(-18.4114038129035,31.6517696131355,122.734771558271)) ;
#93866=CARTESIAN_POINT('Ctrl Pts',(-18.5438394807162,31.6617606189529,122.571741140915)) ;
#93867=CARTESIAN_POINT('Ctrl Pts',(-18.7036285848506,31.6717984104851,122.433903147432)) ;
#93868=CARTESIAN_POINT('Ctrl Pts',(-18.8812503177922,31.6816428102735,122.327667870573)) ;
#93869=CARTESIAN_POINT('Ctrl Pts',(-19.0771971755672,31.6916276108302,122.252460208954)) ;
#93870=CARTESIAN_POINT('Ctrl Pts',(-19.2823298077936,31.7015671342414,122.21249959101)) ;
#93871=CARTESIAN_POINT('Ctrl Pts',(-19.4933471182147,31.7116068533424,122.208776390442)) ;
#93872=CARTESIAN_POINT('Ctrl Pts',(-19.6987028225727,31.7214950252616,122.241153193864)) ;
#93873=CARTESIAN_POINT('Ctrl Pts',(-19.8974425155665,31.7314845876786,122.309009005677)) ;
#93874=CARTESIAN_POINT('Ctrl Pts',(-20.0807345289444,31.7414429598733,122.410164926042)) ;
#93875=CARTESIAN_POINT('Ctrl Pts',(-20.2430472008146,31.751343034104,122.540457091883)) ;
#93876=CARTESIAN_POINT('Ctrl Pts',(-20.3822631308276,31.7613891304776,122.699266960412)) ;
#93877=CARTESIAN_POINT('Ctrl Pts',(-20.4903109489229,31.7712977144747,122.877375084969)) ;
#93878=CARTESIAN_POINT('Ctrl Pts',(-20.566929490437,31.7813082930656,123.073389758785)) ;
#93879=CARTESIAN_POINT('Ctrl Pts',(-20.6080089158008,31.7913374511785,123.280201568448)) ;
#93880=CARTESIAN_POINT('Ctrl Pts',(-20.6127724616542,31.8011903330165,123.487271818897)) ;
#93881=CARTESIAN_POINT('Ctrl Pts',(-20.581806626969,31.8111498941675,123.694357030942)) ;
#93882=CARTESIAN_POINT('Ctrl Pts',(-20.5144687823656,31.8211883287566,123.894350895927)) ;
#93883=CARTESIAN_POINT('Ctrl Pts',(-20.415413063055,31.8310616009837,124.076794583067)) ;
#93884=CARTESIAN_POINT('Ctrl Pts',(-20.2835620404911,31.8411348429773,124.242457424024)) ;
#93885=CARTESIAN_POINT('Ctrl Pts',(-20.1290461488142,31.8509551745104,124.379450070107)) ;
#93886=CARTESIAN_POINT('Ctrl Pts',(-19.9486477522964,31.8610338357371,124.490491065507)) ;
#93887=CARTESIAN_POINT('Ctrl Pts',(-19.7560811050293,31.8708854310314,124.566868118361)) ;
#93888=CARTESIAN_POINT('Ctrl Pts',(-19.5487382827828,31.8809585662602,124.609752344747)) ;
#93889=CARTESIAN_POINT('Ctrl Pts',(-19.3418894357439,31.8908010017852,124.615811183682)) ;
#93890=CARTESIAN_POINT('Ctrl Pts',(-19.1341823671792,31.9007817709186,124.586138256737)) ;
#93891=CARTESIAN_POINT('Ctrl Pts',(-18.9341677996777,31.9107988721625,124.520238635541)) ;
#93892=CARTESIAN_POINT('Ctrl Pts',(-18.7508181677505,31.9206873197643,124.422228288085)) ;
#93893=CARTESIAN_POINT('Ctrl Pts',(-18.5845186028101,31.9307430339452,124.291738473027)) ;
#93894=CARTESIAN_POINT('Ctrl Pts',(-18.4458907438833,31.940618240359,124.137177719014)) ;
#93895=CARTESIAN_POINT('Ctrl Pts',(-18.3344556958182,31.9506132928317,123.959039423795)) ;
#93896=CARTESIAN_POINT('Ctrl Pts',(-18.2557440922024,31.9606351767938,123.763594402639)) ;
#93897=CARTESIAN_POINT('Ctrl Pts',(-18.2124503481654,31.9705391493231,123.559934304139)) ;
#93898=CARTESIAN_POINT('Ctrl Pts',(-18.2048119891636,31.980527645984,123.350081973959)) ;
#93899=CARTESIAN_POINT('Ctrl Pts',(-18.2337946115859,31.990491443232,123.142637302614)) ;
#93900=CARTESIAN_POINT('Ctrl Pts',(-18.2974930953008,32.00039546654,122.944386197689)) ;
#93901=CARTESIAN_POINT('Ctrl Pts',(-18.3963169602381,32.0104559698617,122.757419517568)) ;
#93902=CARTESIAN_POINT('Ctrl Pts',(-18.5230894198488,32.0202965050015,122.593899269698)) ;
#93903=CARTESIAN_POINT('Ctrl Pts',(-18.6795617836755,32.0303587257061,122.451576324891)) ;
#93904=CARTESIAN_POINT('Ctrl Pts',(-18.8555799237942,32.0402558794824,122.340603849521)) ;
#93905=CARTESIAN_POINT('Ctrl Pts',(-19.0485759335199,32.0501870128678,122.260971589894)) ;
#93906=CARTESIAN_POINT('Ctrl Pts',(-19.2548021702129,32.0602293880136,122.21578488518)) ;
#93907=CARTESIAN_POINT('Ctrl Pts',(-19.4624645914711,32.0701153257797,122.207066666525)) ;
#93908=CARTESIAN_POINT('Ctrl Pts',(-19.6707916606036,32.0801111687645,122.234516690486)) ;
#93909=CARTESIAN_POINT('Ctrl Pts',(-19.8701273889737,32.0900531466432,122.297413037221)) ;
#93910=CARTESIAN_POINT('Ctrl Pts',(-20.055949568507,32.1000125211241,122.393870336215)) ;
#93911=CARTESIAN_POINT('Ctrl Pts',(-20.2229151924571,32.1100091369579,122.521538014779)) ;
#93912=CARTESIAN_POINT('Ctrl Pts',(-20.3654870724293,32.1200433555314,122.6770082414)) ;
#93913=CARTESIAN_POINT('Ctrl Pts',(-20.4770646674535,32.129896422742,122.851527849583)) ;
#93914=CARTESIAN_POINT('Ctrl Pts',(-20.5580731723028,32.1398566806196,123.044611510919)) ;
#93915=CARTESIAN_POINT('Ctrl Pts',(-20.6044060123665,32.1498857073252,123.250311138346)) ;
#93916=CARTESIAN_POINT('Ctrl Pts',(-20.6142619787569,32.1597959143596,123.458412203081)) ;
#93917=CARTESIAN_POINT('Ctrl Pts',(-20.5883124116075,32.1697308250073,123.665662854138)) ;
#93918=CARTESIAN_POINT('Ctrl Pts',(-20.5259287030354,32.1797719551865,123.867323632054)) ;
#93919=CARTESIAN_POINT('Ctrl Pts',(-20.4310789187822,32.1896590955564,124.052292571989)) ;
#93920=CARTESIAN_POINT('Ctrl Pts',(-20.304513568402,32.1996513730924,124.219935519192)) ;
#93921=CARTESIAN_POINT('Ctrl Pts',(-20.1513762537152,32.2095999163607,124.362403856439)) ;
#93922=CARTESIAN_POINT('Ctrl Pts',(-19.976222390719,32.2195365911779,124.476218544844)) ;
#93923=CARTESIAN_POINT('Ctrl Pts',(-19.7831273118122,32.2295200121143,124.558523255501)) ;
#93924=CARTESIAN_POINT('Ctrl Pts',(-19.5774220081885,32.2395623273035,124.60598952607)) ;
#93925=CARTESIAN_POINT('Ctrl Pts',(-19.370845783349,32.2494026447427,124.617131308985)) ;
#93926=CARTESIAN_POINT('Ctrl Pts',(-19.1614606932978,32.2594323488002,124.592247049421)) ;
#93927=CARTESIAN_POINT('Ctrl Pts',(-18.9599203041336,32.2694533055227,124.530895300264)) ;
#93928=CARTESIAN_POINT('Ctrl Pts',(-18.7747348258612,32.2793198478263,124.437418896063)) ;
#93929=CARTESIAN_POINT('Ctrl Pts',(-18.6051744995746,32.2893909477715,124.310654941653)) ;
#93930=CARTESIAN_POINT('Ctrl Pts',(-18.4634825926305,32.2992330219491,124.159861061519)) ;
#93931=CARTESIAN_POINT('Ctrl Pts',(-18.3481195405836,32.3091938165361,123.985101895507)) ;
#93932=CARTESIAN_POINT('Ctrl Pts',(-18.2645928561442,32.3192316894369,123.791315971168)) ;
#93933=CARTESIAN_POINT('Ctrl Pts',(-18.2163931560725,32.329105974981,123.589374702714)) ;
#93934=CARTESIAN_POINT('Ctrl Pts',(-18.2037592119265,32.3391757253949,123.378082427202)) ;
#93935=CARTESIAN_POINT('Ctrl Pts',(-18.227329317313,32.3490090099296,123.172687270205)) ;
#93936=CARTESIAN_POINT('Ctrl Pts',(-18.286804334451,32.3590393507296,122.970385364036)) ;
#93937=CARTESIAN_POINT('Ctrl Pts',(-18.3810784901195,32.3690712747292,122.781715083692)) ;
#93938=CARTESIAN_POINT('Ctrl Pts',(-18.5037608147932,32.3788998096651,122.615463900118)) ;
#93939=CARTESIAN_POINT('Ctrl Pts',(-18.6555715303038,32.3888935874298,122.470222048311)) ;
#93940=CARTESIAN_POINT('Ctrl Pts',(-18.831125396415,32.3989212979154,122.353490733339)) ;
#93941=CARTESIAN_POINT('Ctrl Pts',(-19.0214892135476,32.4088097087493,122.269952809508)) ;
#93942=CARTESIAN_POINT('Ctrl Pts',(-19.2251690134222,32.4187865592849,122.219945129683)) ;
#93943=CARTESIAN_POINT('Ctrl Pts',(-19.4347962245961,32.4287783558353,122.206021141122)) ;
#93944=CARTESIAN_POINT('Ctrl Pts',(-19.644506261985,32.438814361929,122.229058208528)) ;
#93945=CARTESIAN_POINT('Ctrl Pts',(-19.8434117000005,32.4486650961918,122.286768450551)) ;
#93946=CARTESIAN_POINT('Ctrl Pts',(-20.0320459339982,32.45865635472,122.379097167223)) ;
#93947=CARTESIAN_POINT('Ctrl Pts',(-20.20065583118,32.4685742496232,122.501801180577)) ;
#93948=CARTESIAN_POINT('Ctrl Pts',(-20.3470163566351,32.4786023912863,122.653517378883)) ;
#93949=CARTESIAN_POINT('Ctrl Pts',(-20.4632160358938,32.4884875594021,122.825818794577)) ;
#93950=CARTESIAN_POINT('Ctrl Pts',(-20.5490902320439,32.4984769229081,123.017471259713)) ;
#93951=CARTESIAN_POINT('Ctrl Pts',(-20.600215334556,32.5085180579182,123.222283152939)) ;
#93952=CARTESIAN_POINT('Ctrl Pts',(-20.6150344433959,32.5183507261062,123.428460755687)) ;
#93953=CARTESIAN_POINT('Ctrl Pts',(-20.5940801019573,32.5283446290607,123.637515476195)) ;
#93954=CARTESIAN_POINT('Ctrl Pts',(-20.5365126203396,32.5383739141452,123.84035345709)) ;
#93955=CARTESIAN_POINT('Ctrl Pts',(-20.4463103931362,32.5482494425871,124.027361177851)) ;
#93956=CARTESIAN_POINT('Ctrl Pts',(-20.3236864942559,32.5582497252032,124.198101790075)) ;
#93957=CARTESIAN_POINT('Ctrl Pts',(-20.1746881469823,32.5681617412602,124.343816676878)) ;
#93958=CARTESIAN_POINT('Ctrl Pts',(-20.0004586794093,32.5782038165992,124.463012680978)) ;
#93959=CARTESIAN_POINT('Ctrl Pts',(-19.8108772885679,32.5881036492553,124.548917301885)) ;
#93960=CARTESIAN_POINT('Ctrl Pts',(-19.6075007703568,32.5980960498334,124.601531937198)) ;
#93961=CARTESIAN_POINT('Ctrl Pts',(-19.3971732299059,32.6081300715927,124.617729269594)) ;
#93962=CARTESIAN_POINT('Ctrl Pts',(-19.1907544289852,32.6179946824339,124.597773975522)) ;
#93963=CARTESIAN_POINT('Ctrl Pts',(-18.9882033401432,32.6279870818951,124.542054825909)) ;
#93964=CARTESIAN_POINT('Ctrl Pts',(-18.7978334954326,32.638019035228,124.451283460562)) ;
#93965=CARTESIAN_POINT('Ctrl Pts',(-18.628758986435,32.6478853941696,124.331111736303)) ;
#93966=CARTESIAN_POINT('Ctrl Pts',(-18.4811111490169,32.6578728696554,124.181860126214)) ;
#93967=CARTESIAN_POINT('Ctrl Pts',(-18.3620060824983,32.6678177758439,124.009992191636)) ;
#93968=CARTESIAN_POINT('Ctrl Pts',(-18.2738030986385,32.6778627405042,123.818139912872)) ;
#93969=CARTESIAN_POINT('Ctrl Pts',(-18.2210369220025,32.687724547409,123.617622964085)) ;
#93970=CARTESIAN_POINT('Ctrl Pts',(-18.2032624857516,32.6977172197148,123.408320481454)) ;
#93971=CARTESIAN_POINT('Ctrl Pts',(-18.2220069176133,32.7076458906601,123.20041822076)) ;
#93972=CARTESIAN_POINT('Ctrl Pts',(-18.2763580861567,32.7175984328854,122.998381912179)) ;
#93973=CARTESIAN_POINT('Ctrl Pts',(-18.3653128531859,32.7275997888813,122.807841810315)) ;
#93974=CARTESIAN_POINT('Ctrl Pts',(-18.4865473980735,32.737628401156,122.635363522157)) ;
#93975=CARTESIAN_POINT('Ctrl Pts',(-18.6332437506047,32.7474927357055,122.488761340732)) ;
#93976=CARTESIAN_POINT('Ctrl Pts',(-18.8051496446684,32.7574850597821,122.36807151102)) ;
#93977=CARTESIAN_POINT('Ctrl Pts',(-18.9941648299301,32.767412552148,122.279502896723)) ;
#93978=CARTESIAN_POINT('Ctrl Pts',(-19.1976622179447,32.7774399106988,122.224574409958)) ;
#93979=CARTESIAN_POINT('Ctrl Pts',(-19.4046917324504,32.7873263287499,122.2058521457)) ;
#93980=CARTESIAN_POINT('Ctrl Pts',(-19.6148150461169,32.7973580634853,122.223507004572)) ;
#93981=CARTESIAN_POINT('Ctrl Pts',(-19.8157515091835,32.8072396447286,122.276392589365)) ;
#93982=CARTESIAN_POINT('Ctrl Pts',(-20.0078550070822,32.8173016227609,122.364875768334)) ;
#93983=CARTESIAN_POINT('Ctrl Pts',(-20.1782306508466,32.8271587011226,122.482889602471)) ;
#93984=CARTESIAN_POINT('Ctrl Pts',(-20.3278335781113,32.8371532742286,122.63038217435)) ;
#93985=CARTESIAN_POINT('Ctrl Pts',(-20.4488151036229,32.8470790705162,122.800439225397)) ;
#93986=CARTESIAN_POINT('Ctrl Pts',(-20.5393606750725,32.857104437686,122.990744699707)) ;
#93987=CARTESIAN_POINT('Ctrl Pts',(-20.5948558931184,32.8670005173398,123.191261961852)) ;
#93988=CARTESIAN_POINT('Ctrl Pts',(-20.6153122258122,32.8769955970454,123.400395012648)) ;
#93989=CARTESIAN_POINT('Ctrl Pts',(-20.5987383876886,32.8870206848612,123.61049872856)) ;
#93990=CARTESIAN_POINT('Ctrl Pts',(-20.5297765684024,32.9002045072285,123.878959402027)) ;
#93991=CARTESIAN_POINT('Ctrl Pts',(-20.3913921904728,32.9135266253744,124.126130710772)) ;
#93992=CARTESIAN_POINT('Ctrl Pts',(-20.19452440354,32.926905835002,124.327020138545)) ;
#93993=CARTESIAN_POINT('Ctrl Pts',(-20.0266226033983,32.9367440722462,124.44783150031)) ;
#93994=CARTESIAN_POINT('Ctrl Pts',(-19.8359283011779,32.946816995505,124.539857209982)) ;
#93995=CARTESIAN_POINT('Ctrl Pts',(-19.636475161509,32.9566736369601,124.596128301881)) ;
#93996=CARTESIAN_POINT('Ctrl Pts',(-19.4276788172328,32.9666590124661,124.617742244852)) ;
#93997=CARTESIAN_POINT('Ctrl Pts',(-19.1491574998988,32.9799430439266,124.597574269333)) ;
#93998=CARTESIAN_POINT('Ctrl Pts',(-18.8168323648983,32.9964618357969,124.483616253666)) ;
#93999=CARTESIAN_POINT('Ctrl Pts',(-18.5395293019572,33.0132475528035,124.258981058193)) ;
#94000=CARTESIAN_POINT('Ctrl Pts',(-18.3774838302802,33.0263607013125,124.03593563537)) ;
#94001=CARTESIAN_POINT('Ctrl Pts',(-18.2842424376634,33.0363962503927,123.846700449347)) ;
#94002=CARTESIAN_POINT('Ctrl Pts',(-18.2259657532557,33.0464123065721,123.644335341061)) ;
#94003=CARTESIAN_POINT('Ctrl Pts',(-18.1960980277627,33.0595903424381,123.368929108419)) ;
#94004=CARTESIAN_POINT('Ctrl Pts',(-18.249009068452,33.0761922196252,123.019870829491)) ;
#94005=CARTESIAN_POINT('Ctrl Pts',(-18.4541282278557,33.0962553642411,122.645836767002)) ;
#94006=CARTESIAN_POINT('Ctrl Pts',(-18.7702599399458,33.1160562543248,122.367699508077)) ;
#94007=CARTESIAN_POINT('Ctrl Pts',(-19.1646436097345,33.1359993796035,122.212088074681)) ;
#94008=CARTESIAN_POINT('Ctrl Pts',(-19.5875674444081,33.1558974247231,122.200707746855)) ;
#94009=CARTESIAN_POINT('Ctrl Pts',(-19.9891372297378,33.1757831843499,122.333269321232)) ;
#94010=CARTESIAN_POINT('Ctrl Pts',(-20.3238757638564,33.1958483595298,122.597734163642)) ;
#94011=CARTESIAN_POINT('Ctrl Pts',(-20.5455361464889,33.2156750026326,122.956408640357)) ;
#94012=CARTESIAN_POINT('Ctrl Pts',(-20.6329532940323,33.2355837120809,123.370483063395)) ;
#94013=CARTESIAN_POINT('Ctrl Pts',(-20.5737633317445,33.2555355491127,123.790683278414)) ;
#94014=CARTESIAN_POINT('Ctrl Pts',(-20.3736428549386,33.2755440238159,124.166059655806)) ;
#94015=CARTESIAN_POINT('Ctrl Pts',(-20.0610026351362,33.2953454825774,124.448078284443)) ;
#94016=CARTESIAN_POINT('Ctrl Pts',(-19.6682567912983,33.3153023708133,124.608739938884)) ;
#94017=CARTESIAN_POINT('Ctrl Pts',(-19.2436658991202,33.3352862082274,124.624794629549)) ;
#94018=CARTESIAN_POINT('Ctrl Pts',(-18.8423051955773,33.3550946474483,124.496925784689)) ;
#94019=CARTESIAN_POINT('Ctrl Pts',(-18.5055646804555,33.3750803568285,124.23792646132)) ;
#94020=CARTESIAN_POINT('Ctrl Pts',(-18.2784679309149,33.3949498798438,123.881467993648)) ;
#94021=CARTESIAN_POINT('Ctrl Pts',(-18.1861872022792,33.414970618961,123.466059954206)) ;
#94022=CARTESIAN_POINT('Ctrl Pts',(-18.2401103646195,33.434774683938,123.04827687891)) ;
#94023=CARTESIAN_POINT('Ctrl Pts',(-18.4356216338899,33.4548366476687,122.669283035996)) ;
#94024=CARTESIAN_POINT('Ctrl Pts',(-18.7455985363762,33.4746698279572,122.383215081559)) ;
#94025=CARTESIAN_POINT('Ctrl Pts',(-19.1356568720352,33.4945890252833,122.218360374469)) ;
#94026=CARTESIAN_POINT('Ctrl Pts',(-19.5590433618675,33.5145270503966,122.196755247906)) ;
#94027=CARTESIAN_POINT('Ctrl Pts',(-19.9633828670812,33.5344050964527,122.319991735649)) ;
#94028=CARTESIAN_POINT('Ctrl Pts',(-20.3031557635292,33.5543898307408,122.575085905004)) ;
#94029=CARTESIAN_POINT('Ctrl Pts',(-20.5347847173385,33.5743006474192,122.929604659567)) ;
#94030=CARTESIAN_POINT('Ctrl Pts',(-20.6316400602913,33.594299622938,123.343555625924)) ;
#94031=CARTESIAN_POINT('Ctrl Pts',(-20.5824164230939,33.6141045435832,123.76186141104)) ;
#94032=CARTESIAN_POINT('Ctrl Pts',(-20.3923377698782,33.6340885038744,124.141776622175)) ;
#94033=CARTESIAN_POINT('Ctrl Pts',(-20.0852720477215,33.6539747075983,124.432586156203)) ;
#94034=CARTESIAN_POINT('Ctrl Pts',(-19.6964740225764,33.6739238859215,124.602080267117)) ;
#94035=CARTESIAN_POINT('Ctrl Pts',(-19.2741491376864,33.6938256851611,124.628564548105)) ;
#94036=CARTESIAN_POINT('Ctrl Pts',(-18.8683285448155,33.7137042902134,124.510329651204)) ;
#94037=CARTESIAN_POINT('Ctrl Pts',(-18.5246878694578,33.7337366499391,124.25860986934)) ;
#94038=CARTESIAN_POINT('Ctrl Pts',(-18.3288960189047,33.7503183758952,123.965412227586)) ;
#94039=CARTESIAN_POINT('Ctrl Pts',(-18.2390050907731,33.7635125461931,123.702986209671)) ;
#94040=CARTESIAN_POINT('Ctrl Pts',(-18.1952156177926,33.7768247242863,123.426625334164)) ;
#94041=CARTESIAN_POINT('Ctrl Pts',(-18.2318570630628,33.7933909038797,123.076205385333)) ;
#94042=CARTESIAN_POINT('Ctrl Pts',(-18.3860721862211,33.8100190987398,122.758154709291)) ;
#94043=CARTESIAN_POINT('Ctrl Pts',(-18.5689208252892,33.8233076804496,122.546840432234)) ;
#94044=CARTESIAN_POINT('Ctrl Pts',(-18.7313513600234,33.8332759285532,122.414464321672)) ;
#94045=CARTESIAN_POINT('Ctrl Pts',(-18.9132140980837,33.8431906848093,122.3126070292)) ;
#94046=CARTESIAN_POINT('Ctrl Pts',(-19.1118793081902,33.8532038354605,122.242971307664)) ;
#94047=CARTESIAN_POINT('Ctrl Pts',(-19.3196579468143,33.8632165426625,122.209223877592)) ;
#94048=CARTESIAN_POINT('Ctrl Pts',(-19.5975383974733,33.8764358313538,122.212437339034)) ;
#94049=CARTESIAN_POINT('Ctrl Pts',(-19.9378289154735,33.8930545123519,122.307523681823)) ;
#94050=CARTESIAN_POINT('Ctrl Pts',(-20.2246132383355,33.9096194201253,122.512032246006)) ;
#94051=CARTESIAN_POINT('Ctrl Pts',(-20.4036557241936,33.9230178917362,122.729519796154)) ;
#94052=CARTESIAN_POINT('Ctrl Pts',(-20.5055966782541,33.9328591472231,122.90956884558)) ;
#94053=CARTESIAN_POINT('Ctrl Pts',(-20.5761690139135,33.9428454628113,123.107261429492)) ;
#94054=CARTESIAN_POINT('Ctrl Pts',(-20.611277650306,33.9527820703977,123.313223876353)) ;
#94055=CARTESIAN_POINT('Ctrl Pts',(-20.6099735810756,33.962831937766,123.524478262439)) ;
#94056=CARTESIAN_POINT('Ctrl Pts',(-20.5729077462783,33.9726824324408,123.728238382038)) ;
#94057=CARTESIAN_POINT('Ctrl Pts',(-20.5006686095977,33.9826542328353,123.925008548222)) ;
#94058=CARTESIAN_POINT('Ctrl Pts',(-20.3950540740797,33.9926501998612,124.10672846331)) ;
#94059=CARTESIAN_POINT('Ctrl Pts',(-20.2587448232907,34.0026876592423,124.267788333487)) ;
#94060=CARTESIAN_POINT('Ctrl Pts',(-20.0999443163612,34.0125283601431,124.400411931469)) ;
#94061=CARTESIAN_POINT('Ctrl Pts',(-19.9169251629919,34.0225763814104,124.505877195558)) ;
#94062=CARTESIAN_POINT('Ctrl Pts',(-19.7202373371653,34.0325237744931,124.576929500884)) ;
#94063=CARTESIAN_POINT('Ctrl Pts',(-19.5150731670735,34.0424339205395,124.613246052084)) ;
#94064=CARTESIAN_POINT('Ctrl Pts',(-19.3036248985833,34.0524928343891,124.613150607423)) ;
#94065=CARTESIAN_POINT('Ctrl Pts',(-19.0998219185754,34.0623336046784,124.577418243024)) ;
#94066=CARTESIAN_POINT('Ctrl Pts',(-18.9008963171724,34.0723964742571,124.505500639989)) ;
#94067=CARTESIAN_POINT('Ctrl Pts',(-18.7205944492889,34.0822907973875,124.40172913725)) ;
#94068=CARTESIAN_POINT('Ctrl Pts',(-18.5599579858126,34.092232604482,124.268052319502)) ;
#94069=CARTESIAN_POINT('Ctrl Pts',(-18.4240523603938,34.1022351154374,124.107549491577)) ;
#94070=CARTESIAN_POINT('Ctrl Pts',(-18.3180449838166,34.1122698362557,123.925171270293)) ;
#94071=CARTESIAN_POINT('Ctrl Pts',(-18.2463591434105,34.1221150137615,123.730992524548)) ;
#94072=CARTESIAN_POINT('Ctrl Pts',(-18.2085560215957,34.1320997741625,123.524543616155)) ;
#94073=CARTESIAN_POINT('Ctrl Pts',(-18.2070790891431,34.1420386804789,123.315570306909)) ;
#94074=CARTESIAN_POINT('Ctrl Pts',(-18.2423345297915,34.1520809081147,123.107437286142)) ;
#94075=CARTESIAN_POINT('Ctrl Pts',(-18.3119591437577,34.161966119699,122.911604453223)) ;
#94076=CARTESIAN_POINT('Ctrl Pts',(-18.415446825498,34.171965049901,122.72866948783)) ;
#94077=CARTESIAN_POINT('Ctrl Pts',(-18.5479551287003,34.1818824728114,122.567652773556)) ;
#94078=CARTESIAN_POINT('Ctrl Pts',(-18.7084701859392,34.1919304048901,122.430380021291)) ;
#94079=CARTESIAN_POINT('Ctrl Pts',(-18.8872472220811,34.2018077806995,122.324675785591)) ;
#94080=CARTESIAN_POINT('Ctrl Pts',(-19.0850314864428,34.2118616738674,122.250237672845)) ;
#94081=CARTESIAN_POINT('Ctrl Pts',(-19.2894839484304,34.2217552971207,122.211783907528)) ;
#94082=CARTESIAN_POINT('Ctrl Pts',(-19.500983623054,34.2318178907437,122.209341438125)) ;
#94083=CARTESIAN_POINT('Ctrl Pts',(-19.7052052740949,34.2416604647328,122.242811570821)) ;
#94084=CARTESIAN_POINT('Ctrl Pts',(-19.9035702084726,34.2516512216157,122.311773010739)) ;
#94085=CARTESIAN_POINT('Ctrl Pts',(-20.0858114345933,34.2615792833737,122.413537168771)) ;
#94086=CARTESIAN_POINT('Ctrl Pts',(-20.2488208114656,34.2715672592628,122.545909741737)) ;
#94087=CARTESIAN_POINT('Ctrl Pts',(-20.3867503154781,34.2816029236193,122.705552972762)) ;
#94088=CARTESIAN_POINT('Ctrl Pts',(-20.4932169372038,34.2914588620389,122.883323157237)) ;
#94089=CARTESIAN_POINT('Ctrl Pts',(-20.5685573075516,34.3014543534358,123.079465833174)) ;
#94090=CARTESIAN_POINT('Ctrl Pts',(-20.6084203311563,34.3113641583893,123.283961980646)) ;
#94091=CARTESIAN_POINT('Ctrl Pts',(-20.612551191493,34.321376380656,123.494414775506)) ;
#94092=CARTESIAN_POINT('Ctrl Pts',(-20.5796204265789,34.3314042613489,123.70264639722)) ;
#94093=CARTESIAN_POINT('Ctrl Pts',(-20.5125423192558,34.3412606573315,123.898699495706)) ;
#94094=CARTESIAN_POINT('Ctrl Pts',(-20.4111153088233,34.3512854545114,124.083444098484)) ;
#94095=CARTESIAN_POINT('Ctrl Pts',(-20.2786642846804,34.3613163844952,124.247549916826)) ;
#94096=CARTESIAN_POINT('Ctrl Pts',(-20.12294110075,34.3711609870039,124.383860206377)) ;
#94097=CARTESIAN_POINT('Ctrl Pts',(-19.9435694725039,34.381151838228,124.493149976291)) ;
#94098=CARTESIAN_POINT('Ctrl Pts',(-19.7468604255009,34.3911896712392,124.569551549301)) ;
#94099=CARTESIAN_POINT('Ctrl Pts',(-19.5439244481446,34.4010340597047,124.610202431211)) ;
#94100=CARTESIAN_POINT('Ctrl Pts',(-19.334106769113,34.4110188640742,124.615482055725)) ;
#94101=CARTESIAN_POINT('Ctrl Pts',(-19.1274314473435,34.4209583835571,124.58447308908)) ;
#94102=CARTESIAN_POINT('Ctrl Pts',(-18.9273406435302,34.4309981145584,124.51734707445)) ;
#94103=CARTESIAN_POINT('Ctrl Pts',(-18.7446690953426,34.4408862428047,124.418099734678)) ;
#94104=CARTESIAN_POINT('Ctrl Pts',(-18.580106238274,34.4508759680132,124.287630599597)) ;
#94105=CARTESIAN_POINT('Ctrl Pts',(-18.4412525947142,34.4608337327147,124.130968239248)) ;
#94106=CARTESIAN_POINT('Ctrl Pts',(-18.3318983126126,34.4707360741267,123.953816562447)) ;
#94107=CARTESIAN_POINT('Ctrl Pts',(-18.2538875112348,34.4807802698331,123.757605424471)) ;
#94108=CARTESIAN_POINT('Ctrl Pts',(-18.2116860626356,34.4906876705924,123.553629701475)) ;
#94109=CARTESIAN_POINT('Ctrl Pts',(-18.2051086171753,34.5006982704667,123.343275079587)) ;
#94110=CARTESIAN_POINT('Ctrl Pts',(-18.235618607737,34.5107285663789,123.134619214814)) ;
#94111=CARTESIAN_POINT('Ctrl Pts',(-18.3004560701024,34.5205833460286,122.937861271904)) ;
#94112=CARTESIAN_POINT('Ctrl Pts',(-18.3989387244169,34.5305406742461,122.753132054691)) ;
#94113=CARTESIAN_POINT('Ctrl Pts',(-18.529340384314,34.540579707153,122.587203293824)) ;
#94114=CARTESIAN_POINT('Ctrl Pts',(-18.6837505633702,34.5504528190423,122.448444472105)) ;
#94115=CARTESIAN_POINT('Ctrl Pts',(-18.8634484664736,34.5605261040694,122.336472032955)) ;
#94116=CARTESIAN_POINT('Ctrl Pts',(-19.0549065955958,34.5703464238062,122.259103635501)) ;
#94117=CARTESIAN_POINT('Ctrl Pts',(-19.2620673866874,34.5804250891846,122.214853277882)) ;
#94118=CARTESIAN_POINT('Ctrl Pts',(-19.4690914175572,34.5902766796684,122.207340232116)) ;
#94119=CARTESIAN_POINT('Ctrl Pts',(-19.6788278083087,34.6003498299873,122.23633458092)) ;
#94120=CARTESIAN_POINT('Ctrl Pts',(-19.8757732790517,34.6101922099624,122.299862332221)) ;
#94121=CARTESIAN_POINT('Ctrl Pts',(-20.0615624570117,34.6201731862054,122.39735650265)) ;
#94122=CARTESIAN_POINT('Ctrl Pts',(-20.22799325484,34.6301895145607,122.526380463607)) ;
#94123=CARTESIAN_POINT('Ctrl Pts',(-20.3680014912739,34.6400873115519,122.680305163105)) ;
#94124=CARTESIAN_POINT('Ctrl Pts',(-20.4807624680601,34.6500998682839,122.858068591646)) ;
#94125=CARTESIAN_POINT('Ctrl Pts',(-20.5606293910211,34.6601319031304,123.053255712585)) ;
#94126=CARTESIAN_POINT('Ctrl Pts',(-20.6050415862944,34.6699713039459,123.255303457443)) ;
#94127=CARTESIAN_POINT('Ctrl Pts',(-20.6140547312464,34.6800370895974,123.466701640251)) ;
#94128=CARTESIAN_POINT('Ctrl Pts',(-20.5866072640144,34.689927544712,123.672832323993)) ;
#94129=CARTESIAN_POINT('Ctrl Pts',(-20.5235800847125,34.6999196633478,123.873208878292)) ;
#94130=CARTESIAN_POINT('Ctrl Pts',(-20.4268258454947,34.7098824901109,124.05896578674)) ;
#94131=CARTESIAN_POINT('Ctrl Pts',(-20.3004423413682,34.7197867733837,124.224463799547)) ;
#94132=CARTESIAN_POINT('Ctrl Pts',(-20.1447352025341,34.7298472073308,124.367564111217)) ;
#94133=CARTESIAN_POINT('Ctrl Pts',(-19.9705405095534,34.739687760004,124.479217029164)) ;
#94134=CARTESIAN_POINT('Ctrl Pts',(-19.7754543274216,34.7497499799497,124.560953476253)) ;
#94135=CARTESIAN_POINT('Ctrl Pts',(-19.5724445177316,34.7596471192283,124.606605437042)) ;
#94136=CARTESIAN_POINT('Ctrl Pts',(-19.3639246090716,34.7695783113634,124.617042218712)) ;
#94137=CARTESIAN_POINT('Ctrl Pts',(-19.1544758574248,34.7796204660084,124.590591195082)) ;
#94138=CARTESIAN_POINT('Ctrl Pts',(-18.9558505145138,34.7895072270277,124.529297402871)) ;
#94139=CARTESIAN_POINT('Ctrl Pts',(-18.7686968083178,34.799506528745,124.433626692028)) ;
#94140=CARTESIAN_POINT('Ctrl Pts',(-18.6021840247918,34.8094273269117,124.307986921244)) ;
#94141=CARTESIAN_POINT('Ctrl Pts',(-18.4584119572292,34.8194613805084,124.153654294584)) ;
#94142=CARTESIAN_POINT('Ctrl Pts',(-18.3447544148885,34.8293844980748,123.978681451143)) ;
#94143=CARTESIAN_POINT('Ctrl Pts',(-18.2621745210567,34.839440621574,123.784088516026)) ;
#94144=CARTESIAN_POINT('Ctrl Pts',(-18.2155383722637,34.8492860632288,123.582420343788)) ;
#94145=CARTESIAN_POINT('Ctrl Pts',(-18.2038107378069,34.8592483643529,123.373323368424)) ;
#94146=CARTESIAN_POINT('Ctrl Pts',(-18.2290111919867,34.8692768436281,123.163990289439)) ;
#94147=CARTESIAN_POINT('Ctrl Pts',(-18.2893801467277,34.8791871971377,122.964592206024)) ;
#94148=CARTESIAN_POINT('Ctrl Pts',(-18.3832066359481,34.8891220693149,122.777983967689)) ;
#94149=CARTESIAN_POINT('Ctrl Pts',(-18.5094937411179,34.8991632069006,122.608837933746)) ;
#94150=CARTESIAN_POINT('Ctrl Pts',(-18.6607872390357,34.9090503561152,122.466288539234)) ;
#94151=CARTESIAN_POINT('Ctrl Pts',(-18.8361659801269,34.9190425908663,122.350681679079)) ;
#94152=CARTESIAN_POINT('Ctrl Pts',(-19.0281614277122,34.9289912964292,122.267692173335)) ;
#94153=CARTESIAN_POINT('Ctrl Pts',(-19.2312959474012,34.9389273648529,122.219071222119)) ;
#94154=CARTESIAN_POINT('Ctrl Pts',(-19.4408495024323,34.9489130490687,122.206154757217)) ;
#94155=CARTESIAN_POINT('Ctrl Pts',(-19.6505366751232,34.9589534756374,122.230278766843)) ;
#94156=CARTESIAN_POINT('Ctrl Pts',(-19.8489056304027,34.9687925891011,122.288911017026)) ;
#94157=CARTESIAN_POINT('Ctrl Pts',(-20.0378790588203,34.9788223232769,122.382455859527)) ;
#94158=CARTESIAN_POINT('Ctrl Pts',(-20.2072811356501,34.9888444227828,122.507735639608)) ;
#94159=CARTESIAN_POINT('Ctrl Pts',(-20.3505219569194,34.9987128626763,122.657836929404)) ;
#94160=CARTESIAN_POINT('Ctrl Pts',(-20.4678365377331,35.0087817273619,122.834011313283)) ;
#94161=CARTESIAN_POINT('Ctrl Pts',(-20.5508879058607,35.0186244004605,123.023544378056)) ;
#94162=CARTESIAN_POINT('Ctrl Pts',(-20.6010962673067,35.0285850346229,123.226835516513)) ;
#94163=CARTESIAN_POINT('Ctrl Pts',(-20.6149388907068,35.0386229503011,123.437402293427)) ;
#94164=CARTESIAN_POINT('Ctrl Pts',(-20.5927617556655,35.0484972251605,123.64382806409)) ;
#94165=CARTESIAN_POINT('Ctrl Pts',(-20.533940744717,35.0585669755356,123.847160626017)) ;
#94166=CARTESIAN_POINT('Ctrl Pts',(-20.4429777659414,35.0684002709101,124.032817622277)) ;
#94167=CARTESIAN_POINT('Ctrl Pts',(-20.3192176608534,35.0784305683898,124.203541018578)) ;
#94168=CARTESIAN_POINT('Ctrl Pts',(-20.167224581628,35.0884626548312,124.349771836117)) ;
#94169=CARTESIAN_POINT('Ctrl Pts',(-19.995982217517,35.0982905833201,124.465363727968)) ;
#94170=CARTESIAN_POINT('Ctrl Pts',(-19.8042655773191,35.1082866244309,124.551422942232)) ;
#94171=CARTESIAN_POINT('Ctrl Pts',(-19.5998043362001,35.1183124365321,124.602646562785)) ;
#94172=CARTESIAN_POINT('Ctrl Pts',(-19.392483135136,35.1281996714269,124.61765284484)) ;
#94173=CARTESIAN_POINT('Ctrl Pts',(-19.1838143214605,35.138176537638,124.596588861163)) ;
#94174=CARTESIAN_POINT('Ctrl Pts',(-18.9815944355793,35.1481694815098,124.539544123873)) ;
#94175=CARTESIAN_POINT('Ctrl Pts',(-18.7916564364344,35.1582074041811,124.447621099837)) ;
#94176=CARTESIAN_POINT('Ctrl Pts',(-18.6235856865479,35.1680558684428,124.326680955003)) ;
#94177=CARTESIAN_POINT('Ctrl Pts',(-18.4767269403657,35.1780477351868,124.176530858899)) ;
#94178=CARTESIAN_POINT('Ctrl Pts',(-18.3589196063816,35.187965467228,124.004467621855)) ;
#94179=CARTESIAN_POINT('Ctrl Pts',(-18.2717855263324,35.1979936521233,123.81251148209)) ;
#94180=CARTESIAN_POINT('Ctrl Pts',(-18.2199640334134,35.2078788101721,123.611253905476)) ;
#94181=CARTESIAN_POINT('Ctrl Pts',(-18.2031956371847,35.2178681707138,123.401912409714)) ;
#94182=CARTESIAN_POINT('Ctrl Pts',(-18.2235772720183,35.2279093276482,123.191802025504)) ;
#94183=CARTESIAN_POINT('Ctrl Pts',(-18.2786256484142,35.2377419111033,122.992558402953)) ;
#94184=CARTESIAN_POINT('Ctrl Pts',(-18.368354396515,35.2477361310653,122.802574696056)) ;
#94185=CARTESIAN_POINT('Ctrl Pts',(-18.4904752618844,35.2577642328526,122.630717578869)) ;
#94186=CARTESIAN_POINT('Ctrl Pts',(-18.6381538690012,35.2676441774757,122.484653314994)) ;
#94187=CARTESIAN_POINT('Ctrl Pts',(-18.810661504175,35.2776345040327,122.364871614765)) ;
#94188=CARTESIAN_POINT('Ctrl Pts',(-19.0004190147032,35.287575435687,122.277289202281)) ;
#94189=CARTESIAN_POINT('Ctrl Pts',(-19.2033735677859,35.2975625541899,122.223445030743)) ;
#94190=CARTESIAN_POINT('Ctrl Pts',(-19.4135608790343,35.3075958870871,122.205909966767)) ;
#94191=CARTESIAN_POINT('Ctrl Pts',(-19.6201740321461,35.3174619915319,122.224414931314)) ;
#94192=CARTESIAN_POINT('Ctrl Pts',(-19.8244618434658,35.3275281054122,122.279549956183)) ;
#94193=CARTESIAN_POINT('Ctrl Pts',(-20.0121134275938,35.3373841171806,122.367450475576)) ;
#94194=CARTESIAN_POINT('Ctrl Pts',(-20.1843772800445,35.3473788208119,122.487755297153)) ;
#94195=CARTESIAN_POINT('Ctrl Pts',(-20.3333683555164,35.3574101565368,122.637013322784)) ;
#94196=CARTESIAN_POINT('Ctrl Pts',(-20.452467682773,35.3672766817405,122.806847362227)) ;
#94197=CARTESIAN_POINT('Ctrl Pts',(-20.5416380634157,35.3772641097863,122.996911545237)) ;
#94198=CARTESIAN_POINT('Ctrl Pts',(-20.5963428038988,35.3872090394727,123.19873346646)) ;
#94199=CARTESIAN_POINT('Ctrl Pts',(-20.6152390421331,35.3972539575812,123.409042039138)) ;
#94200=CARTESIAN_POINT('Ctrl Pts',(-20.5978399936746,35.4071159271951,123.615657183607)) ;
#94201=CARTESIAN_POINT('Ctrl Pts',(-20.544536085097,35.4171079952163,123.818824897124)) ;
#94202=CARTESIAN_POINT('Ctrl Pts',(-20.4572545241193,35.4270389205909,124.008498798573)) ;
#94203=CARTESIAN_POINT('Ctrl Pts',(-20.3384335703723,35.4369895488143,124.180653521946)) ;
#94204=CARTESIAN_POINT('Ctrl Pts',(-20.1908529589591,35.4469897878734,124.33041662932)) ;
#94205=CARTESIAN_POINT('Ctrl Pts',(-20.0188759708664,35.4570182432426,124.452357639647)) ;
#94206=CARTESIAN_POINT('Ctrl Pts',(-19.8315424534969,35.4668842778259,124.541414633258)) ;
#94207=CARTESIAN_POINT('Ctrl Pts',(-19.6291530073058,35.4768765995733,124.597623086158)) ;
#94208=CARTESIAN_POINT('Ctrl Pts',(-19.4213004974954,35.4868088892503,124.617752074069)) ;
#94209=CARTESIAN_POINT('Ctrl Pts',(-19.2116664499479,35.4968105342211,124.601578995507)) ;
#94210=CARTESIAN_POINT('Ctrl Pts',(-18.9405974517021,35.5101231676371,124.53180213647)) ;
#94211=CARTESIAN_POINT('Ctrl Pts',(-18.6953540228748,35.5233549170187,124.393908226192)) ;
#94212=CARTESIAN_POINT('Ctrl Pts',(-18.4950059156847,35.5366781818358,124.198224853695)) ;
#94213=CARTESIAN_POINT('Ctrl Pts',(-18.3736553940196,35.5465538880534,124.029742286232)) ;
#94214=CARTESIAN_POINT('Ctrl Pts',(-18.2821355436399,35.5565434791535,123.840747243636)) ;
#94215=CARTESIAN_POINT('Ctrl Pts',(-18.2250326582066,35.5664705756089,123.639986013485)) ;
#94216=CARTESIAN_POINT('Ctrl Pts',(-18.2034246479505,35.5764957241134,123.430355343543)) ;
#94217=CARTESIAN_POINT('Ctrl Pts',(-18.2182221832867,35.5863913782601,123.222826157615)) ;
#94218=CARTESIAN_POINT('Ctrl Pts',(-18.2690819887798,35.5963949126383,123.018783641525)) ;
#94219=CARTESIAN_POINT('Ctrl Pts',(-18.3544809937856,35.6063800510784,122.826985667331)) ;
#94220=CARTESIAN_POINT('Ctrl Pts',(-18.472633727841,35.6164159756738,122.652198283196)) ;
#94221=CARTESIAN_POINT('Ctrl Pts',(-18.6164712344706,35.6262672511014,122.503192800069)) ;
#94222=CARTESIAN_POINT('Ctrl Pts',(-18.7860470108393,35.6362595122628,122.379193128309)) ;
#94223=CARTESIAN_POINT('Ctrl Pts',(-18.9756946767603,35.6462993962804,122.286567038597)) ;
#94224=CARTESIAN_POINT('Ctrl Pts',(-19.1742898648837,35.6561341707828,122.228953637349)) ;
#94225=CARTESIAN_POINT('Ctrl Pts',(-19.384854864519,35.6662105518031,122.206080561557)) ;
#94226=CARTESIAN_POINT('Ctrl Pts',(-19.5914292540954,35.6760568249538,122.21974207516)) ;
#94227=CARTESIAN_POINT('Ctrl Pts',(-19.8644346438615,35.689421346239,122.28616654284)) ;
#94228=CARTESIAN_POINT('Ctrl Pts',(-20.1107389994271,35.7026275906734,122.421071166414)) ;
#94229=CARTESIAN_POINT('Ctrl Pts',(-20.31289569483,35.7158925453506,122.613085924931)) ;
#94230=CARTESIAN_POINT('Ctrl Pts',(-20.4382108480598,35.7259248259023,122.782748300882)) ;
#94231=CARTESIAN_POINT('Ctrl Pts',(-20.5310088705917,35.7358335594202,122.969242542732)) ;
#94232=CARTESIAN_POINT('Ctrl Pts',(-20.5907141773858,35.7457711102877,123.169457067613)) ;
#94233=CARTESIAN_POINT('Ctrl Pts',(-20.6147942179348,35.7558009578817,123.378913702247)) ;
#94234=CARTESIAN_POINT('Ctrl Pts',(-20.598471691995,35.7690360978021,123.656761562465)) ;
#94235=CARTESIAN_POINT('Ctrl Pts',(-20.4868792880066,35.7857045621733,123.993019501835)) ;
#94236=CARTESIAN_POINT('Ctrl Pts',(-20.2251471753778,35.8055755740472,124.324870618107)) ;
#94237=CARTESIAN_POINT('Ctrl Pts',(-19.9231598977756,35.8222826584301,124.511857504342)) ;
#94238=CARTESIAN_POINT('Ctrl Pts',(-19.6579097068022,35.8354599397407,124.591780242991)) ;
#94239=CARTESIAN_POINT('Ctrl Pts',(-19.3810458831154,35.8487274002548,124.625650252468)) ;
#94240=CARTESIAN_POINT('Ctrl Pts',(-19.0312456986032,35.865341290942,124.576426819404)) ;
#94241=CARTESIAN_POINT('Ctrl Pts',(-18.6565465864892,35.8852900903694,124.377542753024)) ;
#94242=CARTESIAN_POINT('Ctrl Pts',(-18.3727285742286,35.9052112019003,124.063195064491)) ;
#94243=CARTESIAN_POINT('Ctrl Pts',(-18.2127928629799,35.9250776500732,123.672157267493)) ;
#94244=CARTESIAN_POINT('Ctrl Pts',(-18.1960231038597,35.9451039966903,123.246720272053)) ;
#94245=CARTESIAN_POINT('Ctrl Pts',(-18.324491777266,35.9649660410798,122.844336458212)) ;
#94246=CARTESIAN_POINT('Ctrl Pts',(-18.5830322138588,35.984911343761,122.508241861677)) ;
#94247=CARTESIAN_POINT('Ctrl Pts',(-18.9399428040037,36.0048066508198,122.281138146652)) ;
#94248=CARTESIAN_POINT('Ctrl Pts',(-19.3527184258083,36.0246999209875,122.188728146812)) ;
#94249=CARTESIAN_POINT('Ctrl Pts',(-19.7737311453565,36.0446655136679,122.243004299579)) ;
#94250=CARTESIAN_POINT('Ctrl Pts',(-20.1494256886425,36.0645408373527,122.436571014083)) ;
#94251=CARTESIAN_POINT('Ctrl Pts',(-20.4382670267908,36.0845158999277,122.747982676867)) ;
#94252=CARTESIAN_POINT('Ctrl Pts',(-20.6027131365231,36.1044683095588,123.13905599893)) ;
#94253=CARTESIAN_POINT('Ctrl Pts',(-20.6245287238263,36.1243043637949,123.560259112784)) ;
#94254=CARTESIAN_POINT('Ctrl Pts',(-20.5008694097332,36.1442822752124,123.966645271116)) ;
#94255=CARTESIAN_POINT('Ctrl Pts',(-20.2463345181827,36.1642003247159,124.305097725016)) ;
#94256=CARTESIAN_POINT('Ctrl Pts',(-19.8929821410224,36.184068468484,124.536788661941)) ;
#94257=CARTESIAN_POINT('Ctrl Pts',(-19.4780341435189,36.2041193250713,124.634204632469)) ;
#94258=CARTESIAN_POINT('Ctrl Pts',(-19.060185282991,36.2238997615272,124.585267869156)) ;
#94259=CARTESIAN_POINT('Ctrl Pts',(-18.6792614121707,36.243929817205,124.39500532448)) ;
#94260=CARTESIAN_POINT('Ctrl Pts',(-18.3887179287721,36.2638109223798,124.087851926812)) ;
#94261=CARTESIAN_POINT('Ctrl Pts',(-18.2193877315781,36.2836913847476,123.700582700507)) ;
#94262=CARTESIAN_POINT('Ctrl Pts',(-18.1923469123526,36.303676531892,123.276491971302)) ;
#94263=CARTESIAN_POINT('Ctrl Pts',(-18.3111820591187,36.3235671104283,122.870593111507)) ;
#94264=CARTESIAN_POINT('Ctrl Pts',(-18.5608265214419,36.3434611303027,122.529122738286)) ;
#94265=CARTESIAN_POINT('Ctrl Pts',(-18.9123819811256,36.3633825750291,122.292957365866)) ;
#94266=CARTESIAN_POINT('Ctrl Pts',(-19.3229431016927,36.3832807130846,122.190279954938)) ;
#94267=CARTESIAN_POINT('Ctrl Pts',(-19.7472712121546,36.4033514683006,122.235041107038)) ;
#94268=CARTESIAN_POINT('Ctrl Pts',(-20.1256425048648,36.4231370183519,122.419154459229)) ;
#94269=CARTESIAN_POINT('Ctrl Pts',(-20.4220170919712,36.4431200932292,122.723507834447)) ;
#94270=CARTESIAN_POINT('Ctrl Pts',(-20.5955265060614,36.4630291758752,123.109641805405)) ;
#94271=CARTESIAN_POINT('Ctrl Pts',(-20.6279926946846,36.4828877349979,123.530692392537)) ;
#94272=CARTESIAN_POINT('Ctrl Pts',(-20.5133248607848,36.5029311788366,123.941072248336)) ;
#94273=CARTESIAN_POINT('Ctrl Pts',(-20.3093892008094,36.5194312435658,124.226640164465)) ;
#94274=CARTESIAN_POINT('Ctrl Pts',(-20.0922743624117,36.5328209834147,124.405775190964)) ;
#94275=CARTESIAN_POINT('Ctrl Pts',(-19.9119758940525,36.5426778846231,124.50796979735)) ;
#94276=CARTESIAN_POINT('Ctrl Pts',(-19.7142026000164,36.5526694104696,124.578640998708)) ;
#94277=CARTESIAN_POINT('Ctrl Pts',(-19.5084996701913,36.5625940909206,124.613748998774)) ;
#94278=CARTESIAN_POINT('Ctrl Pts',(-19.2980711955176,36.572604680965,124.612675114737)) ;
#94279=CARTESIAN_POINT('Ctrl Pts',(-19.0237189426049,36.5858639416687,124.563191698684)) ;
#94280=CARTESIAN_POINT('Ctrl Pts',(-18.7670047191078,36.5992150168189,124.442157992016)) ;
#94281=CARTESIAN_POINT('Ctrl Pts',(-18.5548978247711,36.6124213260537,124.262901583435)) ;
#94282=CARTESIAN_POINT('Ctrl Pts',(-18.4202072442688,36.622408159644,124.101894853874)) ;
#94283=CARTESIAN_POINT('Ctrl Pts',(-18.315747816348,36.6323608871401,123.92055502923)) ;
#94284=CARTESIAN_POINT('Ctrl Pts',(-18.2438653268003,36.6424089839817,123.721943551495)) ;
#94285=CARTESIAN_POINT('Ctrl Pts',(-18.2080589031175,36.6522504408535,123.518146535911)) ;
#94286=CARTESIAN_POINT('Ctrl Pts',(-18.2077355281506,36.662236707767,123.3082383145)) ;
#94287=CARTESIAN_POINT('Ctrl Pts',(-18.2435931093309,36.6721733086674,123.102404801807)) ;
#94288=CARTESIAN_POINT('Ctrl Pts',(-18.3155367278071,36.6822232514545,122.903771931115)) ;
#94289=CARTESIAN_POINT('Ctrl Pts',(-18.4186658169043,36.6920734511402,122.724179668782)) ;
#94290=CARTESIAN_POINT('Ctrl Pts',(-18.5526159505733,36.7020463560723,122.562916709314)) ;
#94291=CARTESIAN_POINT('Ctrl Pts',(-18.7130217748443,36.712044730552,122.427034994894)) ;
#94292=CARTESIAN_POINT('Ctrl Pts',(-18.8950290521288,36.7220649044219,122.320985373851)) ;
#94293=CARTESIAN_POINT('Ctrl Pts',(-19.0902841742662,36.7319659483639,122.248841931777)) ;
#94294=CARTESIAN_POINT('Ctrl Pts',(-19.2968494423397,36.7419547520882,122.211043582712)) ;
#94295=CARTESIAN_POINT('Ctrl Pts',(-19.5063417767204,36.7519202189201,122.209838370568)) ;
#94296=CARTESIAN_POINT('Ctrl Pts',(-19.7116920199838,36.761823781193,122.244315917006)) ;
#94297=CARTESIAN_POINT('Ctrl Pts',(-19.9109467915122,36.771884459071,122.315177857541)) ;
#94298=CARTESIAN_POINT('Ctrl Pts',(-20.0910226160667,36.7817247570205,122.417070031681)) ;
#94299=CARTESIAN_POINT('Ctrl Pts',(-20.2544023838609,36.7917877519299,122.551425204695)) ;
#94300=CARTESIAN_POINT('Ctrl Pts',(-20.3895668613944,36.8016820460771,122.709563463652)) ;
#94301=CARTESIAN_POINT('Ctrl Pts',(-20.4961913136118,36.8116238437739,122.889298746272)) ;
#94302=CARTESIAN_POINT('Ctrl Pts',(-20.5705305835063,36.821626421303,123.086035728919)) ;
#94303=CARTESIAN_POINT('Ctrl Pts',(-20.6093785768272,36.8316608852241,123.293373251743)) ;
#94304=CARTESIAN_POINT('Ctrl Pts',(-20.6119178337736,36.8415070237452,123.500360827497)) ;
#94305=CARTESIAN_POINT('Ctrl Pts',(-20.5784854232737,36.8514881969822,123.707499070501)) ;
#94306=CARTESIAN_POINT('Ctrl Pts',(-20.5097396908624,36.8614404909394,123.905117972074)) ;
#94307=CARTESIAN_POINT('Ctrl Pts',(-20.407482017507,36.871439286074,124.088793923392)) ;
#94308=CARTESIAN_POINT('Ctrl Pts',(-20.2740542798669,36.8814783943348,124.252304034423)) ;
#94309=CARTESIAN_POINT('Ctrl Pts',(-20.1179432190855,36.891303335774,124.387573713535)) ;
#94310=CARTESIAN_POINT('Ctrl Pts',(-19.9367725759517,36.9013580228484,124.496449032076)) ;
#94311=CARTESIAN_POINT('Ctrl Pts',(-19.7414996675405,36.9113008277885,124.571043200714)) ;
#94312=CARTESIAN_POINT('Ctrl Pts',(-19.5371698887816,36.921204613785,124.611070181007)) ;
#94313=CARTESIAN_POINT('Ctrl Pts',(-19.3260077881404,36.9312514303498,124.614939096116)) ;
#94314=CARTESIAN_POINT('Ctrl Pts',(-19.1204430965301,36.9411469498285,124.582756712928)) ;
#94315=CARTESIAN_POINT('Ctrl Pts',(-18.9203358370429,36.951209035153,124.51425755505)) ;
#94316=CARTESIAN_POINT('Ctrl Pts',(-18.7390960653192,36.9610517461109,124.414360045597)) ;
#94317=CARTESIAN_POINT('Ctrl Pts',(-18.5752583735253,36.9710424634169,124.282977394768)) ;
#94318=CARTESIAN_POINT('Ctrl Pts',(-18.4375935817298,36.9809705465135,124.126081575226)) ;
#94319=CARTESIAN_POINT('Ctrl Pts',(-18.3282968902032,36.9909584766253,123.946781567266)) ;
#94320=CARTESIAN_POINT('Ctrl Pts',(-18.2517622222027,37.0009943027526,123.750174853186)) ;
#94321=CARTESIAN_POINT('Ctrl Pts',(-18.21094080092,37.0108496398662,123.547034402322)) ;
#94322=CARTESIAN_POINT('Ctrl Pts',(-18.2056086306045,37.0208473747163,123.336940861703)) ;
#94323=CARTESIAN_POINT('Ctrl Pts',(-18.2364910695432,37.0307552787008,123.130938239226)) ;
#94324=CARTESIAN_POINT('Ctrl Pts',(-18.3030269286301,37.0407663532492,122.931261335082)) ;
#94325=CARTESIAN_POINT('Ctrl Pts',(-18.4037673321845,37.0507942087849,122.746069536931)) ;
#94326=CARTESIAN_POINT('Ctrl Pts',(-18.5326081036751,37.0606518026901,122.583754403293)) ;
#94327=CARTESIAN_POINT('Ctrl Pts',(-18.6900546143818,37.0706784895282,122.443591540943)) ;
#94328=CARTESIAN_POINT('Ctrl Pts',(-18.8697606942828,37.0807071586819,122.3333196009)) ;
#94329=CARTESIAN_POINT('Ctrl Pts',(-19.0621377136588,37.0905523669633,122.256989628151)) ;
#94330=CARTESIAN_POINT('Ctrl Pts',(-19.2677422078546,37.1005430559265,122.214048078359)) ;
#94331=CARTESIAN_POINT('Ctrl Pts',(-19.47867850993,37.1105809322087,122.207898021882)) ;
#94332=CARTESIAN_POINT('Ctrl Pts',(-19.6835147698545,37.120425309851,122.23752146593)) ;
#94333=CARTESIAN_POINT('Ctrl Pts',(-19.882996079095,37.1304101142424,122.302778957761)) ;
#94334=CARTESIAN_POINT('Ctrl Pts',(-20.067369358765,37.1403496444609,122.401180186944)) ;
#94335=CARTESIAN_POINT('Ctrl Pts',(-20.2334482035673,37.1503893324978,122.531409803417)) ;
#94336=CARTESIAN_POINT('Ctrl Pts',(-20.3723615313859,37.1602776218661,122.686081213826)) ;
#94337=CARTESIAN_POINT('Ctrl Pts',(-20.4837564475809,37.1702667455509,122.864096057991)) ;
#94338=CARTESIAN_POINT('Ctrl Pts',(-20.5621702859723,37.1802267552255,123.0582461287)) ;
#94339=CARTESIAN_POINT('Ctrl Pts',(-20.6059089775534,37.1901271849298,123.26174306091)) ;
#94340=CARTESIAN_POINT('Ctrl Pts',(-20.6137506161671,37.2001702663365,123.472725765684)) ;
#94341=CARTESIAN_POINT('Ctrl Pts',(-20.5852316490187,37.2100776602442,123.679059652411)) ;
#94342=CARTESIAN_POINT('Ctrl Pts',(-20.5210198031363,37.2200893912333,123.879505634922)) ;
#94343=CARTESIAN_POINT('Ctrl Pts',(-20.4224065161209,37.2301216089481,124.065948284503)) ;
#94344=CARTESIAN_POINT('Ctrl Pts',(-20.2954706478781,37.2399741181943,124.229610475779)) ;
#94345=CARTESIAN_POINT('Ctrl Pts',(-20.1408283407611,37.2499320547373,124.370729348929)) ;
#94346=CARTESIAN_POINT('Ctrl Pts',(-19.9624090787008,37.2599709247456,124.483433619568)) ;
#94347=CARTESIAN_POINT('Ctrl Pts',(-19.770458867892,37.2698440799038,124.562502735803)) ;
#94348=CARTESIAN_POINT('Ctrl Pts',(-19.563646481703,37.2799173547535,124.607865009529)) ;
#94349=CARTESIAN_POINT('Ctrl Pts',(-19.3573352708199,37.2897376719309,124.616683319758)) ;
#94350=CARTESIAN_POINT('Ctrl Pts',(-19.1473126860865,37.2998163577244,124.589037296444)) ;
#94351=CARTESIAN_POINT('Ctrl Pts',(-18.9497170318197,37.3096678691075,124.526820893084)) ;
#94352=CARTESIAN_POINT('Ctrl Pts',(-18.7617822357577,37.3197413154142,124.42928813137)) ;
#94353=CARTESIAN_POINT('Ctrl Pts',(-18.597472760088,37.3295825905389,124.303521853965)) ;
#94354=CARTESIAN_POINT('Ctrl Pts',(-18.4549977478559,37.3395676901956,124.14938498897)) ;
#94355=CARTESIAN_POINT('Ctrl Pts',(-18.3414230173114,37.3495751663299,123.972266878599)) ;
#94356=CARTESIAN_POINT('Ctrl Pts',(-18.2608487024426,37.3594977540389,123.779863642835)) ;
#94357=CARTESIAN_POINT('Ctrl Pts',(-18.2142702336131,37.3694843583122,123.575125917761)) ;
#94358=CARTESIAN_POINT('Ctrl Pts',(-18.2042901750797,37.3795244866463,123.364303702255)) ;
#94359=CARTESIAN_POINT('Ctrl Pts',(-18.230089300167,37.3893639211797,123.159042239126)) ;
#94360=CARTESIAN_POINT('Ctrl Pts',(-18.292348591222,37.3994279756707,122.956858629565)) ;
#94361=CARTESIAN_POINT('Ctrl Pts',(-18.3872136846563,37.4093188949079,122.77179662496)) ;
#94362=CARTESIAN_POINT('Ctrl Pts',(-18.5136767800856,37.4193108882139,122.604078934525)) ;
#94363=CARTESIAN_POINT('Ctrl Pts',(-18.6670285892271,37.4292737521732,122.461423780996)) ;
#94364=CARTESIAN_POINT('Ctrl Pts',(-18.8415186482353,37.439178011991,122.34777734917)) ;
#94365=CARTESIAN_POINT('Ctrl Pts',(-19.0361446502019,37.4492385025624,122.265052864531)) ;
#94366=CARTESIAN_POINT('Ctrl Pts',(-19.2376613352379,37.4590788521934,122.218146467935)) ;
#94367=CARTESIAN_POINT('Ctrl Pts',(-19.4488650147915,37.4691418276835,122.206437417777)) ;
#94368=CARTESIAN_POINT('Ctrl Pts',(-19.655401912625,37.4790361478268,122.231332710315)) ;
#94369=CARTESIAN_POINT('Ctrl Pts',(-19.8555475304082,37.4889778609584,122.291445911466)) ;
#94370=CARTESIAN_POINT('Ctrl Pts',(-20.0434590938242,37.4989807507526,122.385921675626)) ;
#94371=CARTESIAN_POINT('Ctrl Pts',(-20.2124620638897,37.509020607913,122.512333007315)) ;
#94372=CARTESIAN_POINT('Ctrl Pts',(-20.3542123192198,37.5188447887507,122.662567186041)) ;
#94373=CARTESIAN_POINT('Ctrl Pts',(-20.4706388940175,37.5289017622539,122.839032422264)) ;
#94374=CARTESIAN_POINT('Ctrl Pts',(-20.5533481377994,37.5388298864409,123.030678499673)) ;
#94375=CARTESIAN_POINT('Ctrl Pts',(-20.6021910243834,37.5487835815143,123.234157885621)) ;
#94376=CARTESIAN_POINT('Ctrl Pts',(-20.6147789290021,37.5588297750896,123.444983226702)) ;
#94377=CARTESIAN_POINT('Ctrl Pts',(-20.5912446307406,37.5686778774495,123.650677843784)) ;
#94378=CARTESIAN_POINT('Ctrl Pts',(-20.5322977294256,37.5786394656771,123.851625109879)) ;
#94379=CARTESIAN_POINT('Ctrl Pts',(-20.4384823229094,37.5886681358334,124.040450631407)) ;
#94380=CARTESIAN_POINT('Ctrl Pts',(-20.3148504709201,37.5985784387151,124.208137758696)) ;
#94381=CARTESIAN_POINT('Ctrl Pts',(-20.1639729630822,37.608513322523,124.352574750252)) ;
#94382=CARTESIAN_POINT('Ctrl Pts',(-19.9883521541963,37.6185544642137,124.469690929429)) ;
#94383=CARTESIAN_POINT('Ctrl Pts',(-19.7980711005547,37.6284415853776,124.553374455304)) ;
#94384=CARTESIAN_POINT('Ctrl Pts',(-19.5941096168226,37.6384339282262,124.603607299162)) ;
#94385=CARTESIAN_POINT('Ctrl Pts',(-19.3854196090159,37.6483822294501,124.617543166686)) ;
#94386=CARTESIAN_POINT('Ctrl Pts',(-19.1776942445068,37.6583198071322,124.59536101191)) ;
#94387=CARTESIAN_POINT('Ctrl Pts',(-18.9759006440841,37.6683063815828,124.537360444332)) ;
#94388=CARTESIAN_POINT('Ctrl Pts',(-18.7865662535122,37.6783351914913,124.44460190326)) ;
#94389=CARTESIAN_POINT('Ctrl Pts',(-18.6186516713856,37.6882135127981,124.322405731051)) ;
#94390=CARTESIAN_POINT('Ctrl Pts',(-18.4724895997512,37.6982051601455,124.171531255687)) ;
#94391=CARTESIAN_POINT('Ctrl Pts',(-18.3546061642673,37.7082396835832,123.996595633162)) ;
#94392=CARTESIAN_POINT('Ctrl Pts',(-18.2699432637342,37.7181030404618,123.807284330611)) ;
#94393=CARTESIAN_POINT('Ctrl Pts',(-18.2183482689039,37.7281732671421,123.601982903703)) ;
#94394=CARTESIAN_POINT('Ctrl Pts',(-18.2035357130047,37.7380155752768,123.395589044217)) ;
#94395=CARTESIAN_POINT('Ctrl Pts',(-18.2242703516,37.7479763073002,123.187217231748)) ;
#94396=CARTESIAN_POINT('Ctrl Pts',(-18.2817100316851,37.7580141964983,122.984164159135)) ;
#94397=CARTESIAN_POINT('Ctrl Pts',(-18.3717050421418,37.7678884794172,122.797069705704)) ;
#94398=CARTESIAN_POINT('Ctrl Pts',(-18.4951947219653,37.7779582240346,122.625155864398)) ;
#94399=CARTESIAN_POINT('Ctrl Pts',(-18.6430558845432,37.7877915343803,122.48065748324)) ;
#94400=CARTESIAN_POINT('Ctrl Pts',(-18.8168224196288,37.7978217777329,122.361207121415)) ;
#94401=CARTESIAN_POINT('Ctrl Pts',(-19.0089987621036,37.8078540657113,122.274295745002)) ;
#94402=CARTESIAN_POINT('Ctrl Pts',(-19.2090434153419,37.8176812421794,122.22266624776)) ;
#94403=CARTESIAN_POINT('Ctrl Pts',(-19.418687613471,37.8276866250463,122.205831123494)) ;
#94404=CARTESIAN_POINT('Ctrl Pts',(-19.6276535689647,37.837669264039,122.225683029359)) ;
#94405=CARTESIAN_POINT('Ctrl Pts',(-19.8311151455432,37.8477133311756,122.282093503812)) ;
#94406=CARTESIAN_POINT('Ctrl Pts',(-20.0176419945496,37.8575345499796,122.370645995862)) ;
#94407=CARTESIAN_POINT('Ctrl Pts',(-20.189959189523,37.8675713889177,122.492420091095)) ;
#94408=CARTESIAN_POINT('Ctrl Pts',(-20.3379110108571,37.8775958010154,122.642508840557)) ;
#94409=CARTESIAN_POINT('Ctrl Pts',(-20.455873413021,37.8874478854207,122.812760429535)) ;
#94410=CARTESIAN_POINT('Ctrl Pts',(-20.5439817121948,37.8974387821639,123.003399294509)) ;
#94411=CARTESIAN_POINT('Ctrl Pts',(-20.5974030957695,37.9073567740648,123.204972770783)) ;
#94412=CARTESIAN_POINT('Ctrl Pts',(-20.6152555329901,37.9173848895218,123.415021611092)) ;
#94413=CARTESIAN_POINT('Ctrl Pts',(-20.5967206689066,37.927270065464,123.622015755364)) ;
#94414=CARTESIAN_POINT('Ctrl Pts',(-20.5424483524076,37.9372594238708,123.824894035704)) ;
#94415=CARTESIAN_POINT('Ctrl Pts',(-20.4529119954387,37.9473005714511,124.01606111414)) ;
#94416=CARTESIAN_POINT('Ctrl Pts',(-20.3343454418545,37.9571331944576,124.185386044338)) ;
#94417=CARTESIAN_POINT('Ctrl Pts',(-20.1862012412486,37.9671272655683,124.334369804642)) ;
#94418=CARTESIAN_POINT('Ctrl Pts',(-20.0135915966174,37.9771559232092,124.455455360965)) ;
#94419=CARTESIAN_POINT('Ctrl Pts',(-19.8254446591091,37.987040249402,124.543643786109)) ;
#94420=CARTESIAN_POINT('Ctrl Pts',(-19.6233091240943,37.9970059928926,124.598773682631)) ;
#94421=CARTESIAN_POINT('Ctrl Pts',(-19.413348853934,38.0070343720238,124.61778442774)) ;
#94422=CARTESIAN_POINT('Ctrl Pts',(-19.2058864365111,38.0169352182307,124.600587770321)) ;
#94423=CARTESIAN_POINT('Ctrl Pts',(-19.001424766505,38.0269938756478,124.546746006836)) ;
#94424=CARTESIAN_POINT('Ctrl Pts',(-18.8131022714077,38.0368514384297,124.460160333376)) ;
#94425=CARTESIAN_POINT('Ctrl Pts',(-18.6390069711874,38.0469198409829,124.339821058919)) ;
#94426=CARTESIAN_POINT('Ctrl Pts',(-18.4916162272033,38.0567752397225,124.19417910208)) ;
#94427=CARTESIAN_POINT('Ctrl Pts',(-18.3695561098639,38.0667701067964,124.023151838683)) ;
#94428=CARTESIAN_POINT('Ctrl Pts',(-18.2791222072154,38.0768014017799,123.832631960833)) ;
#94429=CARTESIAN_POINT('Ctrl Pts',(-18.2237417192545,38.0866679265065,123.63272885643)) ;
#94430=CARTESIAN_POINT('Ctrl Pts',(-18.2033366603829,38.0966553972022,123.423780120613)) ;
#94431=CARTESIAN_POINT('Ctrl Pts',(-18.2193409243599,38.106600156766,123.215291220018)) ;
#94432=CARTESIAN_POINT('Ctrl Pts',(-18.2719426736711,38.1166457127149,123.010781898798)) ;
#94433=CARTESIAN_POINT('Ctrl Pts',(-18.3574578509409,38.12650530109,122.821937896345)) ;
#94434=CARTESIAN_POINT('Ctrl Pts',(-18.4758459936712,38.136506256226,122.648227483148)) ;
#94435=CARTESIAN_POINT('Ctrl Pts',(-18.6211084110624,38.1464104835036,122.499006529391)) ;
#94436=CARTESIAN_POINT('Ctrl Pts',(-18.7923421380688,38.1564525603987,122.375568101982)) ;
#94437=CARTESIAN_POINT('Ctrl Pts',(-18.9798774392675,38.1663601730849,122.284845061643)) ;
#94438=CARTESIAN_POINT('Ctrl Pts',(-19.1832185039879,38.1764147037006,122.227224424834)) ;
#94439=CARTESIAN_POINT('Ctrl Pts',(-19.3894682522631,38.1862754902495,122.206072297823)) ;
#94440=CARTESIAN_POINT('Ctrl Pts',(-19.5990134009756,38.1962692453206,122.220862900909)) ;
#94441=CARTESIAN_POINT('Ctrl Pts',(-19.8015016142954,38.2061946055606,122.271381265112)) ;
#94442=CARTESIAN_POINT('Ctrl Pts',(-19.9940600894447,38.2162225349558,122.357136882958)) ;
#94443=CARTESIAN_POINT('Ctrl Pts',(-20.1665038918111,38.2261088017551,122.473213620408)) ;
#94444=CARTESIAN_POINT('Ctrl Pts',(-20.3184039299682,38.2361405706534,122.619467232324)) ;
#94445=CARTESIAN_POINT('Ctrl Pts',(-20.4409493063373,38.246022166497,122.787261758585)) ;
#94446=CARTESIAN_POINT('Ctrl Pts',(-20.534186053703,38.256084051965,122.977102546347)) ;
#94447=CARTESIAN_POINT('Ctrl Pts',(-20.5919300858513,38.2659414859838,123.17615703249)) ;
#94448=CARTESIAN_POINT('Ctrl Pts',(-20.6149768459741,38.2759347290258,123.384952025093)) ;
#94449=CARTESIAN_POINT('Ctrl Pts',(-20.601518044384,38.2858654899121,123.593303693139)) ;
#94450=CARTESIAN_POINT('Ctrl Pts',(-20.5353365143575,38.2992144821093,123.866067761415)) ;
#94451=CARTESIAN_POINT('Ctrl Pts',(-20.3999665225162,38.3124828549258,124.11359517286)) ;
#94452=CARTESIAN_POINT('Ctrl Pts',(-20.2075244309159,38.3257657963101,124.315918886567)) ;
#94453=CARTESIAN_POINT('Ctrl Pts',(-20.0375783875477,38.3358085821523,124.441187536565)) ;
#94454=CARTESIAN_POINT('Ctrl Pts',(-19.8521843982202,38.3456585247044,124.533448788137)) ;
#94455=CARTESIAN_POINT('Ctrl Pts',(-19.6507787179192,38.3556557576234,124.59349689104)) ;
#94456=CARTESIAN_POINT('Ctrl Pts',(-19.4415865176942,38.3656706529579,124.617384094743)) ;
#94457=CARTESIAN_POINT('Ctrl Pts',(-19.1637206293595,38.3789103295961,124.600727750445)) ;
#94458=CARTESIAN_POINT('Ctrl Pts',(-18.8297225787506,38.3954575540015,124.490328714374)) ;
#94459=CARTESIAN_POINT('Ctrl Pts',(-18.5515626138001,38.4121049911325,124.271315950757)) ;
#94460=CARTESIAN_POINT('Ctrl Pts',(-18.3844931449848,38.4253944886108,124.047426550123)) ;
#94461=CARTESIAN_POINT('Ctrl Pts',(-18.2905580247647,38.4352678964331,123.862315124557)) ;
#94462=CARTESIAN_POINT('Ctrl Pts',(-18.2290723599006,38.4453202740258,123.660137252255)) ;
#94463=CARTESIAN_POINT('Ctrl Pts',(-18.2040857486396,38.4552239275667,123.453418477981)) ;
#94464=CARTESIAN_POINT('Ctrl Pts',(-18.214910209593,38.465168196562,123.244668963896)) ;
#94465=CARTESIAN_POINT('Ctrl Pts',(-18.2776890327656,38.4784992048947,122.971450485448)) ;
#94466=CARTESIAN_POINT('Ctrl Pts',(-18.4435332627468,38.495120785419,122.659461049717)) ;
#94467=CARTESIAN_POINT('Ctrl Pts',(-18.704296009692,38.5116634561174,122.423288645421)) ;
#94468=CARTESIAN_POINT('Ctrl Pts',(-18.9539077831196,38.5250126156803,122.295137360365)) ;
#94469=CARTESIAN_POINT('Ctrl Pts',(-19.2195501392417,38.5382407658398,122.212666362541)) ;
#94470=CARTESIAN_POINT('Ctrl Pts',(-19.5728079711518,38.5548714429773,122.198403766473)) ;
#94471=CARTESIAN_POINT('Ctrl Pts',(-19.976146658423,38.5747743822654,122.326687099106)) ;
#94472=CARTESIAN_POINT('Ctrl Pts',(-20.3116532871837,38.5946772488687,122.584476695311)) ;
#94473=CARTESIAN_POINT('Ctrl Pts',(-20.5398098955763,38.6145904139735,122.941266434743)) ;
#94474=CARTESIAN_POINT('Ctrl Pts',(-20.6324050425988,38.6346262431149,123.357036122555)) ;
#94475=CARTESIAN_POINT('Ctrl Pts',(-20.5783887869263,38.6544448179929,123.775059980348)) ;
#94476=CARTESIAN_POINT('Ctrl Pts',(-20.3841956533743,38.6744151190349,124.152516163581)) ;
#94477=CARTESIAN_POINT('Ctrl Pts',(-20.073957019028,38.6943066513995,124.440209371613)) ;
#94478=CARTESIAN_POINT('Ctrl Pts',(-19.6816966154287,38.714329749216,124.605463094587)) ;
#94479=CARTESIAN_POINT('Ctrl Pts',(-19.2612630755405,38.7341265021359,124.627003828453)) ;
#94480=CARTESIAN_POINT('Ctrl Pts',(-18.8551290904291,38.7540875906247,124.50387119971)) ;
#94481=CARTESIAN_POINT('Ctrl Pts',(-18.5155747208721,38.7740658595569,124.248566076367)) ;
#94482=CARTESIAN_POINT('Ctrl Pts',(-18.2848896984767,38.7938858743479,123.895929221417)) ;
#94483=CARTESIAN_POINT('Ctrl Pts',(-18.1867323093592,38.8138242835997,123.483482278785)) ;
#94484=CARTESIAN_POINT('Ctrl Pts',(-18.2364347422349,38.8338714009922,123.060080100057)) ;
#94485=CARTESIAN_POINT('Ctrl Pts',(-18.4258542295812,38.853717646826,122.683047614378)) ;
#94486=CARTESIAN_POINT('Ctrl Pts',(-18.731512097542,38.873566615338,122.391994315492)) ;
#94487=CARTESIAN_POINT('Ctrl Pts',(-19.1222233612243,38.8936169176493,122.22152470631)) ;
#94488=CARTESIAN_POINT('Ctrl Pts',(-19.543235364252,38.9134518400806,122.194986119466)) ;
#94489=CARTESIAN_POINT('Ctrl Pts',(-19.9499551551053,38.9333822413064,122.313413194632)) ;
#94490=CARTESIAN_POINT('Ctrl Pts',(-20.2916490712342,38.9532671866653,122.562710767896)) ;
#94491=CARTESIAN_POINT('Ctrl Pts',(-20.5292736704849,38.9733397948167,122.917142233502)) ;
#94492=CARTESIAN_POINT('Ctrl Pts',(-20.6303535211115,38.9931311111448,123.325705227082)) ;
#94493=CARTESIAN_POINT('Ctrl Pts',(-20.58686894099,39.0130959009121,123.747941927736)) ;
#94494=CARTESIAN_POINT('Ctrl Pts',(-20.4007639214894,39.0330788566624,124.129914872048)) ;
#94495=CARTESIAN_POINT('Ctrl Pts',(-20.0987294817913,39.0528873786385,124.423515961885)) ;
#94496=CARTESIAN_POINT('Ctrl Pts',(-19.7115170894291,39.0728729533743,124.598356596514)) ;
#94497=CARTESIAN_POINT('Ctrl Pts',(-19.2898685978214,39.0927555934427,124.630327657411)) ;
#94498=CARTESIAN_POINT('Ctrl Pts',(-18.881219954821,39.1127109055746,124.516450708816)) ;
#94499=CARTESIAN_POINT('Ctrl Pts',(-18.5370774718083,39.1325852621824,124.271087878377)) ;
#94500=CARTESIAN_POINT('Ctrl Pts',(-18.2958623645042,39.1525674690435,123.921382047478)) ;
#94501=CARTESIAN_POINT('Ctrl Pts',(-18.188922682226,39.1724985469935,123.511215574697)) ;
#94502=CARTESIAN_POINT('Ctrl Pts',(-18.2282858959202,39.1924255218484,123.089434355908)) ;
#94503=CARTESIAN_POINT('Ctrl Pts',(-18.4076743420481,39.2122579807973,122.707733371159)) ;
#94504=CARTESIAN_POINT('Ctrl Pts',(-18.6583859348494,39.2289156649725,122.457712360878)) ;
#94505=CARTESIAN_POINT('Ctrl Pts',(-18.899856718345,39.2421648888796,122.318686734846)) ;
#94506=CARTESIAN_POINT('Ctrl Pts',(-19.0984024083367,39.2522139103308,122.246593165114)) ;
#94507=CARTESIAN_POINT('Ctrl Pts',(-19.3025722169409,39.2620739185613,122.21069862246)) ;
#94508=CARTESIAN_POINT('Ctrl Pts',(-19.5818091443414,39.2753574317859,122.209905164307)) ;
#94509=CARTESIAN_POINT('Ctrl Pts',(-19.923863738097,39.2920033507868,122.300944035455)) ;
#94510=CARTESIAN_POINT('Ctrl Pts',(-20.212949843861,39.3085573286028,122.501708285792)) ;
#94511=CARTESIAN_POINT('Ctrl Pts',(-20.3943693525762,39.3219170575744,122.716154726011)) ;
#94512=CARTESIAN_POINT('Ctrl Pts',(-20.4992257353742,39.3318101093711,122.895780909833)) ;
#94513=CARTESIAN_POINT('Ctrl Pts',(-20.5722643826613,39.3418000746522,123.092667970751)) ;
#94514=CARTESIAN_POINT('Ctrl Pts',(-20.6099946182295,39.351751955513,123.298490502121)) ;
#94515=CARTESIAN_POINT('Ctrl Pts',(-20.6112491588045,39.3618003072048,123.509712360783)) ;
#94516=CARTESIAN_POINT('Ctrl Pts',(-20.5767745748545,39.371641591311,123.713735938484)) ;
#94517=CARTESIAN_POINT('Ctrl Pts',(-20.5068084537327,39.3816282944367,123.91164782318)) ;
#94518=CARTESIAN_POINT('Ctrl Pts',(-20.4041499408619,39.3915633232541,124.093590241754)) ;
#94519=CARTESIAN_POINT('Ctrl Pts',(-20.2697572274367,39.401619118161,124.256736889901)) ;
#94520=CARTESIAN_POINT('Ctrl Pts',(-20.1128745603871,39.4114474814503,124.391246892535)) ;
#94521=CARTESIAN_POINT('Ctrl Pts',(-19.9310134092115,39.4215084513482,124.499192648327)) ;
#94522=CARTESIAN_POINT('Ctrl Pts',(-19.7359479774225,39.431422730238,124.5726887504)) ;
#94523=CARTESIAN_POINT('Ctrl Pts',(-19.5292236814562,39.4414317247063,124.61196971549)) ;
#94524=CARTESIAN_POINT('Ctrl Pts',(-19.318381422526,39.45146155927,124.614334355691)) ;
#94525=CARTESIAN_POINT('Ctrl Pts',(-19.1138104319035,39.4613197893422,124.581026332675)) ;
#94526=CARTESIAN_POINT('Ctrl Pts',(-18.9153042039635,39.4713184950847,124.511985701486)) ;
#94527=CARTESIAN_POINT('Ctrl Pts',(-18.7335269690382,39.4812131510035,124.410773863355)) ;
#94528=CARTESIAN_POINT('Ctrl Pts',(-18.56943634765,39.4912762153874,124.27729901204)) ;
#94529=CARTESIAN_POINT('Ctrl Pts',(-18.4338684117393,39.5011158736673,124.121008549129)) ;
#94530=CARTESIAN_POINT('Ctrl Pts',(-18.3248828460409,39.5111790407491,123.9397151691)) ;
#94531=CARTESIAN_POINT('Ctrl Pts',(-18.2504503765499,39.5210732858762,123.745455632953)) ;
#94532=CARTESIAN_POINT('Ctrl Pts',(-18.2101397435108,39.5310151074809,123.540397852165)) ;
#94533=CARTESIAN_POINT('Ctrl Pts',(-18.205942485578,39.5410176383989,123.330126951138)) ;
#94534=CARTESIAN_POINT('Ctrl Pts',(-18.2387400810565,39.5510522648564,123.121743690453)) ;
#94535=CARTESIAN_POINT('Ctrl Pts',(-18.3056247092528,39.5608977998429,122.925856505686)) ;
#94536=CARTESIAN_POINT('Ctrl Pts',(-18.4064939010015,39.5708812246819,122.741821095179)) ;
#94537=CARTESIAN_POINT('Ctrl Pts',(-18.5373982428774,39.580831615047,122.578645626432)) ;
#94538=CARTESIAN_POINT('Ctrl Pts',(-18.6952153507087,39.590829255344,122.439801676693)) ;
#94539=CARTESIAN_POINT('Ctrl Pts',(-18.8756822378047,39.6008683359072,122.330394244485)) ;
#94540=CARTESIAN_POINT('Ctrl Pts',(-19.0680855983055,39.6106944866763,122.255165125294)) ;
#94541=CARTESIAN_POINT('Ctrl Pts',(-19.2752888340513,39.6207510616055,122.21320663692)) ;
#94542=CARTESIAN_POINT('Ctrl Pts',(-19.4842192743884,39.6306916009857,122.208288938117)) ;
#94543=CARTESIAN_POINT('Ctrl Pts',(-19.6901728368781,39.6405959939621,122.23896416273)) ;
#94544=CARTESIAN_POINT('Ctrl Pts',(-19.8904453983697,39.650642648167,122.306001788215)) ;
#94545=CARTESIAN_POINT('Ctrl Pts',(-20.0733802115196,39.6605382101054,122.405136530258)) ;
#94546=CARTESIAN_POINT('Ctrl Pts',(-20.239014832524,39.670600287951,122.536666603804)) ;
#94547=CARTESIAN_POINT('Ctrl Pts',(-20.3763608522466,39.6804429863648,122.691467796565)) ;
#94548=CARTESIAN_POINT('Ctrl Pts',(-20.4867687217227,39.6904337613262,122.870114185754)) ;
#94549=CARTESIAN_POINT('Ctrl Pts',(-20.563976360036,39.7003616263453,123.06403607056)) ;
#94550=CARTESIAN_POINT('Ctrl Pts',(-20.6069421620117,39.7103503711115,123.269592670156)) ;
#94551=CARTESIAN_POINT('Ctrl Pts',(-20.6132830463092,39.7203831566985,123.480421504479)) ;
#94552=CARTESIAN_POINT('Ctrl Pts',(-20.5836334775982,39.7302498413191,123.685712607016)) ;
#94553=CARTESIAN_POINT('Ctrl Pts',(-20.518733142917,39.7402117334822,123.884836785975)) ;
#94554=CARTESIAN_POINT('Ctrl Pts',(-20.4192475547195,39.7502452103948,124.070827748899)) ;
#94555=CARTESIAN_POINT('Ctrl Pts',(-20.2911532789775,39.7601295516431,124.234483917297)) ;
#94556=CARTESIAN_POINT('Ctrl Pts',(-20.1338366585851,39.7701924937642,124.375890200317)) ;
#94557=CARTESIAN_POINT('Ctrl Pts',(-19.9581654376488,39.7800428953838,124.485576269177)) ;
#94558=CARTESIAN_POINT('Ctrl Pts',(-19.7628967146071,39.7900697841735,124.564969156338)) ;
#94559=CARTESIAN_POINT('Ctrl Pts',(-19.5566424600458,39.8000983991297,124.608721741187)) ;
#94560=CARTESIAN_POINT('Ctrl Pts',(-19.34981381734,39.8099436222498,124.616255061362)) ;
#94561=CARTESIAN_POINT('Ctrl Pts',(-19.1416957983259,39.8199343060557,124.587896768431)) ;
#94562=CARTESIAN_POINT('Ctrl Pts',(-18.9408691509651,39.8299721881281,124.523084945167)) ;
#94563=CARTESIAN_POINT('Ctrl Pts',(-18.7577650189888,39.839816547767,124.42660549306)) ;
#94564=CARTESIAN_POINT('Ctrl Pts',(-18.5916351240008,39.8498014183817,124.298338388516)) ;
#94565=CARTESIAN_POINT('Ctrl Pts',(-18.4508347820377,39.8597407017104,124.143903025515)) ;
#94566=CARTESIAN_POINT('Ctrl Pts',(-18.337932004996,39.8697813110835,123.965575193897)) ;
#94567=CARTESIAN_POINT('Ctrl Pts',(-18.2587923235217,39.8796661619968,123.773397832722)) ;
#94568=CARTESIAN_POINT('Ctrl Pts',(-18.2134600339638,39.8896681181656,123.568102263173)) ;
#94569=CARTESIAN_POINT('Ctrl Pts',(-18.2043675449943,39.899586714886,123.359747507517)) ;
#94570=CARTESIAN_POINT('Ctrl Pts',(-18.2319750519706,39.9096335369618,123.150373488916)) ;
#94571=CARTESIAN_POINT('Ctrl Pts',(-18.294259354094,39.9195078180745,122.952312235387)) ;
#94572=CARTESIAN_POINT('Ctrl Pts',(-18.3915851916145,39.9295620181191,122.76472228793)) ;
#94573=CARTESIAN_POINT('Ctrl Pts',(-18.5179539634958,39.9394574477544,122.599419731205)) ;
#94574=CARTESIAN_POINT('Ctrl Pts',(-18.6735953495587,39.9495190760717,122.456211511714)) ;
#94575=CARTESIAN_POINT('Ctrl Pts',(-18.847909017395,39.9593637049016,122.344621876972)) ;
#94576=CARTESIAN_POINT('Ctrl Pts',(-19.040889665129,39.9693237525072,122.263369324957)) ;
#94577=CARTESIAN_POINT('Ctrl Pts',(-19.2467363166001,39.9793620586813,122.216899420079)) ;
#94578=CARTESIAN_POINT('Ctrl Pts',(-19.4540820779037,39.989235358114,122.206640501949)) ;
#94579=CARTESIAN_POINT('Ctrl Pts',(-19.6641480891953,39.9993086197002,122.23312299692)) ;
#94580=CARTESIAN_POINT('Ctrl Pts',(-19.8615092289753,40.0091288456569,122.29387007229)) ;
#94581=CARTESIAN_POINT('Ctrl Pts',(-20.050164410473,40.0192079095964,122.390230244533)) ;
#94582=CARTESIAN_POINT('Ctrl Pts',(-20.2155277469042,40.0290579996162,122.51497058454)) ;
#94583=CARTESIAN_POINT('Ctrl Pts',(-20.3600033759325,40.03913675323,122.669891358918)) ;
#94584=CARTESIAN_POINT('Ctrl Pts',(-20.4726264296346,40.0489582204895,122.84300447148)) ;
#94585=CARTESIAN_POINT('Ctrl Pts',(-20.5557528197922,40.0590238188471,123.037552140448)) ;
#94586=CARTESIAN_POINT('Ctrl Pts',(-20.6030259582916,40.0689264746218,123.240351541043)) ;
#94587=CARTESIAN_POINT('Ctrl Pts',(-20.6145983084236,40.0789773004515,123.451291677188)) ;
#94588=CARTESIAN_POINT('Ctrl Pts',(-20.5900018228788,40.0888515047903,123.657461638171)) ;
#94589=CARTESIAN_POINT('Ctrl Pts',(-20.5288150346182,40.0989239548294,123.860137146693)) ;
#94590=CARTESIAN_POINT('Ctrl Pts',(-20.435813281628,40.1087529716029,124.044705968251)) ;
#94591=CARTESIAN_POINT('Ctrl Pts',(-20.3094637582039,40.1188198175177,124.214444012367)) ;
#94592=CARTESIAN_POINT('Ctrl Pts',(-20.1581261550177,40.1287099888195,124.357060544978)) ;
#94593=CARTESIAN_POINT('Ctrl Pts',(-19.982817511392,40.1387021824434,124.47277610636)) ;
#94594=CARTESIAN_POINT('Ctrl Pts',(-19.7905608961819,40.1486649930668,124.555869120237)) ;
#94595=CARTESIAN_POINT('Ctrl Pts',(-19.5880955015858,40.1585692659102,124.604552608596)) ;
#94596=CARTESIAN_POINT('Ctrl Pts',(-19.3770061673514,40.1686297577149,124.617357351724)) ;
#94597=CARTESIAN_POINT('Ctrl Pts',(-19.1714136948424,40.1784700893872,124.594104022115)) ;
#94598=CARTESIAN_POINT('Ctrl Pts',(-18.9684724817499,40.1885331354789,124.534440358675)) ;
#94599=CARTESIAN_POINT('Ctrl Pts',(-18.7821898037075,40.198427191174,124.441849153616)) ;
#94600=CARTESIAN_POINT('Ctrl Pts',(-18.6136872008916,40.208369891497,124.318199456405)) ;
#94601=CARTESIAN_POINT('Ctrl Pts',(-18.4682361054831,40.2183756324246,124.166208401796)) ;
#94602=CARTESIAN_POINT('Ctrl Pts',(-18.3514207087649,40.2283965429401,123.990896073496)) ;
#94603=CARTESIAN_POINT('Ctrl Pts',(-18.2676944149696,40.2382872783901,123.800556542411)) ;
#94604=CARTESIAN_POINT('Ctrl Pts',(-18.2174871494906,40.2482788191189,123.596600054224)) ;
#94605=CARTESIAN_POINT('Ctrl Pts',(-18.2035765205634,40.2582266795406,123.38792968964)) ;
#94606=CARTESIAN_POINT('Ctrl Pts',(-18.2256975206144,40.2681733487269,123.179981160546)) ;
#94607=CARTESIAN_POINT('Ctrl Pts',(-18.284396273702,40.2782214248625,122.977065964015)) ;
#94608=CARTESIAN_POINT('Ctrl Pts',(-18.3754280331903,40.2880690228682,122.791125047696)) ;
#94609=CARTESIAN_POINT('Ctrl Pts',(-18.4982372564915,40.2980307459526,122.621498409883)) ;
#94610=CARTESIAN_POINT('Ctrl Pts',(-18.6498468908888,40.3080593810356,122.474969336951)) ;
#94611=CARTESIAN_POINT('Ctrl Pts',(-18.8224769474675,40.3179696893537,122.358338779298)) ;
#94612=CARTESIAN_POINT('Ctrl Pts',(-19.0129987885673,40.3279045864895,122.272737608116)) ;
#94613=CARTESIAN_POINT('Ctrl Pts',(-19.2176901556967,40.3379456694321,122.221162637048)) ;
#94614=CARTESIAN_POINT('Ctrl Pts',(-19.4250097860347,40.3478330122603,122.206002228677)) ;
#94615=CARTESIAN_POINT('Ctrl Pts',(-19.6340061659135,40.3578245271997,122.226929966425)) ;
#94616=CARTESIAN_POINT('Ctrl Pts',(-19.8353738299517,40.3677759183962,122.283688970992)) ;
#94617=CARTESIAN_POINT('Ctrl Pts',(-20.0236219513541,40.3777084517288,122.37404934811)) ;
#94618=CARTESIAN_POINT('Ctrl Pts',(-20.1944682236127,40.3877056096282,122.496443492551)) ;
#94619=CARTESIAN_POINT('Ctrl Pts',(-20.3413742021362,40.3976906197917,122.64643432917)) ;
#94620=CARTESIAN_POINT('Ctrl Pts',(-20.4604016269849,40.4077334463615,122.820781880567)) ;
#94621=CARTESIAN_POINT('Ctrl Pts',(-20.5459653741827,40.4175636806665,123.008934961586)) ;
#94622=CARTESIAN_POINT('Ctrl Pts',(-20.5989226586347,40.4276397059012,123.213993634072)) ;
#94623=CARTESIAN_POINT('Ctrl Pts',(-20.6152177268763,40.437491942392,123.420521244242)) ;
#94624=CARTESIAN_POINT('Ctrl Pts',(-20.595146375222,40.4475651488262,123.631304239716)) ;
#94625=CARTESIAN_POINT('Ctrl Pts',(-20.540009566013,40.4574066583333,123.830735651141)) ;
#94626=CARTESIAN_POINT('Ctrl Pts',(-20.4507245575497,40.4673676051131,124.020150554085)) ;
#94627=CARTESIAN_POINT('Ctrl Pts',(-20.328629514598,40.4774054339132,124.192262261926)) ;
#94628=CARTESIAN_POINT('Ctrl Pts',(-20.1811994533202,40.4872797436676,124.338439938895)) ;
#94629=CARTESIAN_POINT('Ctrl Pts',(-20.0072892895941,40.4973494413408,124.459100732173)) ;
#94630=CARTESIAN_POINT('Ctrl Pts',(-19.8195861713567,40.5071829126282,124.545769387066)) ;
#94631=CARTESIAN_POINT('Ctrl Pts',(-19.6158723309425,40.5172125591581,124.600164943048)) ;
#94632=CARTESIAN_POINT('Ctrl Pts',(-19.4056431711912,40.5272470734855,124.617731141067)) ;
#94633=CARTESIAN_POINT('Ctrl Pts',(-19.1998966723173,40.5370723589564,124.599424024852)) ;
#94634=CARTESIAN_POINT('Ctrl Pts',(-18.9967300833823,40.5470766005049,124.545129025177)) ;
#94635=CARTESIAN_POINT('Ctrl Pts',(-18.8064674259358,40.557059245584,124.456466509944)) ;
#94636=CARTESIAN_POINT('Ctrl Pts',(-18.6336011039915,40.5671044426755,124.335200583634)) ;
#94637=CARTESIAN_POINT('Ctrl Pts',(-18.4874473744563,40.5769275584357,124.18929088824)) ;
#94638=CARTESIAN_POINT('Ctrl Pts',(-18.3658653991529,40.5869621702359,124.016894776006)) ;
#94639=CARTESIAN_POINT('Ctrl Pts',(-18.276679009699,40.5969871790091,123.825931021267)) ;
#94640=CARTESIAN_POINT('Ctrl Pts',(-18.2225124725489,40.6068391038507,123.626017281028)) ;
#94641=CARTESIAN_POINT('Ctrl Pts',(-18.2032990756932,40.6168300421734,123.416882426706)) ;
#94642=CARTESIAN_POINT('Ctrl Pts',(-18.2204327216342,40.6267480273198,123.209055359799)) ;
#94643=CARTESIAN_POINT('Ctrl Pts',(-18.2739197540757,40.6367761282153,123.005147720835)) ;
#94644=CARTESIAN_POINT('Ctrl Pts',(-18.3606743245139,40.6466613691579,122.816298477163)) ;
#94645=CARTESIAN_POINT('Ctrl Pts',(-18.4797205501909,40.6566504821245,122.643290611343)) ;
#94646=CARTESIAN_POINT('Ctrl Pts',(-18.6281007030375,40.6666925464653,122.493120519007)) ;
#94647=CARTESIAN_POINT('Ctrl Pts',(-18.7964346089522,40.6765217478698,122.373256814763)) ;
#94648=CARTESIAN_POINT('Ctrl Pts',(-18.9861689428524,40.686528588628,122.282435666904)) ;
#94649=CARTESIAN_POINT('Ctrl Pts',(-19.1884902469332,40.6965161128199,122.226152191325)) ;
#94650=CARTESIAN_POINT('Ctrl Pts',(-19.3983530777978,40.7065457586286,122.205918577361)) ;
#94651=CARTESIAN_POINT('Ctrl Pts',(-19.6053392656737,40.7164197893673,122.221929297566)) ;
#94652=CARTESIAN_POINT('Ctrl Pts',(-19.8089638125381,40.7264191122314,122.274027018103)) ;
#94653=CARTESIAN_POINT('Ctrl Pts',(-19.9989028221292,40.736329947807,122.359763953984)) ;
#94654=CARTESIAN_POINT('Ctrl Pts',(-20.1734602714543,40.746384195781,122.478901030537)) ;
#94655=CARTESIAN_POINT('Ctrl Pts',(-20.3219594084371,40.7562429400437,122.62353974604)) ;
#94656=CARTESIAN_POINT('Ctrl Pts',(-20.4457241120794,40.7663110261167,122.795209533681)) ;
#94657=CARTESIAN_POINT('Ctrl Pts',(-20.5358630666679,40.7761665092963,122.981787019375)) ;
#94658=CARTESIAN_POINT('Ctrl Pts',(-20.593633206338,40.7861613550904,123.183805530835)) ;
#94659=CARTESIAN_POINT('Ctrl Pts',(-20.6150774328527,40.796192650753,123.393606073718)) ;
#94660=CARTESIAN_POINT('Ctrl Pts',(-20.6003488764673,40.8060591940429,123.600515261754)) ;
#94661=CARTESIAN_POINT('Ctrl Pts',(-20.549636410078,40.8160465898062,123.804239901806)) ;
#94662=CARTESIAN_POINT('Ctrl Pts',(-20.4647624174403,40.8259916305362,123.995347584397)) ;
#94663=CARTESIAN_POINT('Ctrl Pts',(-20.3467582642971,40.8360361367529,124.170441043399)) ;
#94664=CARTESIAN_POINT('Ctrl Pts',(-20.202893284739,40.8458996428903,124.319807451803)) ;
#94665=CARTESIAN_POINT('Ctrl Pts',(-20.0333415385415,40.8558925037263,124.443797452948)) ;
#94666=CARTESIAN_POINT('Ctrl Pts',(-19.8460832863042,40.8658186974453,124.535960572849)) ;
#94667=CARTESIAN_POINT('Ctrl Pts',(-19.6438582328255,40.8758376234778,124.594776915068)) ;
#94668=CARTESIAN_POINT('Ctrl Pts',(-19.436629966288,40.8857526228454,124.617551938887)) ;
#94669=CARTESIAN_POINT('Ctrl Pts',(-19.2257233942955,40.8958073944027,124.603768109833)) ;
#94670=CARTESIAN_POINT('Ctrl Pts',(-19.0243302771047,40.9056663567003,124.554668324937)) ;
#94671=CARTESIAN_POINT('Ctrl Pts',(-18.8318134848253,40.9156606005381,124.470587726134)) ;
#94672=CARTESIAN_POINT('Ctrl Pts',(-18.6579190371957,40.9255858299624,124.355204812774)) ;
#94673=CARTESIAN_POINT('Ctrl Pts',(-18.5051729778743,40.9356137938538,124.209940570375)) ;
#94674=CARTESIAN_POINT('Ctrl Pts',(-18.3815316830435,40.9455000534842,124.042837464841)) ;
#94675=CARTESIAN_POINT('Ctrl Pts',(-18.2873498073833,40.9555318165621,123.85417507662)) ;
#94676=CARTESIAN_POINT('Ctrl Pts',(-18.2280402867286,40.9654134428562,123.655039667147)) ;
#94677=CARTESIAN_POINT('Ctrl Pts',(-18.2037261411978,40.9754752123424,123.444942837729)) ;
#94678=CARTESIAN_POINT('Ctrl Pts',(-18.2159492443396,40.9853330798378,123.23803488184)) ;
#94679=CARTESIAN_POINT('Ctrl Pts',(-18.2640991622364,40.9953247049552,123.033597970175)) ;
#94680=CARTESIAN_POINT('Ctrl Pts',(-18.3466098904373,41.0052615040634,122.841666372435)) ;
#94681=CARTESIAN_POINT('Ctrl Pts',(-18.4615560564106,41.0152523336208,122.665869282577)) ;
#94682=CARTESIAN_POINT('Ctrl Pts',(-18.605927064442,41.025275569334,122.51236953615)) ;
#94683=CARTESIAN_POINT('Ctrl Pts',(-18.7725080768488,41.0351719173631,122.387730228148)) ;
#94684=CARTESIAN_POINT('Ctrl Pts',(-18.9597603021565,41.0451614798656,122.292617751821)) ;
#94685=CARTESIAN_POINT('Ctrl Pts',(-19.1618068850491,41.0552017875502,122.231566043326)) ;
#94686=CARTESIAN_POINT('Ctrl Pts',(-19.3672327471221,41.0650440908974,122.206620708451)) ;
#94687=CARTESIAN_POINT('Ctrl Pts',(-19.5776399590884,41.0750677991764,122.217643519475)) ;
#94688=CARTESIAN_POINT('Ctrl Pts',(-19.8485691529838,41.0882899766441,122.280066801218)) ;
#94689=CARTESIAN_POINT('Ctrl Pts',(-20.0983814297562,41.1015825617034,122.412162007784)) ;
#94690=CARTESIAN_POINT('Ctrl Pts',(-20.303073380294,41.114867417625,122.602192166436)) ;
#94691=CARTESIAN_POINT('Ctrl Pts',(-20.4297314944804,41.1248396447978,122.769227524099)) ;
#94692=CARTESIAN_POINT('Ctrl Pts',(-20.5251912714743,41.1347482612368,122.954404492746)) ;
#94693=CARTESIAN_POINT('Ctrl Pts',(-20.5878572761394,41.1448014666205,123.156230134344)) ;
#94694=CARTESIAN_POINT('Ctrl Pts',(-20.6141674244472,41.1546666003808,123.361965570932)) ;
#94695=CARTESIAN_POINT('Ctrl Pts',(-20.6014118404237,41.1680056580072,123.642110925614)) ;
#94696=CARTESIAN_POINT('Ctrl Pts',(-20.4948859078202,41.1845748453403,123.977938811576)) ;
#94697=CARTESIAN_POINT('Ctrl Pts',(-20.2793745793678,41.2012199851913,124.258685783762)) ;
#94698=CARTESIAN_POINT('Ctrl Pts',(-20.0579576413168,41.2144922876647,124.428476543224)) ;
#94699=CARTESIAN_POINT('Ctrl Pts',(-19.8719402483463,41.2244732511124,124.5255422906)) ;
#94700=CARTESIAN_POINT('Ctrl Pts',(-19.6726895718307,41.2344150831817,124.588712912963)) ;
#94701=CARTESIAN_POINT('Ctrl Pts',(-19.3951595665634,41.2477346523971,124.625810172033)) ;
#94702=CARTESIAN_POINT('Ctrl Pts',(-19.0464438591427,41.2642648073298,124.581269942614)) ;
#94703=CARTESIAN_POINT('Ctrl Pts',(-18.6680925736183,41.2842865328219,124.38634423409)) ;
#94704=CARTESIAN_POINT('Ctrl Pts',(-18.3816919054068,41.3040979294287,124.077301406411)) ;
#94705=CARTESIAN_POINT('Ctrl Pts',(-18.2159313914178,41.3240831781376,123.686131229408)) ;
#94706=CARTESIAN_POINT('Ctrl Pts',(-18.1939891820258,41.3439772407735,123.263630954678)) ;
#94707=CARTESIAN_POINT('Ctrl Pts',(-18.3171494252576,41.3639089199471,122.858127898099)) ;
#94708=CARTESIAN_POINT('Ctrl Pts',(-18.5719341117351,41.3838729744191,122.518602617013)) ;
#94709=CARTESIAN_POINT('Ctrl Pts',(-18.925647690963,41.403753876182,122.287092819284)) ;
#94710=CARTESIAN_POINT('Ctrl Pts',(-19.3381949379129,41.4236925377904,122.189526544458)) ;
#94711=CARTESIAN_POINT('Ctrl Pts',(-19.7584054124552,41.4435890630457,122.238430586688)) ;
#94712=CARTESIAN_POINT('Ctrl Pts',(-20.1370058269527,41.4634841015001,122.427169281719)) ;
#94713=CARTESIAN_POINT('Ctrl Pts',(-20.4294053679111,41.4834479248061,122.734843310228)) ;
#94714=CARTESIAN_POINT('Ctrl Pts',(-20.5988096691988,41.5033220489352,123.122013486235)) ;
#94715=CARTESIAN_POINT('Ctrl Pts',(-20.6264542810702,41.5232971246625,123.545855807307)) ;
#94716=CARTESIAN_POINT('Ctrl Pts',(-20.5073565762459,41.5432506940191,123.953056711382)) ;
#94717=CARTESIAN_POINT('Ctrl Pts',(-20.2585449822176,41.5630886042069,124.293669103182)) ;
#94718=CARTESIAN_POINT('Ctrl Pts',(-19.9062555480821,41.5830644327778,124.530937490507)) ;
#94719=CARTESIAN_POINT('Ctrl Pts',(-19.4952527745966,41.6029824774881,124.632990018156)) ;
#94720=CARTESIAN_POINT('Ctrl Pts',(-19.074880553393,41.6228527232758,124.589826696202)) ;
#94721=CARTESIAN_POINT('Ctrl Pts',(-18.6915024510565,41.6429017263753,124.403663945132)) ;
#94722=CARTESIAN_POINT('Ctrl Pts',(-18.3981608225191,41.6626809676162,124.102123352267)) ;
#94723=CARTESIAN_POINT('Ctrl Pts',(-18.2226406505377,41.682711031325,123.714185617551)) ;
#94724=CARTESIAN_POINT('Ctrl Pts',(-18.1909502367662,41.702593316227,123.292557485542)) ;
#94725=CARTESIAN_POINT('Ctrl Pts',(-18.3038834095939,41.72247561712,122.885208119923)) ;
#94726=CARTESIAN_POINT('Ctrl Pts',(-18.5504266881587,41.7424587267384,122.539145738283)) ;
#94727=CARTESIAN_POINT('Ctrl Pts',(-18.8986863380999,41.7623491221162,122.299138995889)) ;
#94728=CARTESIAN_POINT('Ctrl Pts',(-19.307832379014,41.7822459121505,122.191754243473)) ;
#94729=CARTESIAN_POINT('Ctrl Pts',(-19.7296142472698,41.8021629660921,122.23001985925)) ;
#94730=CARTESIAN_POINT('Ctrl Pts',(-20.1146546672758,41.8221665142956,122.41084364833)) ;
#94731=CARTESIAN_POINT('Ctrl Pts',(-20.4133983983086,41.8421048079482,122.711612600344)) ;
#94732=CARTESIAN_POINT('Ctrl Pts',(-20.5914741795715,41.8619262953812,123.093609322435)) ;
#94733=CARTESIAN_POINT('Ctrl Pts',(-20.6292246792124,41.881904688372,123.516673333477)) ;
#94734=CARTESIAN_POINT('Ctrl Pts',(-20.5204944182451,41.9018030699857,123.925630858836)) ;
#94735=CARTESIAN_POINT('Ctrl Pts',(-20.3195273566345,41.9183860007156,124.215224343354)) ;
#94736=CARTESIAN_POINT('Ctrl Pts',(-20.1066686455886,41.9316602363045,124.395804425527)) ;
#94737=CARTESIAN_POINT('Ctrl Pts',(-19.9243029169326,41.9417066537607,124.502286315057)) ;
#94738=CARTESIAN_POINT('Ctrl Pts',(-19.7302093112894,41.9515518789799,124.574250358946)) ;
#94739=CARTESIAN_POINT('Ctrl Pts',(-19.4546062106336,41.9648868500193,124.625183233532)) ;
#94740=CARTESIAN_POINT('Ctrl Pts',(-19.1029743251083,41.981469706812,124.597295458286)) ;
#94741=CARTESIAN_POINT('Ctrl Pts',(-18.7810078469193,41.9981127091614,124.450748808051)) ;
#94742=CARTESIAN_POINT('Ctrl Pts',(-18.5658476086863,42.011356440193,124.273892910701)) ;
#94743=CARTESIAN_POINT('Ctrl Pts',(-18.428377019164,42.0214108348676,124.113388604921)) ;
#94744=CARTESIAN_POINT('Ctrl Pts',(-18.3228682434027,42.0312518962562,123.935378215502)) ;
#94745=CARTESIAN_POINT('Ctrl Pts',(-18.2480350752191,42.0413181206127,123.737465714565)) ;
#94746=CARTESIAN_POINT('Ctrl Pts',(-18.2094758284378,42.0511987335323,123.533319948566)) ;
#94747=CARTESIAN_POINT('Ctrl Pts',(-18.2065221821883,42.061192026692,123.323284104449)) ;
#94748=CARTESIAN_POINT('Ctrl Pts',(-18.2398729840911,42.0711430349156,123.116720737839)) ;
#94749=CARTESIAN_POINT('Ctrl Pts',(-18.30938960882,42.0811915492776,122.917259856404)) ;
#94750=CARTESIAN_POINT('Ctrl Pts',(-18.4101750659709,42.0910330553402,122.736544979461)) ;
#94751=CARTESIAN_POINT('Ctrl Pts',(-18.5423307667801,42.1010187079699,122.573475447401)) ;
#94752=CARTESIAN_POINT('Ctrl Pts',(-18.7000496850121,42.1109577168148,122.436369784685)) ;
#94753=CARTESIAN_POINT('Ctrl Pts',(-18.8809998458564,42.1209986421078,122.327702241158)) ;
#94754=CARTESIAN_POINT('Ctrl Pts',(-19.0751046604833,42.1308889638627,122.253109674576)) ;
#94755=CARTESIAN_POINT('Ctrl Pts',(-19.2812986190992,42.1408849371962,122.212630847308)) ;
#94756=CARTESIAN_POINT('Ctrl Pts',(-19.4900576064491,42.1508163367782,122.208578595215)) ;
#94757=CARTESIAN_POINT('Ctrl Pts',(-19.6979366331324,42.1608218772553,122.240781161984)) ;
#94758=CARTESIAN_POINT('Ctrl Pts',(-19.8974710441243,42.1708548611866,122.309135104057)) ;
#94759=CARTESIAN_POINT('Ctrl Pts',(-20.0790398796497,42.1807104920134,122.408984409925)) ;
#94760=CARTESIAN_POINT('Ctrl Pts',(-20.2429987707596,42.1907098942066,122.540492356409)) ;
#94761=CARTESIAN_POINT('Ctrl Pts',(-20.3804073459891,42.2006043635676,122.696711276599)) ;
#94762=CARTESIAN_POINT('Ctrl Pts',(-20.4903548587185,42.2106674777319,122.877413039077)) ;
#94763=CARTESIAN_POINT('Ctrl Pts',(-20.5657866675536,42.2205071234482,123.070066487545)) ;
#94764=CARTESIAN_POINT('Ctrl Pts',(-20.6078006806299,42.230570291004,123.27738258839)) ;
#94765=CARTESIAN_POINT('Ctrl Pts',(-20.6129143393689,42.2404645467989,123.485351033977)) ;
#94766=CARTESIAN_POINT('Ctrl Pts',(-20.5822609059887,42.2504063252585,123.692072376071)) ;
#94767=CARTESIAN_POINT('Ctrl Pts',(-20.5158291243726,42.2604090180887,123.891620705968)) ;
#94768=CARTESIAN_POINT('Ctrl Pts',(-20.41518049129,42.2704430400425,124.076996133679)) ;
#94769=CARTESIAN_POINT('Ctrl Pts',(-20.2865490886093,42.2802908311316,124.239226624219)) ;
#94770=CARTESIAN_POINT('Ctrl Pts',(-20.1299261416797,42.2902723556806,124.378854116596)) ;
#94771=CARTESIAN_POINT('Ctrl Pts',(-19.9519781208104,42.3002215791715,124.488795049372)) ;
#94772=CARTESIAN_POINT('Ctrl Pts',(-19.7567858429726,42.3102192353881,124.566794957214)) ;
#94773=CARTESIAN_POINT('Ctrl Pts',(-19.5500874564602,42.3202594484432,124.609497549694)) ;
#94774=CARTESIAN_POINT('Ctrl Pts',(-19.3435610736037,42.3300874957194,124.615984150951)) ;
#94775=CARTESIAN_POINT('Ctrl Pts',(-19.1343128394333,42.3401418427518,124.586163345048)) ;
#94776=CARTESIAN_POINT('Ctrl Pts',(-18.9357761772501,42.3500829790803,124.520862041799)) ;
#94777=CARTESIAN_POINT('Ctrl Pts',(-18.7519747205506,42.3599872121601,124.423017051762)) ;
#94778=CARTESIAN_POINT('Ctrl Pts',(-18.5856939199172,42.3700339090037,124.292809021581)) ;
#94779=CARTESIAN_POINT('Ctrl Pts',(-18.4464957962176,42.3799294602839,124.138158892235)) ;
#94780=CARTESIAN_POINT('Ctrl Pts',(-18.334443279754,42.3899915381234,123.958773214365)) ;
#94781=CARTESIAN_POINT('Ctrl Pts',(-18.256837301689,42.3998342472195,123.766927669182)) ;
#94782=CARTESIAN_POINT('Ctrl Pts',(-18.2125966969504,42.4098249794579,123.561630551405)) ;
#94783=CARTESIAN_POINT('Ctrl Pts',(-18.2047563018434,42.4197530046867,123.353048502693)) ;
#94784=CARTESIAN_POINT('Ctrl Pts',(-18.2330695475224,42.4297411513373,123.14497892533)) ;
#94785=CARTESIAN_POINT('Ctrl Pts',(-18.2976873818308,42.4397761691772,122.94414783446)) ;
#94786=CARTESIAN_POINT('Ctrl Pts',(-18.3943257711655,42.4496409662824,122.760659909047)) ;
#94787=CARTESIAN_POINT('Ctrl Pts',(-18.5221133525322,42.4596016986385,122.59475870461)) ;
#94788=CARTESIAN_POINT('Ctrl Pts',(-18.6781228036103,42.4696351610355,122.452804645446)) ;
#94789=CARTESIAN_POINT('Ctrl Pts',(-18.8536233329689,42.4795206952469,122.341445380712)) ;
#94790=CARTESIAN_POINT('Ctrl Pts',(-19.0492358131818,42.4895855359269,122.260840291009)) ;
#94791=CARTESIAN_POINT('Ctrl Pts',(-19.2514442452252,42.4994336676558,122.21630249578)) ;
#94792=CARTESIAN_POINT('Ctrl Pts',(-19.462035792714,42.5094611646459,122.206847322069)) ;
#94793=CARTESIAN_POINT('Ctrl Pts',(-19.6710341455677,42.519489616691,122.234659844104)) ;
#94794=CARTESIAN_POINT('Ctrl Pts',(-19.8684540475682,42.5293348832551,122.296792877154)) ;
#94795=CARTESIAN_POINT('Ctrl Pts',(-20.0550737957879,42.539325556196,122.39317911818)) ;
#94796=CARTESIAN_POINT('Ctrl Pts',(-20.2226209287262,42.5493634382845,122.521475154618)) ;
#94797=CARTESIAN_POINT('Ctrl Pts',(-20.3628676182926,42.5592078087242,122.673680073247)) ;
#94798=CARTESIAN_POINT('Ctrl Pts',(-20.4764790775102,42.5691926361195,122.850155943323)) ;
#94799=CARTESIAN_POINT('Ctrl Pts',(-20.5574622812338,42.5791320815248,123.042816214806)) ;
#94800=CARTESIAN_POINT('Ctrl Pts',(-20.6041616161675,42.5891720858107,123.248636405187)) ;
#94801=CARTESIAN_POINT('Ctrl Pts',(-20.6144023767689,42.5990591949964,123.456265586749)) ;
#94802=CARTESIAN_POINT('Ctrl Pts',(-20.5884050739317,42.6090592548988,123.664852226601)) ;
#94803=CARTESIAN_POINT('Ctrl Pts',(-20.527246558674,42.6189766708135,123.86421184067)) ;
#94804=CARTESIAN_POINT('Ctrl Pts',(-20.4311397333606,42.6290234855543,124.0522625542)) ;
#94805=CARTESIAN_POINT('Ctrl Pts',(-20.3061446920854,42.638898962751,124.218074754755)) ;
#94806=CARTESIAN_POINT('Ctrl Pts',(-20.1516108964613,42.6489550584722,124.362292436574)) ;
#94807=CARTESIAN_POINT('Ctrl Pts',(-19.9772349604992,42.6588482204873,124.475727074264)) ;
#94808=CARTESIAN_POINT('Ctrl Pts',(-19.7826262393279,42.6689104565099,124.558584685798)) ;
#94809=CARTESIAN_POINT('Ctrl Pts',(-19.5810180452714,42.6787549221389,124.605386432261)) ;
#94810=CARTESIAN_POINT('Ctrl Pts',(-19.3719712941627,42.688715014843,124.617355628047)) ;
#94811=CARTESIAN_POINT('Ctrl Pts',(-19.1624444705205,42.698753303824,124.592241358661)) ;
#94812=CARTESIAN_POINT('Ctrl Pts',(-18.963625683238,42.7086266269302,124.532502862756)) ;
#94813=CARTESIAN_POINT('Ctrl Pts',(-18.7745424256361,42.7186998110153,124.437233845792)) ;
#94814=CARTESIAN_POINT('Ctrl Pts',(-18.6088995425854,42.7285203233033,124.313922067836)) ;
#94815=CARTESIAN_POINT('Ctrl Pts',(-18.4633850738748,42.7385983194191,124.159993840772)) ;
#94816=CARTESIAN_POINT('Ctrl Pts',(-18.3493042720735,42.7484523944023,123.987014281055)) ;
#94817=CARTESIAN_POINT('Ctrl Pts',(-18.2650619448584,42.758516275986,123.792978353709)) ;
#94818=CARTESIAN_POINT('Ctrl Pts',(-18.2166935674385,42.7683997019598,123.590869324844)) ;
#94819=CARTESIAN_POINT('Ctrl Pts',(-18.2036737593463,42.7784003058808,123.381065517752)) ;
#94820=CARTESIAN_POINT('Ctrl Pts',(-18.2269667434619,42.7883200902187,123.173787221887)) ;
#94821=CARTESIAN_POINT('Ctrl Pts',(-18.2866812459217,42.7983674405756,122.971212989523)) ;
#94822=CARTESIAN_POINT('Ctrl Pts',(-18.3788851943168,42.8082447828098,122.785107699103)) ;
#94823=CARTESIAN_POINT('Ctrl Pts',(-18.5043642018314,42.8183146638845,122.614654132429)) ;
#94824=CARTESIAN_POINT('Ctrl Pts',(-18.653787444883,42.8281443690862,122.4718499437)) ;
#94825=CARTESIAN_POINT('Ctrl Pts',(-18.8296635825875,42.8382110302526,122.354200237369)) ;
#94826=CARTESIAN_POINT('Ctrl Pts',(-19.0200097310949,42.8481012521199,122.270467356892)) ;
#94827=CARTESIAN_POINT('Ctrl Pts',(-19.2239389577315,42.85809342823,122.220108591587)) ;
#94828=CARTESIAN_POINT('Ctrl Pts',(-19.4329190104502,42.8680562583427,122.206163568861)) ;
#94829=CARTESIAN_POINT('Ctrl Pts',(-19.6400001889169,42.877960470743,122.228059000419)) ;
#94830=CARTESIAN_POINT('Ctrl Pts',(-19.8432008513187,42.8880211848308,122.286655338728)) ;
#94831=CARTESIAN_POINT('Ctrl Pts',(-20.0291415866043,42.8978606878136,122.37737031045)) ;
#94832=CARTESIAN_POINT('Ctrl Pts',(-20.2004350174569,42.90792682638,122.501580182519)) ;
#94833=CARTESIAN_POINT('Ctrl Pts',(-20.3448645195168,42.9178093408661,122.650971714434)) ;
#94834=CARTESIAN_POINT('Ctrl Pts',(-20.4627595278798,42.9278016402216,122.824800696927)) ;
#94835=CARTESIAN_POINT('Ctrl Pts',(-20.5484179633364,42.937754707175,123.015743351538)) ;
#94836=CARTESIAN_POINT('Ctrl Pts',(-20.5999443450742,42.9477894153802,123.220298951895)) ;
#94837=CARTESIAN_POINT('Ctrl Pts',(-20.615102005062,42.9576776362844,123.427639323025)) ;
#94838=CARTESIAN_POINT('Ctrl Pts',(-20.5941477423262,42.9676720593148,123.636694524985)) ;
#94839=CARTESIAN_POINT('Ctrl Pts',(-20.5374094938443,42.977617398761,123.837931542936)) ;
#94840=CARTESIAN_POINT('Ctrl Pts',(-20.4469569944454,42.9875647433723,124.026493617296)) ;
#94841=CARTESIAN_POINT('Ctrl Pts',(-20.3237223456528,42.9976126387833,124.19805123647)) ;
#94842=CARTESIAN_POINT('Ctrl Pts',(-20.1757015216844,43.0074602842627,124.342795648031)) ;
#94843=CARTESIAN_POINT('Ctrl Pts',(-20.0031972602108,43.0174219981767,124.461528619492)) ;
#94844=CARTESIAN_POINT('Ctrl Pts',(-19.8112857189198,43.0274506224676,124.548856647514)) ;
#94845=CARTESIAN_POINT('Ctrl Pts',(-19.6095733787523,43.0373609831244,124.600973577748)) ;
#94846=CARTESIAN_POINT('Ctrl Pts',(-19.4013914837202,43.0472956816976,124.617866016103)) ;
#94847=CARTESIAN_POINT('Ctrl Pts',(-19.1912337061601,43.0573375065518,124.597937775619)) ;
#94848=CARTESIAN_POINT('Ctrl Pts',(-18.9908384089771,43.0672220802963,124.542869343014)) ;
#94849=CARTESIAN_POINT('Ctrl Pts',(-18.8007562850313,43.0772239296594,124.453033636457)) ;
#94850=CARTESIAN_POINT('Ctrl Pts',(-18.6304420312896,43.0871432312335,124.332653761318)) ;
#94851=CARTESIAN_POINT('Ctrl Pts',(-18.4817976082182,43.0971873395787,124.182701681001)) ;
#94852=CARTESIAN_POINT('Ctrl Pts',(-18.3632946191163,43.107071763021,124.01199028503)) ;
#94853=CARTESIAN_POINT('Ctrl Pts',(-18.2746464092805,43.1170881249304,123.820975075702)) ;
#94854=CARTESIAN_POINT('Ctrl Pts',(-18.2209433761901,43.1271247804358,123.616933265616)) ;
#94855=CARTESIAN_POINT('Ctrl Pts',(-18.2032793807501,43.1369549106252,123.411004657846)) ;
#94856=CARTESIAN_POINT('Ctrl Pts',(-18.2220212330491,43.147030963715,123.200045552597)) ;
#94857=CARTESIAN_POINT('Ctrl Pts',(-18.2757963269349,43.1568831929008,122.99997816041)) ;
#94858=CARTESIAN_POINT('Ctrl Pts',(-18.3652659275181,43.1669564007001,122.808072809261)) ;
#94859=CARTESIAN_POINT('Ctrl Pts',(-18.4839780874204,43.1767979120515,122.638602038038)) ;
#94860=CARTESIAN_POINT('Ctrl Pts',(-18.6315156023104,43.1867588500891,122.49000028128)) ;
#94861=CARTESIAN_POINT('Ctrl Pts',(-18.8041793061524,43.196796712014,122.36868648056)) ;
#94862=CARTESIAN_POINT('Ctrl Pts',(-18.9920325642784,43.2066708980111,122.28028983119)) ;
#94863=CARTESIAN_POINT('Ctrl Pts',(-19.1963083903937,43.216741057589,122.224806544877)) ;
#94864=CARTESIAN_POINT('Ctrl Pts',(-19.4021609754784,43.2265728050148,122.205953810551)) ;
#94865=CARTESIAN_POINT('Ctrl Pts',(-19.6124556219852,43.2366088850861,122.222937571931)) ;
#94866=CARTESIAN_POINT('Ctrl Pts',(-19.8161059672516,43.2466259319386,122.276596411569)) ;
#94867=CARTESIAN_POINT('Ctrl Pts',(-20.0049292539503,43.2565081901052,122.363254712889)) ;
#94868=CARTESIAN_POINT('Ctrl Pts',(-20.1777775594488,43.2664958729016,122.482430141182)) ;
#94869=CARTESIAN_POINT('Ctrl Pts',(-20.3268505573778,43.2764425296183,122.629119299835)) ;
#94870=CARTESIAN_POINT('Ctrl Pts',(-20.4493262829934,43.2864995876985,122.801435822179)) ;
#94871=CARTESIAN_POINT('Ctrl Pts',(-20.5381405109259,43.2963177672479,122.987771862628)) ;
#94872=CARTESIAN_POINT('Ctrl Pts',(-20.5950205275203,43.3063537016869,123.190941543004)) ;
#94873=CARTESIAN_POINT('Ctrl Pts',(-20.6151355410267,43.3163783561159,123.400737110765)) ;
#94874=CARTESIAN_POINT('Ctrl Pts',(-20.5992612078394,43.3262303756954,123.607251294915)) ;
#94875=CARTESIAN_POINT('Ctrl Pts',(-20.5473617854122,43.3362212894104,123.810752806261)) ;
#94876=CARTESIAN_POINT('Ctrl Pts',(-20.4616503408457,43.3461392782499,124.000855965883)) ;
#94877=CARTESIAN_POINT('Ctrl Pts',(-20.3429941407184,43.3561673889807,124.17509705493)) ;
#94878=CARTESIAN_POINT('Ctrl Pts',(-20.1980312069958,43.3660525868891,124.324012622826)) ;
#94879=CARTESIAN_POINT('Ctrl Pts',(-20.0279376979557,43.3760418621571,124.447192060781)) ;
#94880=CARTESIAN_POINT('Ctrl Pts',(-19.8378630919995,43.3860833203266,124.539030412426)) ;
#94881=CARTESIAN_POINT('Ctrl Pts',(-19.6390701343716,43.395914784115,124.595638016482)) ;
#94882=CARTESIAN_POINT('Ctrl Pts',(-19.4299207018962,43.4059197164188,124.617705082687)) ;
#94883=CARTESIAN_POINT('Ctrl Pts',(-19.2204529483863,43.4159060803136,124.603030015181)) ;
#94884=CARTESIAN_POINT('Ctrl Pts',(-19.0159260281216,43.4259357091994,124.551840172303)) ;
#94885=CARTESIAN_POINT('Ctrl Pts',(-18.8262138021633,43.4358109313078,124.46746772505)) ;
#94886=CARTESIAN_POINT('Ctrl Pts',(-18.6517412398337,43.4458121437049,124.35019270089)) ;
#94887=CARTESIAN_POINT('Ctrl Pts',(-18.5014974666198,43.4557207229405,124.205849688173)) ;
#94888=CARTESIAN_POINT('Ctrl Pts',(-18.3768780504373,43.4657755754965,124.035148132085)) ;
#94889=CARTESIAN_POINT('Ctrl Pts',(-18.2853633360531,43.4756341577712,123.849147653433)) ;
#94890=CARTESIAN_POINT('Ctrl Pts',(-18.2262007819212,43.4857022872139,123.645952408235)) ;
#94891=CARTESIAN_POINT('Ctrl Pts',(-18.2037152670099,43.495557758903,123.439965689953)) ;
#94892=CARTESIAN_POINT('Ctrl Pts',(-18.2168996606046,43.5055526072893,123.230263419917)) ;
#94893=CARTESIAN_POINT('Ctrl Pts',(-18.2669194341459,43.5155839040738,123.025387393044)) ;
#94894=CARTESIAN_POINT('Ctrl Pts',(-18.350057379065,43.5254504402838,122.835344588144)) ;
#94895=CARTESIAN_POINT('Ctrl Pts',(-18.4660377808378,43.5354378632447,122.660345763407)) ;
#94896=CARTESIAN_POINT('Ctrl Pts',(-18.6099846283068,43.5453828022644,122.50867783323)) ;
#94897=CARTESIAN_POINT('Ctrl Pts',(-18.7797941808117,43.5554276881244,122.383164603067)) ;
#94898=CARTESIAN_POINT('Ctrl Pts',(-18.9654667474152,43.5652962232107,122.290585226605)) ;
#94899=CARTESIAN_POINT('Ctrl Pts',(-19.166175253621,43.5752620912173,122.23051446461)) ;
#94900=CARTESIAN_POINT('Ctrl Pts',(-19.3755016238856,43.5852847386698,122.206300298283)) ;
#94901=CARTESIAN_POINT('Ctrl Pts',(-19.5837529479575,43.5952083776774,122.218617123038)) ;
#94902=CARTESIAN_POINT('Ctrl Pts',(-19.7872305435204,43.6051511026832,122.266516185688)) ;
#94903=CARTESIAN_POINT('Ctrl Pts',(-19.9811658118431,43.615196708735,122.350095121641)) ;
#94904=CARTESIAN_POINT('Ctrl Pts',(-20.1545571238917,43.6250581312561,122.463777132953)) ;
#94905=CARTESIAN_POINT('Ctrl Pts',(-20.3078102197578,43.6350516997053,122.607448076421)) ;
#94906=CARTESIAN_POINT('Ctrl Pts',(-20.4330542470153,43.6449771704606,122.774384365223)) ;
#94907=CARTESIAN_POINT('Ctrl Pts',(-20.5283647810184,43.6550048444165,122.962392977543)) ;
#94908=CARTESIAN_POINT('Ctrl Pts',(-20.5889338449823,43.6648920224582,123.161260964783)) ;
#94909=CARTESIAN_POINT('Ctrl Pts',(-20.6145511613344,43.6749204018264,123.370499311071)) ;
#94910=CARTESIAN_POINT('Ctrl Pts',(-20.603708283792,43.6848146445478,123.57824797087)) ;
#94911=CARTESIAN_POINT('Ctrl Pts',(-20.5408575434125,43.6981675611987,123.851835425045)) ;
#94912=CARTESIAN_POINT('Ctrl Pts',(-20.4095228170576,43.7113700789455,124.100006492089)) ;
#94913=CARTESIAN_POINT('Ctrl Pts',(-20.2186590844846,43.7247259842264,124.30584947481)) ;
#94914=CARTESIAN_POINT('Ctrl Pts',(-20.0529407367941,43.7346226328643,124.431709404068)) ;
#94915=CARTESIAN_POINT('Ctrl Pts',(-19.8651333436592,43.7446707709167,124.528373384689)) ;
#94916=CARTESIAN_POINT('Ctrl Pts',(-19.6665214527056,43.7545617310945,124.589983515825)) ;
#94917=CARTESIAN_POINT('Ctrl Pts',(-19.4581739203183,43.7645545669713,124.616965017307)) ;
#94918=CARTESIAN_POINT('Ctrl Pts',(-19.2473737691811,43.7745936619728,124.606831454262)) ;
#94919=CARTESIAN_POINT('Ctrl Pts',(-19.0455363121503,43.784431017824,124.561650497057)) ;
#94920=CARTESIAN_POINT('Ctrl Pts',(-18.7855906921791,43.7978239657547,124.453535628183)) ;
#94921=CARTESIAN_POINT('Ctrl Pts',(-18.5635139422216,43.8109906421817,124.282902191796)) ;
#94922=CARTESIAN_POINT('Ctrl Pts',(-18.3921555658983,43.8243754235884,124.05982076316)) ;
#94923=CARTESIAN_POINT('Ctrl Pts',(-18.2962311864038,43.8342372062323,123.875972351288)) ;
#94924=CARTESIAN_POINT('Ctrl Pts',(-18.2325177060846,43.8442363541853,123.675693020138)) ;
#94925=CARTESIAN_POINT('Ctrl Pts',(-18.2046131430209,43.8541391468024,123.46933726225)) ;
#94926=CARTESIAN_POINT('Ctrl Pts',(-18.2131381453431,43.8641887266934,123.258291456471)) ;
#94927=CARTESIAN_POINT('Ctrl Pts',(-18.2717478838939,43.8773758005028,122.987197867203)) ;
#94928=CARTESIAN_POINT('Ctrl Pts',(-18.4346578307406,43.894128590474,122.670626737531)) ;
#94929=CARTESIAN_POINT('Ctrl Pts',(-18.6920466360006,43.9106172425687,122.432275019255)) ;
#94930=CARTESIAN_POINT('Ctrl Pts',(-18.9400675272099,43.9239740687521,122.300862325712)) ;
#94931=CARTESIAN_POINT('Ctrl Pts',(-19.1380510126641,43.9338704536301,122.236740383754)) ;
#94932=CARTESIAN_POINT('Ctrl Pts',(-19.3463246739333,43.9438769681505,122.207560048397)) ;
#94933=CARTESIAN_POINT('Ctrl Pts',(-19.6235856775625,43.9570670916669,122.216668870961)) ;
#94934=CARTESIAN_POINT('Ctrl Pts',(-19.9644818436407,43.9738336528165,122.320510334503)) ;
#94935=CARTESIAN_POINT('Ctrl Pts',(-20.3009628920008,43.9936181415245,122.573194359598)) ;
#94936=CARTESIAN_POINT('Ctrl Pts',(-20.5338593579288,44.013563589121,122.927488610448)) ;
#94937=CARTESIAN_POINT('Ctrl Pts',(-20.6313432900852,44.0334752512769,123.339498293357)) ;
#94938=CARTESIAN_POINT('Ctrl Pts',(-20.5833486167225,44.0533674432958,123.759794144768)) ;
#94939=CARTESIAN_POINT('Ctrl Pts',(-20.3928831509426,44.0734085738504,124.140920763772)) ;
#94940=CARTESIAN_POINT('Ctrl Pts',(-20.0872651227944,44.093226908466,124.431188469876)) ;
#94941=CARTESIAN_POINT('Ctrl Pts',(-19.6984333457732,44.1131994736856,124.601580100911)) ;
#94942=CARTESIAN_POINT('Ctrl Pts',(-19.2762687397461,44.1330886898572,124.629069312645)) ;
#94943=CARTESIAN_POINT('Ctrl Pts',(-18.8676587652594,44.1531122641799,124.509843388215)) ;
#94944=CARTESIAN_POINT('Ctrl Pts',(-18.5278179721396,44.1729094272682,124.261320737249)) ;
#94945=CARTESIAN_POINT('Ctrl Pts',(-18.2904317837081,44.1928749210919,123.909483288494)) ;
#94946=CARTESIAN_POINT('Ctrl Pts',(-18.1878781194109,44.2128286288334,123.497677701011)) ;
#94947=CARTESIAN_POINT('Ctrl Pts',(-18.2318638131071,44.23273600556,123.076779952571)) ;
#94948=CARTESIAN_POINT('Ctrl Pts',(-18.4153837347408,44.2525882171085,122.696570104589)) ;
#94949=CARTESIAN_POINT('Ctrl Pts',(-18.7212134876534,44.2726606040542,122.398901422161)) ;
#94950=CARTESIAN_POINT('Ctrl Pts',(-19.1059666063529,44.2924984736945,122.226014999044)) ;
#94951=CARTESIAN_POINT('Ctrl Pts',(-19.5267471998441,44.3123491282477,122.192956248607)) ;
#94952=CARTESIAN_POINT('Ctrl Pts',(-19.9374778624856,44.3324010625881,122.30720495541)) ;
#94953=CARTESIAN_POINT('Ctrl Pts',(-20.2808529206033,44.3522342501541,122.552178926916)) ;
#94954=CARTESIAN_POINT('Ctrl Pts',(-20.5217266142263,44.3721634623848,122.900618714666)) ;
#94955=CARTESIAN_POINT('Ctrl Pts',(-20.6295648554186,44.3920484275992,123.309611341229)) ;
#94956=CARTESIAN_POINT('Ctrl Pts',(-20.5903665695791,44.4121221687438,123.734542200108)) ;
#94957=CARTESIAN_POINT('Ctrl Pts',(-20.4110378863135,44.4319153505242,124.115354713152)) ;
#94958=CARTESIAN_POINT('Ctrl Pts',(-20.1109493418059,44.4518780585269,124.415495408752)) ;
#94959=CARTESIAN_POINT('Ctrl Pts',(-19.7255902485524,44.4718610102694,124.594483394183)) ;
#94960=CARTESIAN_POINT('Ctrl Pts',(-19.3059766594542,44.4916716300415,124.631738877851)) ;
#94961=CARTESIAN_POINT('Ctrl Pts',(-18.8952789795798,44.5116553460744,124.523139920647)) ;
#94962=CARTESIAN_POINT('Ctrl Pts',(-18.5479537567652,44.5315368099717,124.28197871897)) ;
#94963=CARTESIAN_POINT('Ctrl Pts',(-18.3027327952688,44.5514921398161,123.935816420611)) ;
#94964=CARTESIAN_POINT('Ctrl Pts',(-18.1904707624219,44.5713676006216,123.528324021289)) ;
#94965=CARTESIAN_POINT('Ctrl Pts',(-18.2239254020228,44.5913519206731,123.104770226885)) ;
#94966=CARTESIAN_POINT('Ctrl Pts',(-18.3996904677657,44.6112799534628,122.71911120197)) ;
#94967=CARTESIAN_POINT('Ctrl Pts',(-18.6468965142443,44.6278887154025,122.467053011659)) ;
#94968=CARTESIAN_POINT('Ctrl Pts',(-18.8854150868298,44.6410763540926,122.32564319516)) ;
#94969=CARTESIAN_POINT('Ctrl Pts',(-19.0816688013698,44.6510627884528,122.251110504888)) ;
#94970=CARTESIAN_POINT('Ctrl Pts',(-19.2884344373437,44.6610721624121,122.211902195328)) ;
#94971=CARTESIAN_POINT('Ctrl Pts',(-19.5677616553926,44.6743621959774,122.208107590345)) ;
#94972=CARTESIAN_POINT('Ctrl Pts',(-19.909946568067,44.6909561836399,122.294466869324)) ;
#94973=CARTESIAN_POINT('Ctrl Pts',(-20.2026693922946,44.7075884389154,122.492797225526)) ;
#94974=CARTESIAN_POINT('Ctrl Pts',(-20.3849910652847,44.7208308225832,122.703234545507)) ;
#94975=CARTESIAN_POINT('Ctrl Pts',(-20.4925937469405,44.7307450308107,122.881741651042)) ;
#94976=CARTESIAN_POINT('Ctrl Pts',(-20.5684167531968,44.7408016700823,123.079084895041)) ;
#94977=CARTESIAN_POINT('Ctrl Pts',(-20.6082256062744,44.7506474765025,123.282226426836)) ;
#94978=CARTESIAN_POINT('Ctrl Pts',(-20.612596699093,44.7606924761356,123.4933577631)) ;
#94979=CARTESIAN_POINT('Ctrl Pts',(-20.5694218883815,44.7739734985084,123.769153441609)) ;
#94980=CARTESIAN_POINT('Ctrl Pts',(-20.4566672831877,44.787170945033,124.026150744995)) ;
#94981=CARTESIAN_POINT('Ctrl Pts',(-20.2801264821268,44.80058524284,124.246100686113)) ;
#94982=CARTESIAN_POINT('Ctrl Pts',(-20.1246823390785,44.8104243082428,124.382580125368)) ;
#94983=CARTESIAN_POINT('Ctrl Pts',(-19.9456254369474,44.8204075145204,124.492026841846)) ;
#94984=CARTESIAN_POINT('Ctrl Pts',(-19.7508537581695,44.8303587494332,124.568420993934)) ;
#94985=CARTESIAN_POINT('Ctrl Pts',(-19.5448027338605,44.8403597491349,124.610291848731)) ;
#94986=CARTESIAN_POINT('Ctrl Pts',(-19.3339773939872,44.8503910949222,124.615434702964)) ;
#94987=CARTESIAN_POINT('Ctrl Pts',(-19.1291026875363,44.8602448596272,124.584732769678)) ;
#94988=CARTESIAN_POINT('Ctrl Pts',(-18.9302085569886,44.8702155132955,124.518626229001)) ;
#94989=CARTESIAN_POINT('Ctrl Pts',(-18.7452782875516,44.8802127569528,124.418690892324)) ;
#94990=CARTESIAN_POINT('Ctrl Pts',(-18.5801193571764,44.8902462128969,124.287508814741)) ;
#94991=CARTESIAN_POINT('Ctrl Pts',(-18.4424514262048,44.9001017171973,124.132637434498)) ;
#94992=CARTESIAN_POINT('Ctrl Pts',(-18.3319695722202,44.9101011534834,123.953834850659)) ;
#94993=CARTESIAN_POINT('Ctrl Pts',(-18.2547793540301,44.9199956129993,123.760632273683)) ;
#94994=CARTESIAN_POINT('Ctrl Pts',(-18.211660949245,44.930058732451,123.553551718447)) ;
#94995=CARTESIAN_POINT('Ctrl Pts',(-18.2050676049964,44.939898366863,123.346762420649)) ;
#94996=CARTESIAN_POINT('Ctrl Pts',(-18.2348732987409,44.9499615743488,123.137341924846)) ;
#94997=CARTESIAN_POINT('Ctrl Pts',(-18.2996654380059,44.9598556817279,122.939659991958)) ;
#94998=CARTESIAN_POINT('Ctrl Pts',(-18.3977574562744,44.9697980139203,122.755119782412)) ;
#94999=CARTESIAN_POINT('Ctrl Pts',(-18.5271124178291,44.9797986402353,122.58933669533)) ;
#95000=CARTESIAN_POINT('Ctrl Pts',(-18.6841544980773,44.9898403745172,122.448281242363)) ;
#95001=CARTESIAN_POINT('Ctrl Pts',(-18.859229594049,44.9996658004663,122.338633544049)) ;
#95002=CARTESIAN_POINT('Ctrl Pts',(-19.0550454607519,45.009722626994,122.258943891546)) ;
#95003=CARTESIAN_POINT('Ctrl Pts',(-19.2591518340344,45.0196500601156,122.215318487338)) ;
#95004=CARTESIAN_POINT('Ctrl Pts',(-19.4681812808614,45.0296000525218,122.207180133437)) ;
#95005=CARTESIAN_POINT('Ctrl Pts',(-19.6775673181932,45.0396552535958,122.2361259376)) ;
#95006=CARTESIAN_POINT('Ctrl Pts',(-19.8742295207309,45.0494775276481,122.299140357203)) ;
#95007=CARTESIAN_POINT('Ctrl Pts',(-20.0614575634697,45.0595334216073,122.397284057892)) ;
#95008=CARTESIAN_POINT('Ctrl Pts',(-20.226674164749,45.0694741434525,122.525274601464)) ;
#95009=CARTESIAN_POINT('Ctrl Pts',(-20.3671232498211,45.079378487539,122.678999528342)) ;
#95010=CARTESIAN_POINT('Ctrl Pts',(-20.4802264787641,45.0894251548385,122.857355770143)) ;
#95011=CARTESIAN_POINT('Ctrl Pts',(-20.5596285796948,45.0993207132885,123.049678684539)) ;
#95012=CARTESIAN_POINT('Ctrl Pts',(-20.605171036414,45.1093827919931,123.256223873062)) ;
#95013=CARTESIAN_POINT('Ctrl Pts',(-20.6140833446589,45.1192254904589,123.462979282518)) ;
#95014=CARTESIAN_POINT('Ctrl Pts',(-20.587052536111,45.1292162643534,123.671243804654)) ;
#95015=CARTESIAN_POINT('Ctrl Pts',(-20.5246209802578,45.1391441335883,123.870412103344)) ;
#95016=CARTESIAN_POINT('Ctrl Pts',(-20.4282957923679,45.1491328625582,124.057023143126)) ;
#95017=CARTESIAN_POINT('Ctrl Pts',(-20.300088730677,45.1591722645419,124.224668107003)) ;
#95018=CARTESIAN_POINT('Ctrl Pts',(-20.1480643896778,45.1690124322787,124.364985798958)) ;
#95019=CARTESIAN_POINT('Ctrl Pts',(-19.9704897857701,45.1790606426532,124.479388556005)) ;
#95020=CARTESIAN_POINT('Ctrl Pts',(-19.7775671927321,45.189007812941,124.560097139882)) ;
#95021=CARTESIAN_POINT('Ctrl Pts',(-19.5744414816242,45.198918661196,124.606523875413)) ;
#95022=CARTESIAN_POINT('Ctrl Pts',(-19.3632945233948,45.2089749888738,124.616929811313)) ;
#95023=CARTESIAN_POINT('Ctrl Pts',(-19.1577990703498,45.2188254016423,124.591231954316)) ;
#95024=CARTESIAN_POINT('Ctrl Pts',(-18.9562025405331,45.228852287476,124.529644851264)) ;
#95025=CARTESIAN_POINT('Ctrl Pts',(-18.7685671992907,45.2388809031068,124.433479713796)) ;
#95026=CARTESIAN_POINT('Ctrl Pts',(-18.6033345212596,45.2487261264844,124.308847809441)) ;
#95027=CARTESIAN_POINT('Ctrl Pts',(-18.4597435365736,45.2587168085859,124.155554340347)) ;
#95028=CARTESIAN_POINT('Ctrl Pts',(-18.3448064981045,45.2687546972184,123.978575669867)) ;
#95029=CARTESIAN_POINT('Ctrl Pts',(-18.2635978150533,45.2785990323215,123.788206668154)) ;
#95030=CARTESIAN_POINT('Ctrl Pts',(-18.2156129207493,45.2885839945191,123.583878862272)) ;
#95031=CARTESIAN_POINT('Ctrl Pts',(-18.2037886149857,45.2985229360524,123.375235476111)) ;
#95032=CARTESIAN_POINT('Ctrl Pts',(-18.2286862668487,45.3085648210239,123.165616917529)) ;
#95033=CARTESIAN_POINT('Ctrl Pts',(-18.2885437806197,45.3184513689321,122.966555293898)) ;
#95034=CARTESIAN_POINT('Ctrl Pts',(-18.3827734035262,45.3284452944321,122.778797331814)) ;
#95035=CARTESIAN_POINT('Ctrl Pts',(-18.5074028841177,45.3383813855586,122.611122603817)) ;
#95036=CARTESIAN_POINT('Ctrl Pts',(-18.6606617419149,45.3484106545385,122.466359785052)) ;
#95037=CARTESIAN_POINT('Ctrl Pts',(-18.8340526690746,45.3582930370979,122.351852199141)) ;
#95038=CARTESIAN_POINT('Ctrl Pts',(-19.0278880503773,45.3683455541857,122.267728236563)) ;
#95039=CARTESIAN_POINT('Ctrl Pts',(-19.2301906008237,45.3782396750096,122.219193863499)) ;
#95040=CARTESIAN_POINT('Ctrl Pts',(-19.4413039174828,45.38830165443,122.206261136697)) ;
#95041=CARTESIAN_POINT('Ctrl Pts',(-19.6469491825146,45.398146187659,122.229642978978)) ;
#95042=CARTESIAN_POINT('Ctrl Pts',(-19.8479428991622,45.4081062665652,122.288339189176)) ;
#95043=CARTESIAN_POINT('Ctrl Pts',(-20.0369764252112,45.4181445431378,122.382139581479)) ;
#95044=CARTESIAN_POINT('Ctrl Pts',(-20.2043294392257,45.4280179296757,122.504984302284)) ;
#95045=CARTESIAN_POINT('Ctrl Pts',(-20.3506163047683,45.4380908724427,122.658044774767)) ;
#95046=CARTESIAN_POINT('Ctrl Pts',(-20.4654246636601,45.4479122865711,122.829707674771)) ;
#95047=CARTESIAN_POINT('Ctrl Pts',(-20.5510305647617,45.4579869166434,123.023395197919)) ;
#95048=CARTESIAN_POINT('Ctrl Pts',(-20.6005900616309,45.4678535539602,123.224841786073)) ;
#95049=CARTESIAN_POINT('Ctrl Pts',(-20.6151763361897,45.477877099332,123.43505318199)) ;
#95050=CARTESIAN_POINT('Ctrl Pts',(-20.5925286407093,45.4879028508492,123.644618706423)) ;
#95051=CARTESIAN_POINT('Ctrl Pts',(-20.535184701194,45.4977564378586,123.843665059279)) ;
#95052=CARTESIAN_POINT('Ctrl Pts',(-20.4435052359796,45.5077333980865,124.032319483579)) ;
#95053=CARTESIAN_POINT('Ctrl Pts',(-20.3196371816528,45.517754541115,124.202720679813)) ;
#95054=CARTESIAN_POINT('Ctrl Pts',(-20.1704223024116,45.5276371471349,124.347330357567)) ;
#95055=CARTESIAN_POINT('Ctrl Pts',(-19.9951347534933,45.5377056177676,124.46592141779)) ;
#95056=CARTESIAN_POINT('Ctrl Pts',(-19.80652763825,45.5475357009513,124.55047845137)) ;
#95057=CARTESIAN_POINT('Ctrl Pts',(-19.6014167542772,45.5576022606317,124.602468011462)) ;
#95058=CARTESIAN_POINT('Ctrl Pts',(-19.3940227762553,45.5674925104609,124.617656228685)) ;
#95059=CARTESIAN_POINT('Ctrl Pts',(-19.1850009207313,45.5774846762097,124.596848277277)) ;
#95060=CARTESIAN_POINT('Ctrl Pts',(-18.9834082543819,45.5874475198058,124.540036396267)) ;
#95061=CARTESIAN_POINT('Ctrl Pts',(-18.7956023609983,45.5973516886336,124.45008818612)) ;
#95062=CARTESIAN_POINT('Ctrl Pts',(-18.623736295235,45.6074125635279,124.326851256807)) ;
#95063=CARTESIAN_POINT('Ctrl Pts',(-18.4788923126259,45.6172514668573,124.179140534936)) ;
#95064=CARTESIAN_POINT('Ctrl Pts',(-18.3590375189782,45.6273198432312,124.004715614886)) ;
#95065=CARTESIAN_POINT('Ctrl Pts',(-18.2729630465884,45.6372004598639,123.815633502549)) ;
#95066=CARTESIAN_POINT('Ctrl Pts',(-18.2200510520963,45.6471916200928,123.612393264672)) ;
#95067=CARTESIAN_POINT('Ctrl Pts',(-18.2032574681038,45.6571446935249,123.403791977135)) ;
#95068=CARTESIAN_POINT('Ctrl Pts',(-18.2231668387161,45.6671805291376,123.193765820803)) ;
#95069=CARTESIAN_POINT('Ctrl Pts',(-18.278298264541,45.6770706558677,122.99327332114)) ;
#95070=CARTESIAN_POINT('Ctrl Pts',(-18.3680085171694,45.6870628376371,122.80333742584)) ;
#95071=CARTESIAN_POINT('Ctrl Pts',(-18.4888375636561,45.6970087776115,122.632688971449)) ;
#95072=CARTESIAN_POINT('Ctrl Pts',(-18.637188992051,45.706955961371,122.485285003098)) ;
#95073=CARTESIAN_POINT('Ctrl Pts',(-18.8107406957346,45.7170038996613,122.364873637851)) ;
#95074=CARTESIAN_POINT('Ctrl Pts',(-18.9986732175206,45.7268515344749,122.278026568986)) ;
#95075=CARTESIAN_POINT('Ctrl Pts',(-19.2009699760855,45.7368132481728,122.22388545414)) ;
#95076=CARTESIAN_POINT('Ctrl Pts',(-19.4110424427331,45.746841883994,122.205834191296)) ;
#95077=CARTESIAN_POINT('Ctrl Pts',(-19.6185632243262,45.7567521987458,122.224242549515)) ;
#95078=CARTESIAN_POINT('Ctrl Pts',(-19.820392725705,45.7666870694084,122.278012302123)) ;
#95079=CARTESIAN_POINT('Ctrl Pts',(-20.0117473837365,45.7767282518102,122.367127706858)) ;
#95080=CARTESIAN_POINT('Ctrl Pts',(-20.1821838127246,45.7866152232749,122.486134490758)) ;
#95081=CARTESIAN_POINT('Ctrl Pts',(-20.3311987926498,45.7966146555375,122.634375510774)) ;
#95082=CARTESIAN_POINT('Ctrl Pts',(-20.4513952143733,45.8065347207942,122.804835855089)) ;
#95083=CARTESIAN_POINT('Ctrl Pts',(-20.5412360456862,45.8165715733783,122.995747910381)) ;
#95084=CARTESIAN_POINT('Ctrl Pts',(-20.5958772836658,45.8264842327183,123.196855969057)) ;
#95085=CARTESIAN_POINT('Ctrl Pts',(-20.615375050569,45.8364754446332,123.406008392214)) ;
#95086=CARTESIAN_POINT('Ctrl Pts',(-20.5977036104295,45.8465170860363,123.616357719273)) ;
#95087=CARTESIAN_POINT('Ctrl Pts',(-20.5454116666777,45.8563458802434,123.816292415274)) ;
#95088=CARTESIAN_POINT('Ctrl Pts',(-20.4571378687505,45.8664222913646,124.008815830626)) ;
#95089=CARTESIAN_POINT('Ctrl Pts',(-20.3394955135026,45.8762744244071,124.179339825008)) ;
#95090=CARTESIAN_POINT('Ctrl Pts',(-20.1909503753333,45.8863476587484,124.330227006031)) ;
#95091=CARTESIAN_POINT('Ctrl Pts',(-20.0223590773789,45.896189160075,124.45018473356)) ;
#95092=CARTESIAN_POINT('Ctrl Pts',(-19.8335905381555,45.9061501116698,124.540828594865)) ;
#95093=CARTESIAN_POINT('Ctrl Pts',(-19.6302804589424,45.9161879293905,124.597348541929)) ;
#95094=CARTESIAN_POINT('Ctrl Pts',(-19.4236714959756,45.9260622786475,124.617764021895)) ;
#95095=CARTESIAN_POINT('Ctrl Pts',(-19.2126193484243,45.9361318293897,124.601674276228)) ;
#95096=CARTESIAN_POINT('Ctrl Pts',(-19.0122873115152,45.9459658488983,124.550514505087)) ;
#95097=CARTESIAN_POINT('Ctrl Pts',(-18.8198465129963,45.9560000034779,124.464134660922)) ;
#95098=CARTESIAN_POINT('Ctrl Pts',(-18.6459181894139,45.9660159293003,124.345423530653)) ;
#95099=CARTESIAN_POINT('Ctrl Pts',(-18.4970009713093,45.9758981844946,124.20055280957)) ;
#95100=CARTESIAN_POINT('Ctrl Pts',(-18.3739944783542,45.9858869910055,124.030382117797)) ;
#95101=CARTESIAN_POINT('Ctrl Pts',(-18.2826051031244,45.9958355582682,123.842218571449)) ;
#95102=CARTESIAN_POINT('Ctrl Pts',(-18.224895071071,46.0058903635702,123.638888686045)) ;
#95103=CARTESIAN_POINT('Ctrl Pts',(-18.2035713061239,46.0157091468338,123.433561311371)) ;
#95104=CARTESIAN_POINT('Ctrl Pts',(-18.2179813427917,46.0257449191944,123.223075314158)) ;
#95105=CARTESIAN_POINT('Ctrl Pts',(-18.2692515836051,46.035769618223,123.018648178243)) ;
#95106=CARTESIAN_POINT('Ctrl Pts',(-18.3533370643761,46.0456216214821,122.829360944997)) ;
#95107=CARTESIAN_POINT('Ctrl Pts',(-18.4703613636276,46.0556125558793,122.654971111735)) ;
#95108=CARTESIAN_POINT('Ctrl Pts',(-18.6147606274529,46.0655304783104,122.504524563448)) ;
#95109=CARTESIAN_POINT('Ctrl Pts',(-18.7849011160605,46.0755588339928,122.380053433214)) ;
#95110=CARTESIAN_POINT('Ctrl Pts',(-18.9713293181431,46.0854431185033,122.288249837825)) ;
#95111=CARTESIAN_POINT('Ctrl Pts',(-19.1729140808588,46.0954358024112,122.229120011602)) ;
#95112=CARTESIAN_POINT('Ctrl Pts',(-19.3824991169952,46.1054645394189,122.206173308902)) ;
#95113=CARTESIAN_POINT('Ctrl Pts',(-19.5899010934406,46.1153499360478,122.219495008975)) ;
#95114=CARTESIAN_POINT('Ctrl Pts',(-19.7939762330509,46.1253378214617,122.268837873898)) ;
#95115=CARTESIAN_POINT('Ctrl Pts',(-19.9857528109284,46.1352885241223,122.352485218337)) ;
#95116=CARTESIAN_POINT('Ctrl Pts',(-20.161556069214,46.1453288422197,122.469269469153)) ;
#95117=CARTESIAN_POINT('Ctrl Pts',(-20.3120617664578,46.155203407553,122.612283972621)) ;
#95118=CARTESIAN_POINT('Ctrl Pts',(-20.4371930752356,46.165203067614,122.781168558695)) ;
#95119=CARTESIAN_POINT('Ctrl Pts',(-20.5304591803611,46.1751120627818,122.967483465853)) ;
#95120=CARTESIAN_POINT('Ctrl Pts',(-20.5907489831864,46.185166803945,123.170050000075)) ;
#95121=CARTESIAN_POINT('Ctrl Pts',(-20.6147246475824,46.1950254158588,123.375954151209)) ;
#95122=CARTESIAN_POINT('Ctrl Pts',(-20.602458271204,46.2050935381382,123.587231216781)) ;
#95123=CARTESIAN_POINT('Ctrl Pts',(-20.55469644977,46.2149490088413,123.788861901964)) ;
#95124=CARTESIAN_POINT('Ctrl Pts',(-20.4720783460226,46.2249438683347,123.982053991813)) ;
#95125=CARTESIAN_POINT('Ctrl Pts',(-20.3563663912359,46.2349751216766,124.158367942863)) ;
#95126=CARTESIAN_POINT('Ctrl Pts',(-20.2144077277106,46.2448418205497,124.309619918367)) ;
#95127=CARTESIAN_POINT('Ctrl Pts',(-20.0465524037554,46.2548286363009,124.435697561144)) ;
#95128=CARTESIAN_POINT('Ctrl Pts',(-19.8600955667998,46.2647758414964,124.530446740553)) ;
#95129=CARTESIAN_POINT('Ctrl Pts',(-19.6581071039658,46.2748188296227,124.591866565516)) ;
#95130=CARTESIAN_POINT('Ctrl Pts',(-19.4521805333531,46.2846861842441,124.616961782451)) ;
#95131=CARTESIAN_POINT('Ctrl Pts',(-19.2429425557365,46.2946520775422,124.606374912702)) ;
#95132=CARTESIAN_POINT('Ctrl Pts',(-19.0375622356336,46.3046758549183,124.559128812759)) ;
#95133=CARTESIAN_POINT('Ctrl Pts',(-18.8454096797733,46.31460140285,124.477797809771)) ;
#95134=CARTESIAN_POINT('Ctrl Pts',(-18.6697469855998,46.324541879271,124.364570062756)) ;
#95135=CARTESIAN_POINT('Ctrl Pts',(-18.5149640326818,46.3345880889339,124.220891191222)) ;
#95136=CARTESIAN_POINT('Ctrl Pts',(-18.3896311429389,46.3444493455957,124.055728922196)) ;
#95137=CARTESIAN_POINT('Ctrl Pts',(-18.293309290402,46.354442973871,123.869046532394)) ;
#95138=CARTESIAN_POINT('Ctrl Pts',(-18.2311685522443,46.3643683711812,123.66981820444)) ;
#95139=CARTESIAN_POINT('Ctrl Pts',(-18.2042912858194,46.3743962790915,123.460747760287)) ;
#95140=CARTESIAN_POINT('Ctrl Pts',(-18.2137735652892,46.3842825947606,123.253091982642)) ;
#95141=CARTESIAN_POINT('Ctrl Pts',(-18.2597106191738,46.3943141896644,123.047294517772)) ;
#95142=CARTESIAN_POINT('Ctrl Pts',(-18.3393268080078,46.4041964326161,122.855362755842)) ;
#95143=CARTESIAN_POINT('Ctrl Pts',(-18.4529567773055,46.414255903646,122.677029418448)) ;
#95144=CARTESIAN_POINT('Ctrl Pts',(-18.593127764121,46.4241223483091,122.524119521912)) ;
#95145=CARTESIAN_POINT('Ctrl Pts',(-18.7589661169091,46.4340884727578,122.396081343942)) ;
#95146=CARTESIAN_POINT('Ctrl Pts',(-18.94587076229,46.444118716149,122.298455525749)) ;
#95147=CARTESIAN_POINT('Ctrl Pts',(-19.1440685803664,46.454011751102,122.235347185995)) ;
#95148=CARTESIAN_POINT('Ctrl Pts',(-19.3534587786841,46.4640626653389,122.207116928678)) ;
#95149=CARTESIAN_POINT('Ctrl Pts',(-19.5612106794145,46.4739524915634,122.215512482208)) ;
#95150=CARTESIAN_POINT('Ctrl Pts',(-19.8352623928839,46.4872873066104,122.274761976514)) ;
#95151=CARTESIAN_POINT('Ctrl Pts',(-20.0862027417132,46.5005643977818,122.404067085043)) ;
#95152=CARTESIAN_POINT('Ctrl Pts',(-20.2927726800463,46.5138126863801,122.590867858062)) ;
#95153=CARTESIAN_POINT('Ctrl Pts',(-20.4224375762287,46.5238675278742,122.757782621042)) ;
#95154=CARTESIAN_POINT('Ctrl Pts',(-20.5192877126657,46.5336985171818,122.940402706794)) ;
#95155=CARTESIAN_POINT('Ctrl Pts',(-20.584675695254,46.543775081505,123.141863716105)) ;
#95156=CARTESIAN_POINT('Ctrl Pts',(-20.6134306365169,46.5536244066389,123.346938502244)) ;
#95157=CARTESIAN_POINT('Ctrl Pts',(-20.6042235970705,46.5669724062762,123.627443254569)) ;
#95158=CARTESIAN_POINT('Ctrl Pts',(-20.5014828458008,46.5835571658128,123.96471352082)) ;
#95159=CARTESIAN_POINT('Ctrl Pts',(-20.2906566247989,46.6001257171609,124.247018966344)) ;
#95160=CARTESIAN_POINT('Ctrl Pts',(-20.0699817614832,46.6134855419799,124.420721848801)) ;
#95161=CARTESIAN_POINT('Ctrl Pts',(-19.8865379628429,46.6233909508105,124.519311216368)) ;
#95162=CARTESIAN_POINT('Ctrl Pts',(-19.6878067636741,46.6333509773946,124.585185790603)) ;
#95163=CARTESIAN_POINT('Ctrl Pts',(-19.412046265777,46.6466085615799,124.625974157288)) ;
#95164=CARTESIAN_POINT('Ctrl Pts',(-19.0603317080607,46.6632597730745,124.585529966129)) ;
#95165=CARTESIAN_POINT('Ctrl Pts',(-18.6814960639514,46.6831779871848,124.39623149894)) ;
#95166=CARTESIAN_POINT('Ctrl Pts',(-18.3898810556828,46.7030557504057,124.090210943311)) ;
#95167=CARTESIAN_POINT('Ctrl Pts',(-18.2194528936374,46.7230684181928,123.700392538323)) ;
#95168=CARTESIAN_POINT('Ctrl Pts',(-18.192146649637,46.7428809408594,123.279930238495)) ;
#95169=CARTESIAN_POINT('Ctrl Pts',(-18.3102874548359,46.7628642408593,122.871872061097)) ;
#95170=CARTESIAN_POINT('Ctrl Pts',(-18.5598053137279,46.7827585179606,122.530215742655)) ;
#95171=CARTESIAN_POINT('Ctrl Pts',(-18.9111817055603,46.8026912797184,122.293251036781)) ;
#95172=CARTESIAN_POINT('Ctrl Pts',(-19.3230997389013,46.8226572854831,122.190530003981)) ;
#95173=CARTESIAN_POINT('Ctrl Pts',(-19.743552728489,46.842535817648,122.234047595164)) ;
#95174=CARTESIAN_POINT('Ctrl Pts',(-20.1251993127685,46.8624754843083,122.418602193788)) ;
#95175=CARTESIAN_POINT('Ctrl Pts',(-20.4204440382174,46.8823703589537,122.721609165698)) ;
#95176=CARTESIAN_POINT('Ctrl Pts',(-20.5949959092053,46.902277498247,123.107115871123)) ;
#95177=CARTESIAN_POINT('Ctrl Pts',(-20.6282641723877,46.9221880463255,123.529296695929)) ;
#95178=CARTESIAN_POINT('Ctrl Pts',(-20.5136941034275,46.9422566316827,123.940243017391)) ;
#95179=CARTESIAN_POINT('Ctrl Pts',(-20.2695209088635,46.9620384289975,124.282898500784)) ;
#95180=CARTESIAN_POINT('Ctrl Pts',(-19.9197275238897,46.982045975942,124.524725530521)) ;
#95181=CARTESIAN_POINT('Ctrl Pts',(-19.5119619250136,47.0018677142448,124.631757161439)) ;
#95182=CARTESIAN_POINT('Ctrl Pts',(-19.0889034196956,47.021847734149,124.593693802023)) ;
#95183=CARTESIAN_POINT('Ctrl Pts',(-18.7055978572191,47.0417651854112,124.413578300062)) ;
#95184=CARTESIAN_POINT('Ctrl Pts',(-18.4066951109051,47.0616401065839,124.114802890344)) ;
#95185=CARTESIAN_POINT('Ctrl Pts',(-18.226617705254,47.0816644751348,123.729017723871)) ;
#95186=CARTESIAN_POINT('Ctrl Pts',(-18.189408601878,47.1015311595082,123.308171256275)) ;
#95187=CARTESIAN_POINT('Ctrl Pts',(-18.2977813628575,47.1214749813544,122.898242687212)) ;
#95188=CARTESIAN_POINT('Ctrl Pts',(-18.5392371883832,47.141382350606,122.550578232716)) ;
#95189=CARTESIAN_POINT('Ctrl Pts',(-18.8838108505728,47.1612570483527,122.305940543012)) ;
#95190=CARTESIAN_POINT('Ctrl Pts',(-19.2933814550574,47.1812389908744,122.192858534516)) ;
#95191=CARTESIAN_POINT('Ctrl Pts',(-19.7151773995363,47.2011416577852,122.226545847084)) ;
#95192=CARTESIAN_POINT('Ctrl Pts',(-20.0998580309074,47.2209970153239,122.400636973891)) ;
#95193=CARTESIAN_POINT('Ctrl Pts',(-20.4047901284186,47.2410610540399,122.698899639654)) ;
#95194=CARTESIAN_POINT('Ctrl Pts',(-20.5876552099661,47.260916233765,123.079589215537)) ;
#95195=CARTESIAN_POINT('Ctrl Pts',(-20.6302016757716,47.2808963384294,123.502119802794)) ;
#95196=CARTESIAN_POINT('Ctrl Pts',(-20.5273230835641,47.3007054435992,123.910681564784)) ;
#95197=CARTESIAN_POINT('Ctrl Pts',(-20.2895042513562,47.3206980639399,124.262875716145)) ;
#95198=CARTESIAN_POINT('Ctrl Pts',(-20.0050353154875,47.337237546444,124.469774715203)) ;
#95199=CARTESIAN_POINT('Ctrl Pts',(-19.7428588681219,47.3506018645082,124.570749567793)) ;
#95200=CARTESIAN_POINT('Ctrl Pts',(-19.4702099178661,47.3638194670097,124.624411955368)) ;
#95201=CARTESIAN_POINT('Ctrl Pts',(-19.1168449437706,47.3804770612875,124.600779206407)) ;
#95202=CARTESIAN_POINT('Ctrl Pts',(-18.7302030844524,47.4003427633293,124.430524065223)) ;
#95203=CARTESIAN_POINT('Ctrl Pts',(-18.4743682787184,47.4169724900193,124.18657910822)) ;
#95204=CARTESIAN_POINT('Ctrl Pts',(-18.3289985873677,47.4302616051571,123.947912570718)) ;
#95205=CARTESIAN_POINT('Ctrl Pts',(-18.2525289057736,47.4402259521342,123.752907821756)) ;
#95206=CARTESIAN_POINT('Ctrl Pts',(-18.211089465491,47.4501543201357,123.54833464698)) ;
#95207=CARTESIAN_POINT('Ctrl Pts',(-18.2034573471076,47.4634377532245,123.269197774288)) ;
#95208=CARTESIAN_POINT('Ctrl Pts',(-18.2859430582896,47.4800898309648,122.924823240725)) ;
#95209=CARTESIAN_POINT('Ctrl Pts',(-18.4796139718569,47.4966412002656,122.631051279502)) ;
#95210=CARTESIAN_POINT('Ctrl Pts',(-18.6881383224874,47.5099286284146,122.445096775758)) ;
#95211=CARTESIAN_POINT('Ctrl Pts',(-18.8678491667087,47.5199731681147,122.334247512461)) ;
#95212=CARTESIAN_POINT('Ctrl Pts',(-19.060072139105,47.5298160099385,122.257599489778)) ;
#95213=CARTESIAN_POINT('Ctrl Pts',(-19.2654626653682,47.5398002941855,122.214420612001)) ;
#95214=CARTESIAN_POINT('Ctrl Pts',(-19.4745348865352,47.5497499395846,122.207626210746)) ;
#95215=CARTESIAN_POINT('Ctrl Pts',(-19.6826924292241,47.559749701273,122.237130762337)) ;
#95216=CARTESIAN_POINT('Ctrl Pts',(-19.8830746491751,47.5697810472319,122.302862428866)) ;
#95217=CARTESIAN_POINT('Ctrl Pts',(-20.0658794802502,47.5796360017091,122.400373786008)) ;
#95218=CARTESIAN_POINT('Ctrl Pts',(-20.2312035024251,47.5896085397096,122.529268274706)) ;
#95219=CARTESIAN_POINT('Ctrl Pts',(-20.3719769005588,47.5996035334445,122.685311427216)) ;
#95220=CARTESIAN_POINT('Ctrl Pts',(-20.4837075622632,47.6096375922386,122.864217867557)) ;
#95221=CARTESIAN_POINT('Ctrl Pts',(-20.5615908356297,47.6194929350616,123.056234985806)) ;
#95222=CARTESIAN_POINT('Ctrl Pts',(-20.6058491720803,47.6294924144072,123.261705418283)) ;
#95223=CARTESIAN_POINT('Ctrl Pts',(-20.6139152854521,47.6393868631625,123.469600680338)) ;
#95224=CARTESIAN_POINT('Ctrl Pts',(-20.5852299915617,47.649449982597,123.679168585818)) ;
#95225=CARTESIAN_POINT('Ctrl Pts',(-20.5222237825288,47.6592896278382,123.876236002791)) ;
#95226=CARTESIAN_POINT('Ctrl Pts',(-20.4240386183092,47.6693527920243,124.063598482172)) ;
#95227=CARTESIAN_POINT('Ctrl Pts',(-20.2968105105558,47.6792470617731,124.228190143397)) ;
#95228=CARTESIAN_POINT('Ctrl Pts',(-20.1426174094489,47.689188787787,124.369245425586)) ;
#95229=CARTESIAN_POINT('Ctrl Pts',(-19.9651875360064,47.6991916764463,124.482184157737)) ;
#95230=CARTESIAN_POINT('Ctrl Pts',(-19.7700259465885,47.7092315252403,124.56251968231)) ;
#95231=CARTESIAN_POINT('Ctrl Pts',(-19.5683733928146,47.7190557407012,124.607243544029)) ;
#95232=CARTESIAN_POINT('Ctrl Pts',(-19.357178076069,47.7291125841947,124.616781601142)) ;
#95233=CARTESIAN_POINT('Ctrl Pts',(-19.1502186587645,47.7390411935907,124.589576536288)) ;
#95234=CARTESIAN_POINT('Ctrl Pts',(-18.9504848199683,47.7489930776286,124.527263965266)) ;
#95235=CARTESIAN_POINT('Ctrl Pts',(-18.7629118733579,47.7590460304362,124.429914058781)) ;
#95236=CARTESIAN_POINT('Ctrl Pts',(-18.598675250349,47.7688689069024,124.304701793222)) ;
#95237=CARTESIAN_POINT('Ctrl Pts',(-18.4551028240335,47.7789246394725,124.149549502336)) ;
#95238=CARTESIAN_POINT('Ctrl Pts',(-18.342258643216,47.7888654044602,123.973638763673)) ;
#95239=CARTESIAN_POINT('Ctrl Pts',(-18.2613684522872,47.7987697373658,123.781768983543)) ;
#95240=CARTESIAN_POINT('Ctrl Pts',(-18.2144911981369,47.8088164062465,123.575842264473)) ;
#95241=CARTESIAN_POINT('Ctrl Pts',(-18.2040462151194,47.8187119695523,123.368035264035)) ;
#95242=CARTESIAN_POINT('Ctrl Pts',(-18.2302679710938,47.8287740272526,123.158160931914)) ;
#95243=CARTESIAN_POINT('Ctrl Pts',(-18.2910782452796,47.8386168048801,122.960347495842)) ;
#95244=CARTESIAN_POINT('Ctrl Pts',(-18.3862593754307,47.848607283132,122.773151851679)) ;
#95245=CARTESIAN_POINT('Ctrl Pts',(-18.5117691333417,47.8585362557755,122.606345574257)) ;
#95246=CARTESIAN_POINT('Ctrl Pts',(-18.6650588022171,47.8685273926551,122.462742646535)) ;
#95247=CARTESIAN_POINT('Ctrl Pts',(-18.8416404848203,47.878549510144,122.34779300154)) ;
#95248=CARTESIAN_POINT('Ctrl Pts',(-19.0330683440688,47.8884500205462,122.266070940275)) ;
#95249=CARTESIAN_POINT('Ctrl Pts',(-19.2375119458177,47.8984390132923,122.218087240548)) ;
#95250=CARTESIAN_POINT('Ctrl Pts',(-19.4466836947895,47.9084042573429,122.206504347222)) ;
#95251=CARTESIAN_POINT('Ctrl Pts',(-19.6534986182555,47.9183085218561,122.230779256276)) ;
#95252=CARTESIAN_POINT('Ctrl Pts',(-19.8559842467169,47.9283666135544,122.291642961633)) ;
#95253=CARTESIAN_POINT('Ctrl Pts',(-20.0410138775998,47.9382165539828,122.384646487928)) ;
#95254=CARTESIAN_POINT('Ctrl Pts',(-20.2103684173728,47.9482435651563,122.510161007995)) ;
#95255=CARTESIAN_POINT('Ctrl Pts',(-20.3549894294798,47.9582721517683,122.663586471316)) ;
#95256=CARTESIAN_POINT('Ctrl Pts',(-20.4689725582954,47.968117365881,122.83633708969)) ;
#95257=CARTESIAN_POINT('Ctrl Pts',(-20.5529671107311,47.9781081140606,123.028853175399)) ;
#95258=CARTESIAN_POINT('Ctrl Pts',(-20.6020368114241,47.9881457476461,123.234091515211)) ;
#95259=CARTESIAN_POINT('Ctrl Pts',(-20.6148256883295,47.9979910368589,123.440677297005)) ;
#95260=CARTESIAN_POINT('Ctrl Pts',(-20.5916944344883,48.0079724376648,123.649222795437)) ;
#95261=CARTESIAN_POINT('Ctrl Pts',(-20.5328217909652,48.0179246706548,123.850002480386)) ;
#95262=CARTESIAN_POINT('Ctrl Pts',(-20.4397876959879,48.0279234821114,124.038518366483)) ;
#95263=CARTESIAN_POINT('Ctrl Pts',(-20.314622836636,48.0379625860421,124.208436635421)) ;
#95264=CARTESIAN_POINT('Ctrl Pts',(-20.1654041864277,48.0477875284614,124.351272569223)) ;
#95265=CARTESIAN_POINT('Ctrl Pts',(-19.9898488473911,48.0578422159373,124.468988134481)) ;
#95266=CARTESIAN_POINT('Ctrl Pts',(-19.7985107732397,48.0677850182941,124.553163168136)) ;
#95267=CARTESIAN_POINT('Ctrl Pts',(-19.5964148826951,48.0776888142339,124.603261719813)) ;
#95268=CARTESIAN_POINT('Ctrl Pts',(-19.3857035042312,48.0877355936089,124.617586751517)) ;
#95269=CARTESIAN_POINT('Ctrl Pts',(-19.1787979589594,48.0976312519035,124.595621176739)) ;
#95270=CARTESIAN_POINT('Ctrl Pts',(-18.9755413219689,48.1076928191541,124.537136972001)) ;
#95271=CARTESIAN_POINT('Ctrl Pts',(-18.7895837292006,48.1175374635914,124.446269126648)) ;
#95272=CARTESIAN_POINT('Ctrl Pts',(-18.6198326590471,48.1274975098341,124.323679639637)) ;
#95273=CARTESIAN_POINT('Ctrl Pts',(-18.4731016928409,48.1375358058525,124.172014573816)) ;
#95274=CARTESIAN_POINT('Ctrl Pts',(-18.3565226921379,48.1474091472708,124.000238839827)) ;
#95275=CARTESIAN_POINT('Ctrl Pts',(-18.2699091481293,48.1574822510701,123.807037664057)) ;
#95276=CARTESIAN_POINT('Ctrl Pts',(-18.2191835116695,48.167303066189,123.606859972749)) ;
#95277=CARTESIAN_POINT('Ctrl Pts',(-18.2033538657066,48.177379931267,123.395643649504)) ;
#95278=CARTESIAN_POINT('Ctrl Pts',(-18.2240803927477,48.1872446709223,123.189269101295)) ;
#95279=CARTESIAN_POINT('Ctrl Pts',(-18.2806840855766,48.1972670741636,122.986320600377)) ;
#95280=CARTESIAN_POINT('Ctrl Pts',(-18.3721813471877,48.2072927984521,122.796429449923)) ;
#95281=CARTESIAN_POINT('Ctrl Pts',(-18.4928501478917,48.2171475814734,122.62803509953)) ;
#95282=CARTESIAN_POINT('Ctrl Pts',(-18.6424187240408,48.2271264251967,122.480923759467)) ;
#95283=CARTESIAN_POINT('Ctrl Pts',(-18.8161459824294,48.2371453174333,122.361848194698)) ;
#95284=CARTESIAN_POINT('Ctrl Pts',(-19.0051677361826,48.2470285264743,122.275518633424)) ;
#95285=CARTESIAN_POINT('Ctrl Pts',(-19.2100373124816,48.2570968358145,122.222445400665)) ;
#95286=CARTESIAN_POINT('Ctrl Pts',(-19.4160689133427,48.2669269611472,122.205898319605)) ;
#95287=CARTESIAN_POINT('Ctrl Pts',(-19.6267500453631,48.2769935135242,122.225565266307)) ;
#95288=CARTESIAN_POINT('Ctrl Pts',(-19.8272641782343,48.2868837504179,122.280674195166)) ;
#95289=CARTESIAN_POINT('Ctrl Pts',(-20.0172632691335,48.2968759752119,122.370249342106)) ;
#95290=CARTESIAN_POINT('Ctrl Pts',(-20.1882096752109,48.3068385955629,122.49125875939)) ;
#95291=CARTESIAN_POINT('Ctrl Pts',(-20.3350743761044,48.316743598326,122.638900187718)) ;
#95292=CARTESIAN_POINT('Ctrl Pts',(-20.4557702033646,48.3268013607242,122.81249208294)) ;
#95293=CARTESIAN_POINT('Ctrl Pts',(-20.5428321220069,48.336651880103,123.000408221936)) ;
#95294=CARTESIAN_POINT('Ctrl Pts',(-20.5973595966834,48.3466834571011,123.204118610426)) ;
#95295=CARTESIAN_POINT('Ctrl Pts',(-20.6152472704688,48.3566931922061,123.413816441878)) ;
#95296=CARTESIAN_POINT('Ctrl Pts',(-20.5968276470534,48.3666027688323,123.621312622451)) ;
#95297=CARTESIAN_POINT('Ctrl Pts',(-20.5430718873729,48.376530154689,123.822985193419)) ;
#95298=CARTESIAN_POINT('Ctrl Pts',(-20.453926297321,48.3865750891793,124.014413092725)) ;
#95299=CARTESIAN_POINT('Ctrl Pts',(-20.3349016235534,48.3964610213672,124.184803456692)) ;
#95300=CARTESIAN_POINT('Ctrl Pts',(-20.1867787673531,48.4064543273203,124.33377573262)) ;
#95301=CARTESIAN_POINT('Ctrl Pts',(-20.0158011743362,48.4163999651021,124.454128850865)) ;
#95302=CARTESIAN_POINT('Ctrl Pts',(-19.826666064814,48.426347233448,124.543373150093)) ;
#95303=CARTESIAN_POINT('Ctrl Pts',(-19.622820788123,48.4363951355851,124.598744953665)) ;
#95304=CARTESIAN_POINT('Ctrl Pts',(-19.4166583633309,48.4462428304253,124.617674236662)) ;
#95305=CARTESIAN_POINT('Ctrl Pts',(-19.2079107407179,48.4562043401698,124.600980623908)) ;
#95306=CARTESIAN_POINT('Ctrl Pts',(-19.003906573456,48.4662337317786,124.547658872427)) ;
#95307=CARTESIAN_POINT('Ctrl Pts',(-18.8145476533878,48.4761412273334,124.460899967926)) ;
#95308=CARTESIAN_POINT('Ctrl Pts',(-18.6422518472801,48.4860866189964,124.342481581082)) ;
#95309=CARTESIAN_POINT('Ctrl Pts',(-18.4921671420408,48.4960885365937,124.195169742631)) ;
#95310=CARTESIAN_POINT('Ctrl Pts',(-18.3698192894223,48.5061286041459,124.023195675752)) ;
#95311=CARTESIAN_POINT('Ctrl Pts',(-18.2806985353055,48.5159529155857,123.83685620093)) ;
#95312=CARTESIAN_POINT('Ctrl Pts',(-18.22370774052,48.5260091567418,123.633290226062)) ;
#95313=CARTESIAN_POINT('Ctrl Pts',(-18.2034272666168,48.5359400784775,123.425474826601)) ;
#95314=CARTESIAN_POINT('Ctrl Pts',(-18.2191289100318,48.5458833145537,123.217054156125)) ;
#95315=CARTESIAN_POINT('Ctrl Pts',(-18.2707969945288,48.5558645985662,123.013643980208)) ;
#95316=CARTESIAN_POINT('Ctrl Pts',(-18.3578513136604,48.5659089001918,122.821289657151)) ;
#95317=CARTESIAN_POINT('Ctrl Pts',(-18.4740534559425,48.5757369814113,122.650406895591)) ;
#95318=CARTESIAN_POINT('Ctrl Pts',(-18.6216781740436,48.5858135842604,122.498533643899)) ;
#95319=CARTESIAN_POINT('Ctrl Pts',(-18.7896140709014,48.595665663379,122.377226252278)) ;
#95320=CARTESIAN_POINT('Ctrl Pts',(-18.9800970249153,48.6057389216879,122.284765876167)) ;
#95321=CARTESIAN_POINT('Ctrl Pts',(-19.1791159034556,48.6155803810682,122.228160560992)) ;
#95322=CARTESIAN_POINT('Ctrl Pts',(-19.3873388361497,48.6255414764805,122.205934289696)) ;
#95323=CARTESIAN_POINT('Ctrl Pts',(-19.5978306492619,48.6355787608773,122.220722308273)) ;
#95324=CARTESIAN_POINT('Ctrl Pts',(-19.799388463471,48.6454550996125,122.270668660089)) ;
#95325=CARTESIAN_POINT('Ctrl Pts',(-19.9927541999136,48.6555172257658,122.356380829401)) ;
#95326=CARTESIAN_POINT('Ctrl Pts',(-20.1649868946281,48.6653853997423,122.472078082189)) ;
#95327=CARTESIAN_POINT('Ctrl Pts',(-20.3168522676943,48.6753909482461,122.617582443954)) ;
#95328=CARTESIAN_POINT('Ctrl Pts',(-20.4408428213035,48.6853735801417,122.786952855138)) ;
#95329=CARTESIAN_POINT('Ctrl Pts',(-20.533889105216,48.6954175225635,122.976482672642)) ;
#95330=CARTESIAN_POINT('Ctrl Pts',(-20.5916223940478,48.7052456705907,123.17487095886)) ;
#95331=CARTESIAN_POINT('Ctrl Pts',(-20.6150709599507,48.7152355379651,123.383577027473)) ;
#95332=CARTESIAN_POINT('Ctrl Pts',(-20.6013063806438,48.7252792769206,123.59427890037)) ;
#95333=CARTESIAN_POINT('Ctrl Pts',(-20.5526930860455,48.7351010254585,123.794957259906)) ;
#95334=CARTESIAN_POINT('Ctrl Pts',(-20.4686518829864,48.7451360030682,123.988462035549)) ;
#95335=CARTESIAN_POINT('Ctrl Pts',(-20.3519125818634,48.7551609158259,124.163938838263)) ;
#95336=CARTESIAN_POINT('Ctrl Pts',(-20.2093168668015,48.7650128589198,124.314159551624)) ;
#95337=CARTESIAN_POINT('Ctrl Pts',(-20.0406693441658,48.7750038202489,124.439317914556)) ;
#95338=CARTESIAN_POINT('Ctrl Pts',(-19.8542415899893,48.7849216951173,124.532750810719)) ;
#95339=CARTESIAN_POINT('Ctrl Pts',(-19.6522481455534,48.7949502141185,124.593089434004)) ;
#95340=CARTESIAN_POINT('Ctrl Pts',(-19.4458572034312,48.8048338929164,124.617196619224)) ;
#95341=CARTESIAN_POINT('Ctrl Pts',(-19.2360620949914,48.8148288363561,124.605427829413)) ;
#95342=CARTESIAN_POINT('Ctrl Pts',(-19.0309256562001,48.8248556901785,124.556904561977)) ;
#95343=CARTESIAN_POINT('Ctrl Pts',(-18.8399656537912,48.8347398545175,124.474946592607)) ;
#95344=CARTESIAN_POINT('Ctrl Pts',(-18.6641807496761,48.8447279525599,124.360128704613)) ;
#95345=CARTESIAN_POINT('Ctrl Pts',(-18.5114556876915,48.8546790590169,124.217117736097)) ;
#95346=CARTESIAN_POINT('Ctrl Pts',(-18.3848137965873,48.864724110185,124.048141101483)) ;
#95347=CARTESIAN_POINT('Ctrl Pts',(-18.2910674776391,48.8745858705433,123.863220172721)) ;
#95348=CARTESIAN_POINT('Ctrl Pts',(-18.2296182843222,48.8845486873738,123.662986258613)) ;
#95349=CARTESIAN_POINT('Ctrl Pts',(-18.2040446117708,48.8945833686545,123.453590801485)) ;
#95350=CARTESIAN_POINT('Ctrl Pts',(-18.2146977108724,48.9044683984353,123.246021045986)) ;
#95351=CARTESIAN_POINT('Ctrl Pts',(-18.262112613018,48.9145339918333,123.039825965983)) ;
#95352=CARTESIAN_POINT('Ctrl Pts',(-18.3425873201439,48.9243731601948,122.849236792747)) ;
#95353=CARTESIAN_POINT('Ctrl Pts',(-18.4572075848471,48.9344357579363,122.671461421509)) ;
#95354=CARTESIAN_POINT('Ctrl Pts',(-18.5987775296174,48.9443327703432,122.518966631599)) ;
#95355=CARTESIAN_POINT('Ctrl Pts',(-18.7648162089244,48.9542640921688,122.392390623785)) ;
#95356=CARTESIAN_POINT('Ctrl Pts',(-18.9524800333232,48.9643058549233,122.295703965336)) ;
#95357=CARTESIAN_POINT('Ctrl Pts',(-19.1509683135226,48.974194053814,122.233882218668)) ;
#95358=CARTESIAN_POINT('Ctrl Pts',(-19.3593098514268,48.9841879924139,122.206854423194)) ;
#95359=CARTESIAN_POINT('Ctrl Pts',(-19.5680935855374,48.9941288134508,122.216376408398)) ;
#95360=CARTESIAN_POINT('Ctrl Pts',(-19.7724671471724,49.004088195739,122.261825265473)) ;
#95361=CARTESIAN_POINT('Ctrl Pts',(-19.9666684295254,49.0140859553913,122.342274294019)) ;
#95362=CARTESIAN_POINT('Ctrl Pts',(-20.1444533832178,49.0241220915936,122.455885746671)) ;
#95363=CARTESIAN_POINT('Ctrl Pts',(-20.2971096778046,49.0339728890845,122.595827077443)) ;
#95364=CARTESIAN_POINT('Ctrl Pts',(-20.42504775658,49.0439337541608,122.761600423317)) ;
#95365=CARTESIAN_POINT('Ctrl Pts',(-20.5227053078636,49.0539626217912,122.948471675384)) ;
#95366=CARTESIAN_POINT('Ctrl Pts',(-20.5857337929231,49.0638728579276,123.14704453)) ;
#95367=CARTESIAN_POINT('Ctrl Pts',(-20.6139392672823,49.0738078112422,123.354001305858)) ;
#95368=CARTESIAN_POINT('Ctrl Pts',(-20.6055025787485,49.0838487416517,123.564919624935)) ;
#95369=CARTESIAN_POINT('Ctrl Pts',(-20.5613836179293,49.0937366384333,123.768066917084)) ;
#95370=CARTESIAN_POINT('Ctrl Pts',(-20.4822199689316,49.103726090092,123.962579586994)) ;
#95371=CARTESIAN_POINT('Ctrl Pts',(-20.37068363497,49.1136851804574,124.139761405237)) ;
#95372=CARTESIAN_POINT('Ctrl Pts',(-20.2313302399948,49.1235824927637,124.294294621323)) ;
#95373=CARTESIAN_POINT('Ctrl Pts',(-20.0645865405684,49.133638918664,124.424243371079)) ;
#95374=CARTESIAN_POINT('Ctrl Pts',(-19.8812921014099,49.1435089212537,124.521540995851)) ;
#95375=CARTESIAN_POINT('Ctrl Pts',(-19.6813785176454,49.1535128544309,124.586788980192)) ;
#95376=CARTESIAN_POINT('Ctrl Pts',(-19.4734493318863,49.1635001148948,124.616182759415)) ;
#95377=CARTESIAN_POINT('Ctrl Pts',(-19.2627909630447,49.1735271664805,124.608876433313)) ;
#95378=CARTESIAN_POINT('Ctrl Pts',(-19.0593248865046,49.1834182563066,124.565892059156)) ;
#95379=CARTESIAN_POINT('Ctrl Pts',(-18.7998848677317,49.1967160110877,124.461822865144)) ;
#95380=CARTESIAN_POINT('Ctrl Pts',(-18.5749110821987,49.2099140706958,124.293969457088)) ;
#95381=CARTESIAN_POINT('Ctrl Pts',(-18.4005901022622,49.223310811265,124.072839397159)) ;
#95382=CARTESIAN_POINT('Ctrl Pts',(-18.3021399164489,49.2331817233385,123.890105683798)) ;
#95383=CARTESIAN_POINT('Ctrl Pts',(-18.2356163002858,49.2432552851066,123.689098892024)) ;
#95384=CARTESIAN_POINT('Ctrl Pts',(-18.205508606502,49.2530766976949,123.484778341202)) ;
#95385=CARTESIAN_POINT('Ctrl Pts',(-18.2112828047954,49.263150714926,123.273123359953)) ;
#95386=CARTESIAN_POINT('Ctrl Pts',(-18.2665396821944,49.2763095018905,123.001992383128)) ;
#95387=CARTESIAN_POINT('Ctrl Pts',(-18.3927903994223,49.2896756049847,122.747437406837)) ;
#95388=CARTESIAN_POINT('Ctrl Pts',(-18.5783673105112,49.3029895398738,122.537851115961)) ;
#95389=CARTESIAN_POINT('Ctrl Pts',(-18.7409926730701,49.3128895793212,122.40799514289)) ;
#95390=CARTESIAN_POINT('Ctrl Pts',(-18.9247420206413,49.3228539824558,122.307378307647)) ;
#95391=CARTESIAN_POINT('Ctrl Pts',(-19.1245308077183,49.3328839495769,122.239933879474)) ;
#95392=CARTESIAN_POINT('Ctrl Pts',(-19.3303117943017,49.342786226186,122.208520853184)) ;
#95393=CARTESIAN_POINT('Ctrl Pts',(-19.6091930994025,49.3560521553551,122.214236467048)) ;
#95394=CARTESIAN_POINT('Ctrl Pts',(-19.9485296513228,49.3726736864615,122.312721965115)) ;
#95395=CARTESIAN_POINT('Ctrl Pts',(-20.2902094521447,49.3925485151062,122.561479447863)) ;
#95396=CARTESIAN_POINT('Ctrl Pts',(-20.4884697082381,49.4092217232081,122.855392698885)) ;
#95397=CARTESIAN_POINT('Ctrl Pts',(-20.578996749337,49.4224728481893,123.118823560105)) ;
#95398=CARTESIAN_POINT('Ctrl Pts',(-20.6234021124794,49.4357151670102,123.393723305564)) ;
#95399=CARTESIAN_POINT('Ctrl Pts',(-20.5867774458657,49.4524484073496,123.747548085192)) ;
#95400=CARTESIAN_POINT('Ctrl Pts',(-20.4028092707548,49.4722775555376,124.127010849328)) ;
#95401=CARTESIAN_POINT('Ctrl Pts',(-20.0997798393814,49.4922022506382,124.422943948998)) ;
#95402=CARTESIAN_POINT('Ctrl Pts',(-19.7138202488184,49.5121254792217,124.597719634898)) ;
#95403=CARTESIAN_POINT('Ctrl Pts',(-19.2914296044062,49.5320526183478,124.630422657138)) ;
#95404=CARTESIAN_POINT('Ctrl Pts',(-18.8840519429806,49.5519290809634,124.517817506517)) ;
#95405=CARTESIAN_POINT('Ctrl Pts',(-18.5377035770347,49.5719063095687,124.27191546715)) ;
#95406=CARTESIAN_POINT('Ctrl Pts',(-18.2968244731111,49.5918411675424,123.923098218903)) ;
#95407=CARTESIAN_POINT('Ctrl Pts',(-18.1892441438947,49.6117376164732,123.513986113187)) ;
#95408=CARTESIAN_POINT('Ctrl Pts',(-18.2273108370955,49.6316589005398,123.092101257408)) ;
#95409=CARTESIAN_POINT('Ctrl Pts',(-18.4075016177291,49.6516155502108,122.707903558998)) ;
#95410=CARTESIAN_POINT('Ctrl Pts',(-18.7066393674634,49.6714928433224,122.409408052842)) ;
#95411=CARTESIAN_POINT('Ctrl Pts',(-19.0894747831973,49.6913793155508,122.229768574258)) ;
#95412=CARTESIAN_POINT('Ctrl Pts',(-19.5143647801207,49.7114408814748,122.191861124704)) ;
#95413=CARTESIAN_POINT('Ctrl Pts',(-19.9220057904957,49.7312812890156,122.300397275708)) ;
#95414=CARTESIAN_POINT('Ctrl Pts',(-20.2693648000579,49.7511326129885,122.54022502922)) ;
#95415=CARTESIAN_POINT('Ctrl Pts',(-20.5159525925647,49.77118588294,122.888006985456)) ;
#95416=CARTESIAN_POINT('Ctrl Pts',(-20.6278796892875,49.7910065403233,123.294433975262)) ;
#95417=CARTESIAN_POINT('Ctrl Pts',(-20.5948465336614,49.8109779616538,123.717653699581)) ;
#95418=CARTESIAN_POINT('Ctrl Pts',(-20.4200331926624,49.8308714540175,124.102995975401)) ;
#95419=CARTESIAN_POINT('Ctrl Pts',(-20.1222394105841,49.8508955402586,124.407164838694)) ;
#95420=CARTESIAN_POINT('Ctrl Pts',(-19.7427027808656,49.8707004193714,124.589700995949)) ;
#95421=CARTESIAN_POINT('Ctrl Pts',(-19.320572120998,49.8906594350693,124.633229800858)) ;
#95422=CARTESIAN_POINT('Ctrl Pts',(-18.9086034132619,49.9106454586984,124.528993193034)) ;
#95423=CARTESIAN_POINT('Ctrl Pts',(-18.5595577529917,49.9304539544589,124.293209163247)) ;
#95424=CARTESIAN_POINT('Ctrl Pts',(-18.3093968681947,49.9504365935644,123.949887426195)) ;
#95425=CARTESIAN_POINT('Ctrl Pts',(-18.1920567335,49.9703180413585,123.543654787052)) ;
#95426=CARTESIAN_POINT('Ctrl Pts',(-18.2201436686759,49.990274508096,123.120348075344)) ;
#95427=CARTESIAN_POINT('Ctrl Pts',(-18.3901206018369,50.0101519050516,122.733311854213)) ;
#95428=CARTESIAN_POINT('Ctrl Pts',(-18.6832551201811,50.0301338512269,122.42582166897)) ;
#95429=CARTESIAN_POINT('Ctrl Pts',(-19.0629301007364,50.0500629502636,122.23745376237)) ;
#95430=CARTESIAN_POINT('Ctrl Pts',(-19.4839074729106,50.0699915734762,122.189906489592)) ;
#95431=CARTESIAN_POINT('Ctrl Pts',(-19.894198197734,50.0898258975826,122.287670868876)) ;
#95432=CARTESIAN_POINT('Ctrl Pts',(-20.1900712867489,50.106478184966,122.481987249183)) ;
#95433=CARTESIAN_POINT('Ctrl Pts',(-20.3755131098878,50.1197386859883,122.690239071981)) ;
#95434=CARTESIAN_POINT('Ctrl Pts',(-20.4862810538597,50.1297401631895,122.868949284785)) ;
#95435=CARTESIAN_POINT('Ctrl Pts',(-20.5642531899787,50.139772184049,123.064919168219)) ;
#95436=CARTESIAN_POINT('Ctrl Pts',(-20.6065416958673,50.1496357277746,123.267915697888)) ;
#95437=CARTESIAN_POINT('Ctrl Pts',(-20.6135616640685,50.1596044414447,123.47738464972)) ;
#95438=CARTESIAN_POINT('Ctrl Pts',(-20.5737479830051,50.1729501888484,123.755049879261)) ;
#95439=CARTESIAN_POINT('Ctrl Pts',(-20.4644112620115,50.1861007439211,124.012460485703)) ;
#95440=CARTESIAN_POINT('Ctrl Pts',(-20.2913079986546,50.199486124471,124.234313522455)) ;
#95441=CARTESIAN_POINT('Ctrl Pts',(-20.1368976756591,50.2093740604638,124.373521069684)) ;
#95442=CARTESIAN_POINT('Ctrl Pts',(-19.9590515319526,50.2193652502764,124.485228994249)) ;
#95443=CARTESIAN_POINT('Ctrl Pts',(-19.7652513682256,50.2293173488147,124.564155979897)) ;
#95444=CARTESIAN_POINT('Ctrl Pts',(-19.5587718065409,50.2393636052652,124.608506614691)) ;
#95445=CARTESIAN_POINT('Ctrl Pts',(-19.3518493726821,50.2492130526593,124.616330380142)) ;
#95446=CARTESIAN_POINT('Ctrl Pts',(-19.1442754869309,50.2591757051545,124.588436789505)) ;
#95447=CARTESIAN_POINT('Ctrl Pts',(-18.9435668464815,50.2691987907966,124.524268865294)) ;
#95448=CARTESIAN_POINT('Ctrl Pts',(-18.7587399819941,50.2791239065536,124.42738459836)) ;
#95449=CARTESIAN_POINT('Ctrl Pts',(-18.5915092032389,50.2891763849534,124.298203175833)) ;
#95450=CARTESIAN_POINT('Ctrl Pts',(-18.4519664352218,50.2990278836561,124.145139239257)) ;
#95451=CARTESIAN_POINT('Ctrl Pts',(-18.3393284129575,50.3089996228586,123.968364344044)) ;
#95452=CARTESIAN_POINT('Ctrl Pts',(-18.2589073101998,50.3189948306243,123.774195195946)) ;
#95453=CARTESIAN_POINT('Ctrl Pts',(-18.2135079750364,50.3290288320934,123.568211118818)) ;
#95454=CARTESIAN_POINT('Ctrl Pts',(-18.2043916892367,50.3388841901857,123.36120035134)) ;
#95455=CARTESIAN_POINT('Ctrl Pts',(-18.2314639911044,50.348883665779,123.152768244065)) ;
#95456=CARTESIAN_POINT('Ctrl Pts',(-18.2934523168804,50.3587781142741,122.95416575342)) ;
#95457=CARTESIAN_POINT('Ctrl Pts',(-18.3906320141663,50.3688412385019,122.766288908924)) ;
#95458=CARTESIAN_POINT('Ctrl Pts',(-18.5159679597529,50.3786808648305,122.601680134446)) ;
#95459=CARTESIAN_POINT('Ctrl Pts',(-18.6712068113223,50.3887440998734,122.457990482356)) ;
#95460=CARTESIAN_POINT('Ctrl Pts',(-18.8461841750949,50.3986381051075,122.345485237456)) ;
#95461=CARTESIAN_POINT('Ctrl Pts',(-19.0387184829255,50.4085808183232,122.264163922882)) ;
#95462=CARTESIAN_POINT('Ctrl Pts',(-19.2437750914236,50.4185865581214,122.217162068249)) ;
#95463=CARTESIAN_POINT('Ctrl Pts',(-19.4541815050549,50.4286074602678,122.20670110388)) ;
#95464=CARTESIAN_POINT('Ctrl Pts',(-19.6605343168355,50.4384982303167,122.232355979485)) ;
#95465=CARTESIAN_POINT('Ctrl Pts',(-19.8613998056627,50.4484896410964,122.293768559807)) ;
#95466=CARTESIAN_POINT('Ctrl Pts',(-20.0477153883951,50.4584379867609,122.388776883293)) ;
#95467=CARTESIAN_POINT('Ctrl Pts',(-20.2149291845068,50.4683828448221,122.514309607201)) ;
#95468=CARTESIAN_POINT('Ctrl Pts',(-20.3591331096358,50.478437680215,122.668841765407)) ;
#95469=CARTESIAN_POINT('Ctrl Pts',(-20.4719728917269,50.4882600523165,122.841803140507)) ;
#95470=CARTESIAN_POINT('Ctrl Pts',(-20.5553314025535,50.4983159197602,123.036064306596)) ;
#95471=CARTESIAN_POINT('Ctrl Pts',(-20.6027823192923,50.5082566496181,123.239599688952)) ;
#95472=CARTESIAN_POINT('Ctrl Pts',(-20.6147815729713,50.5181609881693,123.447477704609)) ;
#95473=CARTESIAN_POINT('Ctrl Pts',(-20.5900240766022,50.5282076695977,123.657216644109)) ;
#95474=CARTESIAN_POINT('Ctrl Pts',(-20.5303079538465,50.538103177067,123.856531744031)) ;
#95475=CARTESIAN_POINT('Ctrl Pts',(-20.4353433398059,50.5481654455656,124.045523747245)) ;
#95476=CARTESIAN_POINT('Ctrl Pts',(-20.3118410018698,50.5580074358362,124.211563922258)) ;
#95477=CARTESIAN_POINT('Ctrl Pts',(-20.1594362473347,50.5680008527172,124.356126655464)) ;
#95478=CARTESIAN_POINT('Ctrl Pts',(-19.9854190359377,50.5779253405694,124.471276809316)) ;
#95479=CARTESIAN_POINT('Ctrl Pts',(-19.7927265255418,50.5879249744778,124.555279974465)) ;
#95480=CARTESIAN_POINT('Ctrl Pts',(-19.588605893336,50.5979110847346,124.604501080592)) ;
#95481=CARTESIAN_POINT('Ctrl Pts',(-19.3780314652536,50.6079470359217,124.61737350002)) ;
#95482=CARTESIAN_POINT('Ctrl Pts',(-19.1720910958803,50.6178036742565,124.594220180838)) ;
#95483=CARTESIAN_POINT('Ctrl Pts',(-18.9704025586501,50.6278026343345,124.535105154761)) ;
#95484=CARTESIAN_POINT('Ctrl Pts',(-18.7838328447076,50.6376978646483,124.443006602214)) ;
#95485=CARTESIAN_POINT('Ctrl Pts',(-18.6133502503988,50.647758377117,124.317874570504)) ;
#95486=CARTESIAN_POINT('Ctrl Pts',(-18.4701391673336,50.6576076686631,124.168301047964)) ;
#95487=CARTESIAN_POINT('Ctrl Pts',(-18.3525641925228,50.6676348545953,123.993338588389)) ;
#95488=CARTESIAN_POINT('Ctrl Pts',(-18.2676431887012,50.6776633910547,123.800354530484)) ;
#95489=CARTESIAN_POINT('Ctrl Pts',(-18.2180604076789,50.6875086310196,123.599415304129)) ;
#95490=CARTESIAN_POINT('Ctrl Pts',(-18.2033518853956,50.6974993259428,123.38988994928)) ;
#95491=CARTESIAN_POINT('Ctrl Pts',(-18.2258151174764,50.7075371467014,123.180062975056)) ;
#95492=CARTESIAN_POINT('Ctrl Pts',(-18.2829055830036,50.7173817404784,122.981124546184)) ;
#95493=CARTESIAN_POINT('Ctrl Pts',(-18.374543817564,50.7273657358544,122.792311148238)) ;
#95494=CARTESIAN_POINT('Ctrl Pts',(-18.4971789128897,50.7373147844158,122.622862427556)) ;
#95495=CARTESIAN_POINT('Ctrl Pts',(-18.6480196024587,50.7473172233904,122.476338505738)) ;
#95496=CARTESIAN_POINT('Ctrl Pts',(-18.8224928562283,50.7573384646867,122.358249526149)) ;
#95497=CARTESIAN_POINT('Ctrl Pts',(-19.012249182242,50.7672311431262,122.273123776154)) ;
#95498=CARTESIAN_POINT('Ctrl Pts',(-19.2158038174537,50.7772211970739,122.221412222857)) ;
#95499=CARTESIAN_POINT('Ctrl Pts',(-19.4245865506918,50.7871795582223,122.206028609236)) ;
#95500=CARTESIAN_POINT('Ctrl Pts',(-19.6317117481237,50.7970791851072,122.226497823876)) ;
#95501=CARTESIAN_POINT('Ctrl Pts',(-19.8350849358326,50.8071270819105,122.283522980139)) ;
#95502=CARTESIAN_POINT('Ctrl Pts',(-20.0226963525784,50.8170224395465,122.37348142898)) ;
#95503=CARTESIAN_POINT('Ctrl Pts',(-20.1946528136683,50.8270840920032,122.496627869575)) ;
#95504=CARTESIAN_POINT('Ctrl Pts',(-20.339466545417,50.8369286962752,122.644499598143)) ;
#95505=CARTESIAN_POINT('Ctrl Pts',(-20.4583900882012,50.8468888179732,122.816839654232)) ;
#95506=CARTESIAN_POINT('Ctrl Pts',(-20.545892012549,50.8569268523357,123.008866414043)) ;
#95507=CARTESIAN_POINT('Ctrl Pts',(-20.5982377476504,50.8668011649221,123.209773634667)) ;
#95508=CARTESIAN_POINT('Ctrl Pts',(-20.6152194208443,50.8768706457048,123.420755060105)) ;
#95509=CARTESIAN_POINT('Ctrl Pts',(-20.5958818093624,50.8867049817219,123.626614527352)) ;
#95510=CARTESIAN_POINT('Ctrl Pts',(-20.5405510103418,50.8967379394501,123.830145656788)) ;
#95511=CARTESIAN_POINT('Ctrl Pts',(-20.4503035287167,50.9067583380253,124.020498784439)) ;
#95512=CARTESIAN_POINT('Ctrl Pts',(-20.330679811375,50.9166239117966,124.189949451206)) ;
#95513=CARTESIAN_POINT('Ctrl Pts',(-20.1804458547993,50.9266927864526,124.339042768337)) ;
#95514=CARTESIAN_POINT('Ctrl Pts',(-20.0104561974406,50.9365382173581,124.457150451308)) ;
#95515=CARTESIAN_POINT('Ctrl Pts',(-19.8202798254585,50.9465178422288,124.545737839869)) ;
#95516=CARTESIAN_POINT('Ctrl Pts',(-19.6167140496344,50.9565365251429,124.599784856543)) ;
#95517=CARTESIAN_POINT('Ctrl Pts',(-19.4096995592073,50.9664197903268,124.617864751239)) ;
#95518=CARTESIAN_POINT('Ctrl Pts',(-19.1988827726302,50.9764880844181,124.599299468508)) ;
#95519=CARTESIAN_POINT('Ctrl Pts',(-18.9991976287175,50.9863182146035,124.545926791371)) ;
#95520=CARTESIAN_POINT('Ctrl Pts',(-18.8072531202101,50.9963847628186,124.456872704251)) ;
#95521=CARTESIAN_POINT('Ctrl Pts',(-18.6367526545896,51.0062750115072,124.337824122225)) ;
#95522=CARTESIAN_POINT('Ctrl Pts',(-18.4876977017262,51.0162671932833,124.189818410515)) ;
#95523=CARTESIAN_POINT('Ctrl Pts',(-18.367117992186,51.0262299739111,124.018565039215)) ;
#95524=CARTESIAN_POINT('Ctrl Pts',(-18.2781469080694,51.0361343785848,123.830292810274)) ;
#95525=CARTESIAN_POINT('Ctrl Pts',(-18.2225158456398,51.0461943730639,123.626267208626)) ;
#95526=CARTESIAN_POINT('Ctrl Pts',(-18.2033820490551,51.0560429950336,123.420089240958)) ;
#95527=CARTESIAN_POINT('Ctrl Pts',(-18.2201764733819,51.0660734344455,123.209899736072)) ;
#95528=CARTESIAN_POINT('Ctrl Pts',(-18.2735217754488,51.0760831500802,123.006313725019)) ;
#95529=CARTESIAN_POINT('Ctrl Pts',(-18.3603349820453,51.0859939027728,122.816927523553)) ;
#95530=CARTESIAN_POINT('Ctrl Pts',(-18.4785193177454,51.0959231757192,122.64484961303)) ;
#95531=CARTESIAN_POINT('Ctrl Pts',(-18.6265724883276,51.1059658671119,122.494343330129)) ;
#95532=CARTESIAN_POINT('Ctrl Pts',(-18.795773334273,51.1158524003294,122.373613121916)) ;
#95533=CARTESIAN_POINT('Ctrl Pts',(-18.9852153228182,51.1258455452615,122.282818780092)) ;
#95534=CARTESIAN_POINT('Ctrl Pts',(-19.1866163420278,51.1357912260979,122.226639317315)) ;
#95535=CARTESIAN_POINT('Ctrl Pts',(-19.3947136728631,51.1457384832465,122.20585296853)) ;
#95536=CARTESIAN_POINT('Ctrl Pts',(-19.6053345284675,51.1557863871185,122.221908805865)) ;
#95537=CARTESIAN_POINT('Ctrl Pts',(-19.8059404785661,51.1656340862164,122.273080716496)) ;
#95538=CARTESIAN_POINT('Ctrl Pts',(-19.9970578886728,51.1755955771951,122.358685495831)) ;
#95539=CARTESIAN_POINT('Ctrl Pts',(-20.1714467400249,51.1856250396091,122.477219151317)) ;
#95540=CARTESIAN_POINT('Ctrl Pts',(-20.3208357163494,51.195532270709,122.62235336646)) ;
#95541=CARTESIAN_POINT('Ctrl Pts',(-20.4435745138722,51.2054786493864,122.79162964494)) ;
#95542=CARTESIAN_POINT('Ctrl Pts',(-20.5356748345117,51.2154834181952,122.980744956243)) ;
#95543=CARTESIAN_POINT('Ctrl Pts',(-20.5933963625538,51.2255045392154,123.183354735425)) ;
#95544=CARTESIAN_POINT('Ctrl Pts',(-20.6150184498712,51.2353954050681,123.39017151081)) ;
#95545=CARTESIAN_POINT('Ctrl Pts',(-20.600564956353,51.2453862138273,123.599699814294)) ;
#95546=CARTESIAN_POINT('Ctrl Pts',(-20.5501095068394,51.2553368720076,123.802728469495)) ;
#95547=CARTESIAN_POINT('Ctrl Pts',(-20.4655583890161,51.2652730816497,123.993724128868)) ;
#95548=CARTESIAN_POINT('Ctrl Pts',(-20.3487803717502,51.2752562483746,124.168144460775)) ;
#95549=CARTESIAN_POINT('Ctrl Pts',(-20.2023615012466,51.285300045585,124.320252177703)) ;
#95550=CARTESIAN_POINT('Ctrl Pts',(-20.0356625745698,51.2951282617532,124.44238355308)) ;
#95551=CARTESIAN_POINT('Ctrl Pts',(-19.8457170438004,51.3052048292224,124.536080296056)) ;
#95552=CARTESIAN_POINT('Ctrl Pts',(-19.6468633806885,51.3150569149118,124.594176632678)) ;
#95553=CARTESIAN_POINT('Ctrl Pts',(-19.4364191272755,51.3251301823172,124.617542350763)) ;
#95554=CARTESIAN_POINT('Ctrl Pts',(-19.2299340341238,51.3349715987408,124.604264987046)) ;
#95555=CARTESIAN_POINT('Ctrl Pts',(-19.0262804267523,51.3449328568836,124.55550789222)) ;
#95556=CARTESIAN_POINT('Ctrl Pts',(-18.8328905252114,51.3549695333155,124.471123425444)) ;
#95557=CARTESIAN_POINT('Ctrl Pts',(-18.6596436743911,51.3648481411793,124.35655766273)) ;
#95558=CARTESIAN_POINT('Ctrl Pts',(-18.5061529523948,51.3749083698181,124.211091751246)) ;
#95559=CARTESIAN_POINT('Ctrl Pts',(-18.3825894276694,51.3847753539789,124.044441773673)) ;
#95560=CARTESIAN_POINT('Ctrl Pts',(-18.288197267175,51.3947809202316,123.856492625025)) ;
#95561=CARTESIAN_POINT('Ctrl Pts',(-18.2280368488677,51.4047647086462,123.655369961215)) ;
#95562=CARTESIAN_POINT('Ctrl Pts',(-18.2037955447711,51.4148105654489,123.445587221076)) ;
#95563=CARTESIAN_POINT('Ctrl Pts',(-18.2158049400224,51.4246364426648,123.239365717477)) ;
#95564=CARTESIAN_POINT('Ctrl Pts',(-18.2635681718687,51.4346269185061,123.034837448249)) ;
#95565=CARTESIAN_POINT('Ctrl Pts',(-18.3470677335809,51.4446704944049,122.840901106001)) ;
#95566=CARTESIAN_POINT('Ctrl Pts',(-18.4600500292513,51.454492286703,122.668070699184)) ;
#95567=CARTESIAN_POINT('Ctrl Pts',(-18.6040154233207,51.4645272523288,122.51386005426)) ;
#95568=CARTESIAN_POINT('Ctrl Pts',(-18.7727580993655,51.4745521692619,122.387582243707)) ;
#95569=CARTESIAN_POINT('Ctrl Pts',(-18.9574116237924,51.484404107638,122.293758448253)) ;
#95570=CARTESIAN_POINT('Ctrl Pts',(-19.1582249069468,51.4943950836628,122.232272282288)) ;
#95571=CARTESIAN_POINT('Ctrl Pts',(-19.365173365588,51.5043129044664,122.20663047978)) ;
#95572=CARTESIAN_POINT('Ctrl Pts',(-19.5757113223788,51.514341625031,122.217393834986)) ;
#95573=CARTESIAN_POINT('Ctrl Pts',(-19.7782673487064,51.5242245516402,122.263734531426)) ;
#95574=CARTESIAN_POINT('Ctrl Pts',(-19.9721412615777,51.5342288367597,122.34520873911)) ;
#95575=CARTESIAN_POINT('Ctrl Pts',(-20.1485965785602,51.5442125179675,122.458925892081)) ;
#95576=CARTESIAN_POINT('Ctrl Pts',(-20.3033084560046,51.5542535166975,122.602515950188)) ;
#95577=CARTESIAN_POINT('Ctrl Pts',(-20.4283341927033,51.5640859615646,122.767130736313)) ;
#95578=CARTESIAN_POINT('Ctrl Pts',(-20.5249880222564,51.5740809599949,122.953701578692)) ;
#95579=CARTESIAN_POINT('Ctrl Pts',(-20.5875824486003,51.5841125087445,123.155104791441)) ;
#95580=CARTESIAN_POINT('Ctrl Pts',(-20.6140701868961,51.59397788705,123.360796238698)) ;
#95581=CARTESIAN_POINT('Ctrl Pts',(-20.6049369881444,51.6039397345103,123.570032779427)) ;
#95582=CARTESIAN_POINT('Ctrl Pts',(-20.5589475424587,51.6139746753246,123.775913423477)) ;
#95583=CARTESIAN_POINT('Ctrl Pts',(-20.4794278297561,51.6238596363417,123.96794213985)) ;
#95584=CARTESIAN_POINT('Ctrl Pts',(-20.3657283834297,51.6339252452606,124.146371557226)) ;
#95585=CARTESIAN_POINT('Ctrl Pts',(-20.2260994109044,51.6437644203022,124.299028749051)) ;
#95586=CARTESIAN_POINT('Ctrl Pts',(-20.0585850388737,51.6538269758022,124.428181896307)) ;
#95587=CARTESIAN_POINT('Ctrl Pts',(-19.8741335395331,51.6637241504951,124.524491581243)) ;
#95588=CARTESIAN_POINT('Ctrl Pts',(-19.6753166265995,51.6736548654184,124.588188265683)) ;
#95589=CARTESIAN_POINT('Ctrl Pts',(-19.4660674185624,51.683698893496,124.616477182508)) ;
#95590=CARTESIAN_POINT('Ctrl Pts',(-19.2583751492451,51.6935850953493,124.60829874282)) ;
#95591=CARTESIAN_POINT('Ctrl Pts',(-19.0530285341832,51.7035782618161,124.56402336225)) ;
#95592=CARTESIAN_POINT('Ctrl Pts',(-18.8594658749353,51.7135177328034,124.485230506411)) ;
#95593=CARTESIAN_POINT('Ctrl Pts',(-18.6811715817189,51.7235342471575,124.373224323027)) ;
#95594=CARTESIAN_POINT('Ctrl Pts',(-18.526225601504,51.7334642736344,124.233278631899)) ;
#95595=CARTESIAN_POINT('Ctrl Pts',(-18.3964520613895,51.7435168091438,124.0665028494)) ;
#95596=CARTESIAN_POINT('Ctrl Pts',(-18.2995181598263,51.7533632123635,123.883591037165)) ;
#95597=CARTESIAN_POINT('Ctrl Pts',(-18.2344303622224,51.7633252552176,123.684540710865)) ;
#95598=CARTESIAN_POINT('Ctrl Pts',(-18.2049633399143,51.7733538060082,123.475764330925)) ;
#95599=CARTESIAN_POINT('Ctrl Pts',(-18.2120381052475,51.7832641317259,123.267547741061)) ;
#95600=CARTESIAN_POINT('Ctrl Pts',(-18.2547347214392,51.7931990435554,123.063088648168)) ;
#95601=CARTESIAN_POINT('Ctrl Pts',(-18.3332871597924,51.8032400503235,122.86716129288)) ;
#95602=CARTESIAN_POINT('Ctrl Pts',(-18.442855514963,51.8131276831557,122.690501450574)) ;
#95603=CARTESIAN_POINT('Ctrl Pts',(-18.5825823298511,51.8231181142538,122.533706140694)) ;
#95604=CARTESIAN_POINT('Ctrl Pts',(-18.7469172782873,51.833073550811,122.404087562565)) ;
#95605=CARTESIAN_POINT('Ctrl Pts',(-18.9302413211217,51.8429844989103,122.305087008928)) ;
#95606=CARTESIAN_POINT('Ctrl Pts',(-19.1299410908847,51.852996575008,122.238509434989)) ;
#95607=CARTESIAN_POINT('Ctrl Pts',(-19.3385091660018,51.863023897083,122.207996699255)) ;
#95608=CARTESIAN_POINT('Ctrl Pts',(-19.5457346779231,51.8728826720372,122.213537180948)) ;
#95609=CARTESIAN_POINT('Ctrl Pts',(-19.8221907089886,51.8863088648496,122.27018561231)) ;
#95610=CARTESIAN_POINT('Ctrl Pts',(-20.0713995852697,51.899392880631,122.394141621416)) ;
#95611=CARTESIAN_POINT('Ctrl Pts',(-20.2838395735766,51.9128663293862,122.581345072923)) ;
#95612=CARTESIAN_POINT('Ctrl Pts',(-20.4126502387728,51.9226992871921,122.74307239301)) ;
#95613=CARTESIAN_POINT('Ctrl Pts',(-20.5134840256695,51.9326625606427,122.92664557816)) ;
#95614=CARTESIAN_POINT('Ctrl Pts',(-20.5809847507344,51.9426996344607,123.126566404722)) ;
#95615=CARTESIAN_POINT('Ctrl Pts',(-20.6126263109704,51.9525746374723,123.331769641933)) ;
#95616=CARTESIAN_POINT('Ctrl Pts',(-20.6080629074932,51.9626423170985,123.543345669984)) ;
#95617=CARTESIAN_POINT('Ctrl Pts',(-20.5678682681263,51.9724831673162,123.746313051267)) ;
#95618=CARTESIAN_POINT('Ctrl Pts',(-20.4670270183732,51.9858193657922,124.007904980157)) ;
#95619=CARTESIAN_POINT('Ctrl Pts',(-20.3015603831813,51.9990368896066,124.235140214784)) ;
#95620=CARTESIAN_POINT('Ctrl Pts',(-20.0837896046647,52.0123718160979,124.411582727351)) ;
#95621=CARTESIAN_POINT('Ctrl Pts',(-19.9002558485253,52.0223549166925,124.513471552646)) ;
#95622=CARTESIAN_POINT('Ctrl Pts',(-19.7005524850227,52.0323996925921,124.58204856447)) ;
#95623=CARTESIAN_POINT('Ctrl Pts',(-19.496714337372,52.042217615778,124.614579101692)) ;
#95624=CARTESIAN_POINT('Ctrl Pts',(-19.2854774239128,52.0522669297334,124.611577325048)) ;
#95625=CARTESIAN_POINT('Ctrl Pts',(-19.010863063282,52.0655706703559,124.55854219251)) ;
#95626=CARTESIAN_POINT('Ctrl Pts',(-18.6949728829699,52.0820608658326,124.40631133582)) ;
#95627=CARTESIAN_POINT('Ctrl Pts',(-18.4467434896524,52.0987800307572,124.151888767484)) ;
#95628=CARTESIAN_POINT('Ctrl Pts',(-18.3113738584945,52.1119410244274,123.910570859981)) ;
#95629=CARTESIAN_POINT('Ctrl Pts',(-18.2412220212376,52.1219372465326,123.712480323946)) ;
#95630=CARTESIAN_POINT('Ctrl Pts',(-18.2069072492689,52.1319610860664,123.504562137768)) ;
#95631=CARTESIAN_POINT('Ctrl Pts',(-18.2093339154971,52.1451544080596,123.227174122353)) ;
#95632=CARTESIAN_POINT('Ctrl Pts',(-18.3035482568181,52.1618135798369,122.885761894292)) ;
#95633=CARTESIAN_POINT('Ctrl Pts',(-18.549002308558,52.1817237553226,122.540816602252)) ;
#95634=CARTESIAN_POINT('Ctrl Pts',(-18.8966024948958,52.201613743167,122.299840239529)) ;
#95635=CARTESIAN_POINT('Ctrl Pts',(-19.3079252637735,52.2216191911818,122.191722536724)) ;
#95636=CARTESIAN_POINT('Ctrl Pts',(-19.7281008697902,52.2414555852091,122.22971345726)) ;
#95637=CARTESIAN_POINT('Ctrl Pts',(-20.1132537936542,52.2614633791058,122.410106100044)) ;
#95638=CARTESIAN_POINT('Ctrl Pts',(-20.4112473017471,52.2812900153998,122.708408638474)) ;
#95639=CARTESIAN_POINT('Ctrl Pts',(-20.5915866931826,52.3012689583536,123.093018147004)) ;
#95640=CARTESIAN_POINT('Ctrl Pts',(-20.6290084909863,52.3212007602227,123.515109886166)) ;
#95641=CARTESIAN_POINT('Ctrl Pts',(-20.5220590647266,52.3410250607202,123.922971194583)) ;
#95642=CARTESIAN_POINT('Ctrl Pts',(-20.2786176342575,52.3611210620601,124.273924800819)) ;
#95643=CARTESIAN_POINT('Ctrl Pts',(-19.9358038633672,52.380879478164,124.517203259655)) ;
#95644=CARTESIAN_POINT('Ctrl Pts',(-19.5241772246425,52.4009731710481,124.630789980782)) ;
#95645=CARTESIAN_POINT('Ctrl Pts',(-19.2461498309204,52.4140841369548,124.608685679991)) ;
#95646=CARTESIAN_POINT('Ctrl Pts',(-19.1099523892177,52.4207975117427,124.573829556462)) ;
#95647=CARTESIAN_POINT('',(-18.2012080090896,13.6718523192586,123.050973081965)) ;
#95648=CARTESIAN_POINT('Ctrl Pts',(-18.9360879628692,13.6947924667251,122.292840803596)) ;
#95649=CARTESIAN_POINT('Ctrl Pts',(-18.8235714014898,13.6922154699032,122.334824139467)) ;
#95650=CARTESIAN_POINT('Ctrl Pts',(-18.717918507247,13.6896773479738,122.393380734364)) ;
#95651=CARTESIAN_POINT('Ctrl Pts',(-18.5046219362228,13.6839804037588,122.555810931824)) ;
#95652=CARTESIAN_POINT('Ctrl Pts',(-18.4238036284642,13.6814287159771,122.651100591995)) ;
#95653=CARTESIAN_POINT('Ctrl Pts',(-18.3231340641736,13.6778224757191,122.790090499525)) ;
#95654=CARTESIAN_POINT('Ctrl Pts',(-18.2820702591376,13.6761482722924,122.860450448584)) ;
#95655=CARTESIAN_POINT('Ctrl Pts',(-18.2300500481297,13.6735665071738,122.973308264649)) ;
#95656=CARTESIAN_POINT('Ctrl Pts',(-18.2145001079492,13.6726943420554,123.012358669986)) ;
#95657=CARTESIAN_POINT('Ctrl Pts',(-18.2012080090896,13.6718523192586,123.050973081965)) ;
#95658=CARTESIAN_POINT('Ctrl Pts',(-18.2012080090896,13.6718523192586,123.050973081965)) ;
#95659=CARTESIAN_POINT('Ctrl Pts',(-18.1581996061038,13.6691278393889,123.175915290792)) ;
#95660=CARTESIAN_POINT('Ctrl Pts',(-18.1387937958945,13.6666598154068,123.296279415935)) ;
#95661=CARTESIAN_POINT('Ctrl Pts',(-18.1257612025128,13.661023496104,123.570342737487)) ;
#95662=CARTESIAN_POINT('Ctrl Pts',(-18.1508137569076,13.6577012237818,123.737417962333)) ;
#95663=CARTESIAN_POINT('Ctrl Pts',(-18.2352191601102,13.6526511564216,123.974578239407)) ;
#95664=CARTESIAN_POINT('Ctrl Pts',(-18.2712831463275,13.6509739277543,124.051197325921)) ;
#95665=CARTESIAN_POINT('Ctrl Pts',(-18.3579770185685,13.6475919378534,124.196910378393)) ;
#95666=CARTESIAN_POINT('Ctrl Pts',(-18.4086013486671,13.6458822226032,124.265780153595)) ;
#95667=CARTESIAN_POINT('Ctrl Pts',(-18.5223724110274,13.6425352830893,124.392419038975)) ;
#95668=CARTESIAN_POINT('Ctrl Pts',(-18.5854306417936,13.6408892425574,124.450124298751)) ;
#95669=CARTESIAN_POINT('Ctrl Pts',(-18.7230337869855,13.6374586642957,124.554029585411)) ;
#95670=CARTESIAN_POINT('Ctrl Pts',(-18.7977853498151,13.6357466098985,124.599582194036)) ;
#95671=CARTESIAN_POINT('Ctrl Pts',(-18.9542303094569,13.6324211081276,124.674756173776)) ;
#95672=CARTESIAN_POINT('Ctrl Pts',(-19.0352628167113,13.6307370012966,124.704593618465)) ;
#95673=CARTESIAN_POINT('Ctrl Pts',(-19.203949871872,13.6273270305868,124.748915542086)) ;
#95674=CARTESIAN_POINT('Ctrl Pts',(-19.2914050956568,13.6256576319658,124.762774348756)) ;
#95675=CARTESIAN_POINT('Ctrl Pts',(-19.4687754438232,13.62226745034,124.773437732167)) ;
#95676=CARTESIAN_POINT('Ctrl Pts',(-19.5581411015172,13.6205446496771,124.77006951148)) ;
#95677=CARTESIAN_POINT('Ctrl Pts',(-19.7354306126231,13.6171441040415,124.745652632289)) ;
#95678=CARTESIAN_POINT('Ctrl Pts',(-19.822565001308,13.6154427854294,124.724844993805)) ;
#95679=CARTESIAN_POINT('Ctrl Pts',(-20.0764731495327,13.6103641080683,124.637307284215)) ;
#95680=CARTESIAN_POINT('Ctrl Pts',(-20.2329408847691,13.6070536493622,124.546357434949)) ;
#95681=CARTESIAN_POINT('Ctrl Pts',(-20.4370829945165,13.6019893485599,124.367567415324)) ;
#95682=CARTESIAN_POINT('Ctrl Pts',(-20.4996594996402,13.6002817418393,124.300939997901)) ;
#95683=CARTESIAN_POINT('Ctrl Pts',(-20.6683074370187,13.5952033913329,124.081669485175)) ;
#95684=CARTESIAN_POINT('Ctrl Pts',(-20.7512472957358,13.5918390838879,123.913926550694)) ;
#95685=CARTESIAN_POINT('Ctrl Pts',(-20.8485292133704,13.5850157442221,123.555907247786)) ;
#95686=CARTESIAN_POINT('Ctrl Pts',(-20.8615435921713,13.5817118196242,123.368766670857)) ;
#95687=CARTESIAN_POINT('Ctrl Pts',(-20.8277134344081,13.5766954025581,123.091458278734)) ;
#95688=CARTESIAN_POINT('Ctrl Pts',(-20.8071567516996,13.5750061219952,122.999086539571)) ;
#95689=CARTESIAN_POINT('Ctrl Pts',(-20.7484711008796,13.5716296807235,122.819618482393)) ;
#95690=CARTESIAN_POINT('Ctrl Pts',(-20.7104369116122,13.5699752678018,122.733015801732)) ;
#95691=CARTESIAN_POINT('Ctrl Pts',(-20.5904523188124,13.5656129119562,122.518345024356)) ;
#95692=CARTESIAN_POINT('Ctrl Pts',(-20.496859833978,13.5629586805197,122.398743249045)) ;
#95693=CARTESIAN_POINT('Ctrl Pts',(-20.3308891118335,13.5589725221892,122.242960467886)) ;
#95694=CARTESIAN_POINT('Ctrl Pts',(-20.2714146128716,13.5576281988933,122.195112314727)) ;
#95695=CARTESIAN_POINT('Ctrl Pts',(-20.1451496366424,13.554975483985,122.10873977592)) ;
#95696=CARTESIAN_POINT('Ctrl Pts',(-20.0784457854721,13.5536392537494,122.070280759549)) ;
#95697=CARTESIAN_POINT('Ctrl Pts',(-20.0093941796458,13.5522956097346,122.037202589381)) ;
#95698=CARTESIAN_POINT('Origin',(-19.4092696390756,14.2022556137854,123.41183365498)) ;
#95699=CARTESIAN_POINT('',(-18.4466282248614,13.7999200508426,123.124282652847)) ;
#95700=CARTESIAN_POINT('Origin',(-19.4092696390756,13.7999200508426,123.41183365498)) ;
#95701=CARTESIAN_POINT('',(-19.217636498755,14.2022556137854,123.354590842934)) ;
#95702=CARTESIAN_POINT('Origin',(-20.3808792107654,13.7999200508426,126.250138578733)) ;
#95703=CARTESIAN_POINT('',(-19.5760412740791,13.7999200508426,122.562017662105)) ;
#95704=CARTESIAN_POINT('',(-18.7566932181948,13.7999200508426,122.84249718599)) ;
#95705=CARTESIAN_POINT('',(-19.5760412740791,13.7999200508426,122.562017662105)) ;
#95706=CARTESIAN_POINT('',(-18.5899215831784,13.7999200508426,123.692313178869)) ;
#95707=CARTESIAN_POINT('',(-18.7566932181948,13.7999200508426,122.84249718599)) ;
#95708=CARTESIAN_POINT('',(-19.2424980040462,13.7999200508426,124.261649647864)) ;
#95709=CARTESIAN_POINT('',(-18.5899215831784,13.7999200508426,123.692313178869)) ;
#95710=CARTESIAN_POINT('',(-20.0618460599304,13.7999200508426,123.981170123979)) ;
#95711=CARTESIAN_POINT('',(-19.2424980040462,13.7999200508426,124.261649647864)) ;
#95712=CARTESIAN_POINT('',(-20.2286176949469,13.7999200508426,123.131354131099)) ;
#95713=CARTESIAN_POINT('',(-20.0618460599304,13.7999200508426,123.981170123979)) ;
#95714=CARTESIAN_POINT('',(-20.2286176949469,13.7999200508426,123.131354131099)) ;
#95715=CARTESIAN_POINT('Origin',(-19.5760412740791,15.3022556137854,122.562017662105)) ;
#95716=CARTESIAN_POINT('',(-19.5760412740791,12.9245228503138,122.562017662105)) ;
#95717=CARTESIAN_POINT('',(-19.5760412740791,13.7999200508426,122.562017662105)) ;
#95718=CARTESIAN_POINT('',(-18.7566932181948,12.9245228503138,122.84249718599)) ;
#95719=CARTESIAN_POINT('',(-19.5760412740791,12.9245228503138,122.562017662105)) ;
#95720=CARTESIAN_POINT('',(-18.7566932181948,13.7999200508426,122.84249718599)) ;
#95721=CARTESIAN_POINT('Origin',(-18.7566932181948,15.3022556137854,122.84249718599)) ;
#95722=CARTESIAN_POINT('',(-18.5899215831784,12.9245228503138,123.692313178869)) ;
#95723=CARTESIAN_POINT('',(-18.7566932181948,12.9245228503138,122.84249718599)) ;
#95724=CARTESIAN_POINT('',(-18.5899215831784,13.7999200508426,123.692313178869)) ;
#95725=CARTESIAN_POINT('Origin',(-18.5899215831784,15.3022556137854,123.692313178869)) ;
#95726=CARTESIAN_POINT('',(-19.2424980040462,12.9245228503138,124.261649647864)) ;
#95727=CARTESIAN_POINT('',(-18.5899215831784,12.9245228503138,123.692313178869)) ;
#95728=CARTESIAN_POINT('',(-19.2424980040462,13.7999200508426,124.261649647864)) ;
#95729=CARTESIAN_POINT('Origin',(-19.2424980040462,15.3022556137854,124.261649647864)) ;
#95730=CARTESIAN_POINT('',(-20.0618460599304,12.9245228503138,123.981170123979)) ;
#95731=CARTESIAN_POINT('',(-19.2424980040462,12.9245228503138,124.261649647864)) ;
#95732=CARTESIAN_POINT('',(-20.0618460599304,13.7999200508426,123.981170123979)) ;
#95733=CARTESIAN_POINT('Origin',(-20.0618460599304,15.3022556137854,123.981170123979)) ;
#95734=CARTESIAN_POINT('',(-20.2286176949469,12.9245228503138,123.131354131099)) ;
#95735=CARTESIAN_POINT('',(-20.0618460599304,12.9245228503138,123.981170123979)) ;
#95736=CARTESIAN_POINT('',(-20.2286176949469,13.7999200508426,123.131354131099)) ;
#95737=CARTESIAN_POINT('Origin',(-20.2286176949469,15.3022556137854,123.131354131099)) ;
#95738=CARTESIAN_POINT('',(-20.2286176949469,12.9245228503138,123.131354131099)) ;
#95739=CARTESIAN_POINT('Origin',(-19.5760412740791,12.9245228503138,122.562017662105)) ;
#196737=UNCERTAINTY_MEASURE_WITH_UNIT(LENGTH_MEASURE(0.01),#196742,
'DISTANCE_ACCURACY_VALUE',
'Maximum model space distance between geometric entities at asserted c
onnectivities') ;
#196738=UNCERTAINTY_MEASURE_WITH_UNIT(LENGTH_MEASURE(0.01),#196742,
'DISTANCE_ACCURACY_VALUE',
'Maximum model space distance between geometric entities at asserted c
onnectivities') ;
#196740=(
GEOMETRIC_REPRESENTATION_CONTEXT(3)
GLOBAL_UNCERTAINTY_ASSIGNED_CONTEXT((#196737))
GLOBAL_UNIT_ASSIGNED_CONTEXT((#196742,#196744,#196745))
REPRESENTATION_CONTEXT('','3D')
) ;
#196741=(
GEOMETRIC_REPRESENTATION_CONTEXT(3)
GLOBAL_UNCERTAINTY_ASSIGNED_CONTEXT((#196738))
GLOBAL_UNIT_ASSIGNED_CONTEXT((#196742,#196744,#196745))
REPRESENTATION_CONTEXT('','3D')
) ;
#196742=(
LENGTH_UNIT()
NAMED_UNIT(*)
SI_UNIT(.MILLI.,.METRE.)
) ;
#196744=(
NAMED_UNIT(*)
PLANE_ANGLE_UNIT()
SI_UNIT($,.RADIAN.)
) ;
#196745=(
NAMED_UNIT(*)
SI_UNIT($,.STERADIAN.)
SOLID_ANGLE_UNIT()
) ;
#196753=PRODUCT_DEFINITION_CONTEXT('part definition',#196761,'design') ;
#196761=APPLICATION_CONTEXT(
'Core Data for Automotive Mechanical Design Process') ;
#196762=PRODUCT_CONTEXT('part definition',#196761,'mechanical') ;
#196765=PRESENTATION_STYLE_ASSIGNMENT((#196767)) ;
#196767=SURFACE_STYLE_USAGE(.BOTH.,#196769) ;
#196769=SURFACE_SIDE_STYLE('',(#196771)) ;
#196771=SURFACE_STYLE_FILL_AREA(#196773) ;
#196773=FILL_AREA_STYLE('Steel - Satin',(#196775)) ;
#196775=FILL_AREA_STYLE_COLOUR('Steel - Satin',#196777) ;
#196777=COLOUR_RGB('Steel - Satin', 0.09019608, 0.27058824, 0.51372549) ;
#196875=CARTESIAN_POINT ( '', ( 0.0, 0.0, 0.0 ) ) ;
#196876=DIRECTION ( '', ( 0.0, 0.0, 1.0 ) ) ;
#196877=DIRECTION ( '', ( 1.0, 0.0, 0.0 ) ) ;
#196878=AXIS2_PLACEMENT_3D ( '', #196875, #196876, #196877 ) ;
#196879=ADVANCED_BREP_SHAPE_REPRESENTATION ( 'Pivot Collar', ( #342, #196878, #196889, #197290, #197485 ), #196740 ) ;
#196880=PRODUCT( 'Pivot Collar', 'Pivot Collar', '', ( #196762 ) ) ;
#196881=PRODUCT_DEFINITION_FORMATION ( '', '', #196880 ) ;
#196882=PRODUCT_DEFINITION( 'Pivot Collar', 'Pivot Collar', #196881, #196753 ) ;
#196883=PRODUCT_DEFINITION_SHAPE ( '', '', #196882 ) ;
#196884=SHAPE_DEFINITION_REPRESENTATION ( #196883, #196879 ) ;
#196886=CARTESIAN_POINT ( '', ( 0.0, 0.0, 0.0 ) ) ;
#196887=DIRECTION ( '', ( 0.0, 0.0, 1.0 ) ) ;
#196888=DIRECTION ( '', ( 1.0, 0.0, 0.0 ) ) ;
#196889=AXIS2_PLACEMENT_3D ( '', #196886, #196887, #196888 ) ;
#197287=CARTESIAN_POINT ( '', ( 0.0, 0.0, 0.0 ) ) ;
#197288=DIRECTION ( '', ( 0.0, 0.0, 1.0 ) ) ;
#197289=DIRECTION ( '', ( 1.0, 0.0, 0.0 ) ) ;
#197290=AXIS2_PLACEMENT_3D ( '', #197287, #197288, #197289 ) ;
#197482=CARTESIAN_POINT ( '', ( 0.0, 0.0, 0.0 ) ) ;
#197483=DIRECTION ( '', ( 0.0, 0.0, 1.0 ) ) ;
#197484=DIRECTION ( '', ( 1.0, 0.0, 0.0 ) ) ;
#197485=AXIS2_PLACEMENT_3D ( '', #197482, #197483, #197484 ) ;
ENDSEC;
END-ISO-10303-21;
